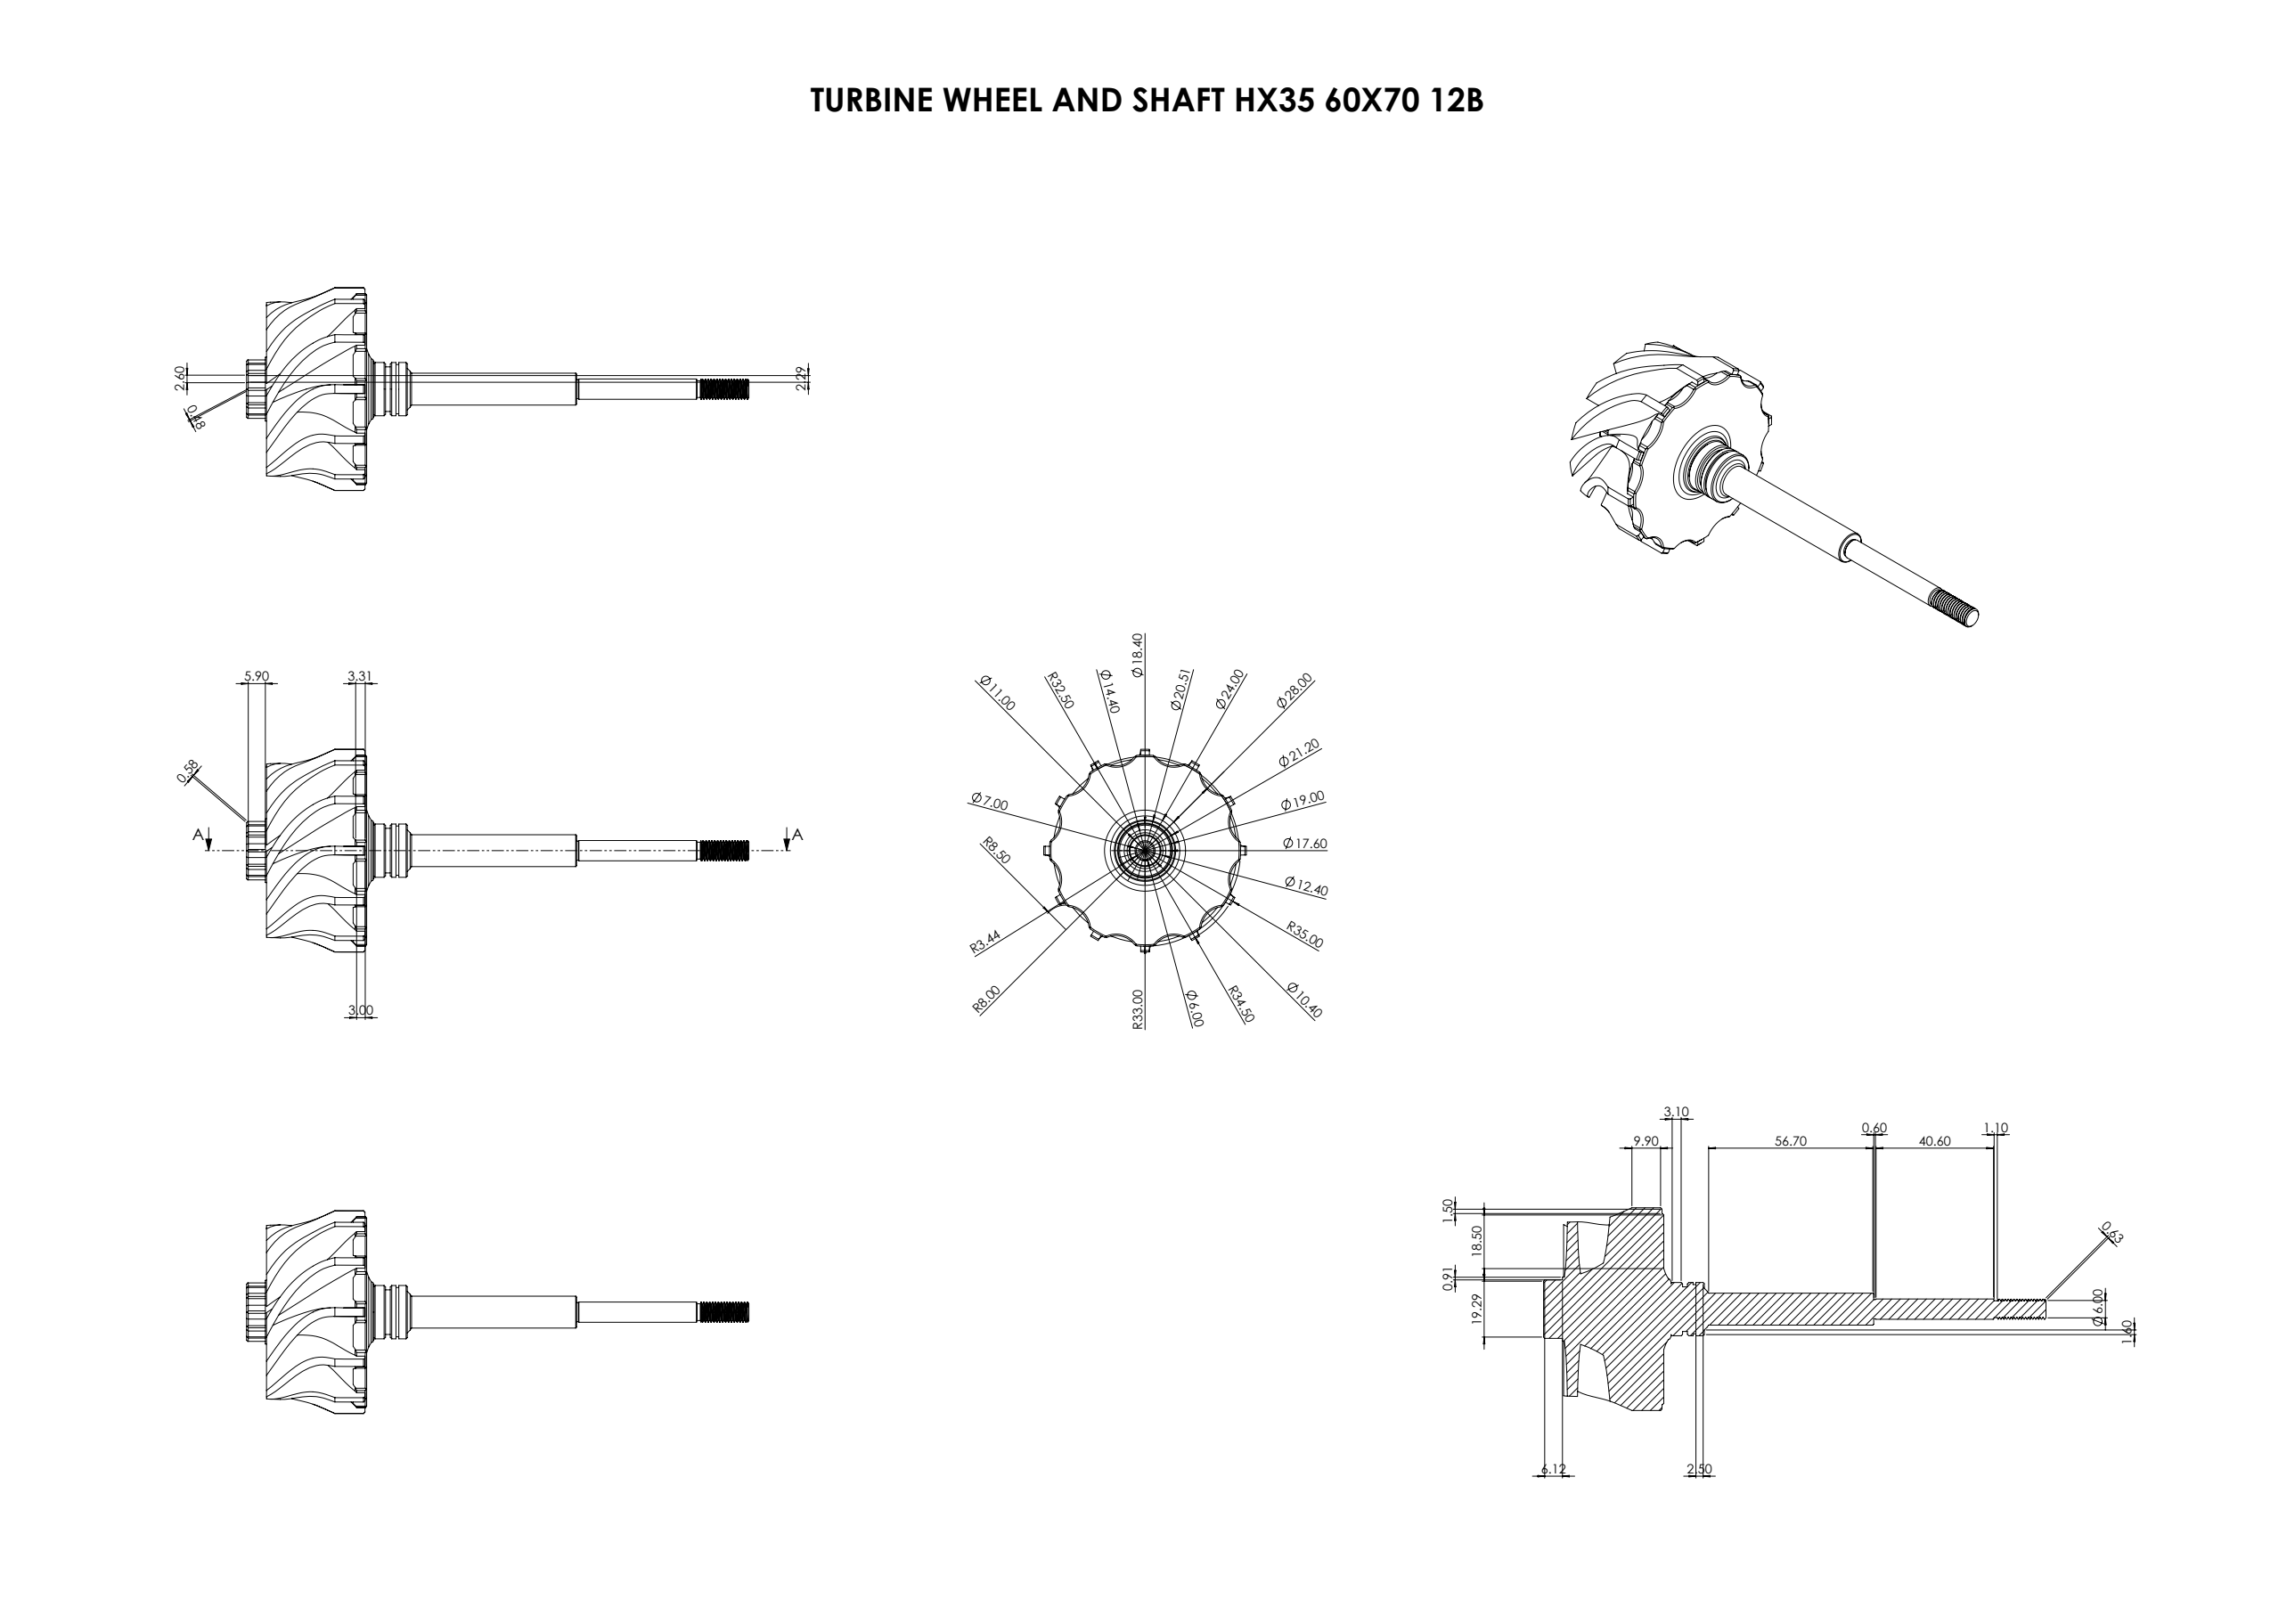
ISO-10303-21;
HEADER;
/* Generated by software containing ST-Developer
 * from STEP Tools, Inc. (www.steptools.com) 
 */

FILE_DESCRIPTION(
/* description */ (''),
/* implementation_level */ '2;1');

FILE_NAME(
/* name */ '01_Turbine_Wheel_and_Shaft_HX35_60x70_12B.step',
/* time_stamp */ '2026-10-25T01:10:36-07:00',
/* author */ (''),
/* organization */ (''),
/* preprocessor_version */ 'ST-DEVELOPER v20.2',
/* originating_system */ 'Autodesk Translation Framework v15.15.0.0',
/* authorisation */ '');

FILE_SCHEMA (('AUTOMOTIVE_DESIGN { 1 0 10303 214 3 1 1 }'));
ENDSEC;

DATA;
#10=MECHANICAL_DESIGN_GEOMETRIC_PRESENTATION_REPRESENTATION('',(#1098,#1099,#1100,#1101,#1102,#1103,#1104,#1105,#1106,#1107,#1108,#1109,#1110,#1111,#1112,#1113,#1114,#1115,#1116,#1117,#1118,#1119,#1120,#1121,#1122,#1123,#1124,#1125,#1126,#1127,#1128,#1129,#1130,#1131,#1132,#1133,#1134,#1135,#1136,#1137,#1138,#1139,#1140,#1141,#1142,#1143,#1144,#1145,#1146,#1147,#1148,#1149,#1150,#1151,#1152,#1153,#1154,#1155,#1156,#1157,#1158,#1159,#1160,#1161,#1162,#1163,#1164,#1165,#1166,#1167,#1168,#1169,#1170,#1171,#1172,#1173,#1174,#1175,#1176,#1177,#1178,#1179,#1180,#1181,#1182,#1183,#1184,#1185,#1186,#1187,#1188,#1189,#1190,#1191,#1192,#1193,#1194,#1195,#1196,#1197,#1198,#1199,#1200,#1201,#1202,#1203,#1204,#1205,#1206,#1207,#1208,#1209,#1210,#1211,#1212,#1213,#1214,#1215,#1216,#1217,#1218,#1219,#1220,#1221,#1222,#1223,#1224,#1225,#1226,#1227,#1228,#1229,#1230,#1231,#1232,#1233,#1234,#1235,#1236,#1237,#1238,#1239,#1240,#1241,#1242,#1243,#1244,#1245,#1246,#1247,#1248,#1249,#1250,#1251,#1252,#1253,#1254,#1255,#1256,#1257,#1258,#1259,#1260,#1261,#1262,#1263,#1264,#1265,#1266,#1267,#1268,#1269,#1270,#1271,#1272,#1273,#1274,#1275,#1276,#1277,#1278,#1279,#1280,#1281,#1282,#1283,#1284,#1285,#1286,#1287,#1288,#1289,#1290,#1291,#1292,#1293,#1294,#1295),#60365);
#67=SHAPE_REPRESENTATION_RELATIONSHIP('SRR','None',#60407,#77);
#77=ADVANCED_BREP_SHAPE_REPRESENTATION('',(#87),#60355);
#87=MANIFOLD_SOLID_BREP('Body1',#18297);
#97=B_SPLINE_SURFACE_WITH_KNOTS('',3,3,((#27482,#27483,#27484,#27485,#27486,
#27487,#27488,#27489,#27490,#27491,#27492,#27493,#27494,#27495,#27496,#27497,
#27498,#27499,#27500,#27501,#27502,#27503,#27504,#27505,#27506,#27507,#27508,
#27509,#27510,#27511,#27512,#27513,#27514,#27515,#27516,#27517,#27518,#27519,
#27520,#27521,#27522,#27523),(#27524,#27525,#27526,#27527,#27528,#27529,
#27530,#27531,#27532,#27533,#27534,#27535,#27536,#27537,#27538,#27539,#27540,
#27541,#27542,#27543,#27544,#27545,#27546,#27547,#27548,#27549,#27550,#27551,
#27552,#27553,#27554,#27555,#27556,#27557,#27558,#27559,#27560,#27561,#27562,
#27563,#27564,#27565),(#27566,#27567,#27568,#27569,#27570,#27571,#27572,
#27573,#27574,#27575,#27576,#27577,#27578,#27579,#27580,#27581,#27582,#27583,
#27584,#27585,#27586,#27587,#27588,#27589,#27590,#27591,#27592,#27593,#27594,
#27595,#27596,#27597,#27598,#27599,#27600,#27601,#27602,#27603,#27604,#27605,
#27606,#27607),(#27608,#27609,#27610,#27611,#27612,#27613,#27614,#27615,
#27616,#27617,#27618,#27619,#27620,#27621,#27622,#27623,#27624,#27625,#27626,
#27627,#27628,#27629,#27630,#27631,#27632,#27633,#27634,#27635,#27636,#27637,
#27638,#27639,#27640,#27641,#27642,#27643,#27644,#27645,#27646,#27647,#27648,
#27649),(#27650,#27651,#27652,#27653,#27654,#27655,#27656,#27657,#27658,
#27659,#27660,#27661,#27662,#27663,#27664,#27665,#27666,#27667,#27668,#27669,
#27670,#27671,#27672,#27673,#27674,#27675,#27676,#27677,#27678,#27679,#27680,
#27681,#27682,#27683,#27684,#27685,#27686,#27687,#27688,#27689,#27690,#27691)),
 .UNSPECIFIED.,.F.,.F.,.F.,(4,1,4),(4,2,2,2,2,2,1,1,2,1,1,1,1,1,1,2,1,2,
1,1,1,1,2,1,1,1,1,1,1,1,4),(0.10381731230502,0.585202227283102,0.946240913516665),
(0.0903575719412648,0.100793262783688,0.212043315812054,0.313257792411489,
0.405143101782566,0.488664067632647,0.50778607271066,0.526908077788674,
0.565152087944702,0.574062129417373,0.582972170890044,0.600792253835385,
0.618612336780727,0.627522378253398,0.631977398989734,0.636432419726069,
0.66210667165326,0.704897091531912,0.716247203396069,0.727597315260226,
0.736109899158344,0.750297538988541,0.79569798644517,0.806906221911025,
0.815312398510416,0.81811445737688,0.840530928308591,0.851739163774446,
0.874155634706157,0.885363870172012,0.975029753898854),.UNSPECIFIED.);
#98=B_SPLINE_SURFACE_WITH_KNOTS('',3,3,((#27985,#27986,#27987,#27988,#27989,
#27990,#27991,#27992,#27993,#27994,#27995,#27996,#27997,#27998,#27999,#28000,
#28001,#28002,#28003,#28004,#28005,#28006,#28007,#28008,#28009,#28010,#28011,
#28012,#28013,#28014,#28015,#28016,#28017,#28018,#28019,#28020,#28021,#28022),
(#28023,#28024,#28025,#28026,#28027,#28028,#28029,#28030,#28031,#28032,
#28033,#28034,#28035,#28036,#28037,#28038,#28039,#28040,#28041,#28042,#28043,
#28044,#28045,#28046,#28047,#28048,#28049,#28050,#28051,#28052,#28053,#28054,
#28055,#28056,#28057,#28058,#28059,#28060),(#28061,#28062,#28063,#28064,
#28065,#28066,#28067,#28068,#28069,#28070,#28071,#28072,#28073,#28074,#28075,
#28076,#28077,#28078,#28079,#28080,#28081,#28082,#28083,#28084,#28085,#28086,
#28087,#28088,#28089,#28090,#28091,#28092,#28093,#28094,#28095,#28096,#28097,
#28098),(#28099,#28100,#28101,#28102,#28103,#28104,#28105,#28106,#28107,
#28108,#28109,#28110,#28111,#28112,#28113,#28114,#28115,#28116,#28117,#28118,
#28119,#28120,#28121,#28122,#28123,#28124,#28125,#28126,#28127,#28128,#28129,
#28130,#28131,#28132,#28133,#28134,#28135,#28136),(#28137,#28138,#28139,
#28140,#28141,#28142,#28143,#28144,#28145,#28146,#28147,#28148,#28149,#28150,
#28151,#28152,#28153,#28154,#28155,#28156,#28157,#28158,#28159,#28160,#28161,
#28162,#28163,#28164,#28165,#28166,#28167,#28168,#28169,#28170,#28171,#28172,
#28173,#28174)),.UNSPECIFIED.,.F.,.F.,.F.,(4,1,4),(4,2,2,2,2,2,1,1,2,1,
1,1,1,1,2,1,2,1,1,1,2,1,1,1,1,1,4),(0.10381731230502,0.464855998538582,
0.946240913516665),(0.0903575719412648,0.100793262783688,0.212043315812054,
0.313257792411489,0.405143101782566,0.488664067632647,0.50778607271066,
0.526908077788674,0.565152087944702,0.574062129417373,0.582972170890044,
0.600792253835385,0.609702295308056,0.618612336780727,0.636432419726069,
0.65354858767753,0.704897091531912,0.716247203396069,0.727597315260226,
0.750297538988541,0.79569798644517,0.806906221911025,0.81811445737688,0.840530928308591,
0.862947399240301,0.885363870172012,0.975029753898854),.UNSPECIFIED.);
#99=B_SPLINE_SURFACE_WITH_KNOTS('',3,3,((#28427,#28428,#28429,#28430,#28431,
#28432,#28433,#28434,#28435,#28436,#28437,#28438,#28439,#28440,#28441,#28442,
#28443,#28444,#28445,#28446,#28447,#28448,#28449,#28450,#28451,#28452,#28453,
#28454,#28455,#28456,#28457,#28458,#28459,#28460,#28461,#28462,#28463,#28464,
#28465,#28466,#28467,#28468,#28469,#28470),(#28471,#28472,#28473,#28474,
#28475,#28476,#28477,#28478,#28479,#28480,#28481,#28482,#28483,#28484,#28485,
#28486,#28487,#28488,#28489,#28490,#28491,#28492,#28493,#28494,#28495,#28496,
#28497,#28498,#28499,#28500,#28501,#28502,#28503,#28504,#28505,#28506,#28507,
#28508,#28509,#28510,#28511,#28512,#28513,#28514),(#28515,#28516,#28517,
#28518,#28519,#28520,#28521,#28522,#28523,#28524,#28525,#28526,#28527,#28528,
#28529,#28530,#28531,#28532,#28533,#28534,#28535,#28536,#28537,#28538,#28539,
#28540,#28541,#28542,#28543,#28544,#28545,#28546,#28547,#28548,#28549,#28550,
#28551,#28552,#28553,#28554,#28555,#28556,#28557,#28558),(#28559,#28560,
#28561,#28562,#28563,#28564,#28565,#28566,#28567,#28568,#28569,#28570,#28571,
#28572,#28573,#28574,#28575,#28576,#28577,#28578,#28579,#28580,#28581,#28582,
#28583,#28584,#28585,#28586,#28587,#28588,#28589,#28590,#28591,#28592,#28593,
#28594,#28595,#28596,#28597,#28598,#28599,#28600,#28601,#28602),(#28603,
#28604,#28605,#28606,#28607,#28608,#28609,#28610,#28611,#28612,#28613,#28614,
#28615,#28616,#28617,#28618,#28619,#28620,#28621,#28622,#28623,#28624,#28625,
#28626,#28627,#28628,#28629,#28630,#28631,#28632,#28633,#28634,#28635,#28636,
#28637,#28638,#28639,#28640,#28641,#28642,#28643,#28644,#28645,#28646)),
 .UNSPECIFIED.,.F.,.F.,.F.,(4,1,4),(4,2,2,2,2,2,1,1,1,2,1,1,1,1,1,1,1,2,
1,2,1,1,1,1,1,2,1,1,1,1,1,1,4),(0.10381731230502,0.464855998538582,0.946240913516665),
(0.0903575719412648,0.100793262783688,0.212043315812054,0.313257792411489,
0.405143101782566,0.488664067632647,0.50778607271066,0.526908077788674,
0.546030082866688,0.565152087944702,0.574062129417373,0.582972170890044,
0.600792253835385,0.609702295308056,0.618612336780727,0.627522378253398,
0.631977398989734,0.636432419726069,0.670664755628991,0.704897091531912,
0.71057214746399,0.716247203396069,0.727597315260226,0.738947427124383,
0.750297538988541,0.79569798644517,0.806906221911025,0.81811445737688,0.829322692842735,
0.840530928308591,0.862947399240301,0.885363870172012,0.975029753898854),
 .UNSPECIFIED.);
#100=B_SPLINE_SURFACE_WITH_KNOTS('',3,3,((#28899,#28900,#28901,#28902,#28903,
#28904,#28905,#28906,#28907,#28908,#28909,#28910,#28911,#28912,#28913,#28914,
#28915,#28916,#28917,#28918,#28919,#28920,#28921,#28922,#28923,#28924,#28925,
#28926,#28927,#28928,#28929,#28930,#28931,#28932,#28933,#28934,#28935,#28936,
#28937,#28938,#28939,#28940),(#28941,#28942,#28943,#28944,#28945,#28946,
#28947,#28948,#28949,#28950,#28951,#28952,#28953,#28954,#28955,#28956,#28957,
#28958,#28959,#28960,#28961,#28962,#28963,#28964,#28965,#28966,#28967,#28968,
#28969,#28970,#28971,#28972,#28973,#28974,#28975,#28976,#28977,#28978,#28979,
#28980,#28981,#28982),(#28983,#28984,#28985,#28986,#28987,#28988,#28989,
#28990,#28991,#28992,#28993,#28994,#28995,#28996,#28997,#28998,#28999,#29000,
#29001,#29002,#29003,#29004,#29005,#29006,#29007,#29008,#29009,#29010,#29011,
#29012,#29013,#29014,#29015,#29016,#29017,#29018,#29019,#29020,#29021,#29022,
#29023,#29024),(#29025,#29026,#29027,#29028,#29029,#29030,#29031,#29032,
#29033,#29034,#29035,#29036,#29037,#29038,#29039,#29040,#29041,#29042,#29043,
#29044,#29045,#29046,#29047,#29048,#29049,#29050,#29051,#29052,#29053,#29054,
#29055,#29056,#29057,#29058,#29059,#29060,#29061,#29062,#29063,#29064,#29065,
#29066),(#29067,#29068,#29069,#29070,#29071,#29072,#29073,#29074,#29075,
#29076,#29077,#29078,#29079,#29080,#29081,#29082,#29083,#29084,#29085,#29086,
#29087,#29088,#29089,#29090,#29091,#29092,#29093,#29094,#29095,#29096,#29097,
#29098,#29099,#29100,#29101,#29102,#29103,#29104,#29105,#29106,#29107,#29108)),
 .UNSPECIFIED.,.F.,.F.,.F.,(4,1,4),(4,2,2,2,2,2,1,1,2,1,1,1,1,1,1,2,1,2,
1,1,1,1,2,1,1,1,1,1,1,1,4),(0.10381731230502,0.585202227283103,0.946240913516665),
(0.0903575719412648,0.100793262783688,0.212043315812054,0.313257792411489,
0.405143101782566,0.488664067632647,0.50778607271066,0.526908077788674,
0.565152087944702,0.574062129417373,0.582972170890044,0.600792253835385,
0.618612336780727,0.627522378253398,0.631977398989734,0.636432419726069,
0.66210667165326,0.704897091531912,0.716247203396069,0.727597315260226,
0.736109899158344,0.750297538988541,0.79569798644517,0.806906221911025,
0.815312398510416,0.81811445737688,0.840530928308591,0.851739163774446,
0.874155634706157,0.885363870172012,0.975029753898854),.UNSPECIFIED.);
#101=B_SPLINE_SURFACE_WITH_KNOTS('',3,3,((#29355,#29356,#29357,#29358,#29359,
#29360,#29361,#29362,#29363,#29364,#29365,#29366,#29367,#29368,#29369,#29370,
#29371,#29372,#29373,#29374,#29375,#29376,#29377,#29378,#29379,#29380,#29381,
#29382,#29383,#29384,#29385,#29386,#29387,#29388,#29389,#29390,#29391,#29392),
(#29393,#29394,#29395,#29396,#29397,#29398,#29399,#29400,#29401,#29402,
#29403,#29404,#29405,#29406,#29407,#29408,#29409,#29410,#29411,#29412,#29413,
#29414,#29415,#29416,#29417,#29418,#29419,#29420,#29421,#29422,#29423,#29424,
#29425,#29426,#29427,#29428,#29429,#29430),(#29431,#29432,#29433,#29434,
#29435,#29436,#29437,#29438,#29439,#29440,#29441,#29442,#29443,#29444,#29445,
#29446,#29447,#29448,#29449,#29450,#29451,#29452,#29453,#29454,#29455,#29456,
#29457,#29458,#29459,#29460,#29461,#29462,#29463,#29464,#29465,#29466,#29467,
#29468),(#29469,#29470,#29471,#29472,#29473,#29474,#29475,#29476,#29477,
#29478,#29479,#29480,#29481,#29482,#29483,#29484,#29485,#29486,#29487,#29488,
#29489,#29490,#29491,#29492,#29493,#29494,#29495,#29496,#29497,#29498,#29499,
#29500,#29501,#29502,#29503,#29504,#29505,#29506),(#29507,#29508,#29509,
#29510,#29511,#29512,#29513,#29514,#29515,#29516,#29517,#29518,#29519,#29520,
#29521,#29522,#29523,#29524,#29525,#29526,#29527,#29528,#29529,#29530,#29531,
#29532,#29533,#29534,#29535,#29536,#29537,#29538,#29539,#29540,#29541,#29542,
#29543,#29544)),.UNSPECIFIED.,.F.,.F.,.F.,(4,1,4),(4,2,2,2,2,2,1,1,2,1,
1,1,1,1,2,1,2,1,1,1,2,1,1,1,1,1,4),(0.10381731230502,0.464855998538582,
0.946240913516665),(0.0903575719412648,0.100793262783688,0.212043315812054,
0.313257792411489,0.405143101782566,0.488664067632647,0.50778607271066,
0.526908077788674,0.565152087944702,0.574062129417373,0.582972170890044,
0.600792253835385,0.609702295308056,0.618612336780727,0.636432419726069,
0.65354858767753,0.704897091531912,0.716247203396069,0.727597315260226,
0.750297538988541,0.79569798644517,0.806906221911025,0.81811445737688,0.840530928308591,
0.862947399240301,0.885363870172012,0.975029753898854),.UNSPECIFIED.);
#102=B_SPLINE_SURFACE_WITH_KNOTS('',3,3,((#29797,#29798,#29799,#29800,#29801,
#29802,#29803,#29804,#29805,#29806,#29807,#29808,#29809,#29810,#29811,#29812,
#29813,#29814,#29815,#29816,#29817,#29818,#29819,#29820,#29821,#29822,#29823,
#29824,#29825,#29826,#29827,#29828,#29829,#29830,#29831,#29832,#29833,#29834,
#29835,#29836,#29837,#29838,#29839,#29840),(#29841,#29842,#29843,#29844,
#29845,#29846,#29847,#29848,#29849,#29850,#29851,#29852,#29853,#29854,#29855,
#29856,#29857,#29858,#29859,#29860,#29861,#29862,#29863,#29864,#29865,#29866,
#29867,#29868,#29869,#29870,#29871,#29872,#29873,#29874,#29875,#29876,#29877,
#29878,#29879,#29880,#29881,#29882,#29883,#29884),(#29885,#29886,#29887,
#29888,#29889,#29890,#29891,#29892,#29893,#29894,#29895,#29896,#29897,#29898,
#29899,#29900,#29901,#29902,#29903,#29904,#29905,#29906,#29907,#29908,#29909,
#29910,#29911,#29912,#29913,#29914,#29915,#29916,#29917,#29918,#29919,#29920,
#29921,#29922,#29923,#29924,#29925,#29926,#29927,#29928),(#29929,#29930,
#29931,#29932,#29933,#29934,#29935,#29936,#29937,#29938,#29939,#29940,#29941,
#29942,#29943,#29944,#29945,#29946,#29947,#29948,#29949,#29950,#29951,#29952,
#29953,#29954,#29955,#29956,#29957,#29958,#29959,#29960,#29961,#29962,#29963,
#29964,#29965,#29966,#29967,#29968,#29969,#29970,#29971,#29972),(#29973,
#29974,#29975,#29976,#29977,#29978,#29979,#29980,#29981,#29982,#29983,#29984,
#29985,#29986,#29987,#29988,#29989,#29990,#29991,#29992,#29993,#29994,#29995,
#29996,#29997,#29998,#29999,#30000,#30001,#30002,#30003,#30004,#30005,#30006,
#30007,#30008,#30009,#30010,#30011,#30012,#30013,#30014,#30015,#30016)),
 .UNSPECIFIED.,.F.,.F.,.F.,(4,1,4),(4,2,2,2,2,2,1,1,1,2,1,1,1,1,1,1,1,2,
1,2,1,1,1,1,1,2,1,1,1,1,1,1,4),(0.10381731230502,0.585202227283102,0.946240913516665),
(0.0903575719412648,0.100793262783688,0.212043315812054,0.313257792411489,
0.405143101782566,0.488664067632647,0.50778607271066,0.526908077788674,
0.546030082866688,0.565152087944702,0.574062129417373,0.582972170890044,
0.600792253835385,0.609702295308056,0.618612336780727,0.627522378253398,
0.631977398989734,0.636432419726069,0.670664755628991,0.704897091531912,
0.71057214746399,0.716247203396069,0.727597315260226,0.738947427124383,
0.750297538988541,0.79569798644517,0.806906221911025,0.81811445737688,0.829322692842735,
0.840530928308591,0.862947399240301,0.885363870172012,0.975029753898854),
 .UNSPECIFIED.);
#103=B_SPLINE_SURFACE_WITH_KNOTS('',3,3,((#30269,#30270,#30271,#30272,#30273,
#30274,#30275,#30276,#30277,#30278,#30279,#30280,#30281,#30282,#30283,#30284,
#30285,#30286,#30287,#30288,#30289,#30290,#30291,#30292,#30293,#30294,#30295,
#30296,#30297,#30298,#30299,#30300,#30301,#30302,#30303,#30304,#30305,#30306,
#30307,#30308,#30309,#30310),(#30311,#30312,#30313,#30314,#30315,#30316,
#30317,#30318,#30319,#30320,#30321,#30322,#30323,#30324,#30325,#30326,#30327,
#30328,#30329,#30330,#30331,#30332,#30333,#30334,#30335,#30336,#30337,#30338,
#30339,#30340,#30341,#30342,#30343,#30344,#30345,#30346,#30347,#30348,#30349,
#30350,#30351,#30352),(#30353,#30354,#30355,#30356,#30357,#30358,#30359,
#30360,#30361,#30362,#30363,#30364,#30365,#30366,#30367,#30368,#30369,#30370,
#30371,#30372,#30373,#30374,#30375,#30376,#30377,#30378,#30379,#30380,#30381,
#30382,#30383,#30384,#30385,#30386,#30387,#30388,#30389,#30390,#30391,#30392,
#30393,#30394),(#30395,#30396,#30397,#30398,#30399,#30400,#30401,#30402,
#30403,#30404,#30405,#30406,#30407,#30408,#30409,#30410,#30411,#30412,#30413,
#30414,#30415,#30416,#30417,#30418,#30419,#30420,#30421,#30422,#30423,#30424,
#30425,#30426,#30427,#30428,#30429,#30430,#30431,#30432,#30433,#30434,#30435,
#30436),(#30437,#30438,#30439,#30440,#30441,#30442,#30443,#30444,#30445,
#30446,#30447,#30448,#30449,#30450,#30451,#30452,#30453,#30454,#30455,#30456,
#30457,#30458,#30459,#30460,#30461,#30462,#30463,#30464,#30465,#30466,#30467,
#30468,#30469,#30470,#30471,#30472,#30473,#30474,#30475,#30476,#30477,#30478)),
 .UNSPECIFIED.,.F.,.F.,.F.,(4,1,4),(4,2,2,2,2,2,1,1,2,1,1,1,1,1,1,2,1,2,
1,1,1,1,2,1,1,1,1,1,1,1,4),(0.10381731230502,0.585202227283102,0.946240913516665),
(0.0903575719412648,0.100793262783688,0.212043315812054,0.313257792411489,
0.405143101782566,0.488664067632647,0.50778607271066,0.526908077788674,
0.565152087944702,0.574062129417373,0.582972170890044,0.600792253835385,
0.618612336780727,0.627522378253398,0.631977398989734,0.636432419726069,
0.66210667165326,0.704897091531912,0.716247203396069,0.727597315260226,
0.736109899158344,0.750297538988541,0.79569798644517,0.806906221911025,
0.815312398510416,0.81811445737688,0.840530928308591,0.851739163774446,
0.874155634706157,0.885363870172012,0.975029753898854),.UNSPECIFIED.);
#104=B_SPLINE_SURFACE_WITH_KNOTS('',3,3,((#30725,#30726,#30727,#30728,#30729,
#30730,#30731,#30732,#30733,#30734,#30735,#30736,#30737,#30738,#30739,#30740,
#30741,#30742,#30743,#30744,#30745,#30746,#30747,#30748,#30749,#30750,#30751,
#30752,#30753,#30754,#30755,#30756,#30757,#30758,#30759,#30760,#30761,#30762),
(#30763,#30764,#30765,#30766,#30767,#30768,#30769,#30770,#30771,#30772,
#30773,#30774,#30775,#30776,#30777,#30778,#30779,#30780,#30781,#30782,#30783,
#30784,#30785,#30786,#30787,#30788,#30789,#30790,#30791,#30792,#30793,#30794,
#30795,#30796,#30797,#30798,#30799,#30800),(#30801,#30802,#30803,#30804,
#30805,#30806,#30807,#30808,#30809,#30810,#30811,#30812,#30813,#30814,#30815,
#30816,#30817,#30818,#30819,#30820,#30821,#30822,#30823,#30824,#30825,#30826,
#30827,#30828,#30829,#30830,#30831,#30832,#30833,#30834,#30835,#30836,#30837,
#30838),(#30839,#30840,#30841,#30842,#30843,#30844,#30845,#30846,#30847,
#30848,#30849,#30850,#30851,#30852,#30853,#30854,#30855,#30856,#30857,#30858,
#30859,#30860,#30861,#30862,#30863,#30864,#30865,#30866,#30867,#30868,#30869,
#30870,#30871,#30872,#30873,#30874,#30875,#30876),(#30877,#30878,#30879,
#30880,#30881,#30882,#30883,#30884,#30885,#30886,#30887,#30888,#30889,#30890,
#30891,#30892,#30893,#30894,#30895,#30896,#30897,#30898,#30899,#30900,#30901,
#30902,#30903,#30904,#30905,#30906,#30907,#30908,#30909,#30910,#30911,#30912,
#30913,#30914)),.UNSPECIFIED.,.F.,.F.,.F.,(4,1,4),(4,2,2,2,2,2,1,1,2,1,
1,1,1,1,2,1,2,1,1,1,2,1,1,1,1,1,4),(0.10381731230502,0.464855998538582,
0.946240913516665),(0.0903575719412648,0.100793262783688,0.212043315812054,
0.313257792411489,0.405143101782566,0.488664067632647,0.50778607271066,
0.526908077788674,0.565152087944702,0.574062129417373,0.582972170890044,
0.600792253835385,0.609702295308056,0.618612336780727,0.636432419726069,
0.65354858767753,0.704897091531912,0.716247203396069,0.727597315260226,
0.750297538988541,0.79569798644517,0.806906221911025,0.81811445737688,0.840530928308591,
0.862947399240301,0.885363870172012,0.975029753898854),.UNSPECIFIED.);
#105=B_SPLINE_SURFACE_WITH_KNOTS('',3,3,((#31167,#31168,#31169,#31170,#31171,
#31172,#31173,#31174,#31175,#31176,#31177,#31178,#31179,#31180,#31181,#31182,
#31183,#31184,#31185,#31186,#31187,#31188,#31189,#31190,#31191,#31192,#31193,
#31194,#31195,#31196,#31197,#31198,#31199,#31200,#31201,#31202,#31203,#31204,
#31205,#31206,#31207,#31208,#31209,#31210),(#31211,#31212,#31213,#31214,
#31215,#31216,#31217,#31218,#31219,#31220,#31221,#31222,#31223,#31224,#31225,
#31226,#31227,#31228,#31229,#31230,#31231,#31232,#31233,#31234,#31235,#31236,
#31237,#31238,#31239,#31240,#31241,#31242,#31243,#31244,#31245,#31246,#31247,
#31248,#31249,#31250,#31251,#31252,#31253,#31254),(#31255,#31256,#31257,
#31258,#31259,#31260,#31261,#31262,#31263,#31264,#31265,#31266,#31267,#31268,
#31269,#31270,#31271,#31272,#31273,#31274,#31275,#31276,#31277,#31278,#31279,
#31280,#31281,#31282,#31283,#31284,#31285,#31286,#31287,#31288,#31289,#31290,
#31291,#31292,#31293,#31294,#31295,#31296,#31297,#31298),(#31299,#31300,
#31301,#31302,#31303,#31304,#31305,#31306,#31307,#31308,#31309,#31310,#31311,
#31312,#31313,#31314,#31315,#31316,#31317,#31318,#31319,#31320,#31321,#31322,
#31323,#31324,#31325,#31326,#31327,#31328,#31329,#31330,#31331,#31332,#31333,
#31334,#31335,#31336,#31337,#31338,#31339,#31340,#31341,#31342),(#31343,
#31344,#31345,#31346,#31347,#31348,#31349,#31350,#31351,#31352,#31353,#31354,
#31355,#31356,#31357,#31358,#31359,#31360,#31361,#31362,#31363,#31364,#31365,
#31366,#31367,#31368,#31369,#31370,#31371,#31372,#31373,#31374,#31375,#31376,
#31377,#31378,#31379,#31380,#31381,#31382,#31383,#31384,#31385,#31386)),
 .UNSPECIFIED.,.F.,.F.,.F.,(4,1,4),(4,2,2,2,2,2,1,1,1,2,1,1,1,1,1,1,1,2,
1,2,1,1,1,1,1,2,1,1,1,1,1,1,4),(0.10381731230502,0.464855998538582,0.946240913516665),
(0.0903575719412648,0.100793262783688,0.212043315812054,0.313257792411489,
0.405143101782566,0.488664067632647,0.50778607271066,0.526908077788674,
0.546030082866688,0.565152087944702,0.574062129417373,0.582972170890044,
0.600792253835385,0.609702295308056,0.618612336780727,0.627522378253398,
0.631977398989734,0.636432419726069,0.670664755628991,0.704897091531912,
0.71057214746399,0.716247203396069,0.727597315260226,0.738947427124383,
0.750297538988541,0.79569798644517,0.806906221911025,0.81811445737688,0.829322692842735,
0.840530928308591,0.862947399240301,0.885363870172012,0.975029753898854),
 .UNSPECIFIED.);
#106=B_SPLINE_SURFACE_WITH_KNOTS('',3,3,((#31639,#31640,#31641,#31642,#31643,
#31644,#31645,#31646,#31647,#31648,#31649,#31650,#31651,#31652,#31653,#31654,
#31655,#31656,#31657,#31658,#31659,#31660,#31661,#31662,#31663,#31664,#31665,
#31666,#31667,#31668,#31669,#31670,#31671,#31672,#31673,#31674,#31675,#31676,
#31677,#31678,#31679,#31680),(#31681,#31682,#31683,#31684,#31685,#31686,
#31687,#31688,#31689,#31690,#31691,#31692,#31693,#31694,#31695,#31696,#31697,
#31698,#31699,#31700,#31701,#31702,#31703,#31704,#31705,#31706,#31707,#31708,
#31709,#31710,#31711,#31712,#31713,#31714,#31715,#31716,#31717,#31718,#31719,
#31720,#31721,#31722),(#31723,#31724,#31725,#31726,#31727,#31728,#31729,
#31730,#31731,#31732,#31733,#31734,#31735,#31736,#31737,#31738,#31739,#31740,
#31741,#31742,#31743,#31744,#31745,#31746,#31747,#31748,#31749,#31750,#31751,
#31752,#31753,#31754,#31755,#31756,#31757,#31758,#31759,#31760,#31761,#31762,
#31763,#31764),(#31765,#31766,#31767,#31768,#31769,#31770,#31771,#31772,
#31773,#31774,#31775,#31776,#31777,#31778,#31779,#31780,#31781,#31782,#31783,
#31784,#31785,#31786,#31787,#31788,#31789,#31790,#31791,#31792,#31793,#31794,
#31795,#31796,#31797,#31798,#31799,#31800,#31801,#31802,#31803,#31804,#31805,
#31806),(#31807,#31808,#31809,#31810,#31811,#31812,#31813,#31814,#31815,
#31816,#31817,#31818,#31819,#31820,#31821,#31822,#31823,#31824,#31825,#31826,
#31827,#31828,#31829,#31830,#31831,#31832,#31833,#31834,#31835,#31836,#31837,
#31838,#31839,#31840,#31841,#31842,#31843,#31844,#31845,#31846,#31847,#31848)),
 .UNSPECIFIED.,.F.,.F.,.F.,(4,1,4),(4,2,2,2,2,2,1,1,2,1,1,1,1,1,1,2,1,2,
1,1,1,1,2,1,1,1,1,1,1,1,4),(0.10381731230502,0.464855998538582,0.946240913516665),
(0.0903575719412648,0.100793262783688,0.212043315812054,0.313257792411489,
0.405143101782566,0.488664067632647,0.50778607271066,0.526908077788674,
0.565152087944702,0.574062129417373,0.582972170890044,0.600792253835385,
0.618612336780727,0.627522378253398,0.631977398989734,0.636432419726069,
0.66210667165326,0.704897091531912,0.716247203396069,0.727597315260226,
0.736109899158344,0.750297538988541,0.79569798644517,0.806906221911025,
0.815312398510416,0.81811445737688,0.840530928308591,0.851739163774446,
0.874155634706157,0.885363870172012,0.975029753898854),.UNSPECIFIED.);
#107=B_SPLINE_SURFACE_WITH_KNOTS('',3,3,((#32095,#32096,#32097,#32098,#32099,
#32100,#32101,#32102,#32103,#32104,#32105,#32106,#32107,#32108,#32109,#32110,
#32111,#32112,#32113,#32114,#32115,#32116,#32117,#32118,#32119,#32120,#32121,
#32122,#32123,#32124,#32125,#32126,#32127,#32128,#32129,#32130,#32131,#32132),
(#32133,#32134,#32135,#32136,#32137,#32138,#32139,#32140,#32141,#32142,
#32143,#32144,#32145,#32146,#32147,#32148,#32149,#32150,#32151,#32152,#32153,
#32154,#32155,#32156,#32157,#32158,#32159,#32160,#32161,#32162,#32163,#32164,
#32165,#32166,#32167,#32168,#32169,#32170),(#32171,#32172,#32173,#32174,
#32175,#32176,#32177,#32178,#32179,#32180,#32181,#32182,#32183,#32184,#32185,
#32186,#32187,#32188,#32189,#32190,#32191,#32192,#32193,#32194,#32195,#32196,
#32197,#32198,#32199,#32200,#32201,#32202,#32203,#32204,#32205,#32206,#32207,
#32208),(#32209,#32210,#32211,#32212,#32213,#32214,#32215,#32216,#32217,
#32218,#32219,#32220,#32221,#32222,#32223,#32224,#32225,#32226,#32227,#32228,
#32229,#32230,#32231,#32232,#32233,#32234,#32235,#32236,#32237,#32238,#32239,
#32240,#32241,#32242,#32243,#32244,#32245,#32246),(#32247,#32248,#32249,
#32250,#32251,#32252,#32253,#32254,#32255,#32256,#32257,#32258,#32259,#32260,
#32261,#32262,#32263,#32264,#32265,#32266,#32267,#32268,#32269,#32270,#32271,
#32272,#32273,#32274,#32275,#32276,#32277,#32278,#32279,#32280,#32281,#32282,
#32283,#32284)),.UNSPECIFIED.,.F.,.F.,.F.,(4,1,4),(4,2,2,2,2,2,1,1,2,1,
1,1,1,1,2,1,2,1,1,1,2,1,1,1,1,1,4),(0.10381731230502,0.464855998538582,
0.946240913516665),(0.0903575719412648,0.100793262783688,0.212043315812054,
0.313257792411489,0.405143101782566,0.488664067632647,0.50778607271066,
0.526908077788674,0.565152087944702,0.574062129417373,0.582972170890044,
0.600792253835385,0.609702295308056,0.618612336780727,0.636432419726069,
0.65354858767753,0.704897091531912,0.716247203396069,0.727597315260226,
0.750297538988541,0.79569798644517,0.806906221911025,0.81811445737688,0.840530928308591,
0.862947399240301,0.885363870172012,0.975029753898854),.UNSPECIFIED.);
#108=B_SPLINE_SURFACE_WITH_KNOTS('',3,3,((#32537,#32538,#32539,#32540,#32541,
#32542,#32543,#32544,#32545,#32546,#32547,#32548,#32549,#32550,#32551,#32552,
#32553,#32554,#32555,#32556,#32557,#32558,#32559,#32560,#32561,#32562,#32563,
#32564,#32565,#32566,#32567,#32568,#32569,#32570,#32571,#32572,#32573,#32574,
#32575,#32576,#32577,#32578,#32579,#32580),(#32581,#32582,#32583,#32584,
#32585,#32586,#32587,#32588,#32589,#32590,#32591,#32592,#32593,#32594,#32595,
#32596,#32597,#32598,#32599,#32600,#32601,#32602,#32603,#32604,#32605,#32606,
#32607,#32608,#32609,#32610,#32611,#32612,#32613,#32614,#32615,#32616,#32617,
#32618,#32619,#32620,#32621,#32622,#32623,#32624),(#32625,#32626,#32627,
#32628,#32629,#32630,#32631,#32632,#32633,#32634,#32635,#32636,#32637,#32638,
#32639,#32640,#32641,#32642,#32643,#32644,#32645,#32646,#32647,#32648,#32649,
#32650,#32651,#32652,#32653,#32654,#32655,#32656,#32657,#32658,#32659,#32660,
#32661,#32662,#32663,#32664,#32665,#32666,#32667,#32668),(#32669,#32670,
#32671,#32672,#32673,#32674,#32675,#32676,#32677,#32678,#32679,#32680,#32681,
#32682,#32683,#32684,#32685,#32686,#32687,#32688,#32689,#32690,#32691,#32692,
#32693,#32694,#32695,#32696,#32697,#32698,#32699,#32700,#32701,#32702,#32703,
#32704,#32705,#32706,#32707,#32708,#32709,#32710,#32711,#32712),(#32713,
#32714,#32715,#32716,#32717,#32718,#32719,#32720,#32721,#32722,#32723,#32724,
#32725,#32726,#32727,#32728,#32729,#32730,#32731,#32732,#32733,#32734,#32735,
#32736,#32737,#32738,#32739,#32740,#32741,#32742,#32743,#32744,#32745,#32746,
#32747,#32748,#32749,#32750,#32751,#32752,#32753,#32754,#32755,#32756)),
 .UNSPECIFIED.,.F.,.F.,.F.,(4,1,4),(4,2,2,2,2,2,1,1,1,2,1,1,1,1,1,1,1,2,
1,2,1,1,1,1,1,2,1,1,1,1,1,1,4),(0.10381731230502,0.585202227283103,0.946240913516665),
(0.0903575719412648,0.100793262783688,0.212043315812054,0.313257792411489,
0.405143101782566,0.488664067632647,0.50778607271066,0.526908077788674,
0.546030082866688,0.565152087944702,0.574062129417373,0.582972170890044,
0.600792253835385,0.609702295308056,0.618612336780727,0.627522378253398,
0.631977398989734,0.636432419726069,0.670664755628991,0.704897091531912,
0.71057214746399,0.716247203396069,0.727597315260226,0.738947427124383,
0.750297538988541,0.79569798644517,0.806906221911025,0.81811445737688,0.829322692842735,
0.840530928308591,0.862947399240301,0.885363870172012,0.975029753898854),
 .UNSPECIFIED.);
#109=B_SPLINE_SURFACE_WITH_KNOTS('',3,3,((#33831,#33832,#33833,#33834,#33835,
#33836,#33837,#33838,#33839,#33840,#33841,#33842,#33843,#33844,#33845,#33846,
#33847,#33848,#33849,#33850,#33851,#33852,#33853,#33854,#33855,#33856,#33857,
#33858,#33859,#33860,#33861,#33862,#33863,#33864,#33865,#33866,#33867,#33868,
#33869,#33870,#33871,#33872,#33873,#33874,#33875,#33876,#33877,#33878,#33879,
#33880,#33881,#33882,#33883,#33884,#33885,#33886,#33887,#33888,#33889,#33890,
#33891,#33892,#33893,#33894,#33895,#33896,#33897,#33898,#33899,#33900,#33901,
#33902,#33903,#33904,#33905,#33906,#33907,#33908,#33909,#33910,#33911,#33912,
#33913,#33914,#33915,#33916,#33917,#33918,#33919,#33920,#33921,#33922,#33923,
#33924,#33925,#33926,#33927,#33928,#33929,#33930,#33931,#33932,#33933,#33934,
#33935,#33936,#33937),(#33938,#33939,#33940,#33941,#33942,#33943,#33944,
#33945,#33946,#33947,#33948,#33949,#33950,#33951,#33952,#33953,#33954,#33955,
#33956,#33957,#33958,#33959,#33960,#33961,#33962,#33963,#33964,#33965,#33966,
#33967,#33968,#33969,#33970,#33971,#33972,#33973,#33974,#33975,#33976,#33977,
#33978,#33979,#33980,#33981,#33982,#33983,#33984,#33985,#33986,#33987,#33988,
#33989,#33990,#33991,#33992,#33993,#33994,#33995,#33996,#33997,#33998,#33999,
#34000,#34001,#34002,#34003,#34004,#34005,#34006,#34007,#34008,#34009,#34010,
#34011,#34012,#34013,#34014,#34015,#34016,#34017,#34018,#34019,#34020,#34021,
#34022,#34023,#34024,#34025,#34026,#34027,#34028,#34029,#34030,#34031,#34032,
#34033,#34034,#34035,#34036,#34037,#34038,#34039,#34040,#34041,#34042,#34043,
#34044),(#34045,#34046,#34047,#34048,#34049,#34050,#34051,#34052,#34053,
#34054,#34055,#34056,#34057,#34058,#34059,#34060,#34061,#34062,#34063,#34064,
#34065,#34066,#34067,#34068,#34069,#34070,#34071,#34072,#34073,#34074,#34075,
#34076,#34077,#34078,#34079,#34080,#34081,#34082,#34083,#34084,#34085,#34086,
#34087,#34088,#34089,#34090,#34091,#34092,#34093,#34094,#34095,#34096,#34097,
#34098,#34099,#34100,#34101,#34102,#34103,#34104,#34105,#34106,#34107,#34108,
#34109,#34110,#34111,#34112,#34113,#34114,#34115,#34116,#34117,#34118,#34119,
#34120,#34121,#34122,#34123,#34124,#34125,#34126,#34127,#34128,#34129,#34130,
#34131,#34132,#34133,#34134,#34135,#34136,#34137,#34138,#34139,#34140,#34141,
#34142,#34143,#34144,#34145,#34146,#34147,#34148,#34149,#34150,#34151),
(#34152,#34153,#34154,#34155,#34156,#34157,#34158,#34159,#34160,#34161,
#34162,#34163,#34164,#34165,#34166,#34167,#34168,#34169,#34170,#34171,#34172,
#34173,#34174,#34175,#34176,#34177,#34178,#34179,#34180,#34181,#34182,#34183,
#34184,#34185,#34186,#34187,#34188,#34189,#34190,#34191,#34192,#34193,#34194,
#34195,#34196,#34197,#34198,#34199,#34200,#34201,#34202,#34203,#34204,#34205,
#34206,#34207,#34208,#34209,#34210,#34211,#34212,#34213,#34214,#34215,#34216,
#34217,#34218,#34219,#34220,#34221,#34222,#34223,#34224,#34225,#34226,#34227,
#34228,#34229,#34230,#34231,#34232,#34233,#34234,#34235,#34236,#34237,#34238,
#34239,#34240,#34241,#34242,#34243,#34244,#34245,#34246,#34247,#34248,#34249,
#34250,#34251,#34252,#34253,#34254,#34255,#34256,#34257,#34258)),
 .UNSPECIFIED.,.F.,.F.,.F.,(4,4),(4,1,1,1,1,1,1,1,1,1,1,1,1,1,1,1,1,1,1,
1,1,1,1,1,1,1,1,1,1,1,1,1,1,1,1,1,1,1,1,1,1,1,1,1,1,1,1,1,1,1,1,1,1,1,1,
1,1,1,1,1,1,1,1,1,1,1,1,1,1,1,1,1,1,1,1,1,1,1,1,1,1,1,1,1,1,1,1,1,1,1,1,
1,1,1,1,1,1,1,1,1,1,1,1,1,4),(0.,0.0658179306876168),(8.30838445208336,
9.3001665031586,10.2919485542338,11.2837306053091,12.2755126563843,13.2672947074596,
14.2590767585348,15.25085880961,16.2426408606853,17.2344229117605,18.2262049628358,
19.217987013911,20.2097690649862,21.2015511160615,22.1933331671367,23.185115218212,
24.1768972692872,25.1686793203624,26.1604613714377,27.1522434225129,28.1440254735882,
29.1358075246634,30.1275895757386,31.1193716268139,32.1111536778891,33.1029357289644,
34.0947177800396,35.0864998311148,36.0782818821901,37.0700639332653,38.0618459843406,
39.0536280354158,40.0454100864911,41.0371921375663,42.0289741886415,43.0207562397168,
44.012538290792,45.0043203418673,45.9961023929425,46.9878844440177,47.979666495093,
48.9714485461682,49.9632305972435,50.9550126483187,51.9467946993939,52.9385767504692,
53.9303588015444,54.9221408526197,55.9139229036949,56.9057049547701,57.8974870058454,
58.8892690569206,59.8810511079959,60.8728331590711,61.8646152101463,62.8563972612216,
63.8481793122968,64.8399613633721,65.8317434144473,66.8235254655226,67.8153075165978,
68.807089567673,69.7988716187483,70.7906536698235,71.7824357208987,72.774217771974,
73.7659998230492,74.7577818741245,75.7495639251997,76.741345976275,77.7331280273502,
78.7249100784254,79.7166921295007,80.7084741805759,81.7002562316512,82.6920382827264,
83.6838203338016,84.6756023848769,85.6673844359521,86.6591664870274,87.6509485381026,
88.6427305891778,89.6345126402531,90.6262946913283,91.6180767424036,92.6098587934788,
93.601640844554,94.5934228956293,95.5852049467045,96.5769869977798,97.568769048855,
98.5605510999303,99.5523331510055,100.544115202081,101.535897253156,102.527679304231,
103.519461355306,104.511243406382,105.503025457457,106.494807508532,107.486589559607,
108.478371610683,109.470153661758,110.461935712833,111.453717763908),
 .UNSPECIFIED.);
#110=B_SPLINE_SURFACE_WITH_KNOTS('',3,3,((#34494,#34495,#34496,#34497,#34498,
#34499,#34500,#34501,#34502,#34503,#34504,#34505,#34506,#34507,#34508,#34509,
#34510,#34511,#34512,#34513,#34514,#34515,#34516,#34517,#34518,#34519,#34520,
#34521,#34522,#34523,#34524,#34525,#34526,#34527,#34528,#34529,#34530,#34531,
#34532,#34533,#34534,#34535,#34536,#34537,#34538,#34539,#34540,#34541,#34542,
#34543,#34544,#34545,#34546,#34547,#34548,#34549,#34550,#34551,#34552,#34553,
#34554,#34555,#34556,#34557,#34558,#34559,#34560,#34561,#34562,#34563,#34564,
#34565,#34566,#34567,#34568,#34569,#34570,#34571,#34572,#34573,#34574,#34575,
#34576,#34577,#34578,#34579,#34580,#34581,#34582,#34583,#34584,#34585,#34586,
#34587,#34588,#34589,#34590,#34591,#34592,#34593,#34594,#34595,#34596,#34597,
#34598,#34599,#34600),(#34601,#34602,#34603,#34604,#34605,#34606,#34607,
#34608,#34609,#34610,#34611,#34612,#34613,#34614,#34615,#34616,#34617,#34618,
#34619,#34620,#34621,#34622,#34623,#34624,#34625,#34626,#34627,#34628,#34629,
#34630,#34631,#34632,#34633,#34634,#34635,#34636,#34637,#34638,#34639,#34640,
#34641,#34642,#34643,#34644,#34645,#34646,#34647,#34648,#34649,#34650,#34651,
#34652,#34653,#34654,#34655,#34656,#34657,#34658,#34659,#34660,#34661,#34662,
#34663,#34664,#34665,#34666,#34667,#34668,#34669,#34670,#34671,#34672,#34673,
#34674,#34675,#34676,#34677,#34678,#34679,#34680,#34681,#34682,#34683,#34684,
#34685,#34686,#34687,#34688,#34689,#34690,#34691,#34692,#34693,#34694,#34695,
#34696,#34697,#34698,#34699,#34700,#34701,#34702,#34703,#34704,#34705,#34706,
#34707),(#34708,#34709,#34710,#34711,#34712,#34713,#34714,#34715,#34716,
#34717,#34718,#34719,#34720,#34721,#34722,#34723,#34724,#34725,#34726,#34727,
#34728,#34729,#34730,#34731,#34732,#34733,#34734,#34735,#34736,#34737,#34738,
#34739,#34740,#34741,#34742,#34743,#34744,#34745,#34746,#34747,#34748,#34749,
#34750,#34751,#34752,#34753,#34754,#34755,#34756,#34757,#34758,#34759,#34760,
#34761,#34762,#34763,#34764,#34765,#34766,#34767,#34768,#34769,#34770,#34771,
#34772,#34773,#34774,#34775,#34776,#34777,#34778,#34779,#34780,#34781,#34782,
#34783,#34784,#34785,#34786,#34787,#34788,#34789,#34790,#34791,#34792,#34793,
#34794,#34795,#34796,#34797,#34798,#34799,#34800,#34801,#34802,#34803,#34804,
#34805,#34806,#34807,#34808,#34809,#34810,#34811,#34812,#34813,#34814),
(#34815,#34816,#34817,#34818,#34819,#34820,#34821,#34822,#34823,#34824,
#34825,#34826,#34827,#34828,#34829,#34830,#34831,#34832,#34833,#34834,#34835,
#34836,#34837,#34838,#34839,#34840,#34841,#34842,#34843,#34844,#34845,#34846,
#34847,#34848,#34849,#34850,#34851,#34852,#34853,#34854,#34855,#34856,#34857,
#34858,#34859,#34860,#34861,#34862,#34863,#34864,#34865,#34866,#34867,#34868,
#34869,#34870,#34871,#34872,#34873,#34874,#34875,#34876,#34877,#34878,#34879,
#34880,#34881,#34882,#34883,#34884,#34885,#34886,#34887,#34888,#34889,#34890,
#34891,#34892,#34893,#34894,#34895,#34896,#34897,#34898,#34899,#34900,#34901,
#34902,#34903,#34904,#34905,#34906,#34907,#34908,#34909,#34910,#34911,#34912,
#34913,#34914,#34915,#34916,#34917,#34918,#34919,#34920,#34921)),
 .UNSPECIFIED.,.F.,.F.,.F.,(4,4),(4,1,1,1,1,1,1,1,1,1,1,1,1,1,1,1,1,1,1,
1,1,1,1,1,1,1,1,1,1,1,1,1,1,1,1,1,1,1,1,1,1,1,1,1,1,1,1,1,1,1,1,1,1,1,1,
1,1,1,1,1,1,1,1,1,1,1,1,1,1,1,1,1,1,1,1,1,1,1,1,1,1,1,1,1,1,1,1,1,1,1,1,
1,1,1,1,1,1,1,1,1,1,1,1,1,4),(0.,0.0658179306876168),(11.6150328478185,
12.6068148988938,13.598596949969,14.5903790010443,15.5821610521195,16.5739431031947,
17.56572515427,18.5575072053452,19.5492892564205,20.5410713074957,21.5328533585709,
22.5246354096462,23.5164174607214,24.5081995117967,25.4999815628719,26.4917636139471,
27.4835456650224,28.4753277160976,29.4671097671729,30.4588918182481,31.4506738693233,
32.4424559203986,33.4342379714738,34.4260200225491,35.4178020736243,36.4095841246995,
37.4013661757748,38.39314822685,39.3849302779253,40.3767123290005,41.3684943800758,
42.360276431151,43.3520584822262,44.3438405333015,45.3356225843767,46.327404635452,
47.3191866865272,48.3109687376024,49.3027507886777,50.2945328397529,51.2863148908282,
52.2780969419034,53.2698789929786,54.2616610440539,55.2534430951291,56.2452251462044,
57.2370071972796,58.2287892483548,59.2205712994301,60.2123533505053,61.2041354015806,
62.1959174526558,63.187699503731,64.1794815548063,65.1712636058815,66.1630456569568,
67.154827708032,68.1466097591072,69.1383918101825,70.1301738612577,71.121955912333,
72.1137379634082,73.1055200144834,74.0973020655587,75.0890841166339,76.0808661677092,
77.0726482187844,78.0644302698597,79.0562123209349,80.0479943720101,81.0397764230854,
82.0315584741606,83.0233405252359,84.0151225763111,85.0069046273863,85.9986866784616,
86.9904687295368,87.9822507806121,88.9740328316873,89.9658148827625,90.9575969338378,
91.949378984913,92.9411610359883,93.9329430870635,94.9247251381387,95.916507189214,
96.9082892402892,97.9000712913645,98.8918533424397,99.883635393515,100.87541744459,
101.867199495665,102.858981546741,103.850763597816,104.842545648891,105.834327699966,
106.826109751042,107.817891802117,108.809673853192,109.801455904267,110.793237955343,
111.785020006418,112.776802057493,113.768584108568,114.760366159644),
 .UNSPECIFIED.);
#111=B_SPLINE_SURFACE_WITH_KNOTS('',3,3,((#35814,#35815,#35816,#35817,#35818,
#35819,#35820,#35821,#35822,#35823,#35824,#35825,#35826,#35827,#35828,#35829,
#35830,#35831,#35832,#35833,#35834,#35835,#35836,#35837,#35838,#35839,#35840,
#35841,#35842,#35843,#35844,#35845,#35846,#35847,#35848,#35849,#35850,#35851,
#35852,#35853),(#35854,#35855,#35856,#35857,#35858,#35859,#35860,#35861,
#35862,#35863,#35864,#35865,#35866,#35867,#35868,#35869,#35870,#35871,#35872,
#35873,#35874,#35875,#35876,#35877,#35878,#35879,#35880,#35881,#35882,#35883,
#35884,#35885,#35886,#35887,#35888,#35889,#35890,#35891,#35892,#35893),
(#35894,#35895,#35896,#35897,#35898,#35899,#35900,#35901,#35902,#35903,
#35904,#35905,#35906,#35907,#35908,#35909,#35910,#35911,#35912,#35913,#35914,
#35915,#35916,#35917,#35918,#35919,#35920,#35921,#35922,#35923,#35924,#35925,
#35926,#35927,#35928,#35929,#35930,#35931,#35932,#35933),(#35934,#35935,
#35936,#35937,#35938,#35939,#35940,#35941,#35942,#35943,#35944,#35945,#35946,
#35947,#35948,#35949,#35950,#35951,#35952,#35953,#35954,#35955,#35956,#35957,
#35958,#35959,#35960,#35961,#35962,#35963,#35964,#35965,#35966,#35967,#35968,
#35969,#35970,#35971,#35972,#35973),(#35974,#35975,#35976,#35977,#35978,
#35979,#35980,#35981,#35982,#35983,#35984,#35985,#35986,#35987,#35988,#35989,
#35990,#35991,#35992,#35993,#35994,#35995,#35996,#35997,#35998,#35999,#36000,
#36001,#36002,#36003,#36004,#36005,#36006,#36007,#36008,#36009,#36010,#36011,
#36012,#36013)),.UNSPECIFIED.,.F.,.F.,.F.,(4,1,4),(4,2,2,2,2,2,1,1,2,1,
1,1,1,1,1,2,1,2,1,1,1,1,2,1,1,1,1,1,4),(0.104020343629189,0.464972094135687,
0.946241094811018),(0.00211325483337195,0.100793262783688,0.212043315812054,
0.313257792411489,0.405143101782566,0.488664067632647,0.50778607271066,
0.526908077788674,0.565152087944702,0.569607108681037,0.574062129417373,
0.582972170890044,0.600792253835385,0.618612336780727,0.627522378253398,
0.636432419726069,0.670664755628991,0.704897091531912,0.71057214746399,
0.716247203396069,0.727597315260226,0.750297538988541,0.79569798644517,
0.806906221911025,0.81811445737688,0.840530928308591,0.862947399240301,
0.885363870172012,0.975029753898854),.UNSPECIFIED.);
#112=B_SPLINE_SURFACE_WITH_KNOTS('',3,3,((#36323,#36324,#36325,#36326,#36327,
#36328,#36329,#36330,#36331,#36332,#36333,#36334,#36335,#36336,#36337,#36338,
#36339,#36340,#36341,#36342,#36343,#36344,#36345,#36346,#36347,#36348,#36349,
#36350,#36351,#36352,#36353,#36354,#36355,#36356,#36357,#36358,#36359,#36360,
#36361,#36362,#36363,#36364),(#36365,#36366,#36367,#36368,#36369,#36370,
#36371,#36372,#36373,#36374,#36375,#36376,#36377,#36378,#36379,#36380,#36381,
#36382,#36383,#36384,#36385,#36386,#36387,#36388,#36389,#36390,#36391,#36392,
#36393,#36394,#36395,#36396,#36397,#36398,#36399,#36400,#36401,#36402,#36403,
#36404,#36405,#36406),(#36407,#36408,#36409,#36410,#36411,#36412,#36413,
#36414,#36415,#36416,#36417,#36418,#36419,#36420,#36421,#36422,#36423,#36424,
#36425,#36426,#36427,#36428,#36429,#36430,#36431,#36432,#36433,#36434,#36435,
#36436,#36437,#36438,#36439,#36440,#36441,#36442,#36443,#36444,#36445,#36446,
#36447,#36448),(#36449,#36450,#36451,#36452,#36453,#36454,#36455,#36456,
#36457,#36458,#36459,#36460,#36461,#36462,#36463,#36464,#36465,#36466,#36467,
#36468,#36469,#36470,#36471,#36472,#36473,#36474,#36475,#36476,#36477,#36478,
#36479,#36480,#36481,#36482,#36483,#36484,#36485,#36486,#36487,#36488,#36489,
#36490),(#36491,#36492,#36493,#36494,#36495,#36496,#36497,#36498,#36499,
#36500,#36501,#36502,#36503,#36504,#36505,#36506,#36507,#36508,#36509,#36510,
#36511,#36512,#36513,#36514,#36515,#36516,#36517,#36518,#36519,#36520,#36521,
#36522,#36523,#36524,#36525,#36526,#36527,#36528,#36529,#36530,#36531,#36532)),
 .UNSPECIFIED.,.F.,.F.,.F.,(4,1,4),(4,2,2,2,1,2,2,1,1,2,1,1,1,1,1,1,1,2,
1,2,1,1,1,1,2,1,1,1,1,1,4),(0.104020343629189,0.464972094135687,0.946241094811018),
(0.00211325483337195,0.100793262783688,0.212043315812054,0.313257792411489,
0.336229119754259,0.405143101782566,0.488664067632647,0.50778607271066,
0.526908077788674,0.565152087944702,0.582972170890044,0.600792253835385,
0.609702295308056,0.618612336780727,0.627522378253398,0.631977398989734,
0.634204909357901,0.636432419726069,0.670664755628991,0.704897091531912,
0.71057214746399,0.716247203396069,0.727597315260226,0.750297538988541,
0.79569798644517,0.806906221911025,0.81811445737688,0.840530928308591,0.862947399240301,
0.885363870172012,0.975029753898854),.UNSPECIFIED.);
#113=B_SPLINE_SURFACE_WITH_KNOTS('',3,3,((#36842,#36843,#36844,#36845,#36846,
#36847,#36848,#36849,#36850,#36851,#36852,#36853,#36854,#36855,#36856,#36857,
#36858,#36859,#36860,#36861,#36862,#36863,#36864,#36865,#36866,#36867,#36868,
#36869,#36870,#36871,#36872,#36873,#36874,#36875,#36876,#36877,#36878,#36879),
(#36880,#36881,#36882,#36883,#36884,#36885,#36886,#36887,#36888,#36889,
#36890,#36891,#36892,#36893,#36894,#36895,#36896,#36897,#36898,#36899,#36900,
#36901,#36902,#36903,#36904,#36905,#36906,#36907,#36908,#36909,#36910,#36911,
#36912,#36913,#36914,#36915,#36916,#36917),(#36918,#36919,#36920,#36921,
#36922,#36923,#36924,#36925,#36926,#36927,#36928,#36929,#36930,#36931,#36932,
#36933,#36934,#36935,#36936,#36937,#36938,#36939,#36940,#36941,#36942,#36943,
#36944,#36945,#36946,#36947,#36948,#36949,#36950,#36951,#36952,#36953,#36954,
#36955),(#36956,#36957,#36958,#36959,#36960,#36961,#36962,#36963,#36964,
#36965,#36966,#36967,#36968,#36969,#36970,#36971,#36972,#36973,#36974,#36975,
#36976,#36977,#36978,#36979,#36980,#36981,#36982,#36983,#36984,#36985,#36986,
#36987,#36988,#36989,#36990,#36991,#36992,#36993),(#36994,#36995,#36996,
#36997,#36998,#36999,#37000,#37001,#37002,#37003,#37004,#37005,#37006,#37007,
#37008,#37009,#37010,#37011,#37012,#37013,#37014,#37015,#37016,#37017,#37018,
#37019,#37020,#37021,#37022,#37023,#37024,#37025,#37026,#37027,#37028,#37029,
#37030,#37031)),.UNSPECIFIED.,.F.,.F.,.F.,(4,1,4),(4,2,2,2,1,2,2,1,2,1,
1,1,1,1,2,1,2,1,1,1,2,1,1,1,1,1,4),(0.104020343629189,0.464972094135687,
0.946241094811018),(0.00211325483337195,0.100793262783688,0.212043315812054,
0.313257792411489,0.336229119754259,0.405143101782566,0.488664067632647,
0.526908077788674,0.565152087944702,0.569607108681037,0.574062129417373,
0.582972170890044,0.600792253835385,0.618612336780727,0.636432419726069,
0.65354858767753,0.704897091531912,0.716247203396069,0.727597315260226,
0.750297538988541,0.79569798644517,0.806906221911025,0.81811445737688,0.840530928308591,
0.851739163774446,0.885363870172012,0.975029753898854),.UNSPECIFIED.);
#114=B_SPLINE_SURFACE_WITH_KNOTS('',3,3,((#37341,#37342,#37343,#37344,#37345,
#37346,#37347,#37348,#37349,#37350,#37351,#37352,#37353,#37354,#37355,#37356,
#37357,#37358,#37359,#37360,#37361,#37362,#37363,#37364,#37365,#37366,#37367,
#37368,#37369,#37370,#37371,#37372,#37373,#37374,#37375,#37376,#37377,#37378,
#37379,#37380),(#37381,#37382,#37383,#37384,#37385,#37386,#37387,#37388,
#37389,#37390,#37391,#37392,#37393,#37394,#37395,#37396,#37397,#37398,#37399,
#37400,#37401,#37402,#37403,#37404,#37405,#37406,#37407,#37408,#37409,#37410,
#37411,#37412,#37413,#37414,#37415,#37416,#37417,#37418,#37419,#37420),
(#37421,#37422,#37423,#37424,#37425,#37426,#37427,#37428,#37429,#37430,
#37431,#37432,#37433,#37434,#37435,#37436,#37437,#37438,#37439,#37440,#37441,
#37442,#37443,#37444,#37445,#37446,#37447,#37448,#37449,#37450,#37451,#37452,
#37453,#37454,#37455,#37456,#37457,#37458,#37459,#37460),(#37461,#37462,
#37463,#37464,#37465,#37466,#37467,#37468,#37469,#37470,#37471,#37472,#37473,
#37474,#37475,#37476,#37477,#37478,#37479,#37480,#37481,#37482,#37483,#37484,
#37485,#37486,#37487,#37488,#37489,#37490,#37491,#37492,#37493,#37494,#37495,
#37496,#37497,#37498,#37499,#37500),(#37501,#37502,#37503,#37504,#37505,
#37506,#37507,#37508,#37509,#37510,#37511,#37512,#37513,#37514,#37515,#37516,
#37517,#37518,#37519,#37520,#37521,#37522,#37523,#37524,#37525,#37526,#37527,
#37528,#37529,#37530,#37531,#37532,#37533,#37534,#37535,#37536,#37537,#37538,
#37539,#37540)),.UNSPECIFIED.,.F.,.F.,.F.,(4,1,4),(4,2,2,2,2,2,1,1,2,1,
1,1,1,1,1,2,1,2,1,1,1,1,2,1,1,1,1,1,4),(0.104020343629189,0.464972094135687,
0.946241094811018),(0.00211325483337195,0.100793262783688,0.212043315812054,
0.313257792411489,0.405143101782566,0.488664067632647,0.50778607271066,
0.526908077788674,0.565152087944702,0.569607108681037,0.574062129417373,
0.582972170890044,0.600792253835385,0.618612336780727,0.627522378253398,
0.636432419726069,0.670664755628991,0.704897091531912,0.71057214746399,
0.716247203396069,0.727597315260226,0.750297538988541,0.79569798644517,
0.806906221911025,0.81811445737688,0.840530928308591,0.862947399240301,
0.885363870172012,0.975029753898854),.UNSPECIFIED.);
#115=B_SPLINE_SURFACE_WITH_KNOTS('',3,3,((#37850,#37851,#37852,#37853,#37854,
#37855,#37856,#37857,#37858,#37859,#37860,#37861,#37862,#37863,#37864,#37865,
#37866,#37867,#37868,#37869,#37870,#37871,#37872,#37873,#37874,#37875,#37876,
#37877,#37878,#37879,#37880,#37881,#37882,#37883,#37884,#37885,#37886,#37887,
#37888,#37889,#37890,#37891),(#37892,#37893,#37894,#37895,#37896,#37897,
#37898,#37899,#37900,#37901,#37902,#37903,#37904,#37905,#37906,#37907,#37908,
#37909,#37910,#37911,#37912,#37913,#37914,#37915,#37916,#37917,#37918,#37919,
#37920,#37921,#37922,#37923,#37924,#37925,#37926,#37927,#37928,#37929,#37930,
#37931,#37932,#37933),(#37934,#37935,#37936,#37937,#37938,#37939,#37940,
#37941,#37942,#37943,#37944,#37945,#37946,#37947,#37948,#37949,#37950,#37951,
#37952,#37953,#37954,#37955,#37956,#37957,#37958,#37959,#37960,#37961,#37962,
#37963,#37964,#37965,#37966,#37967,#37968,#37969,#37970,#37971,#37972,#37973,
#37974,#37975),(#37976,#37977,#37978,#37979,#37980,#37981,#37982,#37983,
#37984,#37985,#37986,#37987,#37988,#37989,#37990,#37991,#37992,#37993,#37994,
#37995,#37996,#37997,#37998,#37999,#38000,#38001,#38002,#38003,#38004,#38005,
#38006,#38007,#38008,#38009,#38010,#38011,#38012,#38013,#38014,#38015,#38016,
#38017),(#38018,#38019,#38020,#38021,#38022,#38023,#38024,#38025,#38026,
#38027,#38028,#38029,#38030,#38031,#38032,#38033,#38034,#38035,#38036,#38037,
#38038,#38039,#38040,#38041,#38042,#38043,#38044,#38045,#38046,#38047,#38048,
#38049,#38050,#38051,#38052,#38053,#38054,#38055,#38056,#38057,#38058,#38059)),
 .UNSPECIFIED.,.F.,.F.,.F.,(4,1,4),(4,2,2,2,1,2,2,1,1,2,1,1,1,1,1,1,1,2,
1,2,1,1,1,1,2,1,1,1,1,1,4),(0.104020343629189,0.464972094135687,0.946241094811018),
(0.00211325483337195,0.100793262783688,0.212043315812054,0.313257792411489,
0.336229119754259,0.405143101782566,0.488664067632647,0.50778607271066,
0.526908077788674,0.565152087944702,0.582972170890044,0.600792253835385,
0.609702295308056,0.618612336780727,0.627522378253398,0.631977398989734,
0.634204909357901,0.636432419726069,0.670664755628991,0.704897091531912,
0.71057214746399,0.716247203396069,0.727597315260226,0.750297538988541,
0.79569798644517,0.806906221911025,0.81811445737688,0.840530928308591,0.862947399240301,
0.885363870172012,0.975029753898854),.UNSPECIFIED.);
#116=B_SPLINE_SURFACE_WITH_KNOTS('',3,3,((#38369,#38370,#38371,#38372,#38373,
#38374,#38375,#38376,#38377,#38378,#38379,#38380,#38381,#38382,#38383,#38384,
#38385,#38386,#38387,#38388,#38389,#38390,#38391,#38392,#38393,#38394,#38395,
#38396,#38397,#38398,#38399,#38400,#38401,#38402,#38403,#38404,#38405,#38406),
(#38407,#38408,#38409,#38410,#38411,#38412,#38413,#38414,#38415,#38416,
#38417,#38418,#38419,#38420,#38421,#38422,#38423,#38424,#38425,#38426,#38427,
#38428,#38429,#38430,#38431,#38432,#38433,#38434,#38435,#38436,#38437,#38438,
#38439,#38440,#38441,#38442,#38443,#38444),(#38445,#38446,#38447,#38448,
#38449,#38450,#38451,#38452,#38453,#38454,#38455,#38456,#38457,#38458,#38459,
#38460,#38461,#38462,#38463,#38464,#38465,#38466,#38467,#38468,#38469,#38470,
#38471,#38472,#38473,#38474,#38475,#38476,#38477,#38478,#38479,#38480,#38481,
#38482),(#38483,#38484,#38485,#38486,#38487,#38488,#38489,#38490,#38491,
#38492,#38493,#38494,#38495,#38496,#38497,#38498,#38499,#38500,#38501,#38502,
#38503,#38504,#38505,#38506,#38507,#38508,#38509,#38510,#38511,#38512,#38513,
#38514,#38515,#38516,#38517,#38518,#38519,#38520),(#38521,#38522,#38523,
#38524,#38525,#38526,#38527,#38528,#38529,#38530,#38531,#38532,#38533,#38534,
#38535,#38536,#38537,#38538,#38539,#38540,#38541,#38542,#38543,#38544,#38545,
#38546,#38547,#38548,#38549,#38550,#38551,#38552,#38553,#38554,#38555,#38556,
#38557,#38558)),.UNSPECIFIED.,.F.,.F.,.F.,(4,1,4),(4,2,2,2,1,2,2,1,2,1,
1,1,1,1,2,1,2,1,1,1,2,1,1,1,1,1,4),(0.104020343629189,0.464972094135687,
0.946241094811018),(0.00211325483337195,0.100793262783688,0.212043315812054,
0.313257792411489,0.336229119754259,0.405143101782566,0.488664067632647,
0.526908077788674,0.565152087944702,0.569607108681037,0.574062129417373,
0.582972170890044,0.600792253835385,0.618612336780727,0.636432419726069,
0.65354858767753,0.704897091531912,0.716247203396069,0.727597315260226,
0.750297538988541,0.79569798644517,0.806906221911025,0.81811445737688,0.840530928308591,
0.851739163774446,0.885363870172012,0.975029753898854),.UNSPECIFIED.);
#117=B_SPLINE_SURFACE_WITH_KNOTS('',3,3,((#38868,#38869,#38870,#38871,#38872,
#38873,#38874,#38875,#38876,#38877,#38878,#38879,#38880,#38881,#38882,#38883,
#38884,#38885,#38886,#38887,#38888,#38889,#38890,#38891,#38892,#38893,#38894,
#38895,#38896,#38897,#38898,#38899,#38900,#38901,#38902,#38903,#38904,#38905,
#38906,#38907),(#38908,#38909,#38910,#38911,#38912,#38913,#38914,#38915,
#38916,#38917,#38918,#38919,#38920,#38921,#38922,#38923,#38924,#38925,#38926,
#38927,#38928,#38929,#38930,#38931,#38932,#38933,#38934,#38935,#38936,#38937,
#38938,#38939,#38940,#38941,#38942,#38943,#38944,#38945,#38946,#38947),
(#38948,#38949,#38950,#38951,#38952,#38953,#38954,#38955,#38956,#38957,
#38958,#38959,#38960,#38961,#38962,#38963,#38964,#38965,#38966,#38967,#38968,
#38969,#38970,#38971,#38972,#38973,#38974,#38975,#38976,#38977,#38978,#38979,
#38980,#38981,#38982,#38983,#38984,#38985,#38986,#38987),(#38988,#38989,
#38990,#38991,#38992,#38993,#38994,#38995,#38996,#38997,#38998,#38999,#39000,
#39001,#39002,#39003,#39004,#39005,#39006,#39007,#39008,#39009,#39010,#39011,
#39012,#39013,#39014,#39015,#39016,#39017,#39018,#39019,#39020,#39021,#39022,
#39023,#39024,#39025,#39026,#39027),(#39028,#39029,#39030,#39031,#39032,
#39033,#39034,#39035,#39036,#39037,#39038,#39039,#39040,#39041,#39042,#39043,
#39044,#39045,#39046,#39047,#39048,#39049,#39050,#39051,#39052,#39053,#39054,
#39055,#39056,#39057,#39058,#39059,#39060,#39061,#39062,#39063,#39064,#39065,
#39066,#39067)),.UNSPECIFIED.,.F.,.F.,.F.,(4,1,4),(4,2,2,2,2,2,1,1,2,1,
1,1,1,1,1,2,1,2,1,1,1,1,2,1,1,1,1,1,4),(0.104020343629189,0.464972094135687,
0.946241094811018),(0.00211325483337195,0.100793262783688,0.212043315812054,
0.313257792411489,0.405143101782566,0.488664067632647,0.50778607271066,
0.526908077788674,0.565152087944702,0.569607108681037,0.574062129417373,
0.582972170890044,0.600792253835385,0.618612336780727,0.627522378253398,
0.636432419726069,0.670664755628991,0.704897091531912,0.71057214746399,
0.716247203396069,0.727597315260226,0.750297538988541,0.79569798644517,
0.806906221911025,0.81811445737688,0.840530928308591,0.862947399240301,
0.885363870172012,0.975029753898854),.UNSPECIFIED.);
#118=B_SPLINE_SURFACE_WITH_KNOTS('',3,3,((#39377,#39378,#39379,#39380,#39381,
#39382,#39383,#39384,#39385,#39386,#39387,#39388,#39389,#39390,#39391,#39392,
#39393,#39394,#39395,#39396,#39397,#39398,#39399,#39400,#39401,#39402,#39403,
#39404,#39405,#39406,#39407,#39408,#39409,#39410,#39411,#39412,#39413,#39414,
#39415,#39416,#39417,#39418),(#39419,#39420,#39421,#39422,#39423,#39424,
#39425,#39426,#39427,#39428,#39429,#39430,#39431,#39432,#39433,#39434,#39435,
#39436,#39437,#39438,#39439,#39440,#39441,#39442,#39443,#39444,#39445,#39446,
#39447,#39448,#39449,#39450,#39451,#39452,#39453,#39454,#39455,#39456,#39457,
#39458,#39459,#39460),(#39461,#39462,#39463,#39464,#39465,#39466,#39467,
#39468,#39469,#39470,#39471,#39472,#39473,#39474,#39475,#39476,#39477,#39478,
#39479,#39480,#39481,#39482,#39483,#39484,#39485,#39486,#39487,#39488,#39489,
#39490,#39491,#39492,#39493,#39494,#39495,#39496,#39497,#39498,#39499,#39500,
#39501,#39502),(#39503,#39504,#39505,#39506,#39507,#39508,#39509,#39510,
#39511,#39512,#39513,#39514,#39515,#39516,#39517,#39518,#39519,#39520,#39521,
#39522,#39523,#39524,#39525,#39526,#39527,#39528,#39529,#39530,#39531,#39532,
#39533,#39534,#39535,#39536,#39537,#39538,#39539,#39540,#39541,#39542,#39543,
#39544),(#39545,#39546,#39547,#39548,#39549,#39550,#39551,#39552,#39553,
#39554,#39555,#39556,#39557,#39558,#39559,#39560,#39561,#39562,#39563,#39564,
#39565,#39566,#39567,#39568,#39569,#39570,#39571,#39572,#39573,#39574,#39575,
#39576,#39577,#39578,#39579,#39580,#39581,#39582,#39583,#39584,#39585,#39586)),
 .UNSPECIFIED.,.F.,.F.,.F.,(4,1,4),(4,2,2,2,1,2,2,1,1,2,1,1,1,1,1,1,1,2,
1,2,1,1,1,1,2,1,1,1,1,1,4),(0.104020343629189,0.464972094135687,0.946241094811018),
(0.00211325483337195,0.100793262783688,0.212043315812054,0.313257792411489,
0.336229119754259,0.405143101782566,0.488664067632647,0.50778607271066,
0.526908077788674,0.565152087944702,0.582972170890044,0.600792253835385,
0.609702295308056,0.618612336780727,0.627522378253398,0.631977398989734,
0.634204909357901,0.636432419726069,0.670664755628991,0.704897091531912,
0.71057214746399,0.716247203396069,0.727597315260226,0.750297538988541,
0.79569798644517,0.806906221911025,0.81811445737688,0.840530928308591,0.862947399240301,
0.885363870172012,0.975029753898854),.UNSPECIFIED.);
#119=B_SPLINE_SURFACE_WITH_KNOTS('',3,3,((#39896,#39897,#39898,#39899,#39900,
#39901,#39902,#39903,#39904,#39905,#39906,#39907,#39908,#39909,#39910,#39911,
#39912,#39913,#39914,#39915,#39916,#39917,#39918,#39919,#39920,#39921,#39922,
#39923,#39924,#39925,#39926,#39927,#39928,#39929,#39930,#39931,#39932,#39933,
#39934,#39935),(#39936,#39937,#39938,#39939,#39940,#39941,#39942,#39943,
#39944,#39945,#39946,#39947,#39948,#39949,#39950,#39951,#39952,#39953,#39954,
#39955,#39956,#39957,#39958,#39959,#39960,#39961,#39962,#39963,#39964,#39965,
#39966,#39967,#39968,#39969,#39970,#39971,#39972,#39973,#39974,#39975),
(#39976,#39977,#39978,#39979,#39980,#39981,#39982,#39983,#39984,#39985,
#39986,#39987,#39988,#39989,#39990,#39991,#39992,#39993,#39994,#39995,#39996,
#39997,#39998,#39999,#40000,#40001,#40002,#40003,#40004,#40005,#40006,#40007,
#40008,#40009,#40010,#40011,#40012,#40013,#40014,#40015),(#40016,#40017,
#40018,#40019,#40020,#40021,#40022,#40023,#40024,#40025,#40026,#40027,#40028,
#40029,#40030,#40031,#40032,#40033,#40034,#40035,#40036,#40037,#40038,#40039,
#40040,#40041,#40042,#40043,#40044,#40045,#40046,#40047,#40048,#40049,#40050,
#40051,#40052,#40053,#40054,#40055),(#40056,#40057,#40058,#40059,#40060,
#40061,#40062,#40063,#40064,#40065,#40066,#40067,#40068,#40069,#40070,#40071,
#40072,#40073,#40074,#40075,#40076,#40077,#40078,#40079,#40080,#40081,#40082,
#40083,#40084,#40085,#40086,#40087,#40088,#40089,#40090,#40091,#40092,#40093,
#40094,#40095)),.UNSPECIFIED.,.F.,.F.,.F.,(4,1,4),(4,2,1,2,1,2,2,2,1,2,
1,1,1,1,1,1,2,1,2,1,1,1,2,1,1,1,1,1,4),(0.104020343629189,0.58528934430452,
0.946241094811018),(0.00211325483337195,0.100793262783688,0.184230802554962,
0.212043315812054,0.287954173261631,0.313257792411489,0.405143101782566,
0.488664067632647,0.526908077788674,0.565152087944702,0.569607108681037,
0.574062129417373,0.582972170890044,0.600792253835385,0.618612336780727,
0.627522378253398,0.636432419726069,0.65354858767753,0.704897091531912,
0.716247203396069,0.727597315260226,0.750297538988541,0.79569798644517,
0.806906221911025,0.81811445737688,0.840530928308591,0.851739163774446,
0.885363870172012,0.975029753898854),.UNSPECIFIED.);
#120=B_SPLINE_SURFACE_WITH_KNOTS('',3,3,((#40405,#40406,#40407,#40408,#40409,
#40410,#40411,#40412,#40413,#40414,#40415,#40416,#40417,#40418,#40419,#40420,
#40421,#40422,#40423,#40424,#40425,#40426,#40427,#40428,#40429,#40430,#40431,
#40432,#40433,#40434,#40435,#40436,#40437,#40438,#40439,#40440,#40441,#40442,
#40443,#40444),(#40445,#40446,#40447,#40448,#40449,#40450,#40451,#40452,
#40453,#40454,#40455,#40456,#40457,#40458,#40459,#40460,#40461,#40462,#40463,
#40464,#40465,#40466,#40467,#40468,#40469,#40470,#40471,#40472,#40473,#40474,
#40475,#40476,#40477,#40478,#40479,#40480,#40481,#40482,#40483,#40484),
(#40485,#40486,#40487,#40488,#40489,#40490,#40491,#40492,#40493,#40494,
#40495,#40496,#40497,#40498,#40499,#40500,#40501,#40502,#40503,#40504,#40505,
#40506,#40507,#40508,#40509,#40510,#40511,#40512,#40513,#40514,#40515,#40516,
#40517,#40518,#40519,#40520,#40521,#40522,#40523,#40524),(#40525,#40526,
#40527,#40528,#40529,#40530,#40531,#40532,#40533,#40534,#40535,#40536,#40537,
#40538,#40539,#40540,#40541,#40542,#40543,#40544,#40545,#40546,#40547,#40548,
#40549,#40550,#40551,#40552,#40553,#40554,#40555,#40556,#40557,#40558,#40559,
#40560,#40561,#40562,#40563,#40564),(#40565,#40566,#40567,#40568,#40569,
#40570,#40571,#40572,#40573,#40574,#40575,#40576,#40577,#40578,#40579,#40580,
#40581,#40582,#40583,#40584,#40585,#40586,#40587,#40588,#40589,#40590,#40591,
#40592,#40593,#40594,#40595,#40596,#40597,#40598,#40599,#40600,#40601,#40602,
#40603,#40604)),.UNSPECIFIED.,.F.,.F.,.F.,(4,1,4),(4,2,2,2,2,2,1,1,2,1,
1,1,1,1,1,2,1,2,1,1,1,1,2,1,1,1,1,1,4),(0.104020343629189,0.464972094135687,
0.946241094811018),(0.00211325483337195,0.100793262783688,0.212043315812054,
0.313257792411489,0.405143101782566,0.488664067632647,0.50778607271066,
0.526908077788674,0.565152087944702,0.569607108681037,0.574062129417373,
0.582972170890044,0.600792253835385,0.618612336780727,0.627522378253398,
0.636432419726069,0.670664755628991,0.704897091531912,0.71057214746399,
0.716247203396069,0.727597315260226,0.750297538988541,0.79569798644517,
0.806906221911025,0.81811445737688,0.840530928308591,0.862947399240301,
0.885363870172012,0.975029753898854),.UNSPECIFIED.);
#121=B_SPLINE_SURFACE_WITH_KNOTS('',3,3,((#40914,#40915,#40916,#40917,#40918,
#40919,#40920,#40921,#40922,#40923,#40924,#40925,#40926,#40927,#40928,#40929,
#40930,#40931,#40932,#40933,#40934,#40935,#40936,#40937,#40938,#40939,#40940,
#40941,#40942,#40943,#40944,#40945,#40946,#40947,#40948,#40949,#40950,#40951,
#40952,#40953,#40954,#40955),(#40956,#40957,#40958,#40959,#40960,#40961,
#40962,#40963,#40964,#40965,#40966,#40967,#40968,#40969,#40970,#40971,#40972,
#40973,#40974,#40975,#40976,#40977,#40978,#40979,#40980,#40981,#40982,#40983,
#40984,#40985,#40986,#40987,#40988,#40989,#40990,#40991,#40992,#40993,#40994,
#40995,#40996,#40997),(#40998,#40999,#41000,#41001,#41002,#41003,#41004,
#41005,#41006,#41007,#41008,#41009,#41010,#41011,#41012,#41013,#41014,#41015,
#41016,#41017,#41018,#41019,#41020,#41021,#41022,#41023,#41024,#41025,#41026,
#41027,#41028,#41029,#41030,#41031,#41032,#41033,#41034,#41035,#41036,#41037,
#41038,#41039),(#41040,#41041,#41042,#41043,#41044,#41045,#41046,#41047,
#41048,#41049,#41050,#41051,#41052,#41053,#41054,#41055,#41056,#41057,#41058,
#41059,#41060,#41061,#41062,#41063,#41064,#41065,#41066,#41067,#41068,#41069,
#41070,#41071,#41072,#41073,#41074,#41075,#41076,#41077,#41078,#41079,#41080,
#41081),(#41082,#41083,#41084,#41085,#41086,#41087,#41088,#41089,#41090,
#41091,#41092,#41093,#41094,#41095,#41096,#41097,#41098,#41099,#41100,#41101,
#41102,#41103,#41104,#41105,#41106,#41107,#41108,#41109,#41110,#41111,#41112,
#41113,#41114,#41115,#41116,#41117,#41118,#41119,#41120,#41121,#41122,#41123)),
 .UNSPECIFIED.,.F.,.F.,.F.,(4,1,4),(4,2,2,2,1,2,2,1,1,2,1,1,1,1,1,1,1,2,
1,2,1,1,1,1,2,1,1,1,1,1,4),(0.104020343629189,0.464972094135687,0.946241094811018),
(0.00211325483337195,0.100793262783688,0.212043315812054,0.313257792411489,
0.336229119754259,0.405143101782566,0.488664067632647,0.50778607271066,
0.526908077788674,0.565152087944702,0.582972170890044,0.600792253835385,
0.609702295308056,0.618612336780727,0.627522378253398,0.631977398989734,
0.634204909357901,0.636432419726069,0.670664755628991,0.704897091531912,
0.71057214746399,0.716247203396069,0.727597315260226,0.750297538988541,
0.79569798644517,0.806906221911025,0.81811445737688,0.840530928308591,0.862947399240301,
0.885363870172012,0.975029753898854),.UNSPECIFIED.);
#122=B_SPLINE_SURFACE_WITH_KNOTS('',3,3,((#41433,#41434,#41435,#41436,#41437,
#41438,#41439,#41440,#41441,#41442,#41443,#41444,#41445,#41446,#41447,#41448,
#41449,#41450,#41451,#41452,#41453,#41454,#41455,#41456,#41457,#41458,#41459,
#41460,#41461,#41462,#41463,#41464,#41465,#41466,#41467,#41468,#41469,#41470),
(#41471,#41472,#41473,#41474,#41475,#41476,#41477,#41478,#41479,#41480,
#41481,#41482,#41483,#41484,#41485,#41486,#41487,#41488,#41489,#41490,#41491,
#41492,#41493,#41494,#41495,#41496,#41497,#41498,#41499,#41500,#41501,#41502,
#41503,#41504,#41505,#41506,#41507,#41508),(#41509,#41510,#41511,#41512,
#41513,#41514,#41515,#41516,#41517,#41518,#41519,#41520,#41521,#41522,#41523,
#41524,#41525,#41526,#41527,#41528,#41529,#41530,#41531,#41532,#41533,#41534,
#41535,#41536,#41537,#41538,#41539,#41540,#41541,#41542,#41543,#41544,#41545,
#41546),(#41547,#41548,#41549,#41550,#41551,#41552,#41553,#41554,#41555,
#41556,#41557,#41558,#41559,#41560,#41561,#41562,#41563,#41564,#41565,#41566,
#41567,#41568,#41569,#41570,#41571,#41572,#41573,#41574,#41575,#41576,#41577,
#41578,#41579,#41580,#41581,#41582,#41583,#41584),(#41585,#41586,#41587,
#41588,#41589,#41590,#41591,#41592,#41593,#41594,#41595,#41596,#41597,#41598,
#41599,#41600,#41601,#41602,#41603,#41604,#41605,#41606,#41607,#41608,#41609,
#41610,#41611,#41612,#41613,#41614,#41615,#41616,#41617,#41618,#41619,#41620,
#41621,#41622)),.UNSPECIFIED.,.F.,.F.,.F.,(4,1,4),(4,2,2,2,1,2,2,1,2,1,
1,1,1,1,2,1,2,1,1,1,2,1,1,1,1,1,4),(0.104020343629189,0.464972094135687,
0.946241094811018),(0.00211325483337195,0.100793262783688,0.212043315812054,
0.313257792411489,0.336229119754259,0.405143101782566,0.488664067632647,
0.526908077788674,0.565152087944702,0.569607108681037,0.574062129417373,
0.582972170890044,0.600792253835385,0.618612336780727,0.636432419726069,
0.65354858767753,0.704897091531912,0.716247203396069,0.727597315260226,
0.750297538988541,0.79569798644517,0.806906221911025,0.81811445737688,0.840530928308591,
0.851739163774446,0.885363870172012,0.975029753898854),.UNSPECIFIED.);
#197=FACE_BOUND('',#2305,.T.);
#198=FACE_BOUND('',#2391,.T.);
#199=FACE_BOUND('',#2395,.T.);
#200=FACE_BOUND('',#2424,.T.);
#201=FACE_BOUND('',#2515,.T.);
#202=FACE_BOUND('',#2517,.T.);
#203=FACE_BOUND('',#2583,.T.);
#204=FACE_BOUND('',#2589,.T.);
#205=FACE_BOUND('',#2595,.T.);
#264=PLANE('',#18483);
#265=PLANE('',#18485);
#266=PLANE('',#18486);
#267=PLANE('',#18487);
#268=PLANE('',#18488);
#269=PLANE('',#18489);
#270=PLANE('',#18490);
#271=PLANE('',#18491);
#272=PLANE('',#18492);
#273=PLANE('',#18493);
#274=PLANE('',#18494);
#275=PLANE('',#18495);
#276=PLANE('',#18496);
#277=PLANE('',#18497);
#278=PLANE('',#18498);
#279=PLANE('',#18499);
#280=PLANE('',#18500);
#281=PLANE('',#18501);
#282=PLANE('',#18502);
#283=PLANE('',#18503);
#284=PLANE('',#18504);
#285=PLANE('',#18505);
#286=PLANE('',#18506);
#287=PLANE('',#18507);
#288=PLANE('',#18508);
#289=PLANE('',#18509);
#290=PLANE('',#18510);
#291=PLANE('',#18511);
#292=PLANE('',#18512);
#293=PLANE('',#18513);
#294=PLANE('',#18514);
#295=PLANE('',#18515);
#296=PLANE('',#18516);
#297=PLANE('',#18517);
#298=PLANE('',#18518);
#299=PLANE('',#18519);
#300=PLANE('',#18520);
#301=PLANE('',#18521);
#302=PLANE('',#18522);
#303=PLANE('',#18523);
#304=PLANE('',#18524);
#305=PLANE('',#18525);
#306=PLANE('',#18526);
#307=PLANE('',#18527);
#308=PLANE('',#18528);
#309=PLANE('',#18529);
#310=PLANE('',#18530);
#311=PLANE('',#18531);
#312=PLANE('',#18595);
#313=PLANE('',#18602);
#314=PLANE('',#18606);
#315=PLANE('',#18617);
#316=PLANE('',#18621);
#317=PLANE('',#18629);
#318=PLANE('',#18633);
#319=PLANE('',#18641);
#320=PLANE('',#18645);
#321=PLANE('',#18653);
#322=PLANE('',#18657);
#323=PLANE('',#18665);
#324=PLANE('',#18669);
#325=PLANE('',#18686);
#326=PLANE('',#18691);
#327=PLANE('',#18696);
#328=PLANE('',#18701);
#329=PLANE('',#18706);
#330=PLANE('',#18711);
#331=PLANE('',#18716);
#332=PLANE('',#18721);
#333=PLANE('',#18726);
#334=PLANE('',#18731);
#335=PLANE('',#18736);
#336=PLANE('',#18741);
#337=PLANE('',#18752);
#338=PLANE('',#18755);
#339=PLANE('',#18760);
#340=PLANE('',#18763);
#341=PLANE('',#18768);
#342=PLANE('',#18771);
#343=PLANE('',#18776);
#344=PLANE('',#18781);
#345=PLANE('',#18786);
#346=PLANE('',#18791);
#347=PLANE('',#18796);
#348=PLANE('',#18801);
#349=PLANE('',#18806);
#350=PLANE('',#18811);
#351=PLANE('',#18816);
#352=PLANE('',#18819);
#353=PLANE('',#18825);
#354=PLANE('',#18826);
#355=PLANE('',#18831);
#356=PLANE('',#18833);
#357=PLANE('',#18834);
#358=PLANE('',#18836);
#359=PLANE('',#18837);
#360=PLANE('',#18839);
#361=PLANE('',#18840);
#362=PLANE('',#18842);
#363=PLANE('',#18843);
#364=PLANE('',#18845);
#365=PLANE('',#18846);
#366=PLANE('',#18848);
#367=PLANE('',#18849);
#368=PLANE('',#18851);
#369=PLANE('',#18852);
#370=PLANE('',#18854);
#371=PLANE('',#18855);
#372=PLANE('',#18857);
#373=PLANE('',#18858);
#374=PLANE('',#18860);
#375=PLANE('',#18861);
#376=PLANE('',#18863);
#377=PLANE('',#18864);
#378=PLANE('',#18866);
#379=PLANE('',#18867);
#380=PLANE('',#18868);
#381=PLANE('',#18869);
#382=PLANE('',#18870);
#383=PLANE('',#18871);
#384=PLANE('',#18872);
#385=PLANE('',#18873);
#386=PLANE('',#18874);
#387=PLANE('',#18875);
#388=PLANE('',#18876);
#389=PLANE('',#18877);
#390=PLANE('',#18878);
#391=PLANE('',#18879);
#392=PLANE('',#18880);
#393=PLANE('',#18881);
#394=PLANE('',#18888);
#395=PLANE('',#18898);
#396=PLANE('',#18915);
#827=CONICAL_SURFACE('',#18477,9.87862393885688,1.05560791353274);
#828=CONICAL_SURFACE('',#18481,10.3,0.540419500270582);
#829=CONICAL_SURFACE('',#18532,34.75,0.785398163397448);
#830=CONICAL_SURFACE('',#18537,34.75,0.785398163397448);
#831=CONICAL_SURFACE('',#18542,34.75,0.785398163397453);
#832=CONICAL_SURFACE('',#18547,34.75,0.785398163397448);
#833=CONICAL_SURFACE('',#18552,34.75,0.785398163397453);
#834=CONICAL_SURFACE('',#18557,34.75,0.785398163397443);
#835=CONICAL_SURFACE('',#18562,34.75,0.785398163397448);
#836=CONICAL_SURFACE('',#18567,34.75,0.785398163397456);
#837=CONICAL_SURFACE('',#18572,34.75,0.785398163397453);
#838=CONICAL_SURFACE('',#18577,34.75,0.785398163397448);
#839=CONICAL_SURFACE('',#18582,34.75,0.785398163397448);
#840=CONICAL_SURFACE('',#18587,34.75,0.785398163397453);
#841=CONICAL_SURFACE('',#18592,8.95,0.785398163397451);
#842=CONICAL_SURFACE('',#18599,8.95,0.785398163397451);
#843=CONICAL_SURFACE('',#18607,8.25,0.785398163397452);
#844=CONICAL_SURFACE('',#18610,32.75,0.785398163397439);
#845=CONICAL_SURFACE('',#18618,8.25,0.785398163397449);
#846=CONICAL_SURFACE('',#18622,32.75,0.785398163397439);
#847=CONICAL_SURFACE('',#18630,8.25,0.785398163397451);
#848=CONICAL_SURFACE('',#18634,32.75,0.785398163397439);
#849=CONICAL_SURFACE('',#18642,8.25,0.785398163397452);
#850=CONICAL_SURFACE('',#18646,32.75,0.785398163397439);
#851=CONICAL_SURFACE('',#18654,8.25,0.785398163397449);
#852=CONICAL_SURFACE('',#18658,32.75,0.785398163397439);
#853=CONICAL_SURFACE('',#18666,8.25,0.785398163397451);
#854=CONICAL_SURFACE('',#18684,32.75,0.785398163397439);
#855=CONICAL_SURFACE('',#18697,8.25,0.785398163397452);
#856=CONICAL_SURFACE('',#18699,32.75,0.785398163397439);
#857=CONICAL_SURFACE('',#18707,8.25,0.785398163397454);
#858=CONICAL_SURFACE('',#18709,32.75,0.785398163397439);
#859=CONICAL_SURFACE('',#18717,8.25,0.785398163397451);
#860=CONICAL_SURFACE('',#18719,32.75,0.785398163397439);
#861=CONICAL_SURFACE('',#18727,8.25,0.785398163397452);
#862=CONICAL_SURFACE('',#18729,32.75,0.785398163397439);
#863=CONICAL_SURFACE('',#18737,8.25,0.78539816339745);
#864=CONICAL_SURFACE('',#18739,32.75,0.785398163397439);
#865=CONICAL_SURFACE('',#18747,32.75,0.785398163397439);
#866=CONICAL_SURFACE('',#18753,8.25,0.785398163397451);
#867=CONICAL_SURFACE('',#18756,32.7,0.876058050598196);
#868=CONICAL_SURFACE('',#18770,32.7,0.876058050598196);
#869=CONICAL_SURFACE('',#18774,32.7,0.876058050598196);
#870=CONICAL_SURFACE('',#18775,32.7,0.876058050598196);
#871=CONICAL_SURFACE('',#18779,32.7,0.876058050598196);
#872=CONICAL_SURFACE('',#18780,32.7,0.876058050598196);
#873=CONICAL_SURFACE('',#18784,32.7,0.876058050598196);
#874=CONICAL_SURFACE('',#18785,32.7,0.876058050598196);
#875=CONICAL_SURFACE('',#18789,32.7,0.876058050598196);
#876=CONICAL_SURFACE('',#18790,32.7,0.876058050598196);
#877=CONICAL_SURFACE('',#18794,32.7,0.876058050598196);
#878=CONICAL_SURFACE('',#18795,32.7,0.876058050598196);
#879=CONICAL_SURFACE('',#18799,32.7,0.876058050598196);
#880=CONICAL_SURFACE('',#18800,32.7,0.876058050598196);
#881=CONICAL_SURFACE('',#18804,32.7,0.876058050598196);
#882=CONICAL_SURFACE('',#18805,32.7,0.876058050598196);
#883=CONICAL_SURFACE('',#18809,32.7,0.876058050598196);
#884=CONICAL_SURFACE('',#18810,32.7,0.876058050598196);
#885=CONICAL_SURFACE('',#18814,32.7,0.876058050598196);
#886=CONICAL_SURFACE('',#18815,32.7,0.876058050598196);
#887=CONICAL_SURFACE('',#18817,32.7,0.876058050598196);
#888=CONICAL_SURFACE('',#18818,32.7,0.876058050598196);
#889=CONICAL_SURFACE('',#18820,32.7,0.876058050598196);
#890=CONICAL_SURFACE('',#18821,32.7,0.876058050598196);
#891=CONICAL_SURFACE('',#18882,13.,1.23412150740817);
#892=CONICAL_SURFACE('',#18884,11.3,1.05165021254838);
#893=CONICAL_SURFACE('',#18885,9.,0.785398163397459);
#894=CONICAL_SURFACE('',#18886,9.,0.785398163397448);
#895=CONICAL_SURFACE('',#18890,6.7,0.785398163397446);
#896=CONICAL_SURFACE('',#18892,5.85,0.950546840812077);
#897=CONICAL_SURFACE('',#18896,5.35,0.785398163397459);
#898=CONICAL_SURFACE('',#18902,3.4,0.785398163397415);
#899=CONICAL_SURFACE('',#18906,3.2,1.24904577239829);
#900=CONICAL_SURFACE('',#18910,3.2,1.10714871779408);
#901=CONICAL_SURFACE('',#18913,3.25,0.785398163397441);
#976=(
BOUNDED_CURVE()
B_SPLINE_CURVE(5,(#24658,#24659,#24660,#24661,#24662,#24663,#24664,#24665,
#24666,#24667,#24668),.UNSPECIFIED.,.F.,.F.)
B_SPLINE_CURVE_WITH_KNOTS((6,1,1,1,1,1,6),(0.167063732147151,0.2,0.24,0.28,
0.32,0.36,0.378267291341468),.UNSPECIFIED.)
CURVE()
GEOMETRIC_REPRESENTATION_ITEM()
RATIONAL_B_SPLINE_CURVE((1.,1.,1.,1.,1.,1.,1.,1.,1.,1.,1.))
REPRESENTATION_ITEM('')
);
#977=(
BOUNDED_CURVE()
B_SPLINE_CURVE(5,(#24696,#24697,#24698,#24699,#24700,#24701),
 .UNSPECIFIED.,.F.,.F.)
B_SPLINE_CURVE_WITH_KNOTS((6,6),(0.,0.0177013282315284),.UNSPECIFIED.)
CURVE()
GEOMETRIC_REPRESENTATION_ITEM()
RATIONAL_B_SPLINE_CURVE((1.,1.,1.,1.,1.,1.))
REPRESENTATION_ITEM('')
);
#978=(
BOUNDED_CURVE()
B_SPLINE_CURVE(2,(#32858,#32859,#32860),.UNSPECIFIED.,.F.,.F.)
B_SPLINE_CURVE_WITH_KNOTS((3,3),(0.0642390630877484,0.159883011113203),
 .UNSPECIFIED.)
CURVE()
GEOMETRIC_REPRESENTATION_ITEM()
RATIONAL_B_SPLINE_CURVE((1.00013237845317,1.00016634217764,1.00000799154408))
REPRESENTATION_ITEM('')
);
#979=(
BOUNDED_CURVE()
B_SPLINE_CURVE(2,(#32864,#32865,#32866),.UNSPECIFIED.,.F.,.F.)
B_SPLINE_CURVE_WITH_KNOTS((3,3),(0.000526061815849738,0.0490373321941988),
 .UNSPECIFIED.)
CURVE()
GEOMETRIC_REPRESENTATION_ITEM()
RATIONAL_B_SPLINE_CURVE((1.00000140604824,1.00006598064969,1.00008344962655))
REPRESENTATION_ITEM('')
);
#980=(
BOUNDED_CURVE()
B_SPLINE_CURVE(2,(#32868,#32869,#32870),.UNSPECIFIED.,.F.,.F.)
B_SPLINE_CURVE_WITH_KNOTS((3,3),(0.0729556909351875,0.123986559684229),
 .UNSPECIFIED.)
CURVE()
GEOMETRIC_REPRESENTATION_ITEM()
RATIONAL_B_SPLINE_CURVE((1.00116052526037,1.0009929348209,1.00002308400869))
REPRESENTATION_ITEM('')
);
#981=(
BOUNDED_CURVE()
B_SPLINE_CURVE(2,(#32886,#32887,#32888),.UNSPECIFIED.,.F.,.F.)
B_SPLINE_CURVE_WITH_KNOTS((3,3),(0.0378274750358814,0.0817111642791895),
 .UNSPECIFIED.)
CURVE()
GEOMETRIC_REPRESENTATION_ITEM()
RATIONAL_B_SPLINE_CURVE((1.01190199115935,1.01846995640957,1.02425882037767))
REPRESENTATION_ITEM('')
);
#982=(
BOUNDED_CURVE()
B_SPLINE_CURVE(2,(#32894,#32895,#32896),.UNSPECIFIED.,.F.,.F.)
B_SPLINE_CURVE_WITH_KNOTS((3,3),(0.0850178447349258,0.133529115174433),
 .UNSPECIFIED.)
CURVE()
GEOMETRIC_REPRESENTATION_ITEM()
RATIONAL_B_SPLINE_CURVE((1.00008344962585,1.00006598064918,1.00000140604823))
REPRESENTATION_ITEM('')
);
#983=(
BOUNDED_CURVE()
B_SPLINE_CURVE(2,(#32917,#32918,#32919),.UNSPECIFIED.,.F.,.F.)
B_SPLINE_CURVE_WITH_KNOTS((3,3),(0.00295018481962982,0.0985937601702449),
 .UNSPECIFIED.)
CURVE()
GEOMETRIC_REPRESENTATION_ITEM()
RATIONAL_B_SPLINE_CURVE((1.00000995626948,1.00016837897441,1.00013448693778))
REPRESENTATION_ITEM('')
);
#984=(
BOUNDED_CURVE()
B_SPLINE_CURVE(2,(#32922,#32923,#32924),.UNSPECIFIED.,.F.,.F.)
B_SPLINE_CURVE_WITH_KNOTS((3,3),(0.000473184985766772,0.0515065306432952),
 .UNSPECIFIED.)
CURVE()
GEOMETRIC_REPRESENTATION_ITEM()
RATIONAL_B_SPLINE_CURVE((1.00001807280714,1.00098893623079,1.00115754364118))
REPRESENTATION_ITEM('')
);
#985=(
BOUNDED_CURVE()
B_SPLINE_CURVE(2,(#32929,#32930,#32931),.UNSPECIFIED.,.F.,.F.)
B_SPLINE_CURVE_WITH_KNOTS((3,3),(0.072955690935184,0.123986559684228),
 .UNSPECIFIED.)
CURVE()
GEOMETRIC_REPRESENTATION_ITEM()
RATIONAL_B_SPLINE_CURVE((1.00116052526042,1.00099293482093,1.00002308400869))
REPRESENTATION_ITEM('')
);
#986=(
BOUNDED_CURVE()
B_SPLINE_CURVE(2,(#32941,#32942,#32943),.UNSPECIFIED.,.F.,.F.)
B_SPLINE_CURVE_WITH_KNOTS((3,3),(0.0642390630877414,0.159883011113205),
 .UNSPECIFIED.)
CURVE()
GEOMETRIC_REPRESENTATION_ITEM()
RATIONAL_B_SPLINE_CURVE((1.00013237845415,1.00016634217886,1.00000799154414))
REPRESENTATION_ITEM('')
);
#987=(
BOUNDED_CURVE()
B_SPLINE_CURVE(2,(#32946,#32947,#32948),.UNSPECIFIED.,.F.,.F.)
B_SPLINE_CURVE_WITH_KNOTS((3,3),(0.000526061815844321,0.0490373321941647),
 .UNSPECIFIED.)
CURVE()
GEOMETRIC_REPRESENTATION_ITEM()
RATIONAL_B_SPLINE_CURVE((1.00000140604826,1.00006598065031,1.00008344962734))
REPRESENTATION_ITEM('')
);
#988=(
BOUNDED_CURVE()
B_SPLINE_CURVE(2,(#32954,#32955,#32956),.UNSPECIFIED.,.F.,.F.)
B_SPLINE_CURVE_WITH_KNOTS((3,3),(0.0850178447349365,0.133529115174432),
 .UNSPECIFIED.)
CURVE()
GEOMETRIC_REPRESENTATION_ITEM()
RATIONAL_B_SPLINE_CURVE((1.00008344962713,1.0000659806502,1.00000140604825))
REPRESENTATION_ITEM('')
);
#989=(
BOUNDED_CURVE()
B_SPLINE_CURVE(2,(#32977,#32978,#32979),.UNSPECIFIED.,.F.,.F.)
B_SPLINE_CURVE_WITH_KNOTS((3,3),(0.0029501848132628,0.0985937601638959),
 .UNSPECIFIED.)
CURVE()
GEOMETRIC_REPRESENTATION_ITEM()
RATIONAL_B_SPLINE_CURVE((1.00000995626947,1.00016837897463,1.00013448693795))
REPRESENTATION_ITEM('')
);
#990=(
BOUNDED_CURVE()
B_SPLINE_CURVE(2,(#32982,#32983,#32984),.UNSPECIFIED.,.F.,.F.)
B_SPLINE_CURVE_WITH_KNOTS((3,3),(0.000473184985766719,0.0515065306433004),
 .UNSPECIFIED.)
CURVE()
GEOMETRIC_REPRESENTATION_ITEM()
RATIONAL_B_SPLINE_CURVE((1.00001807280713,1.00098893623043,1.00115754364076))
REPRESENTATION_ITEM('')
);
#991=(
BOUNDED_CURVE()
B_SPLINE_CURVE(2,(#32989,#32990,#32991),.UNSPECIFIED.,.F.,.F.)
B_SPLINE_CURVE_WITH_KNOTS((3,3),(0.0729556909351876,0.123986559684229),
 .UNSPECIFIED.)
CURVE()
GEOMETRIC_REPRESENTATION_ITEM()
RATIONAL_B_SPLINE_CURVE((1.00116052526059,1.00099293482108,1.0000230840087))
REPRESENTATION_ITEM('')
);
#992=(
BOUNDED_CURVE()
B_SPLINE_CURVE(2,(#33001,#33002,#33003),.UNSPECIFIED.,.F.,.F.)
B_SPLINE_CURVE_WITH_KNOTS((3,3),(0.0642390630877381,0.159883011113203),
 .UNSPECIFIED.)
CURVE()
GEOMETRIC_REPRESENTATION_ITEM()
RATIONAL_B_SPLINE_CURVE((1.00013237845351,1.00016634217805,1.0000079915441))
REPRESENTATION_ITEM('')
);
#993=(
BOUNDED_CURVE()
B_SPLINE_CURVE(2,(#33006,#33007,#33008),.UNSPECIFIED.,.F.,.F.)
B_SPLINE_CURVE_WITH_KNOTS((3,3),(0.000526061815846924,0.0490373321942014),
 .UNSPECIFIED.)
CURVE()
GEOMETRIC_REPRESENTATION_ITEM()
RATIONAL_B_SPLINE_CURVE((1.00000140604824,1.00006598064965,1.0000834496265))
REPRESENTATION_ITEM('')
);
#994=(
BOUNDED_CURVE()
B_SPLINE_CURVE(2,(#33014,#33015,#33016),.UNSPECIFIED.,.F.,.F.)
B_SPLINE_CURVE_WITH_KNOTS((3,3),(0.0850178447349793,0.133529115174434),
 .UNSPECIFIED.)
CURVE()
GEOMETRIC_REPRESENTATION_ITEM()
RATIONAL_B_SPLINE_CURVE((1.00008344962783,1.00006598065075,1.00000140604826))
REPRESENTATION_ITEM('')
);
#995=(
BOUNDED_CURVE()
B_SPLINE_CURVE(2,(#33037,#33038,#33039),.UNSPECIFIED.,.F.,.F.)
B_SPLINE_CURVE_WITH_KNOTS((3,3),(0.00295018481782719,0.0985937601684328),
 .UNSPECIFIED.)
CURVE()
GEOMETRIC_REPRESENTATION_ITEM()
RATIONAL_B_SPLINE_CURVE((1.00000995626944,1.00016837897378,1.00013448693728))
REPRESENTATION_ITEM('')
);
#996=(
BOUNDED_CURVE()
B_SPLINE_CURVE(2,(#33042,#33043,#33044),.UNSPECIFIED.,.F.,.F.)
B_SPLINE_CURVE_WITH_KNOTS((3,3),(0.00047318498576828,0.0515065306432978),
 .UNSPECIFIED.)
CURVE()
GEOMETRIC_REPRESENTATION_ITEM()
RATIONAL_B_SPLINE_CURVE((1.00001807280714,1.00098893623049,1.00115754364084))
REPRESENTATION_ITEM('')
);
#997=(
BOUNDED_CURVE()
B_SPLINE_CURVE(2,(#33049,#33050,#33051),.UNSPECIFIED.,.F.,.F.)
B_SPLINE_CURVE_WITH_KNOTS((3,3),(0.0729556909351862,0.123986559684229),
 .UNSPECIFIED.)
CURVE()
GEOMETRIC_REPRESENTATION_ITEM()
RATIONAL_B_SPLINE_CURVE((1.00116052526039,1.00099293482091,1.00002308400869))
REPRESENTATION_ITEM('')
);
#998=(
BOUNDED_CURVE()
B_SPLINE_CURVE(2,(#33061,#33062,#33063),.UNSPECIFIED.,.F.,.F.)
B_SPLINE_CURVE_WITH_KNOTS((3,3),(0.0642390630877591,0.159883011113204),
 .UNSPECIFIED.)
CURVE()
GEOMETRIC_REPRESENTATION_ITEM()
RATIONAL_B_SPLINE_CURVE((1.00013237845324,1.00016634217771,1.00000799154408))
REPRESENTATION_ITEM('')
);
#999=(
BOUNDED_CURVE()
B_SPLINE_CURVE(2,(#33066,#33067,#33068),.UNSPECIFIED.,.F.,.F.)
B_SPLINE_CURVE_WITH_KNOTS((3,3),(0.000526061815843999,0.0490373321941597),
 .UNSPECIFIED.)
CURVE()
GEOMETRIC_REPRESENTATION_ITEM()
RATIONAL_B_SPLINE_CURVE((1.00000140604825,1.00006598065026,1.00008344962727))
REPRESENTATION_ITEM('')
);
#1000=(
BOUNDED_CURVE()
B_SPLINE_CURVE(2,(#33074,#33075,#33076),.UNSPECIFIED.,.F.,.F.)
B_SPLINE_CURVE_WITH_KNOTS((3,3),(0.085017844734947,0.133529115174433),
 .UNSPECIFIED.)
CURVE()
GEOMETRIC_REPRESENTATION_ITEM()
RATIONAL_B_SPLINE_CURVE((1.00008344962705,1.00006598065013,1.00000140604825))
REPRESENTATION_ITEM('')
);
#1001=(
BOUNDED_CURVE()
B_SPLINE_CURVE(2,(#33097,#33098,#33099),.UNSPECIFIED.,.F.,.F.)
B_SPLINE_CURVE_WITH_KNOTS((3,3),(0.00295018481896423,0.0985937601695785),
 .UNSPECIFIED.)
CURVE()
GEOMETRIC_REPRESENTATION_ITEM()
RATIONAL_B_SPLINE_CURVE((1.00000995626949,1.00016837897465,1.00013448693797))
REPRESENTATION_ITEM('')
);
#1002=(
BOUNDED_CURVE()
B_SPLINE_CURVE(2,(#33102,#33103,#33104),.UNSPECIFIED.,.F.,.F.)
B_SPLINE_CURVE_WITH_KNOTS((3,3),(0.000473184985764736,0.0515065306432933),
 .UNSPECIFIED.)
CURVE()
GEOMETRIC_REPRESENTATION_ITEM()
RATIONAL_B_SPLINE_CURVE((1.00001807280714,1.00098893623083,1.00115754364123))
REPRESENTATION_ITEM('')
);
#1003=(
BOUNDED_CURVE()
B_SPLINE_CURVE(2,(#33109,#33110,#33111),.UNSPECIFIED.,.F.,.F.)
B_SPLINE_CURVE_WITH_KNOTS((3,3),(0.0729556909351823,0.123986559684223),
 .UNSPECIFIED.)
CURVE()
GEOMETRIC_REPRESENTATION_ITEM()
RATIONAL_B_SPLINE_CURVE((1.0011605252602,1.00099293482075,1.00002308400869))
REPRESENTATION_ITEM('')
);
#1004=(
BOUNDED_CURVE()
B_SPLINE_CURVE(2,(#33121,#33122,#33123),.UNSPECIFIED.,.F.,.F.)
B_SPLINE_CURVE_WITH_KNOTS((3,3),(0.0642390630877405,0.159883011113205),
 .UNSPECIFIED.)
CURVE()
GEOMETRIC_REPRESENTATION_ITEM()
RATIONAL_B_SPLINE_CURVE((1.0001323784534,1.00016634217792,1.00000799154409))
REPRESENTATION_ITEM('')
);
#1005=(
BOUNDED_CURVE()
B_SPLINE_CURVE(2,(#33126,#33127,#33128),.UNSPECIFIED.,.F.,.F.)
B_SPLINE_CURVE_WITH_KNOTS((3,3),(0.000526061815841318,0.0490373321941963),
 .UNSPECIFIED.)
CURVE()
GEOMETRIC_REPRESENTATION_ITEM()
RATIONAL_B_SPLINE_CURVE((1.00000140604824,1.00006598064947,1.00008344962627))
REPRESENTATION_ITEM('')
);
#1006=(
BOUNDED_CURVE()
B_SPLINE_CURVE(2,(#33134,#33135,#33136),.UNSPECIFIED.,.F.,.F.)
B_SPLINE_CURVE_WITH_KNOTS((3,3),(0.0850178447349235,0.133529115174428),
 .UNSPECIFIED.)
CURVE()
GEOMETRIC_REPRESENTATION_ITEM()
RATIONAL_B_SPLINE_CURVE((1.00008344962713,1.0000659806502,1.00000140604825))
REPRESENTATION_ITEM('')
);
#1007=(
BOUNDED_CURVE()
B_SPLINE_CURVE(2,(#33157,#33158,#33159),.UNSPECIFIED.,.F.,.F.)
B_SPLINE_CURVE_WITH_KNOTS((3,3),(0.00295018482096791,0.0985937601715863),
 .UNSPECIFIED.)
CURVE()
GEOMETRIC_REPRESENTATION_ITEM()
RATIONAL_B_SPLINE_CURVE((1.00000995626946,1.00016837897397,1.00013448693743))
REPRESENTATION_ITEM('')
);
#1008=(
BOUNDED_CURVE()
B_SPLINE_CURVE(2,(#33162,#33163,#33164),.UNSPECIFIED.,.F.,.F.)
B_SPLINE_CURVE_WITH_KNOTS((3,3),(0.000474651750499241,0.0515079945407172),
 .UNSPECIFIED.)
CURVE()
GEOMETRIC_REPRESENTATION_ITEM()
RATIONAL_B_SPLINE_CURVE((1.0000181290019,1.00098899015283,1.00115759524465))
REPRESENTATION_ITEM('')
);
#1009=(
BOUNDED_CURVE()
B_SPLINE_CURVE(2,(#33169,#33170,#33171),.UNSPECIFIED.,.F.,.F.)
B_SPLINE_CURVE_WITH_KNOTS((3,3),(0.73383872017312,0.777722409416427),
 .UNSPECIFIED.)
CURVE()
GEOMETRIC_REPRESENTATION_ITEM()
RATIONAL_B_SPLINE_CURVE((1.02425882037767,1.01846995640957,1.01190199115935))
REPRESENTATION_ITEM('')
);
#1010=(
BOUNDED_CURVE()
B_SPLINE_CURVE(2,(#33208,#33209,#33210),.UNSPECIFIED.,.F.,.F.)
B_SPLINE_CURVE_WITH_KNOTS((3,3),(0.000478034212987197,0.0489893198676105),
 .UNSPECIFIED.)
CURVE()
GEOMETRIC_REPRESENTATION_ITEM()
RATIONAL_B_SPLINE_CURVE((1.00000127717582,1.00006584948475,1.00008331617371))
REPRESENTATION_ITEM('')
);
#1011=(
BOUNDED_CURVE()
B_SPLINE_CURVE(2,(#33214,#33215,#33216),.UNSPECIFIED.,.F.,.F.)
B_SPLINE_CURVE_WITH_KNOTS((3,3),(0.0849651357209515,0.133476420621903),
 .UNSPECIFIED.)
CURVE()
GEOMETRIC_REPRESENTATION_ITEM()
RATIONAL_B_SPLINE_CURVE((1.00008331617332,1.00006584948388,1.00000127717582))
REPRESENTATION_ITEM('')
);
#1012=(
BOUNDED_CURVE()
B_SPLINE_CURVE(2,(#33225,#33226,#33227),.UNSPECIFIED.,.F.,.F.)
B_SPLINE_CURVE_WITH_KNOTS((3,3),(0.0642390630877396,0.159883011113208),
 .UNSPECIFIED.)
CURVE()
GEOMETRIC_REPRESENTATION_ITEM()
RATIONAL_B_SPLINE_CURVE((1.00013237845388,1.00016634217853,1.00000799154412))
REPRESENTATION_ITEM('')
);
#1013=(
BOUNDED_CURVE()
B_SPLINE_CURVE(2,(#33261,#33262,#33263),.UNSPECIFIED.,.F.,.F.)
B_SPLINE_CURVE_WITH_KNOTS((3,3),(0.0850174365043124,0.13352847207702),
 .UNSPECIFIED.)
CURVE()
GEOMETRIC_REPRESENTATION_ITEM()
RATIONAL_B_SPLINE_CURVE((1.00008336789045,1.00006587559557,1.00000127768044))
REPRESENTATION_ITEM('')
);
#1014=(
BOUNDED_CURVE()
B_SPLINE_CURVE(2,(#33266,#33267,#33268),.UNSPECIFIED.,.F.,.F.)
B_SPLINE_CURVE_WITH_KNOTS((3,3),(0.0029501848107848,0.0985937601613831),
 .UNSPECIFIED.)
CURVE()
GEOMETRIC_REPRESENTATION_ITEM()
RATIONAL_B_SPLINE_CURVE((1.00000995626935,1.00016837897274,1.00013448693644))
REPRESENTATION_ITEM('')
);
#1015=(
BOUNDED_CURVE()
B_SPLINE_CURVE(2,(#33283,#33284,#33285),.UNSPECIFIED.,.F.,.F.)
B_SPLINE_CURVE_WITH_KNOTS((3,3),(0.00295018481829096,0.0985937601689052),
 .UNSPECIFIED.)
CURVE()
GEOMETRIC_REPRESENTATION_ITEM()
RATIONAL_B_SPLINE_CURVE((1.00000995626949,1.00016837897471,1.00013448693802))
REPRESENTATION_ITEM('')
);
#1016=(
BOUNDED_CURVE()
B_SPLINE_CURVE(2,(#33288,#33289,#33290),.UNSPECIFIED.,.F.,.F.)
B_SPLINE_CURVE_WITH_KNOTS((3,3),(0.000474646853444211,0.0515079897376496),
 .UNSPECIFIED.)
CURVE()
GEOMETRIC_REPRESENTATION_ITEM()
RATIONAL_B_SPLINE_CURVE((1.00001812881482,1.00098899000409,1.00115759513441))
REPRESENTATION_ITEM('')
);
#1017=(
BOUNDED_CURVE()
B_SPLINE_CURVE(2,(#33295,#33296,#33297),.UNSPECIFIED.,.F.,.F.)
B_SPLINE_CURVE_WITH_KNOTS((3,3),(0.733838720173112,0.777722409416418),
 .UNSPECIFIED.)
CURVE()
GEOMETRIC_REPRESENTATION_ITEM()
RATIONAL_B_SPLINE_CURVE((1.02425882037767,1.01846995640957,1.01190199115935))
REPRESENTATION_ITEM('')
);
#1018=(
BOUNDED_CURVE()
B_SPLINE_CURVE(2,(#33304,#33305,#33306),.UNSPECIFIED.,.F.,.F.)
B_SPLINE_CURVE_WITH_KNOTS((3,3),(0.000478034212982558,0.0489893198675958),
 .UNSPECIFIED.)
CURVE()
GEOMETRIC_REPRESENTATION_ITEM()
RATIONAL_B_SPLINE_CURVE((1.00000127717582,1.00006584948482,1.0000833161738))
REPRESENTATION_ITEM('')
);
#1019=(
BOUNDED_CURVE()
B_SPLINE_CURVE(2,(#33310,#33311,#33312),.UNSPECIFIED.,.F.,.F.)
B_SPLINE_CURVE_WITH_KNOTS((3,3),(0.084965135720964,0.133476420621902),
 .UNSPECIFIED.)
CURVE()
GEOMETRIC_REPRESENTATION_ITEM()
RATIONAL_B_SPLINE_CURVE((1.00008331617392,1.00006584948435,1.00000127717583))
REPRESENTATION_ITEM('')
);
#1020=(
BOUNDED_CURVE()
B_SPLINE_CURVE(2,(#33321,#33322,#33323),.UNSPECIFIED.,.F.,.F.)
B_SPLINE_CURVE_WITH_KNOTS((3,3),(0.0642390630877467,0.159883011113209),
 .UNSPECIFIED.)
CURVE()
GEOMETRIC_REPRESENTATION_ITEM()
RATIONAL_B_SPLINE_CURVE((1.00013237845391,1.00016634217857,1.00000799154412))
REPRESENTATION_ITEM('')
);
#1021=(
BOUNDED_CURVE()
B_SPLINE_CURVE(2,(#33339,#33340,#33341),.UNSPECIFIED.,.F.,.F.)
B_SPLINE_CURVE_WITH_KNOTS((3,3),(0.00295018480947799,0.0985937601601038),
 .UNSPECIFIED.)
CURVE()
GEOMETRIC_REPRESENTATION_ITEM()
RATIONAL_B_SPLINE_CURVE((1.00000995626944,1.00016837897428,1.00013448693767))
REPRESENTATION_ITEM('')
);
#1022=(
BOUNDED_CURVE()
B_SPLINE_CURVE(2,(#33344,#33345,#33346),.UNSPECIFIED.,.F.,.F.)
B_SPLINE_CURVE_WITH_KNOTS((3,3),(0.000474646853447348,0.0515079897376581),
 .UNSPECIFIED.)
CURVE()
GEOMETRIC_REPRESENTATION_ITEM()
RATIONAL_B_SPLINE_CURVE((1.00001812881482,1.00098899000384,1.00115759513413))
REPRESENTATION_ITEM('')
);
#1023=(
BOUNDED_CURVE()
B_SPLINE_CURVE(2,(#33351,#33352,#33353),.UNSPECIFIED.,.F.,.F.)
B_SPLINE_CURVE_WITH_KNOTS((3,3),(0.733838720173119,0.777722409416428),
 .UNSPECIFIED.)
CURVE()
GEOMETRIC_REPRESENTATION_ITEM()
RATIONAL_B_SPLINE_CURVE((1.02425882037767,1.01846995640957,1.01190199115935))
REPRESENTATION_ITEM('')
);
#1024=(
BOUNDED_CURVE()
B_SPLINE_CURVE(2,(#33360,#33361,#33362),.UNSPECIFIED.,.F.,.F.)
B_SPLINE_CURVE_WITH_KNOTS((3,3),(0.00047803421298473,0.0489893198675923),
 .UNSPECIFIED.)
CURVE()
GEOMETRIC_REPRESENTATION_ITEM()
RATIONAL_B_SPLINE_CURVE((1.00000127717583,1.00006584948522,1.00008331617429))
REPRESENTATION_ITEM('')
);
#1025=(
BOUNDED_CURVE()
B_SPLINE_CURVE(2,(#33366,#33367,#33368),.UNSPECIFIED.,.F.,.F.)
B_SPLINE_CURVE_WITH_KNOTS((3,3),(0.0849651357209518,0.133476420621905),
 .UNSPECIFIED.)
CURVE()
GEOMETRIC_REPRESENTATION_ITEM()
RATIONAL_B_SPLINE_CURVE((1.00008331617313,1.00006584948373,1.00000127717582))
REPRESENTATION_ITEM('')
);
#1026=(
BOUNDED_CURVE()
B_SPLINE_CURVE(2,(#33377,#33378,#33379),.UNSPECIFIED.,.F.,.F.)
B_SPLINE_CURVE_WITH_KNOTS((3,3),(0.0642390630877352,0.15988301111321),
 .UNSPECIFIED.)
CURVE()
GEOMETRIC_REPRESENTATION_ITEM()
RATIONAL_B_SPLINE_CURVE((1.00013237845418,1.0001663421789,1.00000799154414))
REPRESENTATION_ITEM('')
);
#1027=(
BOUNDED_CURVE()
B_SPLINE_CURVE(2,(#33395,#33396,#33397),.UNSPECIFIED.,.F.,.F.)
B_SPLINE_CURVE_WITH_KNOTS((3,3),(0.00295018481006126,0.0985937601607044),
 .UNSPECIFIED.)
CURVE()
GEOMETRIC_REPRESENTATION_ITEM()
RATIONAL_B_SPLINE_CURVE((1.00000995626951,1.00016837897535,1.00013448693852))
REPRESENTATION_ITEM('')
);
#1028=(
BOUNDED_CURVE()
B_SPLINE_CURVE(2,(#33400,#33401,#33402),.UNSPECIFIED.,.F.,.F.)
B_SPLINE_CURVE_WITH_KNOTS((3,3),(0.000474646853442338,0.0515079897376532),
 .UNSPECIFIED.)
CURVE()
GEOMETRIC_REPRESENTATION_ITEM()
RATIONAL_B_SPLINE_CURVE((1.00001812881482,1.00098899000395,1.00115759513426))
REPRESENTATION_ITEM('')
);
#1029=(
BOUNDED_CURVE()
B_SPLINE_CURVE(2,(#33407,#33408,#33409),.UNSPECIFIED.,.F.,.F.)
B_SPLINE_CURVE_WITH_KNOTS((3,3),(0.733838720173123,0.777722409416431),
 .UNSPECIFIED.)
CURVE()
GEOMETRIC_REPRESENTATION_ITEM()
RATIONAL_B_SPLINE_CURVE((1.02425882037767,1.01846995640957,1.01190199115935))
REPRESENTATION_ITEM('')
);
#1030=(
BOUNDED_CURVE()
B_SPLINE_CURVE(2,(#33416,#33417,#33418),.UNSPECIFIED.,.F.,.F.)
B_SPLINE_CURVE_WITH_KNOTS((3,3),(0.000478034212989242,0.0489893198676443),
 .UNSPECIFIED.)
CURVE()
GEOMETRIC_REPRESENTATION_ITEM()
RATIONAL_B_SPLINE_CURVE((1.0000012771758,1.00006584948372,1.0000833161724))
REPRESENTATION_ITEM('')
);
#1031=(
BOUNDED_CURVE()
B_SPLINE_CURVE(2,(#33422,#33423,#33424),.UNSPECIFIED.,.F.,.F.)
B_SPLINE_CURVE_WITH_KNOTS((3,3),(0.0849651357209273,0.133476420621905),
 .UNSPECIFIED.)
CURVE()
GEOMETRIC_REPRESENTATION_ITEM()
RATIONAL_B_SPLINE_CURVE((1.00008331617315,1.00006584948374,1.00000127717582))
REPRESENTATION_ITEM('')
);
#1032=(
BOUNDED_CURVE()
B_SPLINE_CURVE(2,(#33433,#33434,#33435),.UNSPECIFIED.,.F.,.F.)
B_SPLINE_CURVE_WITH_KNOTS((3,3),(0.0642390630877532,0.159883011113204),
 .UNSPECIFIED.)
CURVE()
GEOMETRIC_REPRESENTATION_ITEM()
RATIONAL_B_SPLINE_CURVE((1.00013237845329,1.00016634217778,1.00000799154408))
REPRESENTATION_ITEM('')
);
#1033=(
BOUNDED_CURVE()
B_SPLINE_CURVE(2,(#33451,#33452,#33453),.UNSPECIFIED.,.F.,.F.)
B_SPLINE_CURVE_WITH_KNOTS((3,3),(0.00295018481501485,0.0985937601656302),
 .UNSPECIFIED.)
CURVE()
GEOMETRIC_REPRESENTATION_ITEM()
RATIONAL_B_SPLINE_CURVE((1.00000995626945,1.0001683789741,1.00013448693753))
REPRESENTATION_ITEM('')
);
#1034=(
BOUNDED_CURVE()
B_SPLINE_CURVE(2,(#33456,#33457,#33458),.UNSPECIFIED.,.F.,.F.)
B_SPLINE_CURVE_WITH_KNOTS((3,3),(0.000474646853444173,0.0515079897376518),
 .UNSPECIFIED.)
CURVE()
GEOMETRIC_REPRESENTATION_ITEM()
RATIONAL_B_SPLINE_CURVE((1.00001812881482,1.00098899000411,1.00115759513444))
REPRESENTATION_ITEM('')
);
#1035=(
BOUNDED_CURVE()
B_SPLINE_CURVE(2,(#33463,#33464,#33465),.UNSPECIFIED.,.F.,.F.)
B_SPLINE_CURVE_WITH_KNOTS((3,3),(0.733838720173153,0.777722409416459),
 .UNSPECIFIED.)
CURVE()
GEOMETRIC_REPRESENTATION_ITEM()
RATIONAL_B_SPLINE_CURVE((1.02425882037767,1.01846995640957,1.01190199115935))
REPRESENTATION_ITEM('')
);
#1036=(
BOUNDED_CURVE()
B_SPLINE_CURVE(2,(#33472,#33473,#33474),.UNSPECIFIED.,.F.,.F.)
B_SPLINE_CURVE_WITH_KNOTS((3,3),(0.000478034212985405,0.0489893198675976),
 .UNSPECIFIED.)
CURVE()
GEOMETRIC_REPRESENTATION_ITEM()
RATIONAL_B_SPLINE_CURVE((1.00000127717583,1.00006584948535,1.00008331617446))
REPRESENTATION_ITEM('')
);
#1037=(
BOUNDED_CURVE()
B_SPLINE_CURVE(2,(#33478,#33479,#33480),.UNSPECIFIED.,.F.,.F.)
B_SPLINE_CURVE_WITH_KNOTS((3,3),(0.0849651357209773,0.133476420621906),
 .UNSPECIFIED.)
CURVE()
GEOMETRIC_REPRESENTATION_ITEM()
RATIONAL_B_SPLINE_CURVE((1.00008331617476,1.00006584948501,1.00000127717584))
REPRESENTATION_ITEM('')
);
#1038=(
BOUNDED_CURVE()
B_SPLINE_CURVE(2,(#33489,#33490,#33491),.UNSPECIFIED.,.F.,.F.)
B_SPLINE_CURVE_WITH_KNOTS((3,3),(0.0642390630877643,0.159883011113209),
 .UNSPECIFIED.)
CURVE()
GEOMETRIC_REPRESENTATION_ITEM()
RATIONAL_B_SPLINE_CURVE((1.00013237845267,1.000166342177,1.00000799154405))
REPRESENTATION_ITEM('')
);
#1039=(
BOUNDED_CURVE()
B_SPLINE_CURVE(2,(#33507,#33508,#33509),.UNSPECIFIED.,.F.,.F.)
B_SPLINE_CURVE_WITH_KNOTS((3,3),(0.00295018481095983,0.0985937601615901),
 .UNSPECIFIED.)
CURVE()
GEOMETRIC_REPRESENTATION_ITEM()
RATIONAL_B_SPLINE_CURVE((1.00000995626948,1.00016837897492,1.00013448693818))
REPRESENTATION_ITEM('')
);
#1040=(
BOUNDED_CURVE()
B_SPLINE_CURVE(2,(#33512,#33513,#33514),.UNSPECIFIED.,.F.,.F.)
B_SPLINE_CURVE_WITH_KNOTS((3,3),(0.000474646853443493,0.0515079897376577),
 .UNSPECIFIED.)
CURVE()
GEOMETRIC_REPRESENTATION_ITEM()
RATIONAL_B_SPLINE_CURVE((1.00001812881482,1.00098899000373,1.00115759513399))
REPRESENTATION_ITEM('')
);
#1041=(
BOUNDED_CURVE()
B_SPLINE_CURVE(2,(#33519,#33520,#33521),.UNSPECIFIED.,.F.,.F.)
B_SPLINE_CURVE_WITH_KNOTS((3,3),(0.733838720173112,0.77772240941642),
 .UNSPECIFIED.)
CURVE()
GEOMETRIC_REPRESENTATION_ITEM()
RATIONAL_B_SPLINE_CURVE((1.02425882037767,1.01846995640957,1.01190199115935))
REPRESENTATION_ITEM('')
);
#1042=(
BOUNDED_CURVE()
B_SPLINE_CURVE(2,(#33528,#33529,#33530),.UNSPECIFIED.,.F.,.F.)
B_SPLINE_CURVE_WITH_KNOTS((3,3),(0.000478034212986085,0.0489893198676214),
 .UNSPECIFIED.)
CURVE()
GEOMETRIC_REPRESENTATION_ITEM()
RATIONAL_B_SPLINE_CURVE((1.00000127717582,1.00006584948496,1.00008331617397))
REPRESENTATION_ITEM('')
);
#1043=(
BOUNDED_CURVE()
B_SPLINE_CURVE(2,(#33534,#33535,#33536),.UNSPECIFIED.,.F.,.F.)
B_SPLINE_CURVE_WITH_KNOTS((3,3),(0.0849651357209684,0.133476420621907),
 .UNSPECIFIED.)
CURVE()
GEOMETRIC_REPRESENTATION_ITEM()
RATIONAL_B_SPLINE_CURVE((1.00008331617452,1.00006584948482,1.00000127717584))
REPRESENTATION_ITEM('')
);
#1044=(
BOUNDED_CURVE()
B_SPLINE_CURVE(2,(#33545,#33546,#33547),.UNSPECIFIED.,.F.,.F.)
B_SPLINE_CURVE_WITH_KNOTS((3,3),(0.0642390630877575,0.159883011113204),
 .UNSPECIFIED.)
CURVE()
GEOMETRIC_REPRESENTATION_ITEM()
RATIONAL_B_SPLINE_CURVE((1.00013237845349,1.00016634217804,1.0000079915441))
REPRESENTATION_ITEM('')
);
#1045=(
BOUNDED_CURVE()
B_SPLINE_CURVE(2,(#33569,#33570,#33571),.UNSPECIFIED.,.F.,.F.)
B_SPLINE_CURVE_WITH_KNOTS((3,3),(0.000478034212987892,0.0489893198676202),
 .UNSPECIFIED.)
CURVE()
GEOMETRIC_REPRESENTATION_ITEM()
RATIONAL_B_SPLINE_CURVE((1.00000127717582,1.00006584948477,1.00008331617373))
REPRESENTATION_ITEM('')
);
#1046=(
BOUNDED_CURVE()
B_SPLINE_CURVE(2,(#33586,#33587,#33588),.UNSPECIFIED.,.F.,.F.)
B_SPLINE_CURVE_WITH_KNOTS((3,3),(0.002950184815266,0.0985937601658534),
 .UNSPECIFIED.)
CURVE()
GEOMETRIC_REPRESENTATION_ITEM()
RATIONAL_B_SPLINE_CURVE((1.00000995626939,1.00016837897316,1.00013448693678))
REPRESENTATION_ITEM('')
);
#1047=(
BOUNDED_CURVE()
B_SPLINE_CURVE(2,(#33591,#33592,#33593),.UNSPECIFIED.,.F.,.F.)
B_SPLINE_CURVE_WITH_KNOTS((3,3),(0.000474646853442315,0.051507989737653),
 .UNSPECIFIED.)
CURVE()
GEOMETRIC_REPRESENTATION_ITEM()
RATIONAL_B_SPLINE_CURVE((1.00001812881482,1.00098899000397,1.00115759513428))
REPRESENTATION_ITEM('')
);
#1048=(
BOUNDED_CURVE()
B_SPLINE_CURVE(2,(#33597,#33598,#33599),.UNSPECIFIED.,.F.,.F.)
B_SPLINE_CURVE_WITH_KNOTS((3,3),(0.733838720173123,0.777722409416431),
 .UNSPECIFIED.)
CURVE()
GEOMETRIC_REPRESENTATION_ITEM()
RATIONAL_B_SPLINE_CURVE((1.02425882037767,1.01846995640957,1.01190199115935))
REPRESENTATION_ITEM('')
);
#1049=(
BOUNDED_CURVE()
B_SPLINE_CURVE(2,(#33603,#33604,#33605),.UNSPECIFIED.,.F.,.F.)
B_SPLINE_CURVE_WITH_KNOTS((3,3),(0.0642390630877507,0.159883011113205),
 .UNSPECIFIED.)
CURVE()
GEOMETRIC_REPRESENTATION_ITEM()
RATIONAL_B_SPLINE_CURVE((1.00013237845344,1.00016634217798,1.00000799154409))
REPRESENTATION_ITEM('')
);
#1064=(
BOUNDED_SURFACE()
B_SPLINE_SURFACE(5,2,((#24386,#24387,#24388,#24389,#24390,#24391,#24392,
#24393,#24394),(#24395,#24396,#24397,#24398,#24399,#24400,#24401,#24402,
#24403),(#24404,#24405,#24406,#24407,#24408,#24409,#24410,#24411,#24412),
(#24413,#24414,#24415,#24416,#24417,#24418,#24419,#24420,#24421),(#24422,
#24423,#24424,#24425,#24426,#24427,#24428,#24429,#24430),(#24431,#24432,
#24433,#24434,#24435,#24436,#24437,#24438,#24439),(#24440,#24441,#24442,
#24443,#24444,#24445,#24446,#24447,#24448),(#24449,#24450,#24451,#24452,
#24453,#24454,#24455,#24456,#24457),(#24458,#24459,#24460,#24461,#24462,
#24463,#24464,#24465,#24466),(#24467,#24468,#24469,#24470,#24471,#24472,
#24473,#24474,#24475),(#24476,#24477,#24478,#24479,#24480,#24481,#24482,
#24483,#24484),(#24485,#24486,#24487,#24488,#24489,#24490,#24491,#24492,
#24493),(#24494,#24495,#24496,#24497,#24498,#24499,#24500,#24501,#24502),
(#24503,#24504,#24505,#24506,#24507,#24508,#24509,#24510,#24511),(#24512,
#24513,#24514,#24515,#24516,#24517,#24518,#24519,#24520),(#24521,#24522,
#24523,#24524,#24525,#24526,#24527,#24528,#24529),(#24530,#24531,#24532,
#24533,#24534,#24535,#24536,#24537,#24538),(#24539,#24540,#24541,#24542,
#24543,#24544,#24545,#24546,#24547),(#24548,#24549,#24550,#24551,#24552,
#24553,#24554,#24555,#24556),(#24557,#24558,#24559,#24560,#24561,#24562,
#24563,#24564,#24565),(#24566,#24567,#24568,#24569,#24570,#24571,#24572,
#24573,#24574),(#24575,#24576,#24577,#24578,#24579,#24580,#24581,#24582,
#24583),(#24584,#24585,#24586,#24587,#24588,#24589,#24590,#24591,#24592),
(#24593,#24594,#24595,#24596,#24597,#24598,#24599,#24600,#24601),(#24602,
#24603,#24604,#24605,#24606,#24607,#24608,#24609,#24610),(#24611,#24612,
#24613,#24614,#24615,#24616,#24617,#24618,#24619),(#24620,#24621,#24622,
#24623,#24624,#24625,#24626,#24627,#24628),(#24629,#24630,#24631,#24632,
#24633,#24634,#24635,#24636,#24637),(#24638,#24639,#24640,#24641,#24642,
#24643,#24644,#24645,#24646),(#24647,#24648,#24649,#24650,#24651,#24652,
#24653,#24654,#24655)),.UNSPECIFIED.,.F.,.T.,.F.)
B_SPLINE_SURFACE_WITH_KNOTS((6,1,1,1,1,1,1,1,1,1,1,1,1,1,1,1,1,1,1,1,1,
1,1,1,1,6),(3,2,2,2,3),(-1.,-0.96,-0.92,-0.88,-0.84,-0.8,-0.76,-0.72,-0.68,
-0.64,-0.6,-0.56,-0.52,-0.48,-0.44,-0.4,-0.36,-0.32,-0.28,-0.24,-0.2,-0.16,
-0.12,-0.08,-0.04,0.),(0.,1.5707963267949,3.14159265358979,4.71238898038469,
6.28318530717959),.UNSPECIFIED.)
GEOMETRIC_REPRESENTATION_ITEM()
RATIONAL_B_SPLINE_SURFACE(((1.,0.707106781186548,1.,0.707106781186548,1.,
0.707106781186548,1.,0.707106781186548,1.),(1.,0.707106781186548,1.,0.707106781186548,
1.,0.707106781186548,1.,0.707106781186548,1.),(1.,0.707106781186548,1.,
0.707106781186548,1.,0.707106781186548,1.,0.707106781186548,1.),(1.,0.707106781186548,
1.,0.707106781186548,1.,0.707106781186548,1.,0.707106781186548,1.),(1.,
0.707106781186548,1.,0.707106781186548,1.,0.707106781186548,1.,0.707106781186548,
1.),(1.,0.707106781186548,1.,0.707106781186548,1.,0.707106781186548,1.,
0.707106781186548,1.),(1.,0.707106781186548,1.,0.707106781186548,1.,0.707106781186548,
1.,0.707106781186548,1.),(1.,0.707106781186548,1.,0.707106781186548,1.,
0.707106781186548,1.,0.707106781186548,1.),(1.,0.707106781186548,1.,0.707106781186548,
1.,0.707106781186548,1.,0.707106781186548,1.),(1.,0.707106781186548,1.,
0.707106781186548,1.,0.707106781186548,1.,0.707106781186548,1.),(1.,0.707106781186548,
1.,0.707106781186548,1.,0.707106781186548,1.,0.707106781186548,1.),(1.,
0.707106781186548,1.,0.707106781186548,1.,0.707106781186548,1.,0.707106781186548,
1.),(1.,0.707106781186548,1.,0.707106781186548,1.,0.707106781186548,1.,
0.707106781186548,1.),(1.,0.707106781186548,1.,0.707106781186548,1.,0.707106781186548,
1.,0.707106781186548,1.),(1.,0.707106781186548,1.,0.707106781186548,1.,
0.707106781186548,1.,0.707106781186548,1.),(1.,0.707106781186548,1.,0.707106781186548,
1.,0.707106781186548,1.,0.707106781186548,1.),(1.,0.707106781186548,1.,
0.707106781186548,1.,0.707106781186548,1.,0.707106781186548,1.),(1.,0.707106781186548,
1.,0.707106781186548,1.,0.707106781186548,1.,0.707106781186548,1.),(1.,
0.707106781186548,1.,0.707106781186548,1.,0.707106781186548,1.,0.707106781186548,
1.),(1.,0.707106781186548,1.,0.707106781186548,1.,0.707106781186548,1.,
0.707106781186548,1.),(1.,0.707106781186548,1.,0.707106781186548,1.,0.707106781186548,
1.,0.707106781186548,1.),(1.,0.707106781186548,1.,0.707106781186548,1.,
0.707106781186548,1.,0.707106781186548,1.),(1.,0.707106781186548,1.,0.707106781186548,
1.,0.707106781186548,1.,0.707106781186548,1.),(1.,0.707106781186548,1.,
0.707106781186548,1.,0.707106781186548,1.,0.707106781186548,1.),(1.,0.707106781186548,
1.,0.707106781186548,1.,0.707106781186548,1.,0.707106781186548,1.),(1.,
0.707106781186548,1.,0.707106781186548,1.,0.707106781186548,1.,0.707106781186548,
1.),(1.,0.707106781186548,1.,0.707106781186548,1.,0.707106781186548,1.,
0.707106781186548,1.),(1.,0.707106781186548,1.,0.707106781186548,1.,0.707106781186548,
1.,0.707106781186548,1.),(1.,0.707106781186548,1.,0.707106781186548,1.,
0.707106781186548,1.,0.707106781186548,1.),(1.,0.707106781186548,1.,0.707106781186548,
1.,0.707106781186548,1.,0.707106781186548,1.)))
REPRESENTATION_ITEM('')
SURFACE()
);
#1065=(
BOUNDED_SURFACE()
B_SPLINE_SURFACE(5,2,((#34945,#34946,#34947,#34948,#34949,#34950,#34951,
#34952,#34953),(#34954,#34955,#34956,#34957,#34958,#34959,#34960,#34961,
#34962),(#34963,#34964,#34965,#34966,#34967,#34968,#34969,#34970,#34971),
(#34972,#34973,#34974,#34975,#34976,#34977,#34978,#34979,#34980),(#34981,
#34982,#34983,#34984,#34985,#34986,#34987,#34988,#34989),(#34990,#34991,
#34992,#34993,#34994,#34995,#34996,#34997,#34998),(#34999,#35000,#35001,
#35002,#35003,#35004,#35005,#35006,#35007),(#35008,#35009,#35010,#35011,
#35012,#35013,#35014,#35015,#35016),(#35017,#35018,#35019,#35020,#35021,
#35022,#35023,#35024,#35025),(#35026,#35027,#35028,#35029,#35030,#35031,
#35032,#35033,#35034),(#35035,#35036,#35037,#35038,#35039,#35040,#35041,
#35042,#35043),(#35044,#35045,#35046,#35047,#35048,#35049,#35050,#35051,
#35052),(#35053,#35054,#35055,#35056,#35057,#35058,#35059,#35060,#35061),
(#35062,#35063,#35064,#35065,#35066,#35067,#35068,#35069,#35070),(#35071,
#35072,#35073,#35074,#35075,#35076,#35077,#35078,#35079),(#35080,#35081,
#35082,#35083,#35084,#35085,#35086,#35087,#35088),(#35089,#35090,#35091,
#35092,#35093,#35094,#35095,#35096,#35097),(#35098,#35099,#35100,#35101,
#35102,#35103,#35104,#35105,#35106),(#35107,#35108,#35109,#35110,#35111,
#35112,#35113,#35114,#35115),(#35116,#35117,#35118,#35119,#35120,#35121,
#35122,#35123,#35124),(#35125,#35126,#35127,#35128,#35129,#35130,#35131,
#35132,#35133),(#35134,#35135,#35136,#35137,#35138,#35139,#35140,#35141,
#35142),(#35143,#35144,#35145,#35146,#35147,#35148,#35149,#35150,#35151),
(#35152,#35153,#35154,#35155,#35156,#35157,#35158,#35159,#35160),(#35161,
#35162,#35163,#35164,#35165,#35166,#35167,#35168,#35169),(#35170,#35171,
#35172,#35173,#35174,#35175,#35176,#35177,#35178),(#35179,#35180,#35181,
#35182,#35183,#35184,#35185,#35186,#35187),(#35188,#35189,#35190,#35191,
#35192,#35193,#35194,#35195,#35196),(#35197,#35198,#35199,#35200,#35201,
#35202,#35203,#35204,#35205),(#35206,#35207,#35208,#35209,#35210,#35211,
#35212,#35213,#35214)),.UNSPECIFIED.,.F.,.T.,.F.)
B_SPLINE_SURFACE_WITH_KNOTS((6,1,1,1,1,1,1,1,1,1,1,1,1,1,1,1,1,1,1,1,1,
1,1,1,1,6),(3,2,2,2,3),(-1.,-0.96,-0.92,-0.88,-0.84,-0.8,-0.76,-0.72,-0.68,
-0.64,-0.6,-0.56,-0.52,-0.48,-0.44,-0.4,-0.36,-0.32,-0.28,-0.24,-0.2,-0.16,
-0.12,-0.08,-0.04,0.),(0.,1.5707963267949,3.14159265358979,4.71238898038469,
6.28318530717959),.UNSPECIFIED.)
GEOMETRIC_REPRESENTATION_ITEM()
RATIONAL_B_SPLINE_SURFACE(((1.,0.707106781186548,1.,0.707106781186548,1.,
0.707106781186548,1.,0.707106781186548,1.),(1.,0.707106781186548,1.,0.707106781186548,
1.,0.707106781186548,1.,0.707106781186548,1.),(1.,0.707106781186548,1.,
0.707106781186548,1.,0.707106781186548,1.,0.707106781186548,1.),(1.,0.707106781186548,
1.,0.707106781186548,1.,0.707106781186548,1.,0.707106781186548,1.),(1.,
0.707106781186548,1.,0.707106781186548,1.,0.707106781186548,1.,0.707106781186548,
1.),(1.,0.707106781186548,1.,0.707106781186548,1.,0.707106781186548,1.,
0.707106781186548,1.),(1.,0.707106781186548,1.,0.707106781186548,1.,0.707106781186548,
1.,0.707106781186548,1.),(1.,0.707106781186548,1.,0.707106781186548,1.,
0.707106781186548,1.,0.707106781186548,1.),(1.,0.707106781186548,1.,0.707106781186548,
1.,0.707106781186548,1.,0.707106781186548,1.),(1.,0.707106781186548,1.,
0.707106781186548,1.,0.707106781186548,1.,0.707106781186548,1.),(1.,0.707106781186548,
1.,0.707106781186548,1.,0.707106781186548,1.,0.707106781186548,1.),(1.,
0.707106781186548,1.,0.707106781186548,1.,0.707106781186548,1.,0.707106781186548,
1.),(1.,0.707106781186548,1.,0.707106781186548,1.,0.707106781186548,1.,
0.707106781186548,1.),(1.,0.707106781186548,1.,0.707106781186548,1.,0.707106781186548,
1.,0.707106781186548,1.),(1.,0.707106781186548,1.,0.707106781186548,1.,
0.707106781186548,1.,0.707106781186548,1.),(1.,0.707106781186548,1.,0.707106781186548,
1.,0.707106781186548,1.,0.707106781186548,1.),(1.,0.707106781186548,1.,
0.707106781186548,1.,0.707106781186548,1.,0.707106781186548,1.),(1.,0.707106781186548,
1.,0.707106781186548,1.,0.707106781186548,1.,0.707106781186548,1.),(1.,
0.707106781186548,1.,0.707106781186548,1.,0.707106781186548,1.,0.707106781186548,
1.),(1.,0.707106781186548,1.,0.707106781186548,1.,0.707106781186548,1.,
0.707106781186548,1.),(1.,0.707106781186548,1.,0.707106781186548,1.,0.707106781186548,
1.,0.707106781186548,1.),(1.,0.707106781186548,1.,0.707106781186548,1.,
0.707106781186548,1.,0.707106781186548,1.),(1.,0.707106781186548,1.,0.707106781186548,
1.,0.707106781186548,1.,0.707106781186548,1.),(1.,0.707106781186548,1.,
0.707106781186548,1.,0.707106781186548,1.,0.707106781186548,1.),(1.,0.707106781186548,
1.,0.707106781186548,1.,0.707106781186548,1.,0.707106781186548,1.),(1.,
0.707106781186548,1.,0.707106781186548,1.,0.707106781186548,1.,0.707106781186548,
1.),(1.,0.707106781186548,1.,0.707106781186548,1.,0.707106781186548,1.,
0.707106781186548,1.),(1.,0.707106781186548,1.,0.707106781186548,1.,0.707106781186548,
1.,0.707106781186548,1.),(1.,0.707106781186548,1.,0.707106781186548,1.,
0.707106781186548,1.,0.707106781186548,1.),(1.,0.707106781186548,1.,0.707106781186548,
1.,0.707106781186548,1.,0.707106781186548,1.)))
REPRESENTATION_ITEM('')
SURFACE()
);
#1066=(
BOUNDED_SURFACE()
B_SPLINE_SURFACE(5,2,((#35519,#35520,#35521,#35522,#35523,#35524,#35525,
#35526,#35527,#35528,#35529),(#35530,#35531,#35532,#35533,#35534,#35535,
#35536,#35537,#35538,#35539,#35540),(#35541,#35542,#35543,#35544,#35545,
#35546,#35547,#35548,#35549,#35550,#35551),(#35552,#35553,#35554,#35555,
#35556,#35557,#35558,#35559,#35560,#35561,#35562),(#35563,#35564,#35565,
#35566,#35567,#35568,#35569,#35570,#35571,#35572,#35573),(#35574,#35575,
#35576,#35577,#35578,#35579,#35580,#35581,#35582,#35583,#35584),(#35585,
#35586,#35587,#35588,#35589,#35590,#35591,#35592,#35593,#35594,#35595),
(#35596,#35597,#35598,#35599,#35600,#35601,#35602,#35603,#35604,#35605,
#35606),(#35607,#35608,#35609,#35610,#35611,#35612,#35613,#35614,#35615,
#35616,#35617),(#35618,#35619,#35620,#35621,#35622,#35623,#35624,#35625,
#35626,#35627,#35628),(#35629,#35630,#35631,#35632,#35633,#35634,#35635,
#35636,#35637,#35638,#35639),(#35640,#35641,#35642,#35643,#35644,#35645,
#35646,#35647,#35648,#35649,#35650),(#35651,#35652,#35653,#35654,#35655,
#35656,#35657,#35658,#35659,#35660,#35661),(#35662,#35663,#35664,#35665,
#35666,#35667,#35668,#35669,#35670,#35671,#35672),(#35673,#35674,#35675,
#35676,#35677,#35678,#35679,#35680,#35681,#35682,#35683),(#35684,#35685,
#35686,#35687,#35688,#35689,#35690,#35691,#35692,#35693,#35694),(#35695,
#35696,#35697,#35698,#35699,#35700,#35701,#35702,#35703,#35704,#35705),
(#35706,#35707,#35708,#35709,#35710,#35711,#35712,#35713,#35714,#35715,
#35716),(#35717,#35718,#35719,#35720,#35721,#35722,#35723,#35724,#35725,
#35726,#35727),(#35728,#35729,#35730,#35731,#35732,#35733,#35734,#35735,
#35736,#35737,#35738),(#35739,#35740,#35741,#35742,#35743,#35744,#35745,
#35746,#35747,#35748,#35749),(#35750,#35751,#35752,#35753,#35754,#35755,
#35756,#35757,#35758,#35759,#35760),(#35761,#35762,#35763,#35764,#35765,
#35766,#35767,#35768,#35769,#35770,#35771),(#35772,#35773,#35774,#35775,
#35776,#35777,#35778,#35779,#35780,#35781,#35782),(#35783,#35784,#35785,
#35786,#35787,#35788,#35789,#35790,#35791,#35792,#35793)),.UNSPECIFIED.,
 .F.,.T.,.F.)
B_SPLINE_SURFACE_WITH_KNOTS((6,1,1,1,1,1,1,1,1,1,1,1,1,1,1,1,1,1,1,1,6),
(3,2,2,2,2,3),(-1.,-0.95,-0.9,-0.85,-0.8,-0.75,-0.7,-0.65,-0.6,-0.55,-0.5,
-0.45,-0.4,-0.35,-0.3,-0.25,-0.2,-0.15,-0.1,-0.05,0.),(-0.0491117278067552,
0.,1.5707963267949,3.14159265358979,4.71238898038469,6.23407357937283),
 .UNSPECIFIED.)
GEOMETRIC_REPRESENTATION_ITEM()
RATIONAL_B_SPLINE_SURFACE(((0.982257720483865,0.990842547952629,1.,0.707106781186548,
1.,0.707106781186548,1.,0.707106781186548,1.,0.716264233233919,0.982257720483865),
(0.982257720483865,0.990842547952629,1.,0.707106781186548,1.,0.707106781186548,
1.,0.707106781186548,1.,0.716264233233919,0.982257720483865),(0.982257720483865,
0.990842547952629,1.,0.707106781186548,1.,0.707106781186548,1.,0.707106781186548,
1.,0.716264233233919,0.982257720483865),(0.982257720483865,0.990842547952629,
1.,0.707106781186548,1.,0.707106781186548,1.,0.707106781186548,1.,0.716264233233919,
0.982257720483865),(0.982257720483865,0.990842547952629,1.,0.707106781186548,
1.,0.707106781186548,1.,0.707106781186548,1.,0.716264233233919,0.982257720483865),
(0.982257720483865,0.990842547952629,1.,0.707106781186548,1.,0.707106781186548,
1.,0.707106781186548,1.,0.716264233233919,0.982257720483865),(0.982257720483865,
0.990842547952629,1.,0.707106781186548,1.,0.707106781186548,1.,0.707106781186548,
1.,0.716264233233919,0.982257720483865),(0.982257720483865,0.990842547952629,
1.,0.707106781186548,1.,0.707106781186548,1.,0.707106781186548,1.,0.716264233233919,
0.982257720483865),(0.982257720483865,0.990842547952629,1.,0.707106781186548,
1.,0.707106781186548,1.,0.707106781186548,1.,0.716264233233919,0.982257720483865),
(0.982257720483865,0.990842547952629,1.,0.707106781186548,1.,0.707106781186548,
1.,0.707106781186548,1.,0.716264233233919,0.982257720483865),(0.982257720483865,
0.990842547952629,1.,0.707106781186548,1.,0.707106781186548,1.,0.707106781186548,
1.,0.716264233233919,0.982257720483865),(0.982257720483865,0.990842547952629,
1.,0.707106781186548,1.,0.707106781186548,1.,0.707106781186548,1.,0.716264233233919,
0.982257720483865),(0.982257720483865,0.990842547952629,1.,0.707106781186548,
1.,0.707106781186548,1.,0.707106781186548,1.,0.716264233233919,0.982257720483865),
(0.982257720483865,0.990842547952629,1.,0.707106781186548,1.,0.707106781186548,
1.,0.707106781186548,1.,0.716264233233919,0.982257720483865),(0.982257720483865,
0.990842547952629,1.,0.707106781186548,1.,0.707106781186548,1.,0.707106781186548,
1.,0.716264233233919,0.982257720483865),(0.982257720483865,0.990842547952629,
1.,0.707106781186548,1.,0.707106781186548,1.,0.707106781186548,1.,0.716264233233919,
0.982257720483865),(0.982257720483865,0.990842547952629,1.,0.707106781186548,
1.,0.707106781186548,1.,0.707106781186548,1.,0.716264233233919,0.982257720483865),
(0.982257720483865,0.990842547952629,1.,0.707106781186548,1.,0.707106781186548,
1.,0.707106781186548,1.,0.716264233233919,0.982257720483865),(0.982257720483865,
0.990842547952629,1.,0.707106781186548,1.,0.707106781186548,1.,0.707106781186548,
1.,0.716264233233919,0.982257720483865),(0.982257720483865,0.990842547952629,
1.,0.707106781186548,1.,0.707106781186548,1.,0.707106781186548,1.,0.716264233233919,
0.982257720483865),(0.982257720483865,0.990842547952629,1.,0.707106781186548,
1.,0.707106781186548,1.,0.707106781186548,1.,0.716264233233919,0.982257720483865),
(0.982257720483865,0.990842547952629,1.,0.707106781186548,1.,0.707106781186548,
1.,0.707106781186548,1.,0.716264233233919,0.982257720483865),(0.982257720483865,
0.990842547952629,1.,0.707106781186548,1.,0.707106781186548,1.,0.707106781186548,
1.,0.716264233233919,0.982257720483865),(0.982257720483865,0.990842547952629,
1.,0.707106781186548,1.,0.707106781186548,1.,0.707106781186548,1.,0.716264233233919,
0.982257720483865),(0.982257720483865,0.990842547952629,1.,0.707106781186548,
1.,0.707106781186548,1.,0.707106781186548,1.,0.716264233233919,0.982257720483865)))
REPRESENTATION_ITEM('')
SURFACE()
);
#1067=(
BOUNDED_SURFACE()
B_SPLINE_SURFACE(5,2,((#36028,#36029,#36030,#36031,#36032,#36033,#36034,
#36035,#36036,#36037,#36038),(#36039,#36040,#36041,#36042,#36043,#36044,
#36045,#36046,#36047,#36048,#36049),(#36050,#36051,#36052,#36053,#36054,
#36055,#36056,#36057,#36058,#36059,#36060),(#36061,#36062,#36063,#36064,
#36065,#36066,#36067,#36068,#36069,#36070,#36071),(#36072,#36073,#36074,
#36075,#36076,#36077,#36078,#36079,#36080,#36081,#36082),(#36083,#36084,
#36085,#36086,#36087,#36088,#36089,#36090,#36091,#36092,#36093),(#36094,
#36095,#36096,#36097,#36098,#36099,#36100,#36101,#36102,#36103,#36104),
(#36105,#36106,#36107,#36108,#36109,#36110,#36111,#36112,#36113,#36114,
#36115),(#36116,#36117,#36118,#36119,#36120,#36121,#36122,#36123,#36124,
#36125,#36126),(#36127,#36128,#36129,#36130,#36131,#36132,#36133,#36134,
#36135,#36136,#36137),(#36138,#36139,#36140,#36141,#36142,#36143,#36144,
#36145,#36146,#36147,#36148),(#36149,#36150,#36151,#36152,#36153,#36154,
#36155,#36156,#36157,#36158,#36159),(#36160,#36161,#36162,#36163,#36164,
#36165,#36166,#36167,#36168,#36169,#36170),(#36171,#36172,#36173,#36174,
#36175,#36176,#36177,#36178,#36179,#36180,#36181),(#36182,#36183,#36184,
#36185,#36186,#36187,#36188,#36189,#36190,#36191,#36192),(#36193,#36194,
#36195,#36196,#36197,#36198,#36199,#36200,#36201,#36202,#36203),(#36204,
#36205,#36206,#36207,#36208,#36209,#36210,#36211,#36212,#36213,#36214),
(#36215,#36216,#36217,#36218,#36219,#36220,#36221,#36222,#36223,#36224,
#36225),(#36226,#36227,#36228,#36229,#36230,#36231,#36232,#36233,#36234,
#36235,#36236),(#36237,#36238,#36239,#36240,#36241,#36242,#36243,#36244,
#36245,#36246,#36247),(#36248,#36249,#36250,#36251,#36252,#36253,#36254,
#36255,#36256,#36257,#36258),(#36259,#36260,#36261,#36262,#36263,#36264,
#36265,#36266,#36267,#36268,#36269),(#36270,#36271,#36272,#36273,#36274,
#36275,#36276,#36277,#36278,#36279,#36280),(#36281,#36282,#36283,#36284,
#36285,#36286,#36287,#36288,#36289,#36290,#36291),(#36292,#36293,#36294,
#36295,#36296,#36297,#36298,#36299,#36300,#36301,#36302)),.UNSPECIFIED.,
 .F.,.T.,.F.)
B_SPLINE_SURFACE_WITH_KNOTS((6,1,1,1,1,1,1,1,1,1,1,1,1,1,1,1,1,1,1,1,6),
(3,2,2,2,2,3),(-1.,-0.95,-0.9,-0.85,-0.8,-0.75,-0.7,-0.65,-0.6,-0.55,-0.5,
-0.45,-0.4,-0.35,-0.3,-0.25,-0.2,-0.15,-0.1,-0.05,0.),(-0.0491117278067552,
0.,1.5707963267949,3.14159265358979,4.71238898038469,6.23407357937283),
 .UNSPECIFIED.)
GEOMETRIC_REPRESENTATION_ITEM()
RATIONAL_B_SPLINE_SURFACE(((0.982257720483865,0.990842547952629,1.,0.707106781186548,
1.,0.707106781186548,1.,0.707106781186548,1.,0.716264233233919,0.982257720483865),
(0.982257720483865,0.990842547952629,1.,0.707106781186548,1.,0.707106781186548,
1.,0.707106781186548,1.,0.716264233233919,0.982257720483865),(0.982257720483865,
0.990842547952629,1.,0.707106781186548,1.,0.707106781186548,1.,0.707106781186548,
1.,0.716264233233919,0.982257720483865),(0.982257720483865,0.990842547952629,
1.,0.707106781186548,1.,0.707106781186548,1.,0.707106781186548,1.,0.716264233233919,
0.982257720483865),(0.982257720483865,0.990842547952629,1.,0.707106781186548,
1.,0.707106781186548,1.,0.707106781186548,1.,0.716264233233919,0.982257720483865),
(0.982257720483865,0.990842547952629,1.,0.707106781186548,1.,0.707106781186548,
1.,0.707106781186548,1.,0.716264233233919,0.982257720483865),(0.982257720483865,
0.990842547952629,1.,0.707106781186548,1.,0.707106781186548,1.,0.707106781186548,
1.,0.716264233233919,0.982257720483865),(0.982257720483865,0.990842547952629,
1.,0.707106781186548,1.,0.707106781186548,1.,0.707106781186548,1.,0.716264233233919,
0.982257720483865),(0.982257720483865,0.990842547952629,1.,0.707106781186548,
1.,0.707106781186548,1.,0.707106781186548,1.,0.716264233233919,0.982257720483865),
(0.982257720483865,0.990842547952629,1.,0.707106781186548,1.,0.707106781186548,
1.,0.707106781186548,1.,0.716264233233919,0.982257720483865),(0.982257720483865,
0.990842547952629,1.,0.707106781186548,1.,0.707106781186548,1.,0.707106781186548,
1.,0.716264233233919,0.982257720483865),(0.982257720483865,0.990842547952629,
1.,0.707106781186548,1.,0.707106781186548,1.,0.707106781186548,1.,0.716264233233919,
0.982257720483865),(0.982257720483865,0.990842547952629,1.,0.707106781186548,
1.,0.707106781186548,1.,0.707106781186548,1.,0.716264233233919,0.982257720483865),
(0.982257720483865,0.990842547952629,1.,0.707106781186548,1.,0.707106781186548,
1.,0.707106781186548,1.,0.716264233233919,0.982257720483865),(0.982257720483865,
0.990842547952629,1.,0.707106781186548,1.,0.707106781186548,1.,0.707106781186548,
1.,0.716264233233919,0.982257720483865),(0.982257720483865,0.990842547952629,
1.,0.707106781186548,1.,0.707106781186548,1.,0.707106781186548,1.,0.716264233233919,
0.982257720483865),(0.982257720483865,0.990842547952629,1.,0.707106781186548,
1.,0.707106781186548,1.,0.707106781186548,1.,0.716264233233919,0.982257720483865),
(0.982257720483865,0.990842547952629,1.,0.707106781186548,1.,0.707106781186548,
1.,0.707106781186548,1.,0.716264233233919,0.982257720483865),(0.982257720483865,
0.990842547952629,1.,0.707106781186548,1.,0.707106781186548,1.,0.707106781186548,
1.,0.716264233233919,0.982257720483865),(0.982257720483865,0.990842547952629,
1.,0.707106781186548,1.,0.707106781186548,1.,0.707106781186548,1.,0.716264233233919,
0.982257720483865),(0.982257720483865,0.990842547952629,1.,0.707106781186548,
1.,0.707106781186548,1.,0.707106781186548,1.,0.716264233233919,0.982257720483865),
(0.982257720483865,0.990842547952629,1.,0.707106781186548,1.,0.707106781186548,
1.,0.707106781186548,1.,0.716264233233919,0.982257720483865),(0.982257720483865,
0.990842547952629,1.,0.707106781186548,1.,0.707106781186548,1.,0.707106781186548,
1.,0.716264233233919,0.982257720483865),(0.982257720483865,0.990842547952629,
1.,0.707106781186548,1.,0.707106781186548,1.,0.707106781186548,1.,0.716264233233919,
0.982257720483865),(0.982257720483865,0.990842547952629,1.,0.707106781186548,
1.,0.707106781186548,1.,0.707106781186548,1.,0.716264233233919,0.982257720483865)))
REPRESENTATION_ITEM('')
SURFACE()
);
#1068=(
BOUNDED_SURFACE()
B_SPLINE_SURFACE(5,2,((#36547,#36548,#36549,#36550,#36551,#36552,#36553,
#36554,#36555,#36556,#36557),(#36558,#36559,#36560,#36561,#36562,#36563,
#36564,#36565,#36566,#36567,#36568),(#36569,#36570,#36571,#36572,#36573,
#36574,#36575,#36576,#36577,#36578,#36579),(#36580,#36581,#36582,#36583,
#36584,#36585,#36586,#36587,#36588,#36589,#36590),(#36591,#36592,#36593,
#36594,#36595,#36596,#36597,#36598,#36599,#36600,#36601),(#36602,#36603,
#36604,#36605,#36606,#36607,#36608,#36609,#36610,#36611,#36612),(#36613,
#36614,#36615,#36616,#36617,#36618,#36619,#36620,#36621,#36622,#36623),
(#36624,#36625,#36626,#36627,#36628,#36629,#36630,#36631,#36632,#36633,
#36634),(#36635,#36636,#36637,#36638,#36639,#36640,#36641,#36642,#36643,
#36644,#36645),(#36646,#36647,#36648,#36649,#36650,#36651,#36652,#36653,
#36654,#36655,#36656),(#36657,#36658,#36659,#36660,#36661,#36662,#36663,
#36664,#36665,#36666,#36667),(#36668,#36669,#36670,#36671,#36672,#36673,
#36674,#36675,#36676,#36677,#36678),(#36679,#36680,#36681,#36682,#36683,
#36684,#36685,#36686,#36687,#36688,#36689),(#36690,#36691,#36692,#36693,
#36694,#36695,#36696,#36697,#36698,#36699,#36700),(#36701,#36702,#36703,
#36704,#36705,#36706,#36707,#36708,#36709,#36710,#36711),(#36712,#36713,
#36714,#36715,#36716,#36717,#36718,#36719,#36720,#36721,#36722),(#36723,
#36724,#36725,#36726,#36727,#36728,#36729,#36730,#36731,#36732,#36733),
(#36734,#36735,#36736,#36737,#36738,#36739,#36740,#36741,#36742,#36743,
#36744),(#36745,#36746,#36747,#36748,#36749,#36750,#36751,#36752,#36753,
#36754,#36755),(#36756,#36757,#36758,#36759,#36760,#36761,#36762,#36763,
#36764,#36765,#36766),(#36767,#36768,#36769,#36770,#36771,#36772,#36773,
#36774,#36775,#36776,#36777),(#36778,#36779,#36780,#36781,#36782,#36783,
#36784,#36785,#36786,#36787,#36788),(#36789,#36790,#36791,#36792,#36793,
#36794,#36795,#36796,#36797,#36798,#36799),(#36800,#36801,#36802,#36803,
#36804,#36805,#36806,#36807,#36808,#36809,#36810),(#36811,#36812,#36813,
#36814,#36815,#36816,#36817,#36818,#36819,#36820,#36821)),.UNSPECIFIED.,
 .F.,.T.,.F.)
B_SPLINE_SURFACE_WITH_KNOTS((6,1,1,1,1,1,1,1,1,1,1,1,1,1,1,1,1,1,1,1,6),
(3,2,2,2,2,3),(-1.,-0.95,-0.9,-0.85,-0.8,-0.75,-0.7,-0.65,-0.6,-0.55,-0.5,
-0.45,-0.4,-0.35,-0.3,-0.25,-0.2,-0.15,-0.1,-0.05,0.),(-0.0491117278067552,
0.,1.5707963267949,3.14159265358979,4.71238898038469,6.23407357937283),
 .UNSPECIFIED.)
GEOMETRIC_REPRESENTATION_ITEM()
RATIONAL_B_SPLINE_SURFACE(((0.982257720483865,0.990842547952629,1.,0.707106781186548,
1.,0.707106781186548,1.,0.707106781186548,1.,0.716264233233919,0.982257720483865),
(0.982257720483865,0.990842547952629,1.,0.707106781186548,1.,0.707106781186548,
1.,0.707106781186548,1.,0.716264233233919,0.982257720483865),(0.982257720483865,
0.990842547952629,1.,0.707106781186548,1.,0.707106781186548,1.,0.707106781186548,
1.,0.716264233233919,0.982257720483865),(0.982257720483865,0.990842547952629,
1.,0.707106781186548,1.,0.707106781186548,1.,0.707106781186548,1.,0.716264233233919,
0.982257720483865),(0.982257720483865,0.990842547952629,1.,0.707106781186548,
1.,0.707106781186548,1.,0.707106781186548,1.,0.716264233233919,0.982257720483865),
(0.982257720483865,0.990842547952629,1.,0.707106781186548,1.,0.707106781186548,
1.,0.707106781186548,1.,0.716264233233919,0.982257720483865),(0.982257720483865,
0.990842547952629,1.,0.707106781186548,1.,0.707106781186548,1.,0.707106781186548,
1.,0.716264233233919,0.982257720483865),(0.982257720483865,0.990842547952629,
1.,0.707106781186548,1.,0.707106781186548,1.,0.707106781186548,1.,0.716264233233919,
0.982257720483865),(0.982257720483865,0.990842547952629,1.,0.707106781186548,
1.,0.707106781186548,1.,0.707106781186548,1.,0.716264233233919,0.982257720483865),
(0.982257720483865,0.990842547952629,1.,0.707106781186548,1.,0.707106781186548,
1.,0.707106781186548,1.,0.716264233233919,0.982257720483865),(0.982257720483865,
0.990842547952629,1.,0.707106781186548,1.,0.707106781186548,1.,0.707106781186548,
1.,0.716264233233919,0.982257720483865),(0.982257720483865,0.990842547952629,
1.,0.707106781186548,1.,0.707106781186548,1.,0.707106781186548,1.,0.716264233233919,
0.982257720483865),(0.982257720483865,0.990842547952629,1.,0.707106781186548,
1.,0.707106781186548,1.,0.707106781186548,1.,0.716264233233919,0.982257720483865),
(0.982257720483865,0.990842547952629,1.,0.707106781186548,1.,0.707106781186548,
1.,0.707106781186548,1.,0.716264233233919,0.982257720483865),(0.982257720483865,
0.990842547952629,1.,0.707106781186548,1.,0.707106781186548,1.,0.707106781186548,
1.,0.716264233233919,0.982257720483865),(0.982257720483865,0.990842547952629,
1.,0.707106781186548,1.,0.707106781186548,1.,0.707106781186548,1.,0.716264233233919,
0.982257720483865),(0.982257720483865,0.990842547952629,1.,0.707106781186548,
1.,0.707106781186548,1.,0.707106781186548,1.,0.716264233233919,0.982257720483865),
(0.982257720483865,0.990842547952629,1.,0.707106781186548,1.,0.707106781186548,
1.,0.707106781186548,1.,0.716264233233919,0.982257720483865),(0.982257720483865,
0.990842547952629,1.,0.707106781186548,1.,0.707106781186548,1.,0.707106781186548,
1.,0.716264233233919,0.982257720483865),(0.982257720483865,0.990842547952629,
1.,0.707106781186548,1.,0.707106781186548,1.,0.707106781186548,1.,0.716264233233919,
0.982257720483865),(0.982257720483865,0.990842547952629,1.,0.707106781186548,
1.,0.707106781186548,1.,0.707106781186548,1.,0.716264233233919,0.982257720483865),
(0.982257720483865,0.990842547952629,1.,0.707106781186548,1.,0.707106781186548,
1.,0.707106781186548,1.,0.716264233233919,0.982257720483865),(0.982257720483865,
0.990842547952629,1.,0.707106781186548,1.,0.707106781186548,1.,0.707106781186548,
1.,0.716264233233919,0.982257720483865),(0.982257720483865,0.990842547952629,
1.,0.707106781186548,1.,0.707106781186548,1.,0.707106781186548,1.,0.716264233233919,
0.982257720483865),(0.982257720483865,0.990842547952629,1.,0.707106781186548,
1.,0.707106781186548,1.,0.707106781186548,1.,0.716264233233919,0.982257720483865)))
REPRESENTATION_ITEM('')
SURFACE()
);
#1069=(
BOUNDED_SURFACE()
B_SPLINE_SURFACE(5,2,((#37046,#37047,#37048,#37049,#37050,#37051,#37052,
#37053,#37054,#37055,#37056),(#37057,#37058,#37059,#37060,#37061,#37062,
#37063,#37064,#37065,#37066,#37067),(#37068,#37069,#37070,#37071,#37072,
#37073,#37074,#37075,#37076,#37077,#37078),(#37079,#37080,#37081,#37082,
#37083,#37084,#37085,#37086,#37087,#37088,#37089),(#37090,#37091,#37092,
#37093,#37094,#37095,#37096,#37097,#37098,#37099,#37100),(#37101,#37102,
#37103,#37104,#37105,#37106,#37107,#37108,#37109,#37110,#37111),(#37112,
#37113,#37114,#37115,#37116,#37117,#37118,#37119,#37120,#37121,#37122),
(#37123,#37124,#37125,#37126,#37127,#37128,#37129,#37130,#37131,#37132,
#37133),(#37134,#37135,#37136,#37137,#37138,#37139,#37140,#37141,#37142,
#37143,#37144),(#37145,#37146,#37147,#37148,#37149,#37150,#37151,#37152,
#37153,#37154,#37155),(#37156,#37157,#37158,#37159,#37160,#37161,#37162,
#37163,#37164,#37165,#37166),(#37167,#37168,#37169,#37170,#37171,#37172,
#37173,#37174,#37175,#37176,#37177),(#37178,#37179,#37180,#37181,#37182,
#37183,#37184,#37185,#37186,#37187,#37188),(#37189,#37190,#37191,#37192,
#37193,#37194,#37195,#37196,#37197,#37198,#37199),(#37200,#37201,#37202,
#37203,#37204,#37205,#37206,#37207,#37208,#37209,#37210),(#37211,#37212,
#37213,#37214,#37215,#37216,#37217,#37218,#37219,#37220,#37221),(#37222,
#37223,#37224,#37225,#37226,#37227,#37228,#37229,#37230,#37231,#37232),
(#37233,#37234,#37235,#37236,#37237,#37238,#37239,#37240,#37241,#37242,
#37243),(#37244,#37245,#37246,#37247,#37248,#37249,#37250,#37251,#37252,
#37253,#37254),(#37255,#37256,#37257,#37258,#37259,#37260,#37261,#37262,
#37263,#37264,#37265),(#37266,#37267,#37268,#37269,#37270,#37271,#37272,
#37273,#37274,#37275,#37276),(#37277,#37278,#37279,#37280,#37281,#37282,
#37283,#37284,#37285,#37286,#37287),(#37288,#37289,#37290,#37291,#37292,
#37293,#37294,#37295,#37296,#37297,#37298),(#37299,#37300,#37301,#37302,
#37303,#37304,#37305,#37306,#37307,#37308,#37309),(#37310,#37311,#37312,
#37313,#37314,#37315,#37316,#37317,#37318,#37319,#37320)),.UNSPECIFIED.,
 .F.,.T.,.F.)
B_SPLINE_SURFACE_WITH_KNOTS((6,1,1,1,1,1,1,1,1,1,1,1,1,1,1,1,1,1,1,1,6),
(3,2,2,2,2,3),(-1.,-0.95,-0.9,-0.85,-0.8,-0.75,-0.7,-0.65,-0.6,-0.55,-0.5,
-0.45,-0.4,-0.35,-0.3,-0.25,-0.2,-0.15,-0.1,-0.05,0.),(-0.0491117278067552,
0.,1.5707963267949,3.14159265358979,4.71238898038469,6.23407357937283),
 .UNSPECIFIED.)
GEOMETRIC_REPRESENTATION_ITEM()
RATIONAL_B_SPLINE_SURFACE(((0.982257720483865,0.990842547952629,1.,0.707106781186548,
1.,0.707106781186548,1.,0.707106781186548,1.,0.716264233233919,0.982257720483865),
(0.982257720483865,0.990842547952629,1.,0.707106781186548,1.,0.707106781186548,
1.,0.707106781186548,1.,0.716264233233919,0.982257720483865),(0.982257720483865,
0.990842547952629,1.,0.707106781186548,1.,0.707106781186548,1.,0.707106781186548,
1.,0.716264233233919,0.982257720483865),(0.982257720483865,0.990842547952629,
1.,0.707106781186548,1.,0.707106781186548,1.,0.707106781186548,1.,0.716264233233919,
0.982257720483865),(0.982257720483865,0.990842547952629,1.,0.707106781186548,
1.,0.707106781186548,1.,0.707106781186548,1.,0.716264233233919,0.982257720483865),
(0.982257720483865,0.990842547952629,1.,0.707106781186548,1.,0.707106781186548,
1.,0.707106781186548,1.,0.716264233233919,0.982257720483865),(0.982257720483865,
0.990842547952629,1.,0.707106781186548,1.,0.707106781186548,1.,0.707106781186548,
1.,0.716264233233919,0.982257720483865),(0.982257720483865,0.990842547952629,
1.,0.707106781186548,1.,0.707106781186548,1.,0.707106781186548,1.,0.716264233233919,
0.982257720483865),(0.982257720483865,0.990842547952629,1.,0.707106781186548,
1.,0.707106781186548,1.,0.707106781186548,1.,0.716264233233919,0.982257720483865),
(0.982257720483865,0.990842547952629,1.,0.707106781186548,1.,0.707106781186548,
1.,0.707106781186548,1.,0.716264233233919,0.982257720483865),(0.982257720483865,
0.990842547952629,1.,0.707106781186548,1.,0.707106781186548,1.,0.707106781186548,
1.,0.716264233233919,0.982257720483865),(0.982257720483865,0.990842547952629,
1.,0.707106781186548,1.,0.707106781186548,1.,0.707106781186548,1.,0.716264233233919,
0.982257720483865),(0.982257720483865,0.990842547952629,1.,0.707106781186548,
1.,0.707106781186548,1.,0.707106781186548,1.,0.716264233233919,0.982257720483865),
(0.982257720483865,0.990842547952629,1.,0.707106781186548,1.,0.707106781186548,
1.,0.707106781186548,1.,0.716264233233919,0.982257720483865),(0.982257720483865,
0.990842547952629,1.,0.707106781186548,1.,0.707106781186548,1.,0.707106781186548,
1.,0.716264233233919,0.982257720483865),(0.982257720483865,0.990842547952629,
1.,0.707106781186548,1.,0.707106781186548,1.,0.707106781186548,1.,0.716264233233919,
0.982257720483865),(0.982257720483865,0.990842547952629,1.,0.707106781186548,
1.,0.707106781186548,1.,0.707106781186548,1.,0.716264233233919,0.982257720483865),
(0.982257720483865,0.990842547952629,1.,0.707106781186548,1.,0.707106781186548,
1.,0.707106781186548,1.,0.716264233233919,0.982257720483865),(0.982257720483865,
0.990842547952629,1.,0.707106781186548,1.,0.707106781186548,1.,0.707106781186548,
1.,0.716264233233919,0.982257720483865),(0.982257720483865,0.990842547952629,
1.,0.707106781186548,1.,0.707106781186548,1.,0.707106781186548,1.,0.716264233233919,
0.982257720483865),(0.982257720483865,0.990842547952629,1.,0.707106781186548,
1.,0.707106781186548,1.,0.707106781186548,1.,0.716264233233919,0.982257720483865),
(0.982257720483865,0.990842547952629,1.,0.707106781186548,1.,0.707106781186548,
1.,0.707106781186548,1.,0.716264233233919,0.982257720483865),(0.982257720483865,
0.990842547952629,1.,0.707106781186548,1.,0.707106781186548,1.,0.707106781186548,
1.,0.716264233233919,0.982257720483865),(0.982257720483865,0.990842547952629,
1.,0.707106781186548,1.,0.707106781186548,1.,0.707106781186548,1.,0.716264233233919,
0.982257720483865),(0.982257720483865,0.990842547952629,1.,0.707106781186548,
1.,0.707106781186548,1.,0.707106781186548,1.,0.716264233233919,0.982257720483865)))
REPRESENTATION_ITEM('')
SURFACE()
);
#1070=(
BOUNDED_SURFACE()
B_SPLINE_SURFACE(5,2,((#37555,#37556,#37557,#37558,#37559,#37560,#37561,
#37562,#37563,#37564,#37565),(#37566,#37567,#37568,#37569,#37570,#37571,
#37572,#37573,#37574,#37575,#37576),(#37577,#37578,#37579,#37580,#37581,
#37582,#37583,#37584,#37585,#37586,#37587),(#37588,#37589,#37590,#37591,
#37592,#37593,#37594,#37595,#37596,#37597,#37598),(#37599,#37600,#37601,
#37602,#37603,#37604,#37605,#37606,#37607,#37608,#37609),(#37610,#37611,
#37612,#37613,#37614,#37615,#37616,#37617,#37618,#37619,#37620),(#37621,
#37622,#37623,#37624,#37625,#37626,#37627,#37628,#37629,#37630,#37631),
(#37632,#37633,#37634,#37635,#37636,#37637,#37638,#37639,#37640,#37641,
#37642),(#37643,#37644,#37645,#37646,#37647,#37648,#37649,#37650,#37651,
#37652,#37653),(#37654,#37655,#37656,#37657,#37658,#37659,#37660,#37661,
#37662,#37663,#37664),(#37665,#37666,#37667,#37668,#37669,#37670,#37671,
#37672,#37673,#37674,#37675),(#37676,#37677,#37678,#37679,#37680,#37681,
#37682,#37683,#37684,#37685,#37686),(#37687,#37688,#37689,#37690,#37691,
#37692,#37693,#37694,#37695,#37696,#37697),(#37698,#37699,#37700,#37701,
#37702,#37703,#37704,#37705,#37706,#37707,#37708),(#37709,#37710,#37711,
#37712,#37713,#37714,#37715,#37716,#37717,#37718,#37719),(#37720,#37721,
#37722,#37723,#37724,#37725,#37726,#37727,#37728,#37729,#37730),(#37731,
#37732,#37733,#37734,#37735,#37736,#37737,#37738,#37739,#37740,#37741),
(#37742,#37743,#37744,#37745,#37746,#37747,#37748,#37749,#37750,#37751,
#37752),(#37753,#37754,#37755,#37756,#37757,#37758,#37759,#37760,#37761,
#37762,#37763),(#37764,#37765,#37766,#37767,#37768,#37769,#37770,#37771,
#37772,#37773,#37774),(#37775,#37776,#37777,#37778,#37779,#37780,#37781,
#37782,#37783,#37784,#37785),(#37786,#37787,#37788,#37789,#37790,#37791,
#37792,#37793,#37794,#37795,#37796),(#37797,#37798,#37799,#37800,#37801,
#37802,#37803,#37804,#37805,#37806,#37807),(#37808,#37809,#37810,#37811,
#37812,#37813,#37814,#37815,#37816,#37817,#37818),(#37819,#37820,#37821,
#37822,#37823,#37824,#37825,#37826,#37827,#37828,#37829)),.UNSPECIFIED.,
 .F.,.T.,.F.)
B_SPLINE_SURFACE_WITH_KNOTS((6,1,1,1,1,1,1,1,1,1,1,1,1,1,1,1,1,1,1,1,6),
(3,2,2,2,2,3),(-1.,-0.95,-0.9,-0.85,-0.8,-0.75,-0.7,-0.65,-0.6,-0.55,-0.5,
-0.45,-0.4,-0.35,-0.3,-0.25,-0.2,-0.15,-0.1,-0.05,0.),(-0.0491117278067552,
0.,1.5707963267949,3.14159265358979,4.71238898038469,6.23407357937283),
 .UNSPECIFIED.)
GEOMETRIC_REPRESENTATION_ITEM()
RATIONAL_B_SPLINE_SURFACE(((0.982257720483865,0.990842547952629,1.,0.707106781186548,
1.,0.707106781186548,1.,0.707106781186548,1.,0.716264233233919,0.982257720483865),
(0.982257720483865,0.990842547952629,1.,0.707106781186548,1.,0.707106781186548,
1.,0.707106781186548,1.,0.716264233233919,0.982257720483865),(0.982257720483865,
0.990842547952629,1.,0.707106781186548,1.,0.707106781186548,1.,0.707106781186548,
1.,0.716264233233919,0.982257720483865),(0.982257720483865,0.990842547952629,
1.,0.707106781186548,1.,0.707106781186548,1.,0.707106781186548,1.,0.716264233233919,
0.982257720483865),(0.982257720483865,0.990842547952629,1.,0.707106781186548,
1.,0.707106781186548,1.,0.707106781186548,1.,0.716264233233919,0.982257720483865),
(0.982257720483865,0.990842547952629,1.,0.707106781186548,1.,0.707106781186548,
1.,0.707106781186548,1.,0.716264233233919,0.982257720483865),(0.982257720483865,
0.990842547952629,1.,0.707106781186548,1.,0.707106781186548,1.,0.707106781186548,
1.,0.716264233233919,0.982257720483865),(0.982257720483865,0.990842547952629,
1.,0.707106781186548,1.,0.707106781186548,1.,0.707106781186548,1.,0.716264233233919,
0.982257720483865),(0.982257720483865,0.990842547952629,1.,0.707106781186548,
1.,0.707106781186548,1.,0.707106781186548,1.,0.716264233233919,0.982257720483865),
(0.982257720483865,0.990842547952629,1.,0.707106781186548,1.,0.707106781186548,
1.,0.707106781186548,1.,0.716264233233919,0.982257720483865),(0.982257720483865,
0.990842547952629,1.,0.707106781186548,1.,0.707106781186548,1.,0.707106781186548,
1.,0.716264233233919,0.982257720483865),(0.982257720483865,0.990842547952629,
1.,0.707106781186548,1.,0.707106781186548,1.,0.707106781186548,1.,0.716264233233919,
0.982257720483865),(0.982257720483865,0.990842547952629,1.,0.707106781186548,
1.,0.707106781186548,1.,0.707106781186548,1.,0.716264233233919,0.982257720483865),
(0.982257720483865,0.990842547952629,1.,0.707106781186548,1.,0.707106781186548,
1.,0.707106781186548,1.,0.716264233233919,0.982257720483865),(0.982257720483865,
0.990842547952629,1.,0.707106781186548,1.,0.707106781186548,1.,0.707106781186548,
1.,0.716264233233919,0.982257720483865),(0.982257720483865,0.990842547952629,
1.,0.707106781186548,1.,0.707106781186548,1.,0.707106781186548,1.,0.716264233233919,
0.982257720483865),(0.982257720483865,0.990842547952629,1.,0.707106781186548,
1.,0.707106781186548,1.,0.707106781186548,1.,0.716264233233919,0.982257720483865),
(0.982257720483865,0.990842547952629,1.,0.707106781186548,1.,0.707106781186548,
1.,0.707106781186548,1.,0.716264233233919,0.982257720483865),(0.982257720483865,
0.990842547952629,1.,0.707106781186548,1.,0.707106781186548,1.,0.707106781186548,
1.,0.716264233233919,0.982257720483865),(0.982257720483865,0.990842547952629,
1.,0.707106781186548,1.,0.707106781186548,1.,0.707106781186548,1.,0.716264233233919,
0.982257720483865),(0.982257720483865,0.990842547952629,1.,0.707106781186548,
1.,0.707106781186548,1.,0.707106781186548,1.,0.716264233233919,0.982257720483865),
(0.982257720483865,0.990842547952629,1.,0.707106781186548,1.,0.707106781186548,
1.,0.707106781186548,1.,0.716264233233919,0.982257720483865),(0.982257720483865,
0.990842547952629,1.,0.707106781186548,1.,0.707106781186548,1.,0.707106781186548,
1.,0.716264233233919,0.982257720483865),(0.982257720483865,0.990842547952629,
1.,0.707106781186548,1.,0.707106781186548,1.,0.707106781186548,1.,0.716264233233919,
0.982257720483865),(0.982257720483865,0.990842547952629,1.,0.707106781186548,
1.,0.707106781186548,1.,0.707106781186548,1.,0.716264233233919,0.982257720483865)))
REPRESENTATION_ITEM('')
SURFACE()
);
#1071=(
BOUNDED_SURFACE()
B_SPLINE_SURFACE(5,2,((#38074,#38075,#38076,#38077,#38078,#38079,#38080,
#38081,#38082,#38083,#38084),(#38085,#38086,#38087,#38088,#38089,#38090,
#38091,#38092,#38093,#38094,#38095),(#38096,#38097,#38098,#38099,#38100,
#38101,#38102,#38103,#38104,#38105,#38106),(#38107,#38108,#38109,#38110,
#38111,#38112,#38113,#38114,#38115,#38116,#38117),(#38118,#38119,#38120,
#38121,#38122,#38123,#38124,#38125,#38126,#38127,#38128),(#38129,#38130,
#38131,#38132,#38133,#38134,#38135,#38136,#38137,#38138,#38139),(#38140,
#38141,#38142,#38143,#38144,#38145,#38146,#38147,#38148,#38149,#38150),
(#38151,#38152,#38153,#38154,#38155,#38156,#38157,#38158,#38159,#38160,
#38161),(#38162,#38163,#38164,#38165,#38166,#38167,#38168,#38169,#38170,
#38171,#38172),(#38173,#38174,#38175,#38176,#38177,#38178,#38179,#38180,
#38181,#38182,#38183),(#38184,#38185,#38186,#38187,#38188,#38189,#38190,
#38191,#38192,#38193,#38194),(#38195,#38196,#38197,#38198,#38199,#38200,
#38201,#38202,#38203,#38204,#38205),(#38206,#38207,#38208,#38209,#38210,
#38211,#38212,#38213,#38214,#38215,#38216),(#38217,#38218,#38219,#38220,
#38221,#38222,#38223,#38224,#38225,#38226,#38227),(#38228,#38229,#38230,
#38231,#38232,#38233,#38234,#38235,#38236,#38237,#38238),(#38239,#38240,
#38241,#38242,#38243,#38244,#38245,#38246,#38247,#38248,#38249),(#38250,
#38251,#38252,#38253,#38254,#38255,#38256,#38257,#38258,#38259,#38260),
(#38261,#38262,#38263,#38264,#38265,#38266,#38267,#38268,#38269,#38270,
#38271),(#38272,#38273,#38274,#38275,#38276,#38277,#38278,#38279,#38280,
#38281,#38282),(#38283,#38284,#38285,#38286,#38287,#38288,#38289,#38290,
#38291,#38292,#38293),(#38294,#38295,#38296,#38297,#38298,#38299,#38300,
#38301,#38302,#38303,#38304),(#38305,#38306,#38307,#38308,#38309,#38310,
#38311,#38312,#38313,#38314,#38315),(#38316,#38317,#38318,#38319,#38320,
#38321,#38322,#38323,#38324,#38325,#38326),(#38327,#38328,#38329,#38330,
#38331,#38332,#38333,#38334,#38335,#38336,#38337),(#38338,#38339,#38340,
#38341,#38342,#38343,#38344,#38345,#38346,#38347,#38348)),.UNSPECIFIED.,
 .F.,.T.,.F.)
B_SPLINE_SURFACE_WITH_KNOTS((6,1,1,1,1,1,1,1,1,1,1,1,1,1,1,1,1,1,1,1,6),
(3,2,2,2,2,3),(-1.,-0.95,-0.9,-0.85,-0.8,-0.75,-0.7,-0.65,-0.6,-0.55,-0.5,
-0.45,-0.4,-0.35,-0.3,-0.25,-0.2,-0.15,-0.1,-0.05,0.),(-0.0491117278067552,
0.,1.5707963267949,3.14159265358979,4.71238898038469,6.23407357937283),
 .UNSPECIFIED.)
GEOMETRIC_REPRESENTATION_ITEM()
RATIONAL_B_SPLINE_SURFACE(((0.982257720483865,0.990842547952629,1.,0.707106781186548,
1.,0.707106781186548,1.,0.707106781186548,1.,0.716264233233919,0.982257720483865),
(0.982257720483865,0.990842547952629,1.,0.707106781186548,1.,0.707106781186548,
1.,0.707106781186548,1.,0.716264233233919,0.982257720483865),(0.982257720483865,
0.990842547952629,1.,0.707106781186548,1.,0.707106781186548,1.,0.707106781186548,
1.,0.716264233233919,0.982257720483865),(0.982257720483865,0.990842547952629,
1.,0.707106781186548,1.,0.707106781186548,1.,0.707106781186548,1.,0.716264233233919,
0.982257720483865),(0.982257720483865,0.990842547952629,1.,0.707106781186548,
1.,0.707106781186548,1.,0.707106781186548,1.,0.716264233233919,0.982257720483865),
(0.982257720483865,0.990842547952629,1.,0.707106781186548,1.,0.707106781186548,
1.,0.707106781186548,1.,0.716264233233919,0.982257720483865),(0.982257720483865,
0.990842547952629,1.,0.707106781186548,1.,0.707106781186548,1.,0.707106781186548,
1.,0.716264233233919,0.982257720483865),(0.982257720483865,0.990842547952629,
1.,0.707106781186548,1.,0.707106781186548,1.,0.707106781186548,1.,0.716264233233919,
0.982257720483865),(0.982257720483865,0.990842547952629,1.,0.707106781186548,
1.,0.707106781186548,1.,0.707106781186548,1.,0.716264233233919,0.982257720483865),
(0.982257720483865,0.990842547952629,1.,0.707106781186548,1.,0.707106781186548,
1.,0.707106781186548,1.,0.716264233233919,0.982257720483865),(0.982257720483865,
0.990842547952629,1.,0.707106781186548,1.,0.707106781186548,1.,0.707106781186548,
1.,0.716264233233919,0.982257720483865),(0.982257720483865,0.990842547952629,
1.,0.707106781186548,1.,0.707106781186548,1.,0.707106781186548,1.,0.716264233233919,
0.982257720483865),(0.982257720483865,0.990842547952629,1.,0.707106781186548,
1.,0.707106781186548,1.,0.707106781186548,1.,0.716264233233919,0.982257720483865),
(0.982257720483865,0.990842547952629,1.,0.707106781186548,1.,0.707106781186548,
1.,0.707106781186548,1.,0.716264233233919,0.982257720483865),(0.982257720483865,
0.990842547952629,1.,0.707106781186548,1.,0.707106781186548,1.,0.707106781186548,
1.,0.716264233233919,0.982257720483865),(0.982257720483865,0.990842547952629,
1.,0.707106781186548,1.,0.707106781186548,1.,0.707106781186548,1.,0.716264233233919,
0.982257720483865),(0.982257720483865,0.990842547952629,1.,0.707106781186548,
1.,0.707106781186548,1.,0.707106781186548,1.,0.716264233233919,0.982257720483865),
(0.982257720483865,0.990842547952629,1.,0.707106781186548,1.,0.707106781186548,
1.,0.707106781186548,1.,0.716264233233919,0.982257720483865),(0.982257720483865,
0.990842547952629,1.,0.707106781186548,1.,0.707106781186548,1.,0.707106781186548,
1.,0.716264233233919,0.982257720483865),(0.982257720483865,0.990842547952629,
1.,0.707106781186548,1.,0.707106781186548,1.,0.707106781186548,1.,0.716264233233919,
0.982257720483865),(0.982257720483865,0.990842547952629,1.,0.707106781186548,
1.,0.707106781186548,1.,0.707106781186548,1.,0.716264233233919,0.982257720483865),
(0.982257720483865,0.990842547952629,1.,0.707106781186548,1.,0.707106781186548,
1.,0.707106781186548,1.,0.716264233233919,0.982257720483865),(0.982257720483865,
0.990842547952629,1.,0.707106781186548,1.,0.707106781186548,1.,0.707106781186548,
1.,0.716264233233919,0.982257720483865),(0.982257720483865,0.990842547952629,
1.,0.707106781186548,1.,0.707106781186548,1.,0.707106781186548,1.,0.716264233233919,
0.982257720483865),(0.982257720483865,0.990842547952629,1.,0.707106781186548,
1.,0.707106781186548,1.,0.707106781186548,1.,0.716264233233919,0.982257720483865)))
REPRESENTATION_ITEM('')
SURFACE()
);
#1072=(
BOUNDED_SURFACE()
B_SPLINE_SURFACE(5,2,((#38573,#38574,#38575,#38576,#38577,#38578,#38579,
#38580,#38581,#38582,#38583),(#38584,#38585,#38586,#38587,#38588,#38589,
#38590,#38591,#38592,#38593,#38594),(#38595,#38596,#38597,#38598,#38599,
#38600,#38601,#38602,#38603,#38604,#38605),(#38606,#38607,#38608,#38609,
#38610,#38611,#38612,#38613,#38614,#38615,#38616),(#38617,#38618,#38619,
#38620,#38621,#38622,#38623,#38624,#38625,#38626,#38627),(#38628,#38629,
#38630,#38631,#38632,#38633,#38634,#38635,#38636,#38637,#38638),(#38639,
#38640,#38641,#38642,#38643,#38644,#38645,#38646,#38647,#38648,#38649),
(#38650,#38651,#38652,#38653,#38654,#38655,#38656,#38657,#38658,#38659,
#38660),(#38661,#38662,#38663,#38664,#38665,#38666,#38667,#38668,#38669,
#38670,#38671),(#38672,#38673,#38674,#38675,#38676,#38677,#38678,#38679,
#38680,#38681,#38682),(#38683,#38684,#38685,#38686,#38687,#38688,#38689,
#38690,#38691,#38692,#38693),(#38694,#38695,#38696,#38697,#38698,#38699,
#38700,#38701,#38702,#38703,#38704),(#38705,#38706,#38707,#38708,#38709,
#38710,#38711,#38712,#38713,#38714,#38715),(#38716,#38717,#38718,#38719,
#38720,#38721,#38722,#38723,#38724,#38725,#38726),(#38727,#38728,#38729,
#38730,#38731,#38732,#38733,#38734,#38735,#38736,#38737),(#38738,#38739,
#38740,#38741,#38742,#38743,#38744,#38745,#38746,#38747,#38748),(#38749,
#38750,#38751,#38752,#38753,#38754,#38755,#38756,#38757,#38758,#38759),
(#38760,#38761,#38762,#38763,#38764,#38765,#38766,#38767,#38768,#38769,
#38770),(#38771,#38772,#38773,#38774,#38775,#38776,#38777,#38778,#38779,
#38780,#38781),(#38782,#38783,#38784,#38785,#38786,#38787,#38788,#38789,
#38790,#38791,#38792),(#38793,#38794,#38795,#38796,#38797,#38798,#38799,
#38800,#38801,#38802,#38803),(#38804,#38805,#38806,#38807,#38808,#38809,
#38810,#38811,#38812,#38813,#38814),(#38815,#38816,#38817,#38818,#38819,
#38820,#38821,#38822,#38823,#38824,#38825),(#38826,#38827,#38828,#38829,
#38830,#38831,#38832,#38833,#38834,#38835,#38836),(#38837,#38838,#38839,
#38840,#38841,#38842,#38843,#38844,#38845,#38846,#38847)),.UNSPECIFIED.,
 .F.,.T.,.F.)
B_SPLINE_SURFACE_WITH_KNOTS((6,1,1,1,1,1,1,1,1,1,1,1,1,1,1,1,1,1,1,1,6),
(3,2,2,2,2,3),(-1.,-0.95,-0.9,-0.85,-0.8,-0.75,-0.7,-0.65,-0.6,-0.55,-0.5,
-0.45,-0.4,-0.35,-0.3,-0.25,-0.2,-0.15,-0.1,-0.05,0.),(-0.0491117278067552,
0.,1.5707963267949,3.14159265358979,4.71238898038469,6.23407357937283),
 .UNSPECIFIED.)
GEOMETRIC_REPRESENTATION_ITEM()
RATIONAL_B_SPLINE_SURFACE(((0.982257720483865,0.990842547952629,1.,0.707106781186548,
1.,0.707106781186548,1.,0.707106781186548,1.,0.716264233233919,0.982257720483865),
(0.982257720483865,0.990842547952629,1.,0.707106781186548,1.,0.707106781186548,
1.,0.707106781186548,1.,0.716264233233919,0.982257720483865),(0.982257720483865,
0.990842547952629,1.,0.707106781186548,1.,0.707106781186548,1.,0.707106781186548,
1.,0.716264233233919,0.982257720483865),(0.982257720483865,0.990842547952629,
1.,0.707106781186548,1.,0.707106781186548,1.,0.707106781186548,1.,0.716264233233919,
0.982257720483865),(0.982257720483865,0.990842547952629,1.,0.707106781186548,
1.,0.707106781186548,1.,0.707106781186548,1.,0.716264233233919,0.982257720483865),
(0.982257720483865,0.990842547952629,1.,0.707106781186548,1.,0.707106781186548,
1.,0.707106781186548,1.,0.716264233233919,0.982257720483865),(0.982257720483865,
0.990842547952629,1.,0.707106781186548,1.,0.707106781186548,1.,0.707106781186548,
1.,0.716264233233919,0.982257720483865),(0.982257720483865,0.990842547952629,
1.,0.707106781186548,1.,0.707106781186548,1.,0.707106781186548,1.,0.716264233233919,
0.982257720483865),(0.982257720483865,0.990842547952629,1.,0.707106781186548,
1.,0.707106781186548,1.,0.707106781186548,1.,0.716264233233919,0.982257720483865),
(0.982257720483865,0.990842547952629,1.,0.707106781186548,1.,0.707106781186548,
1.,0.707106781186548,1.,0.716264233233919,0.982257720483865),(0.982257720483865,
0.990842547952629,1.,0.707106781186548,1.,0.707106781186548,1.,0.707106781186548,
1.,0.716264233233919,0.982257720483865),(0.982257720483865,0.990842547952629,
1.,0.707106781186548,1.,0.707106781186548,1.,0.707106781186548,1.,0.716264233233919,
0.982257720483865),(0.982257720483865,0.990842547952629,1.,0.707106781186548,
1.,0.707106781186548,1.,0.707106781186548,1.,0.716264233233919,0.982257720483865),
(0.982257720483865,0.990842547952629,1.,0.707106781186548,1.,0.707106781186548,
1.,0.707106781186548,1.,0.716264233233919,0.982257720483865),(0.982257720483865,
0.990842547952629,1.,0.707106781186548,1.,0.707106781186548,1.,0.707106781186548,
1.,0.716264233233919,0.982257720483865),(0.982257720483865,0.990842547952629,
1.,0.707106781186548,1.,0.707106781186548,1.,0.707106781186548,1.,0.716264233233919,
0.982257720483865),(0.982257720483865,0.990842547952629,1.,0.707106781186548,
1.,0.707106781186548,1.,0.707106781186548,1.,0.716264233233919,0.982257720483865),
(0.982257720483865,0.990842547952629,1.,0.707106781186548,1.,0.707106781186548,
1.,0.707106781186548,1.,0.716264233233919,0.982257720483865),(0.982257720483865,
0.990842547952629,1.,0.707106781186548,1.,0.707106781186548,1.,0.707106781186548,
1.,0.716264233233919,0.982257720483865),(0.982257720483865,0.990842547952629,
1.,0.707106781186548,1.,0.707106781186548,1.,0.707106781186548,1.,0.716264233233919,
0.982257720483865),(0.982257720483865,0.990842547952629,1.,0.707106781186548,
1.,0.707106781186548,1.,0.707106781186548,1.,0.716264233233919,0.982257720483865),
(0.982257720483865,0.990842547952629,1.,0.707106781186548,1.,0.707106781186548,
1.,0.707106781186548,1.,0.716264233233919,0.982257720483865),(0.982257720483865,
0.990842547952629,1.,0.707106781186548,1.,0.707106781186548,1.,0.707106781186548,
1.,0.716264233233919,0.982257720483865),(0.982257720483865,0.990842547952629,
1.,0.707106781186548,1.,0.707106781186548,1.,0.707106781186548,1.,0.716264233233919,
0.982257720483865),(0.982257720483865,0.990842547952629,1.,0.707106781186548,
1.,0.707106781186548,1.,0.707106781186548,1.,0.716264233233919,0.982257720483865)))
REPRESENTATION_ITEM('')
SURFACE()
);
#1073=(
BOUNDED_SURFACE()
B_SPLINE_SURFACE(5,2,((#39082,#39083,#39084,#39085,#39086,#39087,#39088,
#39089,#39090,#39091,#39092),(#39093,#39094,#39095,#39096,#39097,#39098,
#39099,#39100,#39101,#39102,#39103),(#39104,#39105,#39106,#39107,#39108,
#39109,#39110,#39111,#39112,#39113,#39114),(#39115,#39116,#39117,#39118,
#39119,#39120,#39121,#39122,#39123,#39124,#39125),(#39126,#39127,#39128,
#39129,#39130,#39131,#39132,#39133,#39134,#39135,#39136),(#39137,#39138,
#39139,#39140,#39141,#39142,#39143,#39144,#39145,#39146,#39147),(#39148,
#39149,#39150,#39151,#39152,#39153,#39154,#39155,#39156,#39157,#39158),
(#39159,#39160,#39161,#39162,#39163,#39164,#39165,#39166,#39167,#39168,
#39169),(#39170,#39171,#39172,#39173,#39174,#39175,#39176,#39177,#39178,
#39179,#39180),(#39181,#39182,#39183,#39184,#39185,#39186,#39187,#39188,
#39189,#39190,#39191),(#39192,#39193,#39194,#39195,#39196,#39197,#39198,
#39199,#39200,#39201,#39202),(#39203,#39204,#39205,#39206,#39207,#39208,
#39209,#39210,#39211,#39212,#39213),(#39214,#39215,#39216,#39217,#39218,
#39219,#39220,#39221,#39222,#39223,#39224),(#39225,#39226,#39227,#39228,
#39229,#39230,#39231,#39232,#39233,#39234,#39235),(#39236,#39237,#39238,
#39239,#39240,#39241,#39242,#39243,#39244,#39245,#39246),(#39247,#39248,
#39249,#39250,#39251,#39252,#39253,#39254,#39255,#39256,#39257),(#39258,
#39259,#39260,#39261,#39262,#39263,#39264,#39265,#39266,#39267,#39268),
(#39269,#39270,#39271,#39272,#39273,#39274,#39275,#39276,#39277,#39278,
#39279),(#39280,#39281,#39282,#39283,#39284,#39285,#39286,#39287,#39288,
#39289,#39290),(#39291,#39292,#39293,#39294,#39295,#39296,#39297,#39298,
#39299,#39300,#39301),(#39302,#39303,#39304,#39305,#39306,#39307,#39308,
#39309,#39310,#39311,#39312),(#39313,#39314,#39315,#39316,#39317,#39318,
#39319,#39320,#39321,#39322,#39323),(#39324,#39325,#39326,#39327,#39328,
#39329,#39330,#39331,#39332,#39333,#39334),(#39335,#39336,#39337,#39338,
#39339,#39340,#39341,#39342,#39343,#39344,#39345),(#39346,#39347,#39348,
#39349,#39350,#39351,#39352,#39353,#39354,#39355,#39356)),.UNSPECIFIED.,
 .F.,.T.,.F.)
B_SPLINE_SURFACE_WITH_KNOTS((6,1,1,1,1,1,1,1,1,1,1,1,1,1,1,1,1,1,1,1,6),
(3,2,2,2,2,3),(-1.,-0.95,-0.9,-0.85,-0.8,-0.75,-0.7,-0.65,-0.6,-0.55,-0.5,
-0.45,-0.4,-0.35,-0.3,-0.25,-0.2,-0.15,-0.1,-0.05,0.),(-0.0491117278067552,
0.,1.5707963267949,3.14159265358979,4.71238898038469,6.23407357937283),
 .UNSPECIFIED.)
GEOMETRIC_REPRESENTATION_ITEM()
RATIONAL_B_SPLINE_SURFACE(((0.982257720483865,0.990842547952629,1.,0.707106781186548,
1.,0.707106781186548,1.,0.707106781186548,1.,0.716264233233919,0.982257720483865),
(0.982257720483865,0.990842547952629,1.,0.707106781186548,1.,0.707106781186548,
1.,0.707106781186548,1.,0.716264233233919,0.982257720483865),(0.982257720483865,
0.990842547952629,1.,0.707106781186548,1.,0.707106781186548,1.,0.707106781186548,
1.,0.716264233233919,0.982257720483865),(0.982257720483865,0.990842547952629,
1.,0.707106781186548,1.,0.707106781186548,1.,0.707106781186548,1.,0.716264233233919,
0.982257720483865),(0.982257720483865,0.990842547952629,1.,0.707106781186548,
1.,0.707106781186548,1.,0.707106781186548,1.,0.716264233233919,0.982257720483865),
(0.982257720483865,0.990842547952629,1.,0.707106781186548,1.,0.707106781186548,
1.,0.707106781186548,1.,0.716264233233919,0.982257720483865),(0.982257720483865,
0.990842547952629,1.,0.707106781186548,1.,0.707106781186548,1.,0.707106781186548,
1.,0.716264233233919,0.982257720483865),(0.982257720483865,0.990842547952629,
1.,0.707106781186548,1.,0.707106781186548,1.,0.707106781186548,1.,0.716264233233919,
0.982257720483865),(0.982257720483865,0.990842547952629,1.,0.707106781186548,
1.,0.707106781186548,1.,0.707106781186548,1.,0.716264233233919,0.982257720483865),
(0.982257720483865,0.990842547952629,1.,0.707106781186548,1.,0.707106781186548,
1.,0.707106781186548,1.,0.716264233233919,0.982257720483865),(0.982257720483865,
0.990842547952629,1.,0.707106781186548,1.,0.707106781186548,1.,0.707106781186548,
1.,0.716264233233919,0.982257720483865),(0.982257720483865,0.990842547952629,
1.,0.707106781186548,1.,0.707106781186548,1.,0.707106781186548,1.,0.716264233233919,
0.982257720483865),(0.982257720483865,0.990842547952629,1.,0.707106781186548,
1.,0.707106781186548,1.,0.707106781186548,1.,0.716264233233919,0.982257720483865),
(0.982257720483865,0.990842547952629,1.,0.707106781186548,1.,0.707106781186548,
1.,0.707106781186548,1.,0.716264233233919,0.982257720483865),(0.982257720483865,
0.990842547952629,1.,0.707106781186548,1.,0.707106781186548,1.,0.707106781186548,
1.,0.716264233233919,0.982257720483865),(0.982257720483865,0.990842547952629,
1.,0.707106781186548,1.,0.707106781186548,1.,0.707106781186548,1.,0.716264233233919,
0.982257720483865),(0.982257720483865,0.990842547952629,1.,0.707106781186548,
1.,0.707106781186548,1.,0.707106781186548,1.,0.716264233233919,0.982257720483865),
(0.982257720483865,0.990842547952629,1.,0.707106781186548,1.,0.707106781186548,
1.,0.707106781186548,1.,0.716264233233919,0.982257720483865),(0.982257720483865,
0.990842547952629,1.,0.707106781186548,1.,0.707106781186548,1.,0.707106781186548,
1.,0.716264233233919,0.982257720483865),(0.982257720483865,0.990842547952629,
1.,0.707106781186548,1.,0.707106781186548,1.,0.707106781186548,1.,0.716264233233919,
0.982257720483865),(0.982257720483865,0.990842547952629,1.,0.707106781186548,
1.,0.707106781186548,1.,0.707106781186548,1.,0.716264233233919,0.982257720483865),
(0.982257720483865,0.990842547952629,1.,0.707106781186548,1.,0.707106781186548,
1.,0.707106781186548,1.,0.716264233233919,0.982257720483865),(0.982257720483865,
0.990842547952629,1.,0.707106781186548,1.,0.707106781186548,1.,0.707106781186548,
1.,0.716264233233919,0.982257720483865),(0.982257720483865,0.990842547952629,
1.,0.707106781186548,1.,0.707106781186548,1.,0.707106781186548,1.,0.716264233233919,
0.982257720483865),(0.982257720483865,0.990842547952629,1.,0.707106781186548,
1.,0.707106781186548,1.,0.707106781186548,1.,0.716264233233919,0.982257720483865)))
REPRESENTATION_ITEM('')
SURFACE()
);
#1074=(
BOUNDED_SURFACE()
B_SPLINE_SURFACE(5,2,((#39601,#39602,#39603,#39604,#39605,#39606,#39607,
#39608,#39609,#39610,#39611),(#39612,#39613,#39614,#39615,#39616,#39617,
#39618,#39619,#39620,#39621,#39622),(#39623,#39624,#39625,#39626,#39627,
#39628,#39629,#39630,#39631,#39632,#39633),(#39634,#39635,#39636,#39637,
#39638,#39639,#39640,#39641,#39642,#39643,#39644),(#39645,#39646,#39647,
#39648,#39649,#39650,#39651,#39652,#39653,#39654,#39655),(#39656,#39657,
#39658,#39659,#39660,#39661,#39662,#39663,#39664,#39665,#39666),(#39667,
#39668,#39669,#39670,#39671,#39672,#39673,#39674,#39675,#39676,#39677),
(#39678,#39679,#39680,#39681,#39682,#39683,#39684,#39685,#39686,#39687,
#39688),(#39689,#39690,#39691,#39692,#39693,#39694,#39695,#39696,#39697,
#39698,#39699),(#39700,#39701,#39702,#39703,#39704,#39705,#39706,#39707,
#39708,#39709,#39710),(#39711,#39712,#39713,#39714,#39715,#39716,#39717,
#39718,#39719,#39720,#39721),(#39722,#39723,#39724,#39725,#39726,#39727,
#39728,#39729,#39730,#39731,#39732),(#39733,#39734,#39735,#39736,#39737,
#39738,#39739,#39740,#39741,#39742,#39743),(#39744,#39745,#39746,#39747,
#39748,#39749,#39750,#39751,#39752,#39753,#39754),(#39755,#39756,#39757,
#39758,#39759,#39760,#39761,#39762,#39763,#39764,#39765),(#39766,#39767,
#39768,#39769,#39770,#39771,#39772,#39773,#39774,#39775,#39776),(#39777,
#39778,#39779,#39780,#39781,#39782,#39783,#39784,#39785,#39786,#39787),
(#39788,#39789,#39790,#39791,#39792,#39793,#39794,#39795,#39796,#39797,
#39798),(#39799,#39800,#39801,#39802,#39803,#39804,#39805,#39806,#39807,
#39808,#39809),(#39810,#39811,#39812,#39813,#39814,#39815,#39816,#39817,
#39818,#39819,#39820),(#39821,#39822,#39823,#39824,#39825,#39826,#39827,
#39828,#39829,#39830,#39831),(#39832,#39833,#39834,#39835,#39836,#39837,
#39838,#39839,#39840,#39841,#39842),(#39843,#39844,#39845,#39846,#39847,
#39848,#39849,#39850,#39851,#39852,#39853),(#39854,#39855,#39856,#39857,
#39858,#39859,#39860,#39861,#39862,#39863,#39864),(#39865,#39866,#39867,
#39868,#39869,#39870,#39871,#39872,#39873,#39874,#39875)),.UNSPECIFIED.,
 .F.,.T.,.F.)
B_SPLINE_SURFACE_WITH_KNOTS((6,1,1,1,1,1,1,1,1,1,1,1,1,1,1,1,1,1,1,1,6),
(3,2,2,2,2,3),(-1.,-0.95,-0.9,-0.85,-0.8,-0.75,-0.7,-0.65,-0.6,-0.55,-0.5,
-0.45,-0.4,-0.35,-0.3,-0.25,-0.2,-0.15,-0.1,-0.05,0.),(-0.0491117278067552,
0.,1.5707963267949,3.14159265358979,4.71238898038469,6.23407357937283),
 .UNSPECIFIED.)
GEOMETRIC_REPRESENTATION_ITEM()
RATIONAL_B_SPLINE_SURFACE(((0.982257720483865,0.990842547952629,1.,0.707106781186548,
1.,0.707106781186548,1.,0.707106781186548,1.,0.716264233233919,0.982257720483865),
(0.982257720483865,0.990842547952629,1.,0.707106781186548,1.,0.707106781186548,
1.,0.707106781186548,1.,0.716264233233919,0.982257720483865),(0.982257720483865,
0.990842547952629,1.,0.707106781186548,1.,0.707106781186548,1.,0.707106781186548,
1.,0.716264233233919,0.982257720483865),(0.982257720483865,0.990842547952629,
1.,0.707106781186548,1.,0.707106781186548,1.,0.707106781186548,1.,0.716264233233919,
0.982257720483865),(0.982257720483865,0.990842547952629,1.,0.707106781186548,
1.,0.707106781186548,1.,0.707106781186548,1.,0.716264233233919,0.982257720483865),
(0.982257720483865,0.990842547952629,1.,0.707106781186548,1.,0.707106781186548,
1.,0.707106781186548,1.,0.716264233233919,0.982257720483865),(0.982257720483865,
0.990842547952629,1.,0.707106781186548,1.,0.707106781186548,1.,0.707106781186548,
1.,0.716264233233919,0.982257720483865),(0.982257720483865,0.990842547952629,
1.,0.707106781186548,1.,0.707106781186548,1.,0.707106781186548,1.,0.716264233233919,
0.982257720483865),(0.982257720483865,0.990842547952629,1.,0.707106781186548,
1.,0.707106781186548,1.,0.707106781186548,1.,0.716264233233919,0.982257720483865),
(0.982257720483865,0.990842547952629,1.,0.707106781186548,1.,0.707106781186548,
1.,0.707106781186548,1.,0.716264233233919,0.982257720483865),(0.982257720483865,
0.990842547952629,1.,0.707106781186548,1.,0.707106781186548,1.,0.707106781186548,
1.,0.716264233233919,0.982257720483865),(0.982257720483865,0.990842547952629,
1.,0.707106781186548,1.,0.707106781186548,1.,0.707106781186548,1.,0.716264233233919,
0.982257720483865),(0.982257720483865,0.990842547952629,1.,0.707106781186548,
1.,0.707106781186548,1.,0.707106781186548,1.,0.716264233233919,0.982257720483865),
(0.982257720483865,0.990842547952629,1.,0.707106781186548,1.,0.707106781186548,
1.,0.707106781186548,1.,0.716264233233919,0.982257720483865),(0.982257720483865,
0.990842547952629,1.,0.707106781186548,1.,0.707106781186548,1.,0.707106781186548,
1.,0.716264233233919,0.982257720483865),(0.982257720483865,0.990842547952629,
1.,0.707106781186548,1.,0.707106781186548,1.,0.707106781186548,1.,0.716264233233919,
0.982257720483865),(0.982257720483865,0.990842547952629,1.,0.707106781186548,
1.,0.707106781186548,1.,0.707106781186548,1.,0.716264233233919,0.982257720483865),
(0.982257720483865,0.990842547952629,1.,0.707106781186548,1.,0.707106781186548,
1.,0.707106781186548,1.,0.716264233233919,0.982257720483865),(0.982257720483865,
0.990842547952629,1.,0.707106781186548,1.,0.707106781186548,1.,0.707106781186548,
1.,0.716264233233919,0.982257720483865),(0.982257720483865,0.990842547952629,
1.,0.707106781186548,1.,0.707106781186548,1.,0.707106781186548,1.,0.716264233233919,
0.982257720483865),(0.982257720483865,0.990842547952629,1.,0.707106781186548,
1.,0.707106781186548,1.,0.707106781186548,1.,0.716264233233919,0.982257720483865),
(0.982257720483865,0.990842547952629,1.,0.707106781186548,1.,0.707106781186548,
1.,0.707106781186548,1.,0.716264233233919,0.982257720483865),(0.982257720483865,
0.990842547952629,1.,0.707106781186548,1.,0.707106781186548,1.,0.707106781186548,
1.,0.716264233233919,0.982257720483865),(0.982257720483865,0.990842547952629,
1.,0.707106781186548,1.,0.707106781186548,1.,0.707106781186548,1.,0.716264233233919,
0.982257720483865),(0.982257720483865,0.990842547952629,1.,0.707106781186548,
1.,0.707106781186548,1.,0.707106781186548,1.,0.716264233233919,0.982257720483865)))
REPRESENTATION_ITEM('')
SURFACE()
);
#1075=(
BOUNDED_SURFACE()
B_SPLINE_SURFACE(5,2,((#40110,#40111,#40112,#40113,#40114,#40115,#40116,
#40117,#40118,#40119,#40120),(#40121,#40122,#40123,#40124,#40125,#40126,
#40127,#40128,#40129,#40130,#40131),(#40132,#40133,#40134,#40135,#40136,
#40137,#40138,#40139,#40140,#40141,#40142),(#40143,#40144,#40145,#40146,
#40147,#40148,#40149,#40150,#40151,#40152,#40153),(#40154,#40155,#40156,
#40157,#40158,#40159,#40160,#40161,#40162,#40163,#40164),(#40165,#40166,
#40167,#40168,#40169,#40170,#40171,#40172,#40173,#40174,#40175),(#40176,
#40177,#40178,#40179,#40180,#40181,#40182,#40183,#40184,#40185,#40186),
(#40187,#40188,#40189,#40190,#40191,#40192,#40193,#40194,#40195,#40196,
#40197),(#40198,#40199,#40200,#40201,#40202,#40203,#40204,#40205,#40206,
#40207,#40208),(#40209,#40210,#40211,#40212,#40213,#40214,#40215,#40216,
#40217,#40218,#40219),(#40220,#40221,#40222,#40223,#40224,#40225,#40226,
#40227,#40228,#40229,#40230),(#40231,#40232,#40233,#40234,#40235,#40236,
#40237,#40238,#40239,#40240,#40241),(#40242,#40243,#40244,#40245,#40246,
#40247,#40248,#40249,#40250,#40251,#40252),(#40253,#40254,#40255,#40256,
#40257,#40258,#40259,#40260,#40261,#40262,#40263),(#40264,#40265,#40266,
#40267,#40268,#40269,#40270,#40271,#40272,#40273,#40274),(#40275,#40276,
#40277,#40278,#40279,#40280,#40281,#40282,#40283,#40284,#40285),(#40286,
#40287,#40288,#40289,#40290,#40291,#40292,#40293,#40294,#40295,#40296),
(#40297,#40298,#40299,#40300,#40301,#40302,#40303,#40304,#40305,#40306,
#40307),(#40308,#40309,#40310,#40311,#40312,#40313,#40314,#40315,#40316,
#40317,#40318),(#40319,#40320,#40321,#40322,#40323,#40324,#40325,#40326,
#40327,#40328,#40329),(#40330,#40331,#40332,#40333,#40334,#40335,#40336,
#40337,#40338,#40339,#40340),(#40341,#40342,#40343,#40344,#40345,#40346,
#40347,#40348,#40349,#40350,#40351),(#40352,#40353,#40354,#40355,#40356,
#40357,#40358,#40359,#40360,#40361,#40362),(#40363,#40364,#40365,#40366,
#40367,#40368,#40369,#40370,#40371,#40372,#40373),(#40374,#40375,#40376,
#40377,#40378,#40379,#40380,#40381,#40382,#40383,#40384)),.UNSPECIFIED.,
 .F.,.T.,.F.)
B_SPLINE_SURFACE_WITH_KNOTS((6,1,1,1,1,1,1,1,1,1,1,1,1,1,1,1,1,1,1,1,6),
(3,2,2,2,2,3),(-1.,-0.95,-0.9,-0.85,-0.8,-0.75,-0.7,-0.65,-0.6,-0.55,-0.5,
-0.45,-0.4,-0.35,-0.3,-0.25,-0.2,-0.15,-0.1,-0.05,0.),(-0.0491117278067552,
0.,1.5707963267949,3.14159265358979,4.71238898038469,6.23407357937283),
 .UNSPECIFIED.)
GEOMETRIC_REPRESENTATION_ITEM()
RATIONAL_B_SPLINE_SURFACE(((0.982257720483865,0.990842547952629,1.,0.707106781186548,
1.,0.707106781186548,1.,0.707106781186548,1.,0.716264233233919,0.982257720483865),
(0.982257720483865,0.990842547952629,1.,0.707106781186548,1.,0.707106781186548,
1.,0.707106781186548,1.,0.716264233233919,0.982257720483865),(0.982257720483865,
0.990842547952629,1.,0.707106781186548,1.,0.707106781186548,1.,0.707106781186548,
1.,0.716264233233919,0.982257720483865),(0.982257720483865,0.990842547952629,
1.,0.707106781186548,1.,0.707106781186548,1.,0.707106781186548,1.,0.716264233233919,
0.982257720483865),(0.982257720483865,0.990842547952629,1.,0.707106781186548,
1.,0.707106781186548,1.,0.707106781186548,1.,0.716264233233919,0.982257720483865),
(0.982257720483865,0.990842547952629,1.,0.707106781186548,1.,0.707106781186548,
1.,0.707106781186548,1.,0.716264233233919,0.982257720483865),(0.982257720483865,
0.990842547952629,1.,0.707106781186548,1.,0.707106781186548,1.,0.707106781186548,
1.,0.716264233233919,0.982257720483865),(0.982257720483865,0.990842547952629,
1.,0.707106781186548,1.,0.707106781186548,1.,0.707106781186548,1.,0.716264233233919,
0.982257720483865),(0.982257720483865,0.990842547952629,1.,0.707106781186548,
1.,0.707106781186548,1.,0.707106781186548,1.,0.716264233233919,0.982257720483865),
(0.982257720483865,0.990842547952629,1.,0.707106781186548,1.,0.707106781186548,
1.,0.707106781186548,1.,0.716264233233919,0.982257720483865),(0.982257720483865,
0.990842547952629,1.,0.707106781186548,1.,0.707106781186548,1.,0.707106781186548,
1.,0.716264233233919,0.982257720483865),(0.982257720483865,0.990842547952629,
1.,0.707106781186548,1.,0.707106781186548,1.,0.707106781186548,1.,0.716264233233919,
0.982257720483865),(0.982257720483865,0.990842547952629,1.,0.707106781186548,
1.,0.707106781186548,1.,0.707106781186548,1.,0.716264233233919,0.982257720483865),
(0.982257720483865,0.990842547952629,1.,0.707106781186548,1.,0.707106781186548,
1.,0.707106781186548,1.,0.716264233233919,0.982257720483865),(0.982257720483865,
0.990842547952629,1.,0.707106781186548,1.,0.707106781186548,1.,0.707106781186548,
1.,0.716264233233919,0.982257720483865),(0.982257720483865,0.990842547952629,
1.,0.707106781186548,1.,0.707106781186548,1.,0.707106781186548,1.,0.716264233233919,
0.982257720483865),(0.982257720483865,0.990842547952629,1.,0.707106781186548,
1.,0.707106781186548,1.,0.707106781186548,1.,0.716264233233919,0.982257720483865),
(0.982257720483865,0.990842547952629,1.,0.707106781186548,1.,0.707106781186548,
1.,0.707106781186548,1.,0.716264233233919,0.982257720483865),(0.982257720483865,
0.990842547952629,1.,0.707106781186548,1.,0.707106781186548,1.,0.707106781186548,
1.,0.716264233233919,0.982257720483865),(0.982257720483865,0.990842547952629,
1.,0.707106781186548,1.,0.707106781186548,1.,0.707106781186548,1.,0.716264233233919,
0.982257720483865),(0.982257720483865,0.990842547952629,1.,0.707106781186548,
1.,0.707106781186548,1.,0.707106781186548,1.,0.716264233233919,0.982257720483865),
(0.982257720483865,0.990842547952629,1.,0.707106781186548,1.,0.707106781186548,
1.,0.707106781186548,1.,0.716264233233919,0.982257720483865),(0.982257720483865,
0.990842547952629,1.,0.707106781186548,1.,0.707106781186548,1.,0.707106781186548,
1.,0.716264233233919,0.982257720483865),(0.982257720483865,0.990842547952629,
1.,0.707106781186548,1.,0.707106781186548,1.,0.707106781186548,1.,0.716264233233919,
0.982257720483865),(0.982257720483865,0.990842547952629,1.,0.707106781186548,
1.,0.707106781186548,1.,0.707106781186548,1.,0.716264233233919,0.982257720483865)))
REPRESENTATION_ITEM('')
SURFACE()
);
#1076=(
BOUNDED_SURFACE()
B_SPLINE_SURFACE(5,2,((#40619,#40620,#40621,#40622,#40623,#40624,#40625,
#40626,#40627,#40628,#40629),(#40630,#40631,#40632,#40633,#40634,#40635,
#40636,#40637,#40638,#40639,#40640),(#40641,#40642,#40643,#40644,#40645,
#40646,#40647,#40648,#40649,#40650,#40651),(#40652,#40653,#40654,#40655,
#40656,#40657,#40658,#40659,#40660,#40661,#40662),(#40663,#40664,#40665,
#40666,#40667,#40668,#40669,#40670,#40671,#40672,#40673),(#40674,#40675,
#40676,#40677,#40678,#40679,#40680,#40681,#40682,#40683,#40684),(#40685,
#40686,#40687,#40688,#40689,#40690,#40691,#40692,#40693,#40694,#40695),
(#40696,#40697,#40698,#40699,#40700,#40701,#40702,#40703,#40704,#40705,
#40706),(#40707,#40708,#40709,#40710,#40711,#40712,#40713,#40714,#40715,
#40716,#40717),(#40718,#40719,#40720,#40721,#40722,#40723,#40724,#40725,
#40726,#40727,#40728),(#40729,#40730,#40731,#40732,#40733,#40734,#40735,
#40736,#40737,#40738,#40739),(#40740,#40741,#40742,#40743,#40744,#40745,
#40746,#40747,#40748,#40749,#40750),(#40751,#40752,#40753,#40754,#40755,
#40756,#40757,#40758,#40759,#40760,#40761),(#40762,#40763,#40764,#40765,
#40766,#40767,#40768,#40769,#40770,#40771,#40772),(#40773,#40774,#40775,
#40776,#40777,#40778,#40779,#40780,#40781,#40782,#40783),(#40784,#40785,
#40786,#40787,#40788,#40789,#40790,#40791,#40792,#40793,#40794),(#40795,
#40796,#40797,#40798,#40799,#40800,#40801,#40802,#40803,#40804,#40805),
(#40806,#40807,#40808,#40809,#40810,#40811,#40812,#40813,#40814,#40815,
#40816),(#40817,#40818,#40819,#40820,#40821,#40822,#40823,#40824,#40825,
#40826,#40827),(#40828,#40829,#40830,#40831,#40832,#40833,#40834,#40835,
#40836,#40837,#40838),(#40839,#40840,#40841,#40842,#40843,#40844,#40845,
#40846,#40847,#40848,#40849),(#40850,#40851,#40852,#40853,#40854,#40855,
#40856,#40857,#40858,#40859,#40860),(#40861,#40862,#40863,#40864,#40865,
#40866,#40867,#40868,#40869,#40870,#40871),(#40872,#40873,#40874,#40875,
#40876,#40877,#40878,#40879,#40880,#40881,#40882),(#40883,#40884,#40885,
#40886,#40887,#40888,#40889,#40890,#40891,#40892,#40893)),.UNSPECIFIED.,
 .F.,.T.,.F.)
B_SPLINE_SURFACE_WITH_KNOTS((6,1,1,1,1,1,1,1,1,1,1,1,1,1,1,1,1,1,1,1,6),
(3,2,2,2,2,3),(-1.,-0.95,-0.9,-0.85,-0.8,-0.75,-0.7,-0.65,-0.6,-0.55,-0.5,
-0.45,-0.4,-0.35,-0.3,-0.25,-0.2,-0.15,-0.1,-0.05,0.),(-0.0491117278067552,
0.,1.5707963267949,3.14159265358979,4.71238898038469,6.23407357937283),
 .UNSPECIFIED.)
GEOMETRIC_REPRESENTATION_ITEM()
RATIONAL_B_SPLINE_SURFACE(((0.982257720483865,0.990842547952629,1.,0.707106781186548,
1.,0.707106781186548,1.,0.707106781186548,1.,0.716264233233919,0.982257720483865),
(0.982257720483865,0.990842547952629,1.,0.707106781186548,1.,0.707106781186548,
1.,0.707106781186548,1.,0.716264233233919,0.982257720483865),(0.982257720483865,
0.990842547952629,1.,0.707106781186548,1.,0.707106781186548,1.,0.707106781186548,
1.,0.716264233233919,0.982257720483865),(0.982257720483865,0.990842547952629,
1.,0.707106781186548,1.,0.707106781186548,1.,0.707106781186548,1.,0.716264233233919,
0.982257720483865),(0.982257720483865,0.990842547952629,1.,0.707106781186548,
1.,0.707106781186548,1.,0.707106781186548,1.,0.716264233233919,0.982257720483865),
(0.982257720483865,0.990842547952629,1.,0.707106781186548,1.,0.707106781186548,
1.,0.707106781186548,1.,0.716264233233919,0.982257720483865),(0.982257720483865,
0.990842547952629,1.,0.707106781186548,1.,0.707106781186548,1.,0.707106781186548,
1.,0.716264233233919,0.982257720483865),(0.982257720483865,0.990842547952629,
1.,0.707106781186548,1.,0.707106781186548,1.,0.707106781186548,1.,0.716264233233919,
0.982257720483865),(0.982257720483865,0.990842547952629,1.,0.707106781186548,
1.,0.707106781186548,1.,0.707106781186548,1.,0.716264233233919,0.982257720483865),
(0.982257720483865,0.990842547952629,1.,0.707106781186548,1.,0.707106781186548,
1.,0.707106781186548,1.,0.716264233233919,0.982257720483865),(0.982257720483865,
0.990842547952629,1.,0.707106781186548,1.,0.707106781186548,1.,0.707106781186548,
1.,0.716264233233919,0.982257720483865),(0.982257720483865,0.990842547952629,
1.,0.707106781186548,1.,0.707106781186548,1.,0.707106781186548,1.,0.716264233233919,
0.982257720483865),(0.982257720483865,0.990842547952629,1.,0.707106781186548,
1.,0.707106781186548,1.,0.707106781186548,1.,0.716264233233919,0.982257720483865),
(0.982257720483865,0.990842547952629,1.,0.707106781186548,1.,0.707106781186548,
1.,0.707106781186548,1.,0.716264233233919,0.982257720483865),(0.982257720483865,
0.990842547952629,1.,0.707106781186548,1.,0.707106781186548,1.,0.707106781186548,
1.,0.716264233233919,0.982257720483865),(0.982257720483865,0.990842547952629,
1.,0.707106781186548,1.,0.707106781186548,1.,0.707106781186548,1.,0.716264233233919,
0.982257720483865),(0.982257720483865,0.990842547952629,1.,0.707106781186548,
1.,0.707106781186548,1.,0.707106781186548,1.,0.716264233233919,0.982257720483865),
(0.982257720483865,0.990842547952629,1.,0.707106781186548,1.,0.707106781186548,
1.,0.707106781186548,1.,0.716264233233919,0.982257720483865),(0.982257720483865,
0.990842547952629,1.,0.707106781186548,1.,0.707106781186548,1.,0.707106781186548,
1.,0.716264233233919,0.982257720483865),(0.982257720483865,0.990842547952629,
1.,0.707106781186548,1.,0.707106781186548,1.,0.707106781186548,1.,0.716264233233919,
0.982257720483865),(0.982257720483865,0.990842547952629,1.,0.707106781186548,
1.,0.707106781186548,1.,0.707106781186548,1.,0.716264233233919,0.982257720483865),
(0.982257720483865,0.990842547952629,1.,0.707106781186548,1.,0.707106781186548,
1.,0.707106781186548,1.,0.716264233233919,0.982257720483865),(0.982257720483865,
0.990842547952629,1.,0.707106781186548,1.,0.707106781186548,1.,0.707106781186548,
1.,0.716264233233919,0.982257720483865),(0.982257720483865,0.990842547952629,
1.,0.707106781186548,1.,0.707106781186548,1.,0.707106781186548,1.,0.716264233233919,
0.982257720483865),(0.982257720483865,0.990842547952629,1.,0.707106781186548,
1.,0.707106781186548,1.,0.707106781186548,1.,0.716264233233919,0.982257720483865)))
REPRESENTATION_ITEM('')
SURFACE()
);
#1077=(
BOUNDED_SURFACE()
B_SPLINE_SURFACE(5,2,((#41138,#41139,#41140,#41141,#41142,#41143,#41144,
#41145,#41146,#41147,#41148),(#41149,#41150,#41151,#41152,#41153,#41154,
#41155,#41156,#41157,#41158,#41159),(#41160,#41161,#41162,#41163,#41164,
#41165,#41166,#41167,#41168,#41169,#41170),(#41171,#41172,#41173,#41174,
#41175,#41176,#41177,#41178,#41179,#41180,#41181),(#41182,#41183,#41184,
#41185,#41186,#41187,#41188,#41189,#41190,#41191,#41192),(#41193,#41194,
#41195,#41196,#41197,#41198,#41199,#41200,#41201,#41202,#41203),(#41204,
#41205,#41206,#41207,#41208,#41209,#41210,#41211,#41212,#41213,#41214),
(#41215,#41216,#41217,#41218,#41219,#41220,#41221,#41222,#41223,#41224,
#41225),(#41226,#41227,#41228,#41229,#41230,#41231,#41232,#41233,#41234,
#41235,#41236),(#41237,#41238,#41239,#41240,#41241,#41242,#41243,#41244,
#41245,#41246,#41247),(#41248,#41249,#41250,#41251,#41252,#41253,#41254,
#41255,#41256,#41257,#41258),(#41259,#41260,#41261,#41262,#41263,#41264,
#41265,#41266,#41267,#41268,#41269),(#41270,#41271,#41272,#41273,#41274,
#41275,#41276,#41277,#41278,#41279,#41280),(#41281,#41282,#41283,#41284,
#41285,#41286,#41287,#41288,#41289,#41290,#41291),(#41292,#41293,#41294,
#41295,#41296,#41297,#41298,#41299,#41300,#41301,#41302),(#41303,#41304,
#41305,#41306,#41307,#41308,#41309,#41310,#41311,#41312,#41313),(#41314,
#41315,#41316,#41317,#41318,#41319,#41320,#41321,#41322,#41323,#41324),
(#41325,#41326,#41327,#41328,#41329,#41330,#41331,#41332,#41333,#41334,
#41335),(#41336,#41337,#41338,#41339,#41340,#41341,#41342,#41343,#41344,
#41345,#41346),(#41347,#41348,#41349,#41350,#41351,#41352,#41353,#41354,
#41355,#41356,#41357),(#41358,#41359,#41360,#41361,#41362,#41363,#41364,
#41365,#41366,#41367,#41368),(#41369,#41370,#41371,#41372,#41373,#41374,
#41375,#41376,#41377,#41378,#41379),(#41380,#41381,#41382,#41383,#41384,
#41385,#41386,#41387,#41388,#41389,#41390),(#41391,#41392,#41393,#41394,
#41395,#41396,#41397,#41398,#41399,#41400,#41401),(#41402,#41403,#41404,
#41405,#41406,#41407,#41408,#41409,#41410,#41411,#41412)),.UNSPECIFIED.,
 .F.,.T.,.F.)
B_SPLINE_SURFACE_WITH_KNOTS((6,1,1,1,1,1,1,1,1,1,1,1,1,1,1,1,1,1,1,1,6),
(3,2,2,2,2,3),(-1.,-0.95,-0.9,-0.85,-0.8,-0.75,-0.7,-0.65,-0.6,-0.55,-0.5,
-0.45,-0.4,-0.35,-0.3,-0.25,-0.2,-0.15,-0.1,-0.05,0.),(-0.0491117278067552,
0.,1.5707963267949,3.14159265358979,4.71238898038469,6.23407357937283),
 .UNSPECIFIED.)
GEOMETRIC_REPRESENTATION_ITEM()
RATIONAL_B_SPLINE_SURFACE(((0.982257720483865,0.990842547952629,1.,0.707106781186548,
1.,0.707106781186548,1.,0.707106781186548,1.,0.716264233233919,0.982257720483865),
(0.982257720483865,0.990842547952629,1.,0.707106781186548,1.,0.707106781186548,
1.,0.707106781186548,1.,0.716264233233919,0.982257720483865),(0.982257720483865,
0.990842547952629,1.,0.707106781186548,1.,0.707106781186548,1.,0.707106781186548,
1.,0.716264233233919,0.982257720483865),(0.982257720483865,0.990842547952629,
1.,0.707106781186548,1.,0.707106781186548,1.,0.707106781186548,1.,0.716264233233919,
0.982257720483865),(0.982257720483865,0.990842547952629,1.,0.707106781186548,
1.,0.707106781186548,1.,0.707106781186548,1.,0.716264233233919,0.982257720483865),
(0.982257720483865,0.990842547952629,1.,0.707106781186548,1.,0.707106781186548,
1.,0.707106781186548,1.,0.716264233233919,0.982257720483865),(0.982257720483865,
0.990842547952629,1.,0.707106781186548,1.,0.707106781186548,1.,0.707106781186548,
1.,0.716264233233919,0.982257720483865),(0.982257720483865,0.990842547952629,
1.,0.707106781186548,1.,0.707106781186548,1.,0.707106781186548,1.,0.716264233233919,
0.982257720483865),(0.982257720483865,0.990842547952629,1.,0.707106781186548,
1.,0.707106781186548,1.,0.707106781186548,1.,0.716264233233919,0.982257720483865),
(0.982257720483865,0.990842547952629,1.,0.707106781186548,1.,0.707106781186548,
1.,0.707106781186548,1.,0.716264233233919,0.982257720483865),(0.982257720483865,
0.990842547952629,1.,0.707106781186548,1.,0.707106781186548,1.,0.707106781186548,
1.,0.716264233233919,0.982257720483865),(0.982257720483865,0.990842547952629,
1.,0.707106781186548,1.,0.707106781186548,1.,0.707106781186548,1.,0.716264233233919,
0.982257720483865),(0.982257720483865,0.990842547952629,1.,0.707106781186548,
1.,0.707106781186548,1.,0.707106781186548,1.,0.716264233233919,0.982257720483865),
(0.982257720483865,0.990842547952629,1.,0.707106781186548,1.,0.707106781186548,
1.,0.707106781186548,1.,0.716264233233919,0.982257720483865),(0.982257720483865,
0.990842547952629,1.,0.707106781186548,1.,0.707106781186548,1.,0.707106781186548,
1.,0.716264233233919,0.982257720483865),(0.982257720483865,0.990842547952629,
1.,0.707106781186548,1.,0.707106781186548,1.,0.707106781186548,1.,0.716264233233919,
0.982257720483865),(0.982257720483865,0.990842547952629,1.,0.707106781186548,
1.,0.707106781186548,1.,0.707106781186548,1.,0.716264233233919,0.982257720483865),
(0.982257720483865,0.990842547952629,1.,0.707106781186548,1.,0.707106781186548,
1.,0.707106781186548,1.,0.716264233233919,0.982257720483865),(0.982257720483865,
0.990842547952629,1.,0.707106781186548,1.,0.707106781186548,1.,0.707106781186548,
1.,0.716264233233919,0.982257720483865),(0.982257720483865,0.990842547952629,
1.,0.707106781186548,1.,0.707106781186548,1.,0.707106781186548,1.,0.716264233233919,
0.982257720483865),(0.982257720483865,0.990842547952629,1.,0.707106781186548,
1.,0.707106781186548,1.,0.707106781186548,1.,0.716264233233919,0.982257720483865),
(0.982257720483865,0.990842547952629,1.,0.707106781186548,1.,0.707106781186548,
1.,0.707106781186548,1.,0.716264233233919,0.982257720483865),(0.982257720483865,
0.990842547952629,1.,0.707106781186548,1.,0.707106781186548,1.,0.707106781186548,
1.,0.716264233233919,0.982257720483865),(0.982257720483865,0.990842547952629,
1.,0.707106781186548,1.,0.707106781186548,1.,0.707106781186548,1.,0.716264233233919,
0.982257720483865),(0.982257720483865,0.990842547952629,1.,0.707106781186548,
1.,0.707106781186548,1.,0.707106781186548,1.,0.716264233233919,0.982257720483865)))
REPRESENTATION_ITEM('')
SURFACE()
);
#1098=STYLED_ITEM('',(#60527),#17349);
#1099=STYLED_ITEM('',(#60527),#17370);
#1100=STYLED_ITEM('',(#60527),#17371);
#1101=STYLED_ITEM('',(#60527),#17372);
#1102=STYLED_ITEM('',(#60527),#17374);
#1103=STYLED_ITEM('',(#60527),#17375);
#1104=STYLED_ITEM('',(#60527),#17376);
#1105=STYLED_ITEM('',(#60527),#17378);
#1106=STYLED_ITEM('',(#60527),#17379);
#1107=STYLED_ITEM('',(#60527),#17380);
#1108=STYLED_ITEM('',(#60527),#17382);
#1109=STYLED_ITEM('',(#60527),#17383);
#1110=STYLED_ITEM('',(#60527),#17384);
#1111=STYLED_ITEM('',(#60527),#17386);
#1112=STYLED_ITEM('',(#60527),#17387);
#1113=STYLED_ITEM('',(#60527),#17388);
#1114=STYLED_ITEM('',(#60527),#17390);
#1115=STYLED_ITEM('',(#60527),#17391);
#1116=STYLED_ITEM('',(#60527),#17392);
#1117=STYLED_ITEM('',(#60527),#17394);
#1118=STYLED_ITEM('',(#60527),#17395);
#1119=STYLED_ITEM('',(#60527),#17397);
#1120=STYLED_ITEM('',(#60527),#17398);
#1121=STYLED_ITEM('',(#60527),#17399);
#1122=STYLED_ITEM('',(#60527),#17401);
#1123=STYLED_ITEM('',(#60527),#17402);
#1124=STYLED_ITEM('',(#60527),#17403);
#1125=STYLED_ITEM('',(#60527),#17405);
#1126=STYLED_ITEM('',(#60527),#17406);
#1127=STYLED_ITEM('',(#60527),#17407);
#1128=STYLED_ITEM('',(#60527),#17409);
#1129=STYLED_ITEM('',(#60527),#17410);
#1130=STYLED_ITEM('',(#60527),#17411);
#1131=STYLED_ITEM('',(#60527),#17413);
#1132=STYLED_ITEM('',(#60527),#17414);
#1133=STYLED_ITEM('',(#60527),#17415);
#1134=STYLED_ITEM('',(#60527),#17417);
#1135=STYLED_ITEM('',(#60527),#17418);
#1136=STYLED_ITEM('',(#60527),#17420);
#1137=STYLED_ITEM('',(#60527),#17421);
#1138=STYLED_ITEM('',(#60527),#17423);
#1139=STYLED_ITEM('',(#60527),#17424);
#1140=STYLED_ITEM('',(#60527),#17426);
#1141=STYLED_ITEM('',(#60527),#17427);
#1142=STYLED_ITEM('',(#60527),#17429);
#1143=STYLED_ITEM('',(#60527),#17430);
#1144=STYLED_ITEM('',(#60527),#17432);
#1145=STYLED_ITEM('',(#60527),#17433);
#1146=STYLED_ITEM('',(#60527),#17435);
#1147=STYLED_ITEM('',(#60527),#17436);
#1148=STYLED_ITEM('',(#60527),#17438);
#1149=STYLED_ITEM('',(#60527),#17439);
#1150=STYLED_ITEM('',(#60527),#17441);
#1151=STYLED_ITEM('',(#60527),#17442);
#1152=STYLED_ITEM('',(#60527),#17444);
#1153=STYLED_ITEM('',(#60527),#17445);
#1154=STYLED_ITEM('',(#60527),#17447);
#1155=STYLED_ITEM('',(#60527),#17448);
#1156=STYLED_ITEM('',(#60527),#17450);
#1157=STYLED_ITEM('',(#60527),#17451);
#1158=STYLED_ITEM('',(#60527),#17460);
#1159=STYLED_ITEM('',(#60527),#17461);
#1160=STYLED_ITEM('',(#60527),#17465);
#1161=STYLED_ITEM('',(#60527),#17466);
#1162=STYLED_ITEM('',(#60527),#17470);
#1163=STYLED_ITEM('',(#60527),#17471);
#1164=STYLED_ITEM('',(#60527),#17475);
#1165=STYLED_ITEM('',(#60527),#17476);
#1166=STYLED_ITEM('',(#60527),#17480);
#1167=STYLED_ITEM('',(#60527),#17481);
#1168=STYLED_ITEM('',(#60527),#17484);
#1169=STYLED_ITEM('',(#60527),#17485);
#1170=STYLED_ITEM('',(#60527),#17487);
#1171=STYLED_ITEM('',(#60527),#17488);
#1172=STYLED_ITEM('',(#60527),#17490);
#1173=STYLED_ITEM('',(#60527),#17493);
#1174=STYLED_ITEM('',(#60527),#17495);
#1175=STYLED_ITEM('',(#60527),#17498);
#1176=STYLED_ITEM('',(#60527),#17500);
#1177=STYLED_ITEM('',(#60527),#17503);
#1178=STYLED_ITEM('',(#60527),#17505);
#1179=STYLED_ITEM('',(#60527),#17508);
#1180=STYLED_ITEM('',(#60527),#17510);
#1181=STYLED_ITEM('',(#60527),#17513);
#1182=STYLED_ITEM('',(#60527),#17515);
#1183=STYLED_ITEM('',(#60527),#17516);
#1184=STYLED_ITEM('',(#60527),#17517);
#1185=STYLED_ITEM('',(#60527),#17521);
#1186=STYLED_ITEM('',(#60527),#17522);
#1187=STYLED_ITEM('',(#60527),#17528);
#1188=STYLED_ITEM('',(#60527),#17529);
#1189=STYLED_ITEM('',(#60527),#17530);
#1190=STYLED_ITEM('',(#60527),#17531);
#1191=STYLED_ITEM('',(#60527),#17532);
#1192=STYLED_ITEM('',(#60527),#17533);
#1193=STYLED_ITEM('',(#60527),#17534);
#1194=STYLED_ITEM('',(#60527),#17535);
#1195=STYLED_ITEM('',(#60527),#17536);
#1196=STYLED_ITEM('',(#60527),#17537);
#1197=STYLED_ITEM('',(#60527),#17538);
#1198=STYLED_ITEM('',(#60527),#17539);
#1199=STYLED_ITEM('',(#60527),#17540);
#1200=STYLED_ITEM('',(#60527),#17541);
#1201=STYLED_ITEM('',(#60527),#17542);
#1202=STYLED_ITEM('',(#60527),#17543);
#1203=STYLED_ITEM('',(#60527),#17544);
#1204=STYLED_ITEM('',(#60527),#17545);
#1205=STYLED_ITEM('',(#60527),#17546);
#1206=STYLED_ITEM('',(#60527),#17547);
#1207=STYLED_ITEM('',(#60527),#17548);
#1208=STYLED_ITEM('',(#60527),#17549);
#1209=STYLED_ITEM('',(#60527),#17550);
#1210=STYLED_ITEM('',(#60527),#17551);
#1211=STYLED_ITEM('',(#60527),#17552);
#1212=STYLED_ITEM('',(#60527),#17553);
#1213=STYLED_ITEM('',(#60527),#17554);
#1214=STYLED_ITEM('',(#60527),#17555);
#1215=STYLED_ITEM('',(#60527),#17556);
#1216=STYLED_ITEM('',(#60527),#17557);
#1217=STYLED_ITEM('',(#60527),#17558);
#1218=STYLED_ITEM('',(#60527),#17559);
#1219=STYLED_ITEM('',(#60527),#17560);
#1220=STYLED_ITEM('',(#60527),#17561);
#1221=STYLED_ITEM('',(#60527),#17562);
#1222=STYLED_ITEM('',(#60527),#17563);
#1223=STYLED_ITEM('',(#60527),#17564);
#1224=STYLED_ITEM('',(#60527),#17565);
#1225=STYLED_ITEM('',(#60527),#17566);
#1226=STYLED_ITEM('',(#60527),#17567);
#1227=STYLED_ITEM('',(#60527),#17568);
#1228=STYLED_ITEM('',(#60527),#17569);
#1229=STYLED_ITEM('',(#60527),#17570);
#1230=STYLED_ITEM('',(#60527),#17571);
#1231=STYLED_ITEM('',(#60527),#17572);
#1232=STYLED_ITEM('',(#60527),#17578);
#1233=STYLED_ITEM('',(#60527),#17579);
#1234=STYLED_ITEM('',(#60527),#17580);
#1235=STYLED_ITEM('',(#60527),#17581);
#1236=STYLED_ITEM('',(#60527),#17582);
#1237=STYLED_ITEM('',(#60527),#17583);
#1238=STYLED_ITEM('',(#60527),#17584);
#1239=STYLED_ITEM('',(#60527),#17585);
#1240=STYLED_ITEM('',(#60527),#17586);
#1241=STYLED_ITEM('',(#60527),#17587);
#1242=STYLED_ITEM('',(#60527),#17588);
#1243=STYLED_ITEM('',(#60527),#17589);
#1244=STYLED_ITEM('',(#60527),#17590);
#1245=STYLED_ITEM('',(#60527),#17591);
#1246=STYLED_ITEM('',(#60527),#17592);
#1247=STYLED_ITEM('',(#60527),#17593);
#1248=STYLED_ITEM('',(#60527),#17594);
#1249=STYLED_ITEM('',(#60527),#17595);
#1250=STYLED_ITEM('',(#60527),#17596);
#1251=STYLED_ITEM('',(#60527),#17597);
#1252=STYLED_ITEM('',(#60527),#17598);
#1253=STYLED_ITEM('',(#60527),#17599);
#1254=STYLED_ITEM('',(#60527),#17600);
#1255=STYLED_ITEM('',(#60527),#17601);
#1256=STYLED_ITEM('',(#60527),#17602);
#1257=STYLED_ITEM('',(#60527),#17603);
#1258=STYLED_ITEM('',(#60527),#17604);
#1259=STYLED_ITEM('',(#60527),#17605);
#1260=STYLED_ITEM('',(#60527),#17606);
#1261=STYLED_ITEM('',(#60527),#17607);
#1262=STYLED_ITEM('',(#60527),#17608);
#1263=STYLED_ITEM('',(#60527),#17609);
#1264=STYLED_ITEM('',(#60527),#17610);
#1265=STYLED_ITEM('',(#60527),#17611);
#1266=STYLED_ITEM('',(#60527),#17612);
#1267=STYLED_ITEM('',(#60527),#17613);
#1268=STYLED_ITEM('',(#60527),#17614);
#1269=STYLED_ITEM('',(#60527),#17615);
#1270=STYLED_ITEM('',(#60527),#17616);
#1271=STYLED_ITEM('',(#60527),#17617);
#1272=STYLED_ITEM('',(#60527),#17618);
#1273=STYLED_ITEM('',(#60527),#17619);
#1274=STYLED_ITEM('',(#60527),#17620);
#1275=STYLED_ITEM('',(#60527),#17621);
#1276=STYLED_ITEM('',(#60527),#17622);
#1277=STYLED_ITEM('',(#60527),#17623);
#1278=STYLED_ITEM('',(#60527),#17624);
#1279=STYLED_ITEM('',(#60527),#17625);
#1280=STYLED_ITEM('',(#60527),#17626);
#1281=STYLED_ITEM('',(#60527),#17627);
#1282=STYLED_ITEM('',(#60527),#17628);
#1283=STYLED_ITEM('',(#60527),#17629);
#1284=STYLED_ITEM('',(#60527),#17630);
#1285=STYLED_ITEM('',(#60527),#17631);
#1286=STYLED_ITEM('',(#60527),#17632);
#1287=STYLED_ITEM('',(#60527),#17633);
#1288=STYLED_ITEM('',(#60527),#17634);
#1289=STYLED_ITEM('',(#60527),#17635);
#1290=STYLED_ITEM('',(#60527),#17636);
#1291=STYLED_ITEM('',(#60527),#17637);
#1292=STYLED_ITEM('',(#60527),#17638);
#1293=STYLED_ITEM('',(#60527),#17639);
#1294=STYLED_ITEM('',(#60527),#17640);
#1295=STYLED_ITEM('',(#60527),#87);
#1305=FACE_OUTER_BOUND('',#2269,.T.);
#1306=FACE_OUTER_BOUND('',#2270,.T.);
#1307=FACE_OUTER_BOUND('',#2271,.T.);
#1308=FACE_OUTER_BOUND('',#2272,.T.);
#1309=FACE_OUTER_BOUND('',#2273,.T.);
#1310=FACE_OUTER_BOUND('',#2274,.T.);
#1311=FACE_OUTER_BOUND('',#2275,.T.);
#1312=FACE_OUTER_BOUND('',#2276,.T.);
#1313=FACE_OUTER_BOUND('',#2277,.T.);
#1314=FACE_OUTER_BOUND('',#2278,.T.);
#1315=FACE_OUTER_BOUND('',#2279,.T.);
#1316=FACE_OUTER_BOUND('',#2280,.T.);
#1317=FACE_OUTER_BOUND('',#2281,.T.);
#1318=FACE_OUTER_BOUND('',#2282,.T.);
#1319=FACE_OUTER_BOUND('',#2283,.T.);
#1320=FACE_OUTER_BOUND('',#2284,.T.);
#1321=FACE_OUTER_BOUND('',#2285,.T.);
#1322=FACE_OUTER_BOUND('',#2286,.T.);
#1323=FACE_OUTER_BOUND('',#2287,.T.);
#1324=FACE_OUTER_BOUND('',#2288,.T.);
#1325=FACE_OUTER_BOUND('',#2289,.T.);
#1326=FACE_OUTER_BOUND('',#2290,.T.);
#1327=FACE_OUTER_BOUND('',#2291,.T.);
#1328=FACE_OUTER_BOUND('',#2292,.T.);
#1329=FACE_OUTER_BOUND('',#2293,.T.);
#1330=FACE_OUTER_BOUND('',#2294,.T.);
#1331=FACE_OUTER_BOUND('',#2295,.T.);
#1332=FACE_OUTER_BOUND('',#2296,.T.);
#1333=FACE_OUTER_BOUND('',#2297,.T.);
#1334=FACE_OUTER_BOUND('',#2298,.T.);
#1335=FACE_OUTER_BOUND('',#2299,.T.);
#1336=FACE_OUTER_BOUND('',#2300,.T.);
#1337=FACE_OUTER_BOUND('',#2301,.T.);
#1338=FACE_OUTER_BOUND('',#2302,.T.);
#1339=FACE_OUTER_BOUND('',#2303,.T.);
#1340=FACE_OUTER_BOUND('',#2304,.T.);
#1341=FACE_OUTER_BOUND('',#2306,.T.);
#1342=FACE_OUTER_BOUND('',#2307,.T.);
#1343=FACE_OUTER_BOUND('',#2308,.T.);
#1344=FACE_OUTER_BOUND('',#2309,.T.);
#1345=FACE_OUTER_BOUND('',#2310,.T.);
#1346=FACE_OUTER_BOUND('',#2311,.T.);
#1347=FACE_OUTER_BOUND('',#2312,.T.);
#1348=FACE_OUTER_BOUND('',#2313,.T.);
#1349=FACE_OUTER_BOUND('',#2314,.T.);
#1350=FACE_OUTER_BOUND('',#2315,.T.);
#1351=FACE_OUTER_BOUND('',#2316,.T.);
#1352=FACE_OUTER_BOUND('',#2317,.T.);
#1353=FACE_OUTER_BOUND('',#2318,.T.);
#1354=FACE_OUTER_BOUND('',#2319,.T.);
#1355=FACE_OUTER_BOUND('',#2320,.T.);
#1356=FACE_OUTER_BOUND('',#2321,.T.);
#1357=FACE_OUTER_BOUND('',#2322,.T.);
#1358=FACE_OUTER_BOUND('',#2323,.T.);
#1359=FACE_OUTER_BOUND('',#2324,.T.);
#1360=FACE_OUTER_BOUND('',#2325,.T.);
#1361=FACE_OUTER_BOUND('',#2326,.T.);
#1362=FACE_OUTER_BOUND('',#2327,.T.);
#1363=FACE_OUTER_BOUND('',#2328,.T.);
#1364=FACE_OUTER_BOUND('',#2329,.T.);
#1365=FACE_OUTER_BOUND('',#2330,.T.);
#1366=FACE_OUTER_BOUND('',#2331,.T.);
#1367=FACE_OUTER_BOUND('',#2332,.T.);
#1368=FACE_OUTER_BOUND('',#2333,.T.);
#1369=FACE_OUTER_BOUND('',#2334,.T.);
#1370=FACE_OUTER_BOUND('',#2335,.T.);
#1371=FACE_OUTER_BOUND('',#2336,.T.);
#1372=FACE_OUTER_BOUND('',#2337,.T.);
#1373=FACE_OUTER_BOUND('',#2338,.T.);
#1374=FACE_OUTER_BOUND('',#2339,.T.);
#1375=FACE_OUTER_BOUND('',#2340,.T.);
#1376=FACE_OUTER_BOUND('',#2341,.T.);
#1377=FACE_OUTER_BOUND('',#2342,.T.);
#1378=FACE_OUTER_BOUND('',#2343,.T.);
#1379=FACE_OUTER_BOUND('',#2344,.T.);
#1380=FACE_OUTER_BOUND('',#2345,.T.);
#1381=FACE_OUTER_BOUND('',#2346,.T.);
#1382=FACE_OUTER_BOUND('',#2347,.T.);
#1383=FACE_OUTER_BOUND('',#2348,.T.);
#1384=FACE_OUTER_BOUND('',#2349,.T.);
#1385=FACE_OUTER_BOUND('',#2350,.T.);
#1386=FACE_OUTER_BOUND('',#2351,.T.);
#1387=FACE_OUTER_BOUND('',#2352,.T.);
#1388=FACE_OUTER_BOUND('',#2353,.T.);
#1389=FACE_OUTER_BOUND('',#2354,.T.);
#1390=FACE_OUTER_BOUND('',#2355,.T.);
#1391=FACE_OUTER_BOUND('',#2356,.T.);
#1392=FACE_OUTER_BOUND('',#2357,.T.);
#1393=FACE_OUTER_BOUND('',#2358,.T.);
#1394=FACE_OUTER_BOUND('',#2359,.T.);
#1395=FACE_OUTER_BOUND('',#2360,.T.);
#1396=FACE_OUTER_BOUND('',#2361,.T.);
#1397=FACE_OUTER_BOUND('',#2362,.T.);
#1398=FACE_OUTER_BOUND('',#2363,.T.);
#1399=FACE_OUTER_BOUND('',#2364,.T.);
#1400=FACE_OUTER_BOUND('',#2365,.T.);
#1401=FACE_OUTER_BOUND('',#2366,.T.);
#1402=FACE_OUTER_BOUND('',#2367,.T.);
#1403=FACE_OUTER_BOUND('',#2368,.T.);
#1404=FACE_OUTER_BOUND('',#2369,.T.);
#1405=FACE_OUTER_BOUND('',#2370,.T.);
#1406=FACE_OUTER_BOUND('',#2371,.T.);
#1407=FACE_OUTER_BOUND('',#2372,.T.);
#1408=FACE_OUTER_BOUND('',#2373,.T.);
#1409=FACE_OUTER_BOUND('',#2374,.T.);
#1410=FACE_OUTER_BOUND('',#2375,.T.);
#1411=FACE_OUTER_BOUND('',#2376,.T.);
#1412=FACE_OUTER_BOUND('',#2377,.T.);
#1413=FACE_OUTER_BOUND('',#2378,.T.);
#1414=FACE_OUTER_BOUND('',#2379,.T.);
#1415=FACE_OUTER_BOUND('',#2380,.T.);
#1416=FACE_OUTER_BOUND('',#2381,.T.);
#1417=FACE_OUTER_BOUND('',#2382,.T.);
#1418=FACE_OUTER_BOUND('',#2383,.T.);
#1419=FACE_OUTER_BOUND('',#2384,.T.);
#1420=FACE_OUTER_BOUND('',#2385,.T.);
#1421=FACE_OUTER_BOUND('',#2386,.T.);
#1422=FACE_OUTER_BOUND('',#2387,.T.);
#1423=FACE_OUTER_BOUND('',#2388,.T.);
#1424=FACE_OUTER_BOUND('',#2389,.T.);
#1425=FACE_OUTER_BOUND('',#2390,.T.);
#1426=FACE_OUTER_BOUND('',#2392,.T.);
#1427=FACE_OUTER_BOUND('',#2393,.T.);
#1428=FACE_OUTER_BOUND('',#2394,.T.);
#1429=FACE_OUTER_BOUND('',#2396,.T.);
#1430=FACE_OUTER_BOUND('',#2397,.T.);
#1431=FACE_OUTER_BOUND('',#2398,.T.);
#1432=FACE_OUTER_BOUND('',#2399,.T.);
#1433=FACE_OUTER_BOUND('',#2400,.T.);
#1434=FACE_OUTER_BOUND('',#2401,.T.);
#1435=FACE_OUTER_BOUND('',#2402,.T.);
#1436=FACE_OUTER_BOUND('',#2403,.T.);
#1437=FACE_OUTER_BOUND('',#2404,.T.);
#1438=FACE_OUTER_BOUND('',#2405,.T.);
#1439=FACE_OUTER_BOUND('',#2406,.T.);
#1440=FACE_OUTER_BOUND('',#2407,.T.);
#1441=FACE_OUTER_BOUND('',#2408,.T.);
#1442=FACE_OUTER_BOUND('',#2409,.T.);
#1443=FACE_OUTER_BOUND('',#2410,.T.);
#1444=FACE_OUTER_BOUND('',#2411,.T.);
#1445=FACE_OUTER_BOUND('',#2412,.T.);
#1446=FACE_OUTER_BOUND('',#2413,.T.);
#1447=FACE_OUTER_BOUND('',#2414,.T.);
#1448=FACE_OUTER_BOUND('',#2415,.T.);
#1449=FACE_OUTER_BOUND('',#2416,.T.);
#1450=FACE_OUTER_BOUND('',#2417,.T.);
#1451=FACE_OUTER_BOUND('',#2418,.T.);
#1452=FACE_OUTER_BOUND('',#2419,.T.);
#1453=FACE_OUTER_BOUND('',#2420,.T.);
#1454=FACE_OUTER_BOUND('',#2421,.T.);
#1455=FACE_OUTER_BOUND('',#2422,.T.);
#1456=FACE_OUTER_BOUND('',#2423,.T.);
#1457=FACE_OUTER_BOUND('',#2425,.T.);
#1458=FACE_OUTER_BOUND('',#2426,.T.);
#1459=FACE_OUTER_BOUND('',#2427,.T.);
#1460=FACE_OUTER_BOUND('',#2428,.T.);
#1461=FACE_OUTER_BOUND('',#2429,.T.);
#1462=FACE_OUTER_BOUND('',#2430,.T.);
#1463=FACE_OUTER_BOUND('',#2431,.T.);
#1464=FACE_OUTER_BOUND('',#2432,.T.);
#1465=FACE_OUTER_BOUND('',#2433,.T.);
#1466=FACE_OUTER_BOUND('',#2434,.T.);
#1467=FACE_OUTER_BOUND('',#2435,.T.);
#1468=FACE_OUTER_BOUND('',#2436,.T.);
#1469=FACE_OUTER_BOUND('',#2437,.T.);
#1470=FACE_OUTER_BOUND('',#2438,.T.);
#1471=FACE_OUTER_BOUND('',#2439,.T.);
#1472=FACE_OUTER_BOUND('',#2440,.T.);
#1473=FACE_OUTER_BOUND('',#2441,.T.);
#1474=FACE_OUTER_BOUND('',#2442,.T.);
#1475=FACE_OUTER_BOUND('',#2443,.T.);
#1476=FACE_OUTER_BOUND('',#2444,.T.);
#1477=FACE_OUTER_BOUND('',#2445,.T.);
#1478=FACE_OUTER_BOUND('',#2446,.T.);
#1479=FACE_OUTER_BOUND('',#2447,.T.);
#1480=FACE_OUTER_BOUND('',#2448,.T.);
#1481=FACE_OUTER_BOUND('',#2449,.T.);
#1482=FACE_OUTER_BOUND('',#2450,.T.);
#1483=FACE_OUTER_BOUND('',#2451,.T.);
#1484=FACE_OUTER_BOUND('',#2452,.T.);
#1485=FACE_OUTER_BOUND('',#2453,.T.);
#1486=FACE_OUTER_BOUND('',#2454,.T.);
#1487=FACE_OUTER_BOUND('',#2455,.T.);
#1488=FACE_OUTER_BOUND('',#2456,.T.);
#1489=FACE_OUTER_BOUND('',#2457,.T.);
#1490=FACE_OUTER_BOUND('',#2458,.T.);
#1491=FACE_OUTER_BOUND('',#2459,.T.);
#1492=FACE_OUTER_BOUND('',#2460,.T.);
#1493=FACE_OUTER_BOUND('',#2461,.T.);
#1494=FACE_OUTER_BOUND('',#2462,.T.);
#1495=FACE_OUTER_BOUND('',#2463,.T.);
#1496=FACE_OUTER_BOUND('',#2464,.T.);
#1497=FACE_OUTER_BOUND('',#2465,.T.);
#1498=FACE_OUTER_BOUND('',#2466,.T.);
#1499=FACE_OUTER_BOUND('',#2467,.T.);
#1500=FACE_OUTER_BOUND('',#2468,.T.);
#1501=FACE_OUTER_BOUND('',#2469,.T.);
#1502=FACE_OUTER_BOUND('',#2470,.T.);
#1503=FACE_OUTER_BOUND('',#2471,.T.);
#1504=FACE_OUTER_BOUND('',#2472,.T.);
#1505=FACE_OUTER_BOUND('',#2473,.T.);
#1506=FACE_OUTER_BOUND('',#2474,.T.);
#1507=FACE_OUTER_BOUND('',#2475,.T.);
#1508=FACE_OUTER_BOUND('',#2476,.T.);
#1509=FACE_OUTER_BOUND('',#2477,.T.);
#1510=FACE_OUTER_BOUND('',#2478,.T.);
#1511=FACE_OUTER_BOUND('',#2479,.T.);
#1512=FACE_OUTER_BOUND('',#2480,.T.);
#1513=FACE_OUTER_BOUND('',#2481,.T.);
#1514=FACE_OUTER_BOUND('',#2482,.T.);
#1515=FACE_OUTER_BOUND('',#2483,.T.);
#1516=FACE_OUTER_BOUND('',#2484,.T.);
#1517=FACE_OUTER_BOUND('',#2485,.T.);
#1518=FACE_OUTER_BOUND('',#2486,.T.);
#1519=FACE_OUTER_BOUND('',#2487,.T.);
#1520=FACE_OUTER_BOUND('',#2488,.T.);
#1521=FACE_OUTER_BOUND('',#2489,.T.);
#1522=FACE_OUTER_BOUND('',#2490,.T.);
#1523=FACE_OUTER_BOUND('',#2491,.T.);
#1524=FACE_OUTER_BOUND('',#2492,.T.);
#1525=FACE_OUTER_BOUND('',#2493,.T.);
#1526=FACE_OUTER_BOUND('',#2494,.T.);
#1527=FACE_OUTER_BOUND('',#2495,.T.);
#1528=FACE_OUTER_BOUND('',#2496,.T.);
#1529=FACE_OUTER_BOUND('',#2497,.T.);
#1530=FACE_OUTER_BOUND('',#2498,.T.);
#1531=FACE_OUTER_BOUND('',#2499,.T.);
#1532=FACE_OUTER_BOUND('',#2500,.T.);
#1533=FACE_OUTER_BOUND('',#2501,.T.);
#1534=FACE_OUTER_BOUND('',#2502,.T.);
#1535=FACE_OUTER_BOUND('',#2503,.T.);
#1536=FACE_OUTER_BOUND('',#2504,.T.);
#1537=FACE_OUTER_BOUND('',#2505,.T.);
#1538=FACE_OUTER_BOUND('',#2506,.T.);
#1539=FACE_OUTER_BOUND('',#2507,.T.);
#1540=FACE_OUTER_BOUND('',#2508,.T.);
#1541=FACE_OUTER_BOUND('',#2509,.T.);
#1542=FACE_OUTER_BOUND('',#2510,.T.);
#1543=FACE_OUTER_BOUND('',#2511,.T.);
#1544=FACE_OUTER_BOUND('',#2512,.T.);
#1545=FACE_OUTER_BOUND('',#2513,.T.);
#1546=FACE_OUTER_BOUND('',#2514,.T.);
#1547=FACE_OUTER_BOUND('',#2516,.T.);
#1548=FACE_OUTER_BOUND('',#2518,.T.);
#1549=FACE_OUTER_BOUND('',#2519,.T.);
#1550=FACE_OUTER_BOUND('',#2520,.T.);
#1551=FACE_OUTER_BOUND('',#2521,.T.);
#1552=FACE_OUTER_BOUND('',#2522,.T.);
#1553=FACE_OUTER_BOUND('',#2523,.T.);
#1554=FACE_OUTER_BOUND('',#2524,.T.);
#1555=FACE_OUTER_BOUND('',#2525,.T.);
#1556=FACE_OUTER_BOUND('',#2526,.T.);
#1557=FACE_OUTER_BOUND('',#2527,.T.);
#1558=FACE_OUTER_BOUND('',#2528,.T.);
#1559=FACE_OUTER_BOUND('',#2529,.T.);
#1560=FACE_OUTER_BOUND('',#2530,.T.);
#1561=FACE_OUTER_BOUND('',#2531,.T.);
#1562=FACE_OUTER_BOUND('',#2532,.T.);
#1563=FACE_OUTER_BOUND('',#2533,.T.);
#1564=FACE_OUTER_BOUND('',#2534,.T.);
#1565=FACE_OUTER_BOUND('',#2535,.T.);
#1566=FACE_OUTER_BOUND('',#2536,.T.);
#1567=FACE_OUTER_BOUND('',#2537,.T.);
#1568=FACE_OUTER_BOUND('',#2538,.T.);
#1569=FACE_OUTER_BOUND('',#2539,.T.);
#1570=FACE_OUTER_BOUND('',#2540,.T.);
#1571=FACE_OUTER_BOUND('',#2541,.T.);
#1572=FACE_OUTER_BOUND('',#2542,.T.);
#1573=FACE_OUTER_BOUND('',#2543,.T.);
#1574=FACE_OUTER_BOUND('',#2544,.T.);
#1575=FACE_OUTER_BOUND('',#2545,.T.);
#1576=FACE_OUTER_BOUND('',#2546,.T.);
#1577=FACE_OUTER_BOUND('',#2547,.T.);
#1578=FACE_OUTER_BOUND('',#2548,.T.);
#1579=FACE_OUTER_BOUND('',#2549,.T.);
#1580=FACE_OUTER_BOUND('',#2550,.T.);
#1581=FACE_OUTER_BOUND('',#2551,.T.);
#1582=FACE_OUTER_BOUND('',#2552,.T.);
#1583=FACE_OUTER_BOUND('',#2553,.T.);
#1584=FACE_OUTER_BOUND('',#2554,.T.);
#1585=FACE_OUTER_BOUND('',#2555,.T.);
#1586=FACE_OUTER_BOUND('',#2556,.T.);
#1587=FACE_OUTER_BOUND('',#2557,.T.);
#1588=FACE_OUTER_BOUND('',#2558,.T.);
#1589=FACE_OUTER_BOUND('',#2559,.T.);
#1590=FACE_OUTER_BOUND('',#2560,.T.);
#1591=FACE_OUTER_BOUND('',#2561,.T.);
#1592=FACE_OUTER_BOUND('',#2562,.T.);
#1593=FACE_OUTER_BOUND('',#2563,.T.);
#1594=FACE_OUTER_BOUND('',#2564,.T.);
#1595=FACE_OUTER_BOUND('',#2565,.T.);
#1596=FACE_OUTER_BOUND('',#2566,.T.);
#1597=FACE_OUTER_BOUND('',#2567,.T.);
#1598=FACE_OUTER_BOUND('',#2568,.T.);
#1599=FACE_OUTER_BOUND('',#2569,.T.);
#1600=FACE_OUTER_BOUND('',#2570,.T.);
#1601=FACE_OUTER_BOUND('',#2571,.T.);
#1602=FACE_OUTER_BOUND('',#2572,.T.);
#1603=FACE_OUTER_BOUND('',#2573,.T.);
#1604=FACE_OUTER_BOUND('',#2574,.T.);
#1605=FACE_OUTER_BOUND('',#2575,.T.);
#1606=FACE_OUTER_BOUND('',#2576,.T.);
#1607=FACE_OUTER_BOUND('',#2577,.T.);
#1608=FACE_OUTER_BOUND('',#2578,.T.);
#1609=FACE_OUTER_BOUND('',#2579,.T.);
#1610=FACE_OUTER_BOUND('',#2580,.T.);
#1611=FACE_OUTER_BOUND('',#2581,.T.);
#1612=FACE_OUTER_BOUND('',#2582,.T.);
#1613=FACE_OUTER_BOUND('',#2584,.T.);
#1614=FACE_OUTER_BOUND('',#2585,.T.);
#1615=FACE_OUTER_BOUND('',#2586,.T.);
#1616=FACE_OUTER_BOUND('',#2587,.T.);
#1617=FACE_OUTER_BOUND('',#2588,.T.);
#1618=FACE_OUTER_BOUND('',#2590,.T.);
#1619=FACE_OUTER_BOUND('',#2591,.T.);
#1620=FACE_OUTER_BOUND('',#2592,.T.);
#1621=FACE_OUTER_BOUND('',#2593,.T.);
#1622=FACE_OUTER_BOUND('',#2594,.T.);
#1623=FACE_OUTER_BOUND('',#2596,.T.);
#1624=FACE_OUTER_BOUND('',#2597,.T.);
#1625=FACE_OUTER_BOUND('',#2598,.T.);
#1626=FACE_OUTER_BOUND('',#2599,.T.);
#1627=FACE_OUTER_BOUND('',#2600,.T.);
#1628=FACE_OUTER_BOUND('',#2601,.T.);
#1629=FACE_OUTER_BOUND('',#2602,.T.);
#1630=FACE_OUTER_BOUND('',#2603,.T.);
#1631=FACE_OUTER_BOUND('',#2604,.T.);
#2269=EDGE_LOOP('',(#11815,#11816,#11817,#11818));
#2270=EDGE_LOOP('',(#11819,#11820,#11821,#11822));
#2271=EDGE_LOOP('',(#11823,#11824,#11825,#11826));
#2272=EDGE_LOOP('',(#11827,#11828,#11829,#11830));
#2273=EDGE_LOOP('',(#11831,#11832,#11833,#11834));
#2274=EDGE_LOOP('',(#11835,#11836,#11837,#11838));
#2275=EDGE_LOOP('',(#11839,#11840,#11841,#11842));
#2276=EDGE_LOOP('',(#11843,#11844,#11845,#11846));
#2277=EDGE_LOOP('',(#11847,#11848,#11849,#11850));
#2278=EDGE_LOOP('',(#11851,#11852,#11853,#11854));
#2279=EDGE_LOOP('',(#11855,#11856,#11857,#11858));
#2280=EDGE_LOOP('',(#11859,#11860,#11861,#11862));
#2281=EDGE_LOOP('',(#11863,#11864,#11865,#11866));
#2282=EDGE_LOOP('',(#11867,#11868,#11869,#11870));
#2283=EDGE_LOOP('',(#11871,#11872,#11873,#11874));
#2284=EDGE_LOOP('',(#11875,#11876,#11877,#11878));
#2285=EDGE_LOOP('',(#11879,#11880,#11881,#11882,#11883,#11884,#11885,#11886,
#11887,#11888,#11889,#11890,#11891,#11892,#11893,#11894,#11895,#11896,#11897,
#11898,#11899,#11900,#11901,#11902,#11903,#11904,#11905,#11906,#11907,#11908,
#11909,#11910,#11911,#11912,#11913,#11914,#11915,#11916,#11917,#11918,#11919,
#11920,#11921,#11922,#11923,#11924,#11925,#11926,#11927,#11928,#11929,#11930,
#11931,#11932,#11933,#11934,#11935,#11936,#11937,#11938,#11939,#11940,#11941,
#11942,#11943,#11944,#11945,#11946,#11947,#11948,#11949,#11950,#11951,#11952,
#11953,#11954,#11955,#11956,#11957,#11958,#11959,#11960,#11961,#11962,#11963,
#11964,#11965,#11966,#11967,#11968,#11969,#11970,#11971,#11972,#11973,#11974));
#2286=EDGE_LOOP('',(#11975,#11976,#11977,#11978));
#2287=EDGE_LOOP('',(#11979,#11980,#11981,#11982));
#2288=EDGE_LOOP('',(#11983,#11984,#11985,#11986));
#2289=EDGE_LOOP('',(#11987,#11988,#11989,#11990));
#2290=EDGE_LOOP('',(#11991,#11992,#11993,#11994));
#2291=EDGE_LOOP('',(#11995,#11996,#11997,#11998));
#2292=EDGE_LOOP('',(#11999,#12000,#12001,#12002));
#2293=EDGE_LOOP('',(#12003,#12004,#12005,#12006));
#2294=EDGE_LOOP('',(#12007,#12008,#12009,#12010));
#2295=EDGE_LOOP('',(#12011,#12012,#12013,#12014));
#2296=EDGE_LOOP('',(#12015,#12016,#12017,#12018));
#2297=EDGE_LOOP('',(#12019,#12020,#12021,#12022));
#2298=EDGE_LOOP('',(#12023,#12024,#12025,#12026));
#2299=EDGE_LOOP('',(#12027,#12028,#12029,#12030));
#2300=EDGE_LOOP('',(#12031,#12032,#12033,#12034));
#2301=EDGE_LOOP('',(#12035,#12036,#12037,#12038));
#2302=EDGE_LOOP('',(#12039,#12040,#12041,#12042,#12043));
#2303=EDGE_LOOP('',(#12044,#12045,#12046,#12047,#12048));
#2304=EDGE_LOOP('',(#12049));
#2305=EDGE_LOOP('',(#12050));
#2306=EDGE_LOOP('',(#12051,#12052,#12053,#12054,#12055));
#2307=EDGE_LOOP('',(#12056,#12057,#12058,#12059));
#2308=EDGE_LOOP('',(#12060,#12061,#12062,#12063,#12064));
#2309=EDGE_LOOP('',(#12065,#12066,#12067,#12068,#12069));
#2310=EDGE_LOOP('',(#12070,#12071,#12072,#12073,#12074));
#2311=EDGE_LOOP('',(#12075,#12076,#12077,#12078));
#2312=EDGE_LOOP('',(#12079,#12080,#12081,#12082,#12083));
#2313=EDGE_LOOP('',(#12084,#12085,#12086,#12087,#12088));
#2314=EDGE_LOOP('',(#12089,#12090,#12091,#12092,#12093));
#2315=EDGE_LOOP('',(#12094,#12095,#12096,#12097));
#2316=EDGE_LOOP('',(#12098,#12099,#12100,#12101,#12102));
#2317=EDGE_LOOP('',(#12103,#12104,#12105,#12106,#12107));
#2318=EDGE_LOOP('',(#12108,#12109,#12110,#12111,#12112));
#2319=EDGE_LOOP('',(#12113,#12114,#12115,#12116));
#2320=EDGE_LOOP('',(#12117,#12118,#12119,#12120,#12121));
#2321=EDGE_LOOP('',(#12122,#12123,#12124,#12125,#12126));
#2322=EDGE_LOOP('',(#12127,#12128,#12129,#12130,#12131));
#2323=EDGE_LOOP('',(#12132,#12133,#12134,#12135));
#2324=EDGE_LOOP('',(#12136,#12137,#12138,#12139,#12140));
#2325=EDGE_LOOP('',(#12141,#12142,#12143,#12144,#12145));
#2326=EDGE_LOOP('',(#12146,#12147,#12148,#12149,#12150));
#2327=EDGE_LOOP('',(#12151,#12152,#12153,#12154));
#2328=EDGE_LOOP('',(#12155,#12156,#12157,#12158,#12159));
#2329=EDGE_LOOP('',(#12160,#12161,#12162,#12163,#12164));
#2330=EDGE_LOOP('',(#12165,#12166,#12167,#12168,#12169));
#2331=EDGE_LOOP('',(#12170,#12171,#12172,#12173));
#2332=EDGE_LOOP('',(#12174,#12175,#12176,#12177,#12178));
#2333=EDGE_LOOP('',(#12179,#12180,#12181,#12182,#12183));
#2334=EDGE_LOOP('',(#12184,#12185,#12186,#12187));
#2335=EDGE_LOOP('',(#12188,#12189,#12190,#12191,#12192));
#2336=EDGE_LOOP('',(#12193,#12194,#12195,#12196,#12197));
#2337=EDGE_LOOP('',(#12198,#12199,#12200,#12201,#12202));
#2338=EDGE_LOOP('',(#12203,#12204,#12205,#12206));
#2339=EDGE_LOOP('',(#12207,#12208,#12209,#12210,#12211));
#2340=EDGE_LOOP('',(#12212,#12213,#12214,#12215,#12216));
#2341=EDGE_LOOP('',(#12217,#12218,#12219,#12220,#12221));
#2342=EDGE_LOOP('',(#12222,#12223,#12224,#12225));
#2343=EDGE_LOOP('',(#12226,#12227,#12228,#12229,#12230));
#2344=EDGE_LOOP('',(#12231,#12232,#12233,#12234,#12235));
#2345=EDGE_LOOP('',(#12236,#12237,#12238,#12239,#12240));
#2346=EDGE_LOOP('',(#12241,#12242,#12243,#12244));
#2347=EDGE_LOOP('',(#12245,#12246,#12247,#12248,#12249));
#2348=EDGE_LOOP('',(#12250,#12251,#12252,#12253,#12254));
#2349=EDGE_LOOP('',(#12255,#12256,#12257,#12258,#12259));
#2350=EDGE_LOOP('',(#12260,#12261,#12262,#12263));
#2351=EDGE_LOOP('',(#12264,#12265,#12266,#12267,#12268));
#2352=EDGE_LOOP('',(#12269,#12270,#12271,#12272,#12273));
#2353=EDGE_LOOP('',(#12274,#12275,#12276,#12277));
#2354=EDGE_LOOP('',(#12278,#12279,#12280,#12281));
#2355=EDGE_LOOP('',(#12282,#12283,#12284,#12285,#12286,#12287,#12288,#12289,
#12290,#12291));
#2356=EDGE_LOOP('',(#12292,#12293,#12294,#12295));
#2357=EDGE_LOOP('',(#12296,#12297,#12298,#12299));
#2358=EDGE_LOOP('',(#12300,#12301,#12302,#12303,#12304,#12305,#12306,#12307,
#12308));
#2359=EDGE_LOOP('',(#12309,#12310,#12311,#12312));
#2360=EDGE_LOOP('',(#12313,#12314,#12315,#12316));
#2361=EDGE_LOOP('',(#12317,#12318,#12319,#12320,#12321,#12322,#12323,#12324,
#12325));
#2362=EDGE_LOOP('',(#12326,#12327,#12328,#12329));
#2363=EDGE_LOOP('',(#12330,#12331,#12332,#12333));
#2364=EDGE_LOOP('',(#12334,#12335,#12336,#12337,#12338,#12339,#12340,#12341,
#12342));
#2365=EDGE_LOOP('',(#12343,#12344,#12345,#12346));
#2366=EDGE_LOOP('',(#12347,#12348,#12349,#12350));
#2367=EDGE_LOOP('',(#12351,#12352,#12353,#12354,#12355,#12356,#12357,#12358,
#12359));
#2368=EDGE_LOOP('',(#12360,#12361,#12362,#12363));
#2369=EDGE_LOOP('',(#12364,#12365,#12366,#12367));
#2370=EDGE_LOOP('',(#12368,#12369,#12370,#12371,#12372,#12373,#12374,#12375,
#12376));
#2371=EDGE_LOOP('',(#12377,#12378,#12379,#12380));
#2372=EDGE_LOOP('',(#12381,#12382,#12383,#12384));
#2373=EDGE_LOOP('',(#12385,#12386,#12387,#12388,#12389,#12390,#12391,#12392,
#12393));
#2374=EDGE_LOOP('',(#12394,#12395,#12396,#12397));
#2375=EDGE_LOOP('',(#12398,#12399,#12400,#12401));
#2376=EDGE_LOOP('',(#12402,#12403,#12404,#12405,#12406,#12407,#12408,#12409,
#12410));
#2377=EDGE_LOOP('',(#12411,#12412,#12413,#12414));
#2378=EDGE_LOOP('',(#12415,#12416,#12417,#12418));
#2379=EDGE_LOOP('',(#12419,#12420,#12421,#12422,#12423,#12424,#12425,#12426,
#12427));
#2380=EDGE_LOOP('',(#12428,#12429,#12430,#12431));
#2381=EDGE_LOOP('',(#12432,#12433,#12434,#12435));
#2382=EDGE_LOOP('',(#12436,#12437,#12438,#12439,#12440,#12441,#12442,#12443,
#12444));
#2383=EDGE_LOOP('',(#12445,#12446,#12447,#12448));
#2384=EDGE_LOOP('',(#12449,#12450,#12451,#12452));
#2385=EDGE_LOOP('',(#12453,#12454,#12455,#12456,#12457,#12458,#12459,#12460,
#12461));
#2386=EDGE_LOOP('',(#12462,#12463,#12464,#12465));
#2387=EDGE_LOOP('',(#12466,#12467,#12468,#12469));
#2388=EDGE_LOOP('',(#12470,#12471,#12472,#12473,#12474,#12475,#12476,#12477,
#12478,#12479));
#2389=EDGE_LOOP('',(#12480,#12481,#12482,#12483));
#2390=EDGE_LOOP('',(#12484));
#2391=EDGE_LOOP('',(#12485));
#2392=EDGE_LOOP('',(#12486,#12487,#12488,#12489));
#2393=EDGE_LOOP('',(#12490,#12491,#12492,#12493));
#2394=EDGE_LOOP('',(#12494));
#2395=EDGE_LOOP('',(#12495));
#2396=EDGE_LOOP('',(#12496,#12497,#12498,#12499));
#2397=EDGE_LOOP('',(#12500,#12501,#12502,#12503,#12504));
#2398=EDGE_LOOP('',(#12505,#12506,#12507,#12508,#12509,#12510));
#2399=EDGE_LOOP('',(#12511,#12512,#12513,#12514,#12515,#12516));
#2400=EDGE_LOOP('',(#12517,#12518,#12519,#12520,#12521,#12522,#12523,#12524));
#2401=EDGE_LOOP('',(#12525,#12526,#12527,#12528,#12529));
#2402=EDGE_LOOP('',(#12530,#12531,#12532,#12533,#12534,#12535));
#2403=EDGE_LOOP('',(#12536,#12537,#12538,#12539,#12540));
#2404=EDGE_LOOP('',(#12541,#12542,#12543,#12544,#12545,#12546));
#2405=EDGE_LOOP('',(#12547,#12548,#12549,#12550,#12551,#12552,#12553,#12554));
#2406=EDGE_LOOP('',(#12555,#12556,#12557,#12558,#12559));
#2407=EDGE_LOOP('',(#12560,#12561,#12562,#12563,#12564,#12565));
#2408=EDGE_LOOP('',(#12566,#12567,#12568,#12569,#12570));
#2409=EDGE_LOOP('',(#12571,#12572,#12573,#12574,#12575,#12576));
#2410=EDGE_LOOP('',(#12577,#12578,#12579,#12580,#12581,#12582,#12583,#12584));
#2411=EDGE_LOOP('',(#12585,#12586,#12587,#12588,#12589));
#2412=EDGE_LOOP('',(#12590,#12591,#12592,#12593,#12594,#12595));
#2413=EDGE_LOOP('',(#12596,#12597,#12598,#12599,#12600));
#2414=EDGE_LOOP('',(#12601,#12602,#12603,#12604,#12605,#12606));
#2415=EDGE_LOOP('',(#12607,#12608,#12609,#12610,#12611,#12612,#12613,#12614));
#2416=EDGE_LOOP('',(#12615,#12616,#12617,#12618,#12619));
#2417=EDGE_LOOP('',(#12620,#12621,#12622,#12623,#12624,#12625));
#2418=EDGE_LOOP('',(#12626,#12627,#12628,#12629,#12630));
#2419=EDGE_LOOP('',(#12631,#12632,#12633,#12634,#12635,#12636));
#2420=EDGE_LOOP('',(#12637,#12638,#12639,#12640,#12641,#12642,#12643,#12644));
#2421=EDGE_LOOP('',(#12645,#12646,#12647,#12648,#12649));
#2422=EDGE_LOOP('',(#12650,#12651,#12652,#12653,#12654,#12655));
#2423=EDGE_LOOP('',(#12656,#12657,#12658,#12659,#12660,#12661,#12662,#12663,
#12664,#12665,#12666,#12667,#12668,#12669,#12670,#12671,#12672,#12673,#12674,
#12675,#12676,#12677,#12678,#12679));
#2424=EDGE_LOOP('',(#12680));
#2425=EDGE_LOOP('',(#12681,#12682,#12683,#12684,#12685,#12686));
#2426=EDGE_LOOP('',(#12687,#12688,#12689,#12690,#12691));
#2427=EDGE_LOOP('',(#12692,#12693,#12694,#12695,#12696,#12697,#12698,#12699));
#2428=EDGE_LOOP('',(#12700,#12701,#12702,#12703,#12704,#12705,#12706,#12707));
#2429=EDGE_LOOP('',(#12708,#12709,#12710,#12711,#12712));
#2430=EDGE_LOOP('',(#12713,#12714,#12715,#12716,#12717,#12718,#12719,#12720));
#2431=EDGE_LOOP('',(#12721,#12722,#12723,#12724,#12725));
#2432=EDGE_LOOP('',(#12726,#12727,#12728,#12729,#12730,#12731));
#2433=EDGE_LOOP('',(#12732,#12733,#12734,#12735,#12736,#12737));
#2434=EDGE_LOOP('',(#12738,#12739,#12740,#12741,#12742));
#2435=EDGE_LOOP('',(#12743,#12744,#12745,#12746,#12747,#12748,#12749,#12750));
#2436=EDGE_LOOP('',(#12751,#12752,#12753,#12754,#12755));
#2437=EDGE_LOOP('',(#12756,#12757,#12758,#12759,#12760,#12761));
#2438=EDGE_LOOP('',(#12762,#12763,#12764,#12765,#12766,#12767));
#2439=EDGE_LOOP('',(#12768,#12769,#12770,#12771,#12772));
#2440=EDGE_LOOP('',(#12773,#12774,#12775,#12776,#12777,#12778,#12779,#12780));
#2441=EDGE_LOOP('',(#12781,#12782,#12783,#12784,#12785));
#2442=EDGE_LOOP('',(#12786,#12787,#12788,#12789,#12790,#12791));
#2443=EDGE_LOOP('',(#12792,#12793,#12794,#12795,#12796,#12797));
#2444=EDGE_LOOP('',(#12798,#12799,#12800,#12801,#12802));
#2445=EDGE_LOOP('',(#12803,#12804,#12805,#12806,#12807,#12808,#12809,#12810));
#2446=EDGE_LOOP('',(#12811,#12812,#12813,#12814,#12815));
#2447=EDGE_LOOP('',(#12816,#12817,#12818,#12819,#12820,#12821));
#2448=EDGE_LOOP('',(#12822,#12823,#12824,#12825,#12826,#12827));
#2449=EDGE_LOOP('',(#12828,#12829,#12830,#12831,#12832));
#2450=EDGE_LOOP('',(#12833,#12834,#12835,#12836,#12837,#12838,#12839,#12840));
#2451=EDGE_LOOP('',(#12841,#12842,#12843,#12844,#12845));
#2452=EDGE_LOOP('',(#12846,#12847,#12848,#12849,#12850,#12851));
#2453=EDGE_LOOP('',(#12852,#12853,#12854,#12855,#12856,#12857));
#2454=EDGE_LOOP('',(#12858,#12859,#12860,#12861,#12862));
#2455=EDGE_LOOP('',(#12863,#12864,#12865,#12866,#12867,#12868,#12869,#12870));
#2456=EDGE_LOOP('',(#12871,#12872,#12873,#12874,#12875,#12876));
#2457=EDGE_LOOP('',(#12877,#12878,#12879,#12880,#12881,#12882,#12883,#12884));
#2458=EDGE_LOOP('',(#12885,#12886,#12887,#12888,#12889));
#2459=EDGE_LOOP('',(#12890,#12891,#12892,#12893,#12894,#12895));
#2460=EDGE_LOOP('',(#12896,#12897,#12898,#12899,#12900));
#2461=EDGE_LOOP('',(#12901,#12902,#12903,#12904,#12905));
#2462=EDGE_LOOP('',(#12906,#12907,#12908,#12909,#12910,#12911,#12912,#12913));
#2463=EDGE_LOOP('',(#12914,#12915,#12916,#12917,#12918));
#2464=EDGE_LOOP('',(#12919,#12920,#12921,#12922,#12923,#12924,#12925,#12926,
#12927,#12928,#12929,#12930,#12931,#12932,#12933,#12934,#12935,#12936,#12937,
#12938,#12939,#12940,#12941,#12942,#12943,#12944,#12945,#12946,#12947,#12948,
#12949,#12950,#12951,#12952,#12953,#12954));
#2465=EDGE_LOOP('',(#12955,#12956,#12957,#12958,#12959));
#2466=EDGE_LOOP('',(#12960,#12961,#12962,#12963));
#2467=EDGE_LOOP('',(#12964,#12965,#12966,#12967,#12968,#12969,#12970,#12971,
#12972,#12973,#12974,#12975,#12976,#12977,#12978,#12979,#12980,#12981,#12982,
#12983,#12984,#12985,#12986,#12987,#12988,#12989,#12990,#12991,#12992,#12993,
#12994,#12995,#12996,#12997,#12998,#12999));
#2468=EDGE_LOOP('',(#13000,#13001));
#2469=EDGE_LOOP('',(#13002,#13003,#13004,#13005,#13006,#13007,#13008,#13009));
#2470=EDGE_LOOP('',(#13010,#13011,#13012,#13013,#13014));
#2471=EDGE_LOOP('',(#13015,#13016));
#2472=EDGE_LOOP('',(#13017,#13018,#13019,#13020,#13021,#13022,#13023,#13024));
#2473=EDGE_LOOP('',(#13025,#13026,#13027,#13028,#13029));
#2474=EDGE_LOOP('',(#13030,#13031,#13032,#13033,#13034));
#2475=EDGE_LOOP('',(#13035,#13036));
#2476=EDGE_LOOP('',(#13037,#13038,#13039,#13040,#13041,#13042,#13043,#13044));
#2477=EDGE_LOOP('',(#13045,#13046,#13047,#13048,#13049));
#2478=EDGE_LOOP('',(#13050,#13051,#13052,#13053,#13054));
#2479=EDGE_LOOP('',(#13055,#13056));
#2480=EDGE_LOOP('',(#13057,#13058,#13059,#13060,#13061,#13062,#13063,#13064));
#2481=EDGE_LOOP('',(#13065,#13066,#13067,#13068,#13069));
#2482=EDGE_LOOP('',(#13070,#13071,#13072,#13073,#13074));
#2483=EDGE_LOOP('',(#13075,#13076));
#2484=EDGE_LOOP('',(#13077,#13078,#13079,#13080,#13081,#13082,#13083,#13084));
#2485=EDGE_LOOP('',(#13085,#13086,#13087,#13088,#13089));
#2486=EDGE_LOOP('',(#13090,#13091,#13092,#13093,#13094));
#2487=EDGE_LOOP('',(#13095,#13096));
#2488=EDGE_LOOP('',(#13097,#13098,#13099,#13100,#13101,#13102,#13103,#13104));
#2489=EDGE_LOOP('',(#13105,#13106,#13107,#13108,#13109));
#2490=EDGE_LOOP('',(#13110,#13111,#13112,#13113,#13114));
#2491=EDGE_LOOP('',(#13115,#13116));
#2492=EDGE_LOOP('',(#13117,#13118,#13119,#13120,#13121,#13122,#13123,#13124));
#2493=EDGE_LOOP('',(#13125,#13126,#13127,#13128,#13129));
#2494=EDGE_LOOP('',(#13130,#13131,#13132,#13133,#13134));
#2495=EDGE_LOOP('',(#13135,#13136));
#2496=EDGE_LOOP('',(#13137,#13138,#13139,#13140,#13141,#13142,#13143,#13144));
#2497=EDGE_LOOP('',(#13145,#13146,#13147,#13148,#13149));
#2498=EDGE_LOOP('',(#13150,#13151,#13152,#13153,#13154));
#2499=EDGE_LOOP('',(#13155,#13156));
#2500=EDGE_LOOP('',(#13157,#13158,#13159,#13160,#13161,#13162,#13163,#13164));
#2501=EDGE_LOOP('',(#13165,#13166,#13167,#13168,#13169));
#2502=EDGE_LOOP('',(#13170,#13171,#13172,#13173,#13174));
#2503=EDGE_LOOP('',(#13175,#13176));
#2504=EDGE_LOOP('',(#13177,#13178,#13179,#13180,#13181,#13182,#13183,#13184));
#2505=EDGE_LOOP('',(#13185,#13186,#13187,#13188,#13189));
#2506=EDGE_LOOP('',(#13190,#13191,#13192,#13193,#13194));
#2507=EDGE_LOOP('',(#13195,#13196));
#2508=EDGE_LOOP('',(#13197,#13198,#13199,#13200,#13201));
#2509=EDGE_LOOP('',(#13202,#13203,#13204,#13205,#13206));
#2510=EDGE_LOOP('',(#13207,#13208));
#2511=EDGE_LOOP('',(#13209,#13210,#13211,#13212,#13213));
#2512=EDGE_LOOP('',(#13214,#13215,#13216,#13217,#13218));
#2513=EDGE_LOOP('',(#13219,#13220,#13221,#13222));
#2514=EDGE_LOOP('',(#13223));
#2515=EDGE_LOOP('',(#13224));
#2516=EDGE_LOOP('',(#13225));
#2517=EDGE_LOOP('',(#13226));
#2518=EDGE_LOOP('',(#13227,#13228,#13229,#13230));
#2519=EDGE_LOOP('',(#13231,#13232,#13233,#13234));
#2520=EDGE_LOOP('',(#13235,#13236,#13237,#13238));
#2521=EDGE_LOOP('',(#13239,#13240,#13241,#13242));
#2522=EDGE_LOOP('',(#13243,#13244,#13245,#13246,#13247));
#2523=EDGE_LOOP('',(#13248,#13249,#13250,#13251,#13252,#13253,#13254,#13255,
#13256));
#2524=EDGE_LOOP('',(#13257,#13258,#13259,#13260));
#2525=EDGE_LOOP('',(#13261,#13262,#13263,#13264));
#2526=EDGE_LOOP('',(#13265,#13266,#13267,#13268,#13269));
#2527=EDGE_LOOP('',(#13270,#13271,#13272,#13273,#13274,#13275,#13276,#13277));
#2528=EDGE_LOOP('',(#13278,#13279,#13280,#13281));
#2529=EDGE_LOOP('',(#13282,#13283,#13284,#13285));
#2530=EDGE_LOOP('',(#13286,#13287,#13288,#13289,#13290));
#2531=EDGE_LOOP('',(#13291,#13292,#13293,#13294,#13295,#13296,#13297,#13298));
#2532=EDGE_LOOP('',(#13299,#13300,#13301,#13302));
#2533=EDGE_LOOP('',(#13303,#13304,#13305,#13306));
#2534=EDGE_LOOP('',(#13307,#13308,#13309,#13310,#13311));
#2535=EDGE_LOOP('',(#13312,#13313,#13314,#13315,#13316,#13317,#13318,#13319));
#2536=EDGE_LOOP('',(#13320,#13321,#13322,#13323));
#2537=EDGE_LOOP('',(#13324,#13325,#13326,#13327));
#2538=EDGE_LOOP('',(#13328,#13329,#13330,#13331,#13332));
#2539=EDGE_LOOP('',(#13333,#13334,#13335,#13336,#13337,#13338,#13339,#13340));
#2540=EDGE_LOOP('',(#13341,#13342,#13343,#13344));
#2541=EDGE_LOOP('',(#13345,#13346,#13347,#13348));
#2542=EDGE_LOOP('',(#13349,#13350,#13351,#13352,#13353));
#2543=EDGE_LOOP('',(#13354,#13355,#13356,#13357,#13358,#13359,#13360,#13361));
#2544=EDGE_LOOP('',(#13362,#13363,#13364,#13365));
#2545=EDGE_LOOP('',(#13366,#13367,#13368,#13369));
#2546=EDGE_LOOP('',(#13370,#13371,#13372,#13373,#13374));
#2547=EDGE_LOOP('',(#13375,#13376,#13377,#13378,#13379,#13380,#13381,#13382));
#2548=EDGE_LOOP('',(#13383,#13384,#13385,#13386));
#2549=EDGE_LOOP('',(#13387,#13388,#13389,#13390));
#2550=EDGE_LOOP('',(#13391,#13392,#13393,#13394,#13395));
#2551=EDGE_LOOP('',(#13396,#13397,#13398,#13399,#13400,#13401,#13402,#13403));
#2552=EDGE_LOOP('',(#13404,#13405,#13406,#13407));
#2553=EDGE_LOOP('',(#13408,#13409,#13410,#13411));
#2554=EDGE_LOOP('',(#13412,#13413,#13414,#13415,#13416));
#2555=EDGE_LOOP('',(#13417,#13418,#13419,#13420,#13421,#13422,#13423,#13424));
#2556=EDGE_LOOP('',(#13425,#13426,#13427,#13428));
#2557=EDGE_LOOP('',(#13429,#13430,#13431,#13432));
#2558=EDGE_LOOP('',(#13433,#13434,#13435,#13436,#13437));
#2559=EDGE_LOOP('',(#13438,#13439,#13440,#13441,#13442,#13443,#13444,#13445));
#2560=EDGE_LOOP('',(#13446,#13447,#13448,#13449));
#2561=EDGE_LOOP('',(#13450,#13451,#13452,#13453));
#2562=EDGE_LOOP('',(#13454,#13455,#13456,#13457,#13458));
#2563=EDGE_LOOP('',(#13459,#13460,#13461,#13462,#13463,#13464,#13465,#13466));
#2564=EDGE_LOOP('',(#13467,#13468,#13469,#13470));
#2565=EDGE_LOOP('',(#13471,#13472,#13473,#13474));
#2566=EDGE_LOOP('',(#13475,#13476,#13477,#13478,#13479));
#2567=EDGE_LOOP('',(#13480,#13481,#13482,#13483,#13484,#13485,#13486,#13487));
#2568=EDGE_LOOP('',(#13488,#13489,#13490,#13491,#13492));
#2569=EDGE_LOOP('',(#13493,#13494,#13495,#13496));
#2570=EDGE_LOOP('',(#13497,#13498,#13499,#13500));
#2571=EDGE_LOOP('',(#13501,#13502,#13503,#13504));
#2572=EDGE_LOOP('',(#13505,#13506,#13507,#13508));
#2573=EDGE_LOOP('',(#13509,#13510,#13511,#13512));
#2574=EDGE_LOOP('',(#13513,#13514,#13515,#13516));
#2575=EDGE_LOOP('',(#13517,#13518,#13519,#13520,#13521,#13522,#13523,#13524,
#13525,#13526,#13527,#13528,#13529,#13530,#13531,#13532,#13533,#13534,#13535,
#13536,#13537,#13538,#13539,#13540));
#2576=EDGE_LOOP('',(#13541,#13542,#13543,#13544));
#2577=EDGE_LOOP('',(#13545,#13546,#13547,#13548));
#2578=EDGE_LOOP('',(#13549,#13550,#13551,#13552));
#2579=EDGE_LOOP('',(#13553,#13554,#13555,#13556));
#2580=EDGE_LOOP('',(#13557,#13558,#13559,#13560));
#2581=EDGE_LOOP('',(#13561,#13562,#13563,#13564));
#2582=EDGE_LOOP('',(#13565));
#2583=EDGE_LOOP('',(#13566,#13567,#13568,#13569,#13570,#13571,#13572,#13573,
#13574,#13575,#13576,#13577,#13578,#13579,#13580,#13581,#13582,#13583,#13584,
#13585,#13586,#13587,#13588,#13589,#13590,#13591,#13592,#13593,#13594,#13595,
#13596,#13597,#13598,#13599,#13600,#13601));
#2584=EDGE_LOOP('',(#13602,#13603,#13604,#13605));
#2585=EDGE_LOOP('',(#13606,#13607,#13608,#13609));
#2586=EDGE_LOOP('',(#13610,#13611,#13612,#13613));
#2587=EDGE_LOOP('',(#13614,#13615,#13616,#13617));
#2588=EDGE_LOOP('',(#13618));
#2589=EDGE_LOOP('',(#13619));
#2590=EDGE_LOOP('',(#13620,#13621,#13622,#13623));
#2591=EDGE_LOOP('',(#13624,#13625,#13626,#13627));
#2592=EDGE_LOOP('',(#13628,#13629,#13630,#13631));
#2593=EDGE_LOOP('',(#13632,#13633,#13634,#13635));
#2594=EDGE_LOOP('',(#13636));
#2595=EDGE_LOOP('',(#13637));
#2596=EDGE_LOOP('',(#13638,#13639,#13640,#13641));
#2597=EDGE_LOOP('',(#13642,#13643,#13644,#13645));
#2598=EDGE_LOOP('',(#13646,#13647,#13648,#13649));
#2599=EDGE_LOOP('',(#13650,#13651,#13652,#13653));
#2600=EDGE_LOOP('',(#13654,#13655,#13656,#13657));
#2601=EDGE_LOOP('',(#13658,#13659,#13660,#13661,#13662,#13663));
#2602=EDGE_LOOP('',(#13664,#13665,#13666,#13667));
#2603=EDGE_LOOP('',(#13668,#13669,#13670,#13671,#13672,#13673));
#2604=EDGE_LOOP('',(#13674));
#3300=CIRCLE('',#18421,3.442);
#3301=CIRCLE('',#18437,11.);
#3302=CIRCLE('',#18438,32.4);
#3303=CIRCLE('',#18439,32.4);
#3304=CIRCLE('',#18440,32.4);
#3305=CIRCLE('',#18441,32.4);
#3306=CIRCLE('',#18442,32.4);
#3307=CIRCLE('',#18443,32.4);
#3308=CIRCLE('',#18444,32.4);
#3309=CIRCLE('',#18445,32.4);
#3310=CIRCLE('',#18446,32.4);
#3311=CIRCLE('',#18447,32.4);
#3312=CIRCLE('',#18448,32.4);
#3313=CIRCLE('',#18449,32.4);
#3314=CIRCLE('',#18450,32.4);
#3315=CIRCLE('',#18451,32.4);
#3316=CIRCLE('',#18452,32.4);
#3317=CIRCLE('',#18453,32.4);
#3318=CIRCLE('',#18454,32.4);
#3319=CIRCLE('',#18455,32.4);
#3320=CIRCLE('',#18456,32.4);
#3321=CIRCLE('',#18457,32.4);
#3322=CIRCLE('',#18458,32.4);
#3323=CIRCLE('',#18459,32.4);
#3324=CIRCLE('',#18461,2.872);
#3325=CIRCLE('',#18478,9.5);
#3326=CIRCLE('',#18479,10.2572478777138);
#3327=CIRCLE('',#18480,10.2572478777138);
#3328=CIRCLE('',#18482,10.6);
#3329=CIRCLE('',#18484,8.8);
#3330=CIRCLE('',#18533,34.5);
#3331=CIRCLE('',#18534,35.);
#3332=CIRCLE('',#18536,35.);
#3333=CIRCLE('',#18538,34.5);
#3334=CIRCLE('',#18539,35.);
#3335=CIRCLE('',#18541,35.);
#3336=CIRCLE('',#18543,34.5);
#3337=CIRCLE('',#18544,35.);
#3338=CIRCLE('',#18546,35.);
#3339=CIRCLE('',#18548,34.5);
#3340=CIRCLE('',#18549,35.);
#3341=CIRCLE('',#18551,35.);
#3342=CIRCLE('',#18553,34.5);
#3343=CIRCLE('',#18554,35.);
#3344=CIRCLE('',#18556,35.);
#3345=CIRCLE('',#18558,34.5);
#3346=CIRCLE('',#18559,35.);
#3347=CIRCLE('',#18561,35.);
#3348=CIRCLE('',#18563,34.5);
#3349=CIRCLE('',#18564,35.);
#3350=CIRCLE('',#18566,35.);
#3351=CIRCLE('',#18568,34.5);
#3352=CIRCLE('',#18569,35.);
#3353=CIRCLE('',#18571,35.);
#3354=CIRCLE('',#18573,34.5);
#3355=CIRCLE('',#18574,35.);
#3356=CIRCLE('',#18576,35.);
#3357=CIRCLE('',#18578,34.5);
#3358=CIRCLE('',#18579,35.);
#3359=CIRCLE('',#18581,35.);
#3360=CIRCLE('',#18583,34.5);
#3361=CIRCLE('',#18584,35.);
#3362=CIRCLE('',#18586,35.);
#3363=CIRCLE('',#18588,34.5);
#3364=CIRCLE('',#18589,35.);
#3365=CIRCLE('',#18591,35.);
#3366=CIRCLE('',#18593,9.2);
#3367=CIRCLE('',#18594,8.7);
#3368=CIRCLE('',#18596,7.7);
#3369=CIRCLE('',#18598,9.2);
#3370=CIRCLE('',#18600,9.2);
#3371=CIRCLE('',#18601,8.7);
#3372=CIRCLE('',#18603,7.7);
#3373=CIRCLE('',#18605,9.2);
#3374=CIRCLE('',#18608,8.5);
#3375=CIRCLE('',#18609,8.);
#3376=CIRCLE('',#18611,33.);
#3377=CIRCLE('',#18612,32.5);
#3378=CIRCLE('',#18614,33.);
#3379=CIRCLE('',#18615,33.);
#3380=CIRCLE('',#18616,33.);
#3381=CIRCLE('',#18619,8.);
#3382=CIRCLE('',#18620,8.5);
#3383=CIRCLE('',#18623,33.);
#3384=CIRCLE('',#18624,32.5);
#3385=CIRCLE('',#18626,33.);
#3386=CIRCLE('',#18627,33.);
#3387=CIRCLE('',#18628,33.);
#3388=CIRCLE('',#18631,8.);
#3389=CIRCLE('',#18632,8.5);
#3390=CIRCLE('',#18635,33.);
#3391=CIRCLE('',#18636,32.5);
#3392=CIRCLE('',#18638,33.);
#3393=CIRCLE('',#18639,33.);
#3394=CIRCLE('',#18640,33.);
#3395=CIRCLE('',#18643,8.);
#3396=CIRCLE('',#18644,8.5);
#3397=CIRCLE('',#18647,33.);
#3398=CIRCLE('',#18648,32.5);
#3399=CIRCLE('',#18650,33.);
#3400=CIRCLE('',#18651,33.);
#3401=CIRCLE('',#18652,33.);
#3402=CIRCLE('',#18655,8.);
#3403=CIRCLE('',#18656,8.5);
#3404=CIRCLE('',#18659,33.);
#3405=CIRCLE('',#18660,32.5);
#3406=CIRCLE('',#18662,33.);
#3407=CIRCLE('',#18663,33.);
#3408=CIRCLE('',#18664,33.);
#3409=CIRCLE('',#18667,8.);
#3410=CIRCLE('',#18668,8.5);
#3411=CIRCLE('',#18670,32.5);
#3412=CIRCLE('',#18671,8.5);
#3413=CIRCLE('',#18672,32.5);
#3414=CIRCLE('',#18673,8.5);
#3415=CIRCLE('',#18674,32.5);
#3416=CIRCLE('',#18675,8.5);
#3417=CIRCLE('',#18676,32.5);
#3418=CIRCLE('',#18677,8.5);
#3419=CIRCLE('',#18678,32.5);
#3420=CIRCLE('',#18679,8.5);
#3421=CIRCLE('',#18680,32.5);
#3422=CIRCLE('',#18681,8.5);
#3423=CIRCLE('',#18682,32.5);
#3424=CIRCLE('',#18683,14.);
#3425=CIRCLE('',#18685,33.);
#3426=CIRCLE('',#18688,8.);
#3427=CIRCLE('',#18690,8.);
#3428=CIRCLE('',#18693,33.);
#3429=CIRCLE('',#18694,33.);
#3430=CIRCLE('',#18695,33.);
#3431=CIRCLE('',#18698,8.);
#3432=CIRCLE('',#18700,33.);
#3433=CIRCLE('',#18703,33.);
#3434=CIRCLE('',#18704,33.);
#3435=CIRCLE('',#18705,33.);
#3436=CIRCLE('',#18708,8.);
#3437=CIRCLE('',#18710,33.);
#3438=CIRCLE('',#18713,33.);
#3439=CIRCLE('',#18714,33.);
#3440=CIRCLE('',#18715,33.);
#3441=CIRCLE('',#18718,8.);
#3442=CIRCLE('',#18720,33.);
#3443=CIRCLE('',#18723,33.);
#3444=CIRCLE('',#18724,33.);
#3445=CIRCLE('',#18725,33.);
#3446=CIRCLE('',#18728,8.);
#3447=CIRCLE('',#18730,33.);
#3448=CIRCLE('',#18733,33.);
#3449=CIRCLE('',#18734,33.);
#3450=CIRCLE('',#18735,33.);
#3451=CIRCLE('',#18738,8.);
#3452=CIRCLE('',#18740,33.);
#3453=CIRCLE('',#18743,33.);
#3454=CIRCLE('',#18744,33.);
#3455=CIRCLE('',#18745,33.);
#3456=CIRCLE('',#18746,33.);
#3457=CIRCLE('',#18749,33.);
#3458=CIRCLE('',#18750,33.);
#3459=CIRCLE('',#18751,33.);
#3460=CIRCLE('',#18754,8.);
#3461=CIRCLE('',#18757,32.4);
#3462=CIRCLE('',#18759,8.);
#3463=CIRCLE('',#18761,3.442);
#3464=CIRCLE('',#18762,3.442);
#3465=CIRCLE('',#18764,3.442);
#3466=CIRCLE('',#18765,3.442);
#3467=CIRCLE('',#18766,2.872);
#3468=CIRCLE('',#18769,32.4);
#3469=CIRCLE('',#18772,8.);
#3470=CIRCLE('',#18777,8.);
#3471=CIRCLE('',#18782,8.);
#3472=CIRCLE('',#18787,8.);
#3473=CIRCLE('',#18792,8.);
#3474=CIRCLE('',#18797,8.);
#3475=CIRCLE('',#18802,8.);
#3476=CIRCLE('',#18807,8.);
#3477=CIRCLE('',#18812,8.);
#3478=CIRCLE('',#18823,8.5);
#3479=CIRCLE('',#18824,8.5);
#3480=CIRCLE('',#18827,9.2);
#3481=CIRCLE('',#18829,9.2);
#3482=CIRCLE('',#18832,30.);
#3483=CIRCLE('',#18835,30.);
#3484=CIRCLE('',#18838,30.);
#3485=CIRCLE('',#18841,30.);
#3486=CIRCLE('',#18844,30.);
#3487=CIRCLE('',#18847,30.);
#3488=CIRCLE('',#18850,30.);
#3489=CIRCLE('',#18853,30.);
#3490=CIRCLE('',#18856,30.);
#3491=CIRCLE('',#18859,30.);
#3492=CIRCLE('',#18862,30.);
#3493=CIRCLE('',#18865,30.);
#3494=CIRCLE('',#18883,12.);
#3495=CIRCLE('',#18887,8.8);
#3496=CIRCLE('',#18889,7.2);
#3497=CIRCLE('',#18891,6.2);
#3498=CIRCLE('',#18893,5.5);
#3499=CIRCLE('',#18895,5.5);
#3500=CIRCLE('',#18897,5.2);
#3501=CIRCLE('',#18899,3.3);
#3502=CIRCLE('',#18901,3.3);
#3503=CIRCLE('',#18903,3.5);
#3504=CIRCLE('',#18905,3.5);
#3505=CIRCLE('',#18907,2.9);
#3506=CIRCLE('',#18909,2.9);
#3507=CIRCLE('',#18912,3.442);
#3508=CIRCLE('',#18914,3.);
#3705=B_SPLINE_CURVE_WITH_KNOTS('',3,(#23617,#23618,#23619,#23620,#23621,
#23622,#23623,#23624,#23625,#23626),.UNSPECIFIED.,.F.,.F.,(4,3,3,4),(-4.0929304201303,
-3.96712820430096,-2.97534615322572,-2.06773127522693),.UNSPECIFIED.);
#3706=B_SPLINE_CURVE_WITH_KNOTS('',3,(#23629,#23630,#23631,#23632,#23633,
#23634,#23635),.UNSPECIFIED.,.F.,.F.,(4,3,4),(0.,0.991782051075235,1.1163935086858),
 .UNSPECIFIED.);
#3707=B_SPLINE_CURVE_WITH_KNOTS('',3,(#23640,#23641,#23642,#23643,#23644,
#23645,#23646,#23647,#23648,#23649,#23650,#23651,#23652,#23653,#23654,#23655,
#23656,#23657,#23658,#23659,#23660,#23661),.UNSPECIFIED.,.F.,.F.,(4,3,3,
3,3,3,3,4),(-10.37611572731,-9.9178205107524,-8.92603845967716,-7.93425640860193,
-6.94247435752668,-5.95069230645144,-4.9589102553762,-4.0929304201303),
 .UNSPECIFIED.);
#3708=B_SPLINE_CURVE_WITH_KNOTS('',3,(#23662,#23663,#23664,#23665,#23666,
#23667,#23668,#23669,#23670,#23671,#23672,#23673,#23674,#23675,#23676,#23677,
#23678,#23679,#23680,#23681,#23682,#23683),.UNSPECIFIED.,.F.,.F.,(4,3,3,
3,3,3,3,4),(1.1163935086858,1.98356410215048,2.97534615322572,3.96712820430096,
4.9589102553762,5.95069230645144,6.94247435752668,7.39957881586548),
 .UNSPECIFIED.);
#3709=B_SPLINE_CURVE_WITH_KNOTS('',3,(#23688,#23689,#23690,#23691,#23692,
#23693,#23694,#23695,#23696,#23697,#23698,#23699,#23700,#23701,#23702,#23703,
#23704,#23705,#23706,#23707,#23708,#23709),.UNSPECIFIED.,.F.,.F.,(4,3,3,
3,3,3,3,4),(-16.6593010344895,-15.8685128172038,-14.8767307661286,-13.8849487150534,
-12.8931666639781,-11.9013846129029,-10.9096025618276,-10.37611572731),
 .UNSPECIFIED.);
#3710=B_SPLINE_CURVE_WITH_KNOTS('',3,(#23710,#23711,#23712,#23713,#23714,
#23715,#23716,#23717,#23718,#23719,#23720,#23721,#23722,#23723,#23724,#23725,
#23726,#23727,#23728,#23729,#23730,#23731),.UNSPECIFIED.,.F.,.F.,(4,3,3,
3,3,3,3,4),(7.39957881586548,7.93425640860192,8.92603845967716,9.9178205107524,
10.9096025618276,11.9013846129029,12.8931666639781,13.682764123045),
 .UNSPECIFIED.);
#3711=B_SPLINE_CURVE_WITH_KNOTS('',3,(#23736,#23737,#23738,#23739,#23740,
#23741,#23742,#23743,#23744,#23745,#23746,#23747,#23748,#23749,#23750,#23751,
#23752,#23753,#23754,#23755,#23756,#23757,#23758,#23759,#23760),
 .UNSPECIFIED.,.F.,.F.,(4,3,3,3,3,3,3,3,4),(-22.9424863416691,-22.8109871747305,
-21.8192051236553,-20.8274230725801,-19.8356410215048,-18.8438589704296,
-17.8520769193543,-16.8602948682791,-16.6593010344895),.UNSPECIFIED.);
#3712=B_SPLINE_CURVE_WITH_KNOTS('',3,(#23761,#23762,#23763,#23764,#23765,
#23766,#23767,#23768,#23769,#23770,#23771,#23772,#23773,#23774,#23775,#23776,
#23777,#23778,#23779,#23780,#23781,#23782,#23783,#23784,#23785),
 .UNSPECIFIED.,.F.,.F.,(4,3,3,3,3,3,3,3,4),(13.682764123045,13.8849487150534,
14.8767307661286,15.8685128172039,16.8602948682791,17.8520769193543,18.8438589704296,
19.8356410215048,19.9659494302246),.UNSPECIFIED.);
#3713=B_SPLINE_CURVE_WITH_KNOTS('',3,(#23790,#23791,#23792,#23793,#23794,
#23795,#23796,#23797,#23798,#23799,#23800,#23801,#23802,#23803,#23804,#23805,
#23806,#23807,#23808,#23809,#23810,#23811),.UNSPECIFIED.,.F.,.F.,(4,3,3,
3,3,3,3,4),(-29.2256716488488,-28.761679481182,-27.7698974301067,-26.7781153790315,
-25.7863333279563,-24.794551276881,-23.8027692258058,-22.9424863416691),
 .UNSPECIFIED.);
#3714=B_SPLINE_CURVE_WITH_KNOTS('',3,(#23812,#23813,#23814,#23815,#23816,
#23817,#23818,#23819,#23820,#23821,#23822,#23823,#23824,#23825,#23826,#23827,
#23828,#23829,#23830,#23831,#23832,#23833),.UNSPECIFIED.,.F.,.F.,(4,3,3,
3,3,3,3,4),(19.9659494302246,20.8274230725801,21.8192051236553,22.8109871747305,
23.8027692258058,24.794551276881,25.7863333279562,26.2491347374043),
 .UNSPECIFIED.);
#3715=B_SPLINE_CURVE_WITH_KNOTS('',3,(#23838,#23839,#23840,#23841,#23842,
#23843,#23844,#23845,#23846,#23847,#23848,#23849,#23850,#23851,#23852,#23853,
#23854,#23855,#23856,#23857,#23858,#23859),.UNSPECIFIED.,.F.,.F.,(4,3,3,
3,3,3,3,4),(-35.5088569560282,-34.7123717876334,-33.7205897365582,-32.7288076854829,
-31.7370256344077,-30.7452435833325,-29.7534615322572,-29.2256716488488),
 .UNSPECIFIED.);
#3716=B_SPLINE_CURVE_WITH_KNOTS('',3,(#23860,#23861,#23862,#23863,#23864,
#23865,#23866,#23867,#23868,#23869,#23870,#23871,#23872,#23873,#23874,#23875,
#23876,#23877,#23878,#23879,#23880,#23881),.UNSPECIFIED.,.F.,.F.,(4,3,3,
3,3,3,3,4),(26.2491347374043,26.7781153790315,27.7698974301067,28.761679481182,
29.7534615322572,30.7452435833325,31.7370256344077,32.5323200445837),
 .UNSPECIFIED.);
#3717=B_SPLINE_CURVE_WITH_KNOTS('',3,(#23886,#23887,#23888,#23889,#23890,
#23891,#23892,#23893,#23894,#23895,#23896,#23897,#23898,#23899,#23900,#23901,
#23902,#23903,#23904,#23905,#23906,#23907,#23908,#23909,#23910),
 .UNSPECIFIED.,.F.,.F.,(4,3,3,3,3,3,3,3,4),(-41.7920422632079,-41.6548461451601,
-40.6630640940849,-39.6712820430096,-38.6794999919344,-37.6877179408591,
-36.6959358897839,-35.7041538387087,-35.5088569560282),.UNSPECIFIED.);
#3718=B_SPLINE_CURVE_WITH_KNOTS('',3,(#23911,#23912,#23913,#23914,#23915,
#23916,#23917,#23918,#23919,#23920,#23921,#23922,#23923,#23924,#23925,#23926,
#23927,#23928,#23929,#23930,#23931,#23932,#23933,#23934,#23935),
 .UNSPECIFIED.,.F.,.F.,(4,3,3,3,3,3,3,3,4),(32.5323200445837,32.7288076854829,
33.7205897365582,34.7123717876334,35.7041538387086,36.6959358897839,37.6877179408591,
38.6794999919344,38.8155053517634),.UNSPECIFIED.);
#3719=B_SPLINE_CURVE_WITH_KNOTS('',3,(#23940,#23941,#23942,#23943,#23944,
#23945,#23946,#23947,#23948,#23949,#23950,#23951,#23952,#23953,#23954,#23955,
#23956,#23957,#23958,#23959,#23960,#23961),.UNSPECIFIED.,.F.,.F.,(4,3,3,
3,3,3,3,4),(-48.0752275703874,-47.6055384516115,-46.6137564005363,-45.6219743494611,
-44.6301922983858,-43.6384102473106,-42.6466281962353,-41.7920422632079),
 .UNSPECIFIED.);
#3720=B_SPLINE_CURVE_WITH_KNOTS('',3,(#23962,#23963,#23964,#23965,#23966,
#23967,#23968,#23969,#23970,#23971,#23972,#23973,#23974,#23975,#23976,#23977,
#23978,#23979,#23980,#23981,#23982,#23983),.UNSPECIFIED.,.F.,.F.,(4,3,3,
3,3,3,3,4),(38.8155053517634,39.6712820430096,40.6630640940849,41.6548461451601,
42.6466281962353,43.6384102473106,44.6301922983858,45.0986906589429),
 .UNSPECIFIED.);
#3721=B_SPLINE_CURVE_WITH_KNOTS('',3,(#23988,#23989,#23990,#23991,#23992,
#23993,#23994,#23995,#23996,#23997,#23998,#23999,#24000,#24001,#24002,#24003,
#24004,#24005,#24006,#24007,#24008,#24009),.UNSPECIFIED.,.F.,.F.,(4,3,3,
3,3,3,3,4),(-54.358412877567,-53.556230758063,-52.5644487069877,-51.5726666559125,
-50.5808846048373,-49.589102553762,-48.5973205026868,-48.0752275703874),
 .UNSPECIFIED.);
#3722=B_SPLINE_CURVE_WITH_KNOTS('',3,(#24010,#24011,#24012,#24013,#24014,
#24015,#24016,#24017,#24018,#24019,#24020,#24021,#24022,#24023,#24024,#24025,
#24026,#24027,#24028,#24029,#24030,#24031),.UNSPECIFIED.,.F.,.F.,(4,3,3,
3,3,3,3,4),(45.0986906589429,45.6219743494611,46.6137564005363,47.6055384516115,
48.5973205026868,49.589102553762,50.5808846048373,51.3818759661225),
 .UNSPECIFIED.);
#3723=B_SPLINE_CURVE_WITH_KNOTS('',3,(#24036,#24037,#24038,#24039,#24040,
#24041,#24042,#24043,#24044,#24045,#24046,#24047,#24048,#24049,#24050,#24051,
#24052,#24053,#24054,#24055,#24056,#24057,#24058,#24059,#24060),
 .UNSPECIFIED.,.F.,.F.,(4,3,3,3,3,3,3,3,4),(-60.6415981847467,-60.4987051155897,
-59.5069230645144,-58.5151410134392,-57.5233589623639,-56.5315769112887,
-55.5397948602135,-54.5480128091382,-54.358412877567),.UNSPECIFIED.);
#3724=B_SPLINE_CURVE_WITH_KNOTS('',3,(#24061,#24062,#24063,#24064,#24065,
#24066,#24067,#24068,#24069,#24070,#24071,#24072,#24073,#24074,#24075,#24076,
#24077,#24078,#24079,#24080,#24081,#24082,#24083,#24084,#24085),
 .UNSPECIFIED.,.F.,.F.,(4,3,3,3,3,3,3,3,4),(51.3818759661225,51.5726666559125,
52.5644487069878,53.556230758063,54.5480128091382,55.5397948602135,56.5315769112887,
57.523358962364,57.6650612733022),.UNSPECIFIED.);
#3725=B_SPLINE_CURVE_WITH_KNOTS('',3,(#24090,#24091,#24092,#24093,#24094,
#24095,#24096,#24097,#24098,#24099,#24100,#24101,#24102,#24103,#24104,#24105,
#24106,#24107,#24108,#24109,#24110,#24111),.UNSPECIFIED.,.F.,.F.,(4,3,3,
3,3,3,3,4),(-66.9247834919262,-66.4493974220411,-65.4576153709659,-64.4658333198906,
-63.4740512688154,-62.4822692177402,-61.4904871666649,-60.6415981847467),
 .UNSPECIFIED.);
#3726=B_SPLINE_CURVE_WITH_KNOTS('',3,(#24112,#24113,#24114,#24115,#24116,
#24117,#24118,#24119,#24120,#24121,#24122,#24123,#24124,#24125,#24126,#24127,
#24128,#24129,#24130,#24131,#24132,#24133),.UNSPECIFIED.,.F.,.F.,(4,3,3,
3,3,3,3,4),(57.6650612733022,58.5151410134392,59.5069230645144,60.4987051155897,
61.4904871666649,62.4822692177402,63.4740512688154,63.9482465804817),
 .UNSPECIFIED.);
#3727=B_SPLINE_CURVE_WITH_KNOTS('',3,(#24138,#24139,#24140,#24141,#24142,
#24143,#24144,#24145,#24146,#24147,#24148,#24149,#24150,#24151,#24152,#24153,
#24154,#24155,#24156,#24157,#24158,#24159),.UNSPECIFIED.,.F.,.F.,(4,3,3,
3,3,3,3,4),(-73.2079687991058,-72.4000897284926,-71.4083076774173,-70.4165256263421,
-69.4247435752668,-68.4329615241916,-67.4411794731163,-66.9247834919262),
 .UNSPECIFIED.);
#3728=B_SPLINE_CURVE_WITH_KNOTS('',3,(#24160,#24161,#24162,#24163,#24164,
#24165,#24166,#24167,#24168,#24169,#24170,#24171,#24172,#24173,#24174,#24175,
#24176,#24177,#24178,#24179,#24180,#24181),.UNSPECIFIED.,.F.,.F.,(4,3,3,
3,3,3,3,4),(63.9482465804817,64.4658333198906,65.4576153709659,66.4493974220411,
67.4411794731163,68.4329615241916,69.4247435752668,70.2314318876613),
 .UNSPECIFIED.);
#3729=B_SPLINE_CURVE_WITH_KNOTS('',3,(#24186,#24187,#24188,#24189,#24190,
#24191,#24192,#24193,#24194,#24195,#24196,#24197,#24198,#24199,#24200,#24201,
#24202,#24203,#24204,#24205,#24206,#24207,#24208,#24209,#24210),
 .UNSPECIFIED.,.F.,.F.,(4,3,3,3,3,3,3,3,4),(-79.4911541062855,-79.3425640860193,
-78.350782034944,-77.3589999838688,-76.3672179327935,-75.3754358817183,
-74.383653830643,-73.3918717795678,-73.2079687991058),.UNSPECIFIED.);
#3730=B_SPLINE_CURVE_WITH_KNOTS('',3,(#24211,#24212,#24213,#24214,#24215,
#24216,#24217,#24218,#24219,#24220,#24221,#24222,#24223,#24224,#24225,#24226,
#24227,#24228,#24229,#24230,#24231,#24232,#24233,#24234,#24235),
 .UNSPECIFIED.,.F.,.F.,(4,3,3,3,3,3,3,3,4),(70.2314318876613,70.4165256263421,
71.4083076774173,72.4000897284925,73.3918717795678,74.383653830643,75.3754358817183,
76.3672179327935,76.514617194841),.UNSPECIFIED.);
#3731=B_SPLINE_CURVE_WITH_KNOTS('',3,(#24240,#24241,#24242,#24243,#24244,
#24245,#24246,#24247,#24248,#24249,#24250,#24251,#24252,#24253,#24254,#24255,
#24256,#24257,#24258,#24259,#24260,#24261),.UNSPECIFIED.,.F.,.F.,(4,3,3,
3,3,3,3,4),(-85.774339413465,-85.2932563924707,-84.3014743413955,-83.3096922903202,
-82.317910239245,-81.3261281881697,-80.3343461370945,-79.4911541062855),
 .UNSPECIFIED.);
#3732=B_SPLINE_CURVE_WITH_KNOTS('',3,(#24262,#24263,#24264,#24265,#24266,
#24267,#24268,#24269,#24270,#24271,#24272,#24273,#24274,#24275,#24276,#24277,
#24278,#24279,#24280,#24281,#24282,#24283),.UNSPECIFIED.,.F.,.F.,(4,3,3,
3,3,3,3,4),(76.514617194841,77.3589999838687,78.350782034944,79.3425640860192,
80.3343461370945,81.3261281881697,82.317910239245,82.7978025020205),
 .UNSPECIFIED.);
#3733=B_SPLINE_CURVE_WITH_KNOTS('',3,(#24288,#24289,#24290,#24291,#24292,
#24293,#24294,#24295,#24296,#24297,#24298,#24299,#24300,#24301,#24302,#24303,
#24304,#24305,#24306,#24307,#24308,#24309),.UNSPECIFIED.,.F.,.F.,(4,3,3,
3,3,3,3,4),(-92.0575247206446,-91.2439486989222,-90.2521666478469,-89.2603845967717,
-88.2686025456964,-87.2768204946212,-86.2850384435459,-85.774339413465),
 .UNSPECIFIED.);
#3734=B_SPLINE_CURVE_WITH_KNOTS('',3,(#24310,#24311,#24312,#24313,#24314,
#24315,#24316,#24317,#24318,#24319,#24320,#24321,#24322,#24323,#24324,#24325,
#24326,#24327,#24328,#24329,#24330,#24331),.UNSPECIFIED.,.F.,.F.,(4,3,3,
3,3,3,3,4),(82.7978025020205,83.3096922903202,84.3014743413955,85.2932563924707,
86.2850384435459,87.2768204946212,88.2686025456964,89.0809878092001),
 .UNSPECIFIED.);
#3735=B_SPLINE_CURVE_WITH_KNOTS('',3,(#24336,#24337,#24338,#24339,#24340,
#24341,#24342,#24343,#24344,#24345,#24346,#24347,#24348,#24349,#24350,#24351,
#24352,#24353,#24354,#24355,#24356,#24357,#24358,#24359,#24360),
 .UNSPECIFIED.,.F.,.F.,(4,3,3,3,3,3,3,3,4),(-98.3407100278241,-98.1864230564488,
-97.1946410053736,-96.2028589542983,-95.2110769032231,-94.2192948521479,
-93.2275128010726,-92.2357307499974,-92.0575247206446),.UNSPECIFIED.);
#3736=B_SPLINE_CURVE_WITH_KNOTS('',3,(#24361,#24362,#24363,#24364,#24365,
#24366,#24367,#24368,#24369,#24370,#24371,#24372,#24373,#24374,#24375,#24376,
#24377,#24378,#24379,#24380,#24381,#24382,#24383,#24384,#24385),
 .UNSPECIFIED.,.F.,.F.,(4,3,3,3,3,3,3,3,4),(89.0809878092001,89.2603845967717,
90.2521666478469,91.2439486989221,92.2357307499974,93.2275128010726,94.2192948521479,
95.2110769032231,95.3641731163798),.UNSPECIFIED.);
#3737=B_SPLINE_CURVE_WITH_KNOTS('',3,(#24670,#24671,#24672,#24673,#24674,
#24675,#24676,#24677,#24678,#24679,#24680,#24681,#24682),.UNSPECIFIED.,
 .F.,.F.,(4,3,3,3,4),(-0.621212683296683,-0.547442578207368,-0.286906424613279,
-0.13635260812343,-0.0501381164492948),.UNSPECIFIED.);
#3738=B_SPLINE_CURVE_WITH_KNOTS('',3,(#24684,#24685,#24686,#24687,#24688,
#24689),.UNSPECIFIED.,.F.,.F.,(4,2,4),(-0.59625459278609,-0.430840814871636,
-0.228304293786418),.UNSPECIFIED.);
#3739=B_SPLINE_CURVE_WITH_KNOTS('',3,(#24691,#24692,#24693,#24694),
 .UNSPECIFIED.,.F.,.F.,(4,4),(-7.28045043043161,-7.11297879609542),
 .UNSPECIFIED.);
#3740=B_SPLINE_CURVE_WITH_KNOTS('',3,(#24704,#24705,#24706,#24707,#24708,
#24709,#24710,#24711,#24712,#24713,#24714,#24715,#24716,#24717,#24718,#24719,
#24720,#24721,#24722,#24723,#24724,#24725,#24726,#24727,#24728,#24729,#24730,
#24731,#24732,#24733,#24734,#24735,#24736,#24737,#24738,#24739,#24740,#24741,
#24742,#24743,#24744,#24745,#24746,#24747,#24748,#24749,#24750,#24751,#24752,
#24753,#24754,#24755,#24756,#24757,#24758,#24759,#24760,#24761,#24762,#24763,
#24764,#24765,#24766,#24767,#24768,#24769,#24770),.UNSPECIFIED.,.F.,.F.,
(4,3,3,3,3,3,3,3,3,3,3,3,3,3,3,3,3,3,3,3,3,3,4),(-7.11297879609542,-7.10146924893286,
-5.58665127018164,-5.35053694579391,-5.18292437028481,-4.93518995665546,
-4.59847254575879,-4.20592684575953,-3.66025783498759,-3.16635853426091,
-2.76138423965328,-2.31987517722514,-2.01229466828823,-1.72292721736197,
-1.60295645902473,-1.18526991652666,-0.932600063372656,-0.806265136795657,
-0.720980394300845,-0.679930210218657,-0.615963294349632,-0.164312231354017,
0.),.UNSPECIFIED.);
#3741=B_SPLINE_CURVE_WITH_KNOTS('',3,(#24774,#24775,#24776,#24777),
 .UNSPECIFIED.,.F.,.F.,(4,4),(-0.123320533354435,0.),.UNSPECIFIED.);
#3742=B_SPLINE_CURVE_WITH_KNOTS('',3,(#24779,#24780,#24781,#24782,#24783,
#24784),.UNSPECIFIED.,.F.,.F.,(4,2,4),(-1.20932024771483,-0.985380063173393,
-0.454839283541959),.UNSPECIFIED.);
#3743=B_SPLINE_CURVE_WITH_KNOTS('',3,(#24786,#24787,#24788,#24789),
 .UNSPECIFIED.,.F.,.F.,(4,4),(-0.123345114071721,0.),.UNSPECIFIED.);
#3744=B_SPLINE_CURVE_WITH_KNOTS('',3,(#24793,#24794,#24795,#24796,#24797,
#24798,#24799,#24800,#24801,#24802,#24803,#24804,#24805,#24806,#24807,#24808,
#24809,#24810,#24811,#24812,#24813,#24814,#24815,#24816,#24817,#24818,#24819,
#24820,#24821,#24822,#24823,#24824,#24825,#24826,#24827,#24828,#24829,#24830,
#24831,#24832,#24833,#24834,#24835,#24836,#24837,#24838,#24839,#24840,#24841,
#24842,#24843,#24844,#24845,#24846,#24847,#24848,#24849,#24850,#24851,#24852,
#24853,#24854,#24855,#24856,#24857,#24858,#24859,#24860,#24861,#24862,#24863,
#24864,#24865),.UNSPECIFIED.,.F.,.F.,(4,3,3,3,3,3,3,3,3,3,3,3,3,3,3,3,3,
3,3,3,3,3,3,3,4),(-12.8459374903622,-11.4794095596864,-10.7961455943485,
-10.3238102702983,-10.1128816290106,-9.79002513500549,-7.17546445018599,
-5.86818410777624,-5.21454393657137,-4.88772385096893,-4.68535987608564,
-4.56090376536649,-4.42075803997013,-3.48474489263661,-2.76035534392185,
-2.17493233268881,-1.74712655326283,-1.70292711374468,-1.28137423833938,
-0.996111179634618,-0.765912925480064,-0.547442578207694,-0.286906424613352,
-0.136326843594367,-0.0501381164492894),.UNSPECIFIED.);
#3745=B_SPLINE_CURVE_WITH_KNOTS('',3,(#24867,#24868,#24869,#24870,#24871,
#24872),.UNSPECIFIED.,.F.,.F.,(4,2,4),(-0.993618385713602,-0.861681629743272,
-0.62552951637108),.UNSPECIFIED.);
#3746=B_SPLINE_CURVE_WITH_KNOTS('',3,(#24874,#24875,#24876,#24877,#24878,
#24879,#24880,#24881,#24882,#24883,#24884,#24885,#24886,#24887,#24888,#24889,
#24890,#24891,#24892,#24893,#24894,#24895,#24896,#24897,#24898,#24899,#24900,
#24901,#24902,#24903,#24904,#24905,#24906,#24907,#24908,#24909,#24910,#24911,
#24912,#24913,#24914,#24915,#24916,#24917,#24918,#24919,#24920,#24921,#24922,
#24923,#24924,#24925,#24926,#24927,#24928,#24929,#24930,#24931,#24932,#24933,
#24934,#24935,#24936,#24937,#24938,#24939,#24940),.UNSPECIFIED.,.F.,.F.,
(4,3,3,3,3,3,3,3,3,3,3,3,3,3,3,3,3,3,3,3,3,3,4),(-7.28045043097461,-7.10146924951175,
-5.58665127099474,-5.3505385242668,-5.18292571362766,-4.93518995738714,
-4.59847254647905,-4.20592684649596,-3.66025783571592,-3.16635853508255,
-2.76138424004969,-2.31987517755785,-2.01230406739047,-1.72292916443561,
-1.60295645915655,-1.18526991660116,-0.932600063410003,-0.806265136814425,
-0.720980394325866,-0.679930210218847,-0.615963294364446,-0.164312231361294,
0.),.UNSPECIFIED.);
#3747=B_SPLINE_CURVE_WITH_KNOTS('',3,(#24944,#24945,#24946,#24947),
 .UNSPECIFIED.,.F.,.F.,(4,4),(-0.123320533354439,0.),.UNSPECIFIED.);
#3748=B_SPLINE_CURVE_WITH_KNOTS('',3,(#24949,#24950,#24951,#24952),
 .UNSPECIFIED.,.F.,.F.,(4,4),(-1.0626156692464,-0.306410932880036),
 .UNSPECIFIED.);
#3749=B_SPLINE_CURVE_WITH_KNOTS('',3,(#24954,#24955,#24956,#24957),
 .UNSPECIFIED.,.F.,.F.,(4,4),(-0.12334511407167,0.),.UNSPECIFIED.);
#3750=B_SPLINE_CURVE_WITH_KNOTS('',3,(#24961,#24962,#24963,#24964,#24965,
#24966,#24967,#24968,#24969,#24970,#24971,#24972,#24973,#24974,#24975,#24976,
#24977,#24978,#24979,#24980,#24981,#24982,#24983,#24984,#24985,#24986,#24987,
#24988,#24989,#24990,#24991,#24992,#24993,#24994,#24995,#24996,#24997,#24998,
#24999,#25000,#25001,#25002,#25003,#25004,#25005,#25006,#25007,#25008,#25009,
#25010,#25011,#25012,#25013,#25014,#25015,#25016,#25017,#25018,#25019,#25020,
#25021,#25022,#25023,#25024,#25025,#25026,#25027,#25028,#25029,#25030,#25031,
#25032,#25033),.UNSPECIFIED.,.F.,.F.,(4,3,3,3,3,3,3,3,3,3,3,3,3,3,3,3,3,
3,3,3,3,3,3,3,4),(-12.8459374829188,-11.4794095553317,-10.7961455915381,
-10.3238102685133,-10.1128816277446,-9.79002513405492,-7.17546444972407,
-5.86818410755865,-5.21454393647594,-4.88772385093459,-4.68535987595121,
-4.56090376539323,-4.4207580397955,-3.48474489237297,-2.76035534392132,
-2.17493233268991,-1.74712655325337,-1.70292711374332,-1.28137423833823,
-0.996111179633743,-0.765912925479433,-0.547442578207301,-0.286906424613261,
-0.136326843593883,-0.0501381164492951),.UNSPECIFIED.);
#3751=B_SPLINE_CURVE_WITH_KNOTS('',3,(#25035,#25036,#25037,#25038,#25039,
#25040),.UNSPECIFIED.,.F.,.F.,(4,2,4),(-0.562962425256162,-0.401675631762058,
-0.194993927866297),.UNSPECIFIED.);
#3752=B_SPLINE_CURVE_WITH_KNOTS('',3,(#25042,#25043,#25044,#25045,#25046,
#25047,#25048,#25049,#25050,#25051,#25052,#25053,#25054,#25055,#25056,#25057,
#25058,#25059,#25060,#25061,#25062,#25063,#25064,#25065,#25066,#25067,#25068,
#25069,#25070,#25071,#25072,#25073,#25074,#25075,#25076,#25077,#25078,#25079,
#25080,#25081,#25082,#25083,#25084,#25085,#25086,#25087,#25088,#25089,#25090,
#25091,#25092,#25093,#25094,#25095,#25096,#25097,#25098,#25099,#25100,#25101,
#25102,#25103,#25104,#25105,#25106,#25107,#25108),.UNSPECIFIED.,.F.,.F.,
(4,3,3,3,3,3,3,3,3,3,3,3,3,3,3,3,3,3,3,3,3,3,4),(-7.28045043032899,-7.10146924891762,
-5.58665127078463,-5.3505385241117,-5.18292571340915,-4.93518995720784,
-4.59847254633886,-4.20592684642313,-3.6602578357137,-3.16635853522375,
-2.761384239933,-2.31987517752994,-2.01230406745978,-1.72292916434363,-1.60295645905542,
-1.18526991655219,-0.932600063385415,-0.806265136802025,-0.720980394296157,
-0.679930210218636,-0.615963294341316,-0.16431223136616,0.),
 .UNSPECIFIED.);
#3753=B_SPLINE_CURVE_WITH_KNOTS('',3,(#25112,#25113,#25114,#25115),
 .UNSPECIFIED.,.F.,.F.,(4,4),(-0.123320533354441,0.),.UNSPECIFIED.);
#3754=B_SPLINE_CURVE_WITH_KNOTS('',3,(#25117,#25118,#25119,#25120,#25121,
#25122),.UNSPECIFIED.,.F.,.F.,(4,2,4),(-1.35394250197628,-0.852961572903344,
-0.599740178024191),.UNSPECIFIED.);
#3755=B_SPLINE_CURVE_WITH_KNOTS('',3,(#25124,#25125,#25126,#25127),
 .UNSPECIFIED.,.F.,.F.,(4,4),(-0.12334511407174,0.),.UNSPECIFIED.);
#3756=B_SPLINE_CURVE_WITH_KNOTS('',3,(#25131,#25132,#25133,#25134,#25135,
#25136,#25137,#25138,#25139,#25140,#25141,#25142,#25143,#25144,#25145,#25146,
#25147,#25148,#25149,#25150,#25151,#25152,#25153,#25154,#25155,#25156,#25157,
#25158,#25159,#25160,#25161,#25162,#25163,#25164,#25165,#25166,#25167,#25168,
#25169,#25170,#25171,#25172,#25173,#25174,#25175,#25176,#25177,#25178,#25179,
#25180,#25181,#25182,#25183,#25184,#25185,#25186,#25187,#25188,#25189,#25190,
#25191,#25192,#25193,#25194,#25195,#25196,#25197,#25198,#25199,#25200,#25201,
#25202,#25203),.UNSPECIFIED.,.F.,.F.,(4,3,3,3,3,3,3,3,3,3,3,3,3,3,3,3,3,
3,3,3,3,3,3,3,4),(-12.8459375038567,-11.4794095705419,-10.7961456038845,
-10.3238102789195,-10.112881637227,-9.79002514266153,-7.1754644540322,-5.86818410971753,
-5.2145439375602,-4.88772385148153,-4.68535987651687,-4.56090376540287,
-4.42075804010368,-3.4847448928061,-2.76035534392402,-2.17493233269109,
-1.74712655325811,-1.70292711374465,-1.28137423833928,-0.996111179634543,
-0.765912925480012,-0.547442578207666,-0.286906424613349,-0.136326843594312,
-0.0501381164492891),.UNSPECIFIED.);
#3757=B_SPLINE_CURVE_WITH_KNOTS('',3,(#25205,#25206,#25207,#25208,#25209,
#25210),.UNSPECIFIED.,.F.,.F.,(4,2,4),(-0.59625459278609,-0.430840814871637,
-0.228304293786418),.UNSPECIFIED.);
#3758=B_SPLINE_CURVE_WITH_KNOTS('',3,(#25212,#25213,#25214,#25215,#25216,
#25217,#25218,#25219,#25220,#25221,#25222,#25223,#25224,#25225,#25226,#25227,
#25228,#25229,#25230,#25231,#25232,#25233,#25234,#25235,#25236,#25237,#25238,
#25239,#25240,#25241,#25242,#25243,#25244,#25245,#25246,#25247,#25248,#25249,
#25250,#25251,#25252,#25253,#25254,#25255,#25256,#25257,#25258,#25259,#25260,
#25261,#25262,#25263,#25264,#25265,#25266,#25267,#25268,#25269,#25270,#25271,
#25272,#25273,#25274,#25275,#25276,#25277,#25278),.UNSPECIFIED.,.F.,.F.,
(4,3,3,3,3,3,3,3,3,3,3,3,3,3,3,3,3,3,3,3,3,3,4),(-7.28045043166272,-7.10146925011317,
-5.58665127095826,-5.35053852414499,-5.18292571362894,-4.93518995732684,
-4.59847254636421,-4.2059268462769,-3.66025783539328,-3.16635853453117,
-2.76138423998915,-2.31987517746889,-2.01230406724825,-1.72292916446406,
-1.60295645919639,-1.18526991661974,-0.932600063420101,-0.806265136820283,
-0.72098039431399,-0.679930210220465,-0.615963294353296,-0.164312231344775,
0.),.UNSPECIFIED.);
#3759=B_SPLINE_CURVE_WITH_KNOTS('',3,(#25282,#25283,#25284,#25285),
 .UNSPECIFIED.,.F.,.F.,(4,4),(-0.123320533354419,0.),.UNSPECIFIED.);
#3760=B_SPLINE_CURVE_WITH_KNOTS('',3,(#25287,#25288,#25289,#25290,#25291,
#25292),.UNSPECIFIED.,.F.,.F.,(4,2,4),(-1.20932024771483,-0.985380063173395,
-0.454839283541961),.UNSPECIFIED.);
#3761=B_SPLINE_CURVE_WITH_KNOTS('',3,(#25294,#25295,#25296,#25297),
 .UNSPECIFIED.,.F.,.F.,(4,4),(-0.123345114071717,0.),.UNSPECIFIED.);
#3762=B_SPLINE_CURVE_WITH_KNOTS('',3,(#25301,#25302,#25303,#25304,#25305,
#25306,#25307,#25308,#25309,#25310,#25311,#25312,#25313,#25314,#25315,#25316,
#25317,#25318,#25319,#25320,#25321,#25322,#25323,#25324,#25325,#25326,#25327,
#25328,#25329,#25330,#25331,#25332,#25333,#25334,#25335,#25336,#25337,#25338,
#25339,#25340,#25341,#25342,#25343,#25344,#25345,#25346,#25347,#25348,#25349,
#25350,#25351,#25352,#25353,#25354,#25355,#25356,#25357,#25358,#25359,#25360,
#25361,#25362,#25363,#25364,#25365,#25366,#25367,#25368,#25369,#25370,#25371,
#25372,#25373),.UNSPECIFIED.,.F.,.F.,(4,3,3,3,3,3,3,3,3,3,3,3,3,3,3,3,3,
3,3,3,3,3,3,3,4),(-12.845937481397,-11.4794095526284,-10.7961455882441,
-10.3238102648368,-10.1128816238599,-9.79002513019444,-7.1754644477685,
-5.86818410655552,-5.21454393594904,-4.88772385064579,-4.68535987568061,
-4.56090376534255,-4.42075803979776,-3.48474489238989,-2.76035534391794,
-2.17493233268459,-1.7471265532667,-1.7029271137431,-1.28137423833835,-0.996111179633872,
-0.765912925479539,-0.547442578207378,-0.286906424613282,-0.136326843594111,
-0.0501381164492929),.UNSPECIFIED.);
#3763=B_SPLINE_CURVE_WITH_KNOTS('',3,(#25375,#25376,#25377,#25378,#25379,
#25380),.UNSPECIFIED.,.F.,.F.,(4,2,4),(-0.993618385713604,-0.861681629743274,
-0.625529516371081),.UNSPECIFIED.);
#3764=B_SPLINE_CURVE_WITH_KNOTS('',3,(#25382,#25383,#25384,#25385,#25386,
#25387,#25388,#25389,#25390,#25391,#25392,#25393,#25394,#25395,#25396,#25397,
#25398,#25399,#25400,#25401,#25402,#25403,#25404,#25405,#25406,#25407,#25408,
#25409,#25410,#25411,#25412,#25413,#25414,#25415,#25416,#25417,#25418,#25419,
#25420,#25421,#25422,#25423,#25424,#25425,#25426,#25427,#25428,#25429,#25430,
#25431,#25432,#25433,#25434,#25435,#25436,#25437,#25438,#25439,#25440,#25441,
#25442,#25443,#25444,#25445,#25446,#25447,#25448),.UNSPECIFIED.,.F.,.F.,
(4,3,3,3,3,3,3,3,3,3,3,3,3,3,3,3,3,3,3,3,3,3,4),(-7.28045042893884,-7.10146924747538,
-5.58665126903134,-5.35053852232403,-5.18292571185153,-4.93518995565818,
-4.59847254483662,-4.2059268449215,-3.66025783426991,-3.16635853364197,
-2.76138423916958,-2.31987517683752,-2.01230406676,-1.7229291640395,-1.60295645881592,
-1.18526991641048,-0.932600063313362,-0.806265136764801,-0.720980394288129,
-0.67993021021624,-0.615963294347702,-0.164312231346664,0.),
 .UNSPECIFIED.);
#3765=B_SPLINE_CURVE_WITH_KNOTS('',3,(#25452,#25453,#25454,#25455),
 .UNSPECIFIED.,.F.,.F.,(4,4),(-0.123320533354399,0.),.UNSPECIFIED.);
#3766=B_SPLINE_CURVE_WITH_KNOTS('',3,(#25457,#25458,#25459,#25460),
 .UNSPECIFIED.,.F.,.F.,(4,4),(-1.0626156692464,-0.306410932880038),
 .UNSPECIFIED.);
#3767=B_SPLINE_CURVE_WITH_KNOTS('',3,(#25462,#25463,#25464,#25465),
 .UNSPECIFIED.,.F.,.F.,(4,4),(-0.123345114071698,0.),.UNSPECIFIED.);
#3768=B_SPLINE_CURVE_WITH_KNOTS('',3,(#25469,#25470,#25471,#25472,#25473,
#25474,#25475,#25476,#25477,#25478,#25479,#25480,#25481,#25482,#25483,#25484,
#25485,#25486,#25487,#25488,#25489,#25490,#25491,#25492,#25493,#25494,#25495,
#25496,#25497,#25498,#25499,#25500,#25501,#25502,#25503,#25504,#25505,#25506,
#25507,#25508,#25509,#25510,#25511,#25512,#25513,#25514,#25515,#25516,#25517,
#25518,#25519,#25520,#25521,#25522,#25523,#25524,#25525,#25526,#25527,#25528,
#25529,#25530,#25531,#25532,#25533,#25534,#25535,#25536,#25537,#25538,#25539,
#25540,#25541),.UNSPECIFIED.,.F.,.F.,(4,3,3,3,3,3,3,3,3,3,3,3,3,3,3,3,3,
3,3,3,3,3,3,3,4),(-12.8459374966351,-11.47940956567,-10.7961456001875,-10.3238102760087,
-10.112881634705,-9.79002514042822,-7.17546445291215,-5.86818410915412,
-5.2145439372751,-4.88772385133559,-4.68535987628659,-4.56090376539608,
-4.42075803990238,-3.48474489262088,-2.76035534392035,-2.17493233268499,
-1.74712655327526,-1.70292711374321,-1.28137423833862,-0.996111179634085,
-0.765912925479667,-0.547442578207445,-0.286906424613299,-0.136326843594094,
-0.0501381164492935),.UNSPECIFIED.);
#3769=B_SPLINE_CURVE_WITH_KNOTS('',3,(#25543,#25544,#25545,#25546,#25547,
#25548),.UNSPECIFIED.,.F.,.F.,(4,2,4),(-0.562962425256162,-0.401675631762059,
-0.194993927866297),.UNSPECIFIED.);
#3770=B_SPLINE_CURVE_WITH_KNOTS('',3,(#25550,#25551,#25552,#25553,#25554,
#25555,#25556,#25557,#25558,#25559,#25560,#25561,#25562,#25563,#25564,#25565,
#25566,#25567,#25568,#25569,#25570,#25571,#25572,#25573,#25574,#25575,#25576,
#25577,#25578,#25579,#25580,#25581,#25582,#25583,#25584,#25585,#25586,#25587,
#25588,#25589,#25590,#25591,#25592,#25593,#25594,#25595,#25596,#25597,#25598,
#25599,#25600,#25601,#25602,#25603,#25604,#25605,#25606,#25607,#25608,#25609,
#25610,#25611,#25612,#25613,#25614,#25615,#25616),.UNSPECIFIED.,.F.,.F.,
(4,3,3,3,3,3,3,3,3,3,3,3,3,3,3,3,3,3,3,3,3,3,4),(-7.28045043082453,-7.10146924927971,
-5.58665127018918,-5.35053852339042,-5.18292571293016,-4.93518995664928,
-4.59847254572338,-4.20592684566866,-3.6602578348416,-3.16635853399249,
-2.76138423964393,-2.31987517718532,-2.01230406700153,-1.72292916430381,
-1.60295645905806,-1.18526991654249,-0.932600063380627,-0.806265136799696,
-0.720980394307554,-0.679930210218765,-0.615963294354504,-0.164312231365093,
0.),.UNSPECIFIED.);
#3771=B_SPLINE_CURVE_WITH_KNOTS('',3,(#25620,#25621,#25622,#25623),
 .UNSPECIFIED.,.F.,.F.,(4,4),(-0.123320533354414,0.),.UNSPECIFIED.);
#3772=B_SPLINE_CURVE_WITH_KNOTS('',3,(#25625,#25626,#25627,#25628,#25629,
#25630),.UNSPECIFIED.,.F.,.F.,(4,2,4),(-1.35394250197628,-0.852961572903346,
-0.59974017802419),.UNSPECIFIED.);
#3773=B_SPLINE_CURVE_WITH_KNOTS('',3,(#25632,#25633,#25634,#25635),
 .UNSPECIFIED.,.F.,.F.,(4,4),(-0.123345114071673,0.),.UNSPECIFIED.);
#3774=B_SPLINE_CURVE_WITH_KNOTS('',3,(#25639,#25640,#25641,#25642,#25643,
#25644,#25645,#25646,#25647,#25648,#25649,#25650,#25651,#25652,#25653,#25654,
#25655,#25656,#25657,#25658,#25659,#25660,#25661,#25662,#25663,#25664,#25665,
#25666,#25667,#25668,#25669,#25670,#25671,#25672,#25673,#25674,#25675,#25676,
#25677,#25678,#25679,#25680,#25681,#25682,#25683,#25684,#25685,#25686,#25687,
#25688,#25689,#25690,#25691,#25692,#25693,#25694,#25695,#25696,#25697,#25698,
#25699,#25700,#25701,#25702,#25703,#25704,#25705,#25706,#25707,#25708,#25709,
#25710,#25711),.UNSPECIFIED.,.F.,.F.,(4,3,3,3,3,3,3,3,3,3,3,3,3,3,3,3,3,
3,3,3,3,3,3,3,4),(-12.8459374941425,-11.4794095636326,-10.7961455983776,
-10.3238102743478,-10.1128816331227,-9.79002513892905,-7.17546445215169,
-5.86818410876301,-5.21454393706867,-4.8877238512215,-4.68535987616866,
-4.56090376537433,-4.42075803987497,-3.48474489239197,-2.76035534391279,
-2.17493233267342,-1.74712655332313,-1.70292711374052,-1.28137423833797,
-0.996111179633762,-0.765912925479437,-0.5474425782073,-0.286906424613261,
-0.136326843593853,-0.0501381164492956),.UNSPECIFIED.);
#3775=B_SPLINE_CURVE_WITH_KNOTS('',3,(#25713,#25714,#25715,#25716,#25717,
#25718),.UNSPECIFIED.,.F.,.F.,(4,2,4),(-0.59625459278609,-0.430840814871637,
-0.228304293786418),.UNSPECIFIED.);
#3776=B_SPLINE_CURVE_WITH_KNOTS('',3,(#25720,#25721,#25722,#25723,#25724,
#25725,#25726,#25727,#25728,#25729,#25730,#25731,#25732,#25733,#25734,#25735,
#25736,#25737,#25738,#25739,#25740,#25741,#25742,#25743,#25744,#25745,#25746,
#25747,#25748,#25749,#25750,#25751,#25752,#25753,#25754,#25755,#25756,#25757,
#25758,#25759,#25760,#25761,#25762,#25763,#25764,#25765,#25766,#25767,#25768,
#25769,#25770,#25771,#25772,#25773,#25774,#25775,#25776,#25777,#25778,#25779,
#25780,#25781,#25782,#25783,#25784,#25785,#25786),.UNSPECIFIED.,.F.,.F.,
(4,3,3,3,3,3,3,3,3,3,3,3,3,3,3,3,3,3,3,3,3,3,4),(-7.28045043046879,-7.10146924897955,
-5.5866512702956,-5.35053852355109,-5.18292571300685,-4.93518995676392,
-4.59847254587039,-4.20592684588041,-3.66025783511541,-3.16635853441469,
-2.7613842397294,-2.31987517727554,-2.01230406711462,-1.72292916430658,
-1.6029564590523,-1.18526991653489,-0.932600063375318,-0.806265136795533,
-0.72098039430825,-0.679930210215748,-0.615963294352945,-0.164312231215415,
0.),.UNSPECIFIED.);
#3777=B_SPLINE_CURVE_WITH_KNOTS('',3,(#25790,#25791,#25792,#25793),
 .UNSPECIFIED.,.F.,.F.,(4,4),(-0.123320533354419,0.),.UNSPECIFIED.);
#3778=B_SPLINE_CURVE_WITH_KNOTS('',3,(#25795,#25796,#25797,#25798,#25799,
#25800),.UNSPECIFIED.,.F.,.F.,(4,2,4),(-1.20932024771483,-0.985380063173395,
-0.454839283541961),.UNSPECIFIED.);
#3779=B_SPLINE_CURVE_WITH_KNOTS('',3,(#25802,#25803,#25804,#25805),
 .UNSPECIFIED.,.F.,.F.,(4,4),(-0.123345114071701,0.),.UNSPECIFIED.);
#3780=B_SPLINE_CURVE_WITH_KNOTS('',3,(#25809,#25810,#25811,#25812,#25813,
#25814,#25815,#25816,#25817,#25818,#25819,#25820,#25821,#25822,#25823,#25824,
#25825,#25826,#25827,#25828,#25829,#25830,#25831,#25832,#25833,#25834,#25835,
#25836,#25837,#25838,#25839,#25840,#25841,#25842,#25843,#25844,#25845,#25846,
#25847,#25848,#25849,#25850,#25851,#25852,#25853,#25854,#25855,#25856,#25857,
#25858,#25859,#25860,#25861,#25862,#25863,#25864,#25865,#25866,#25867,#25868,
#25869,#25870,#25871,#25872,#25873,#25874,#25875,#25876,#25877,#25878,#25879,
#25880,#25881),.UNSPECIFIED.,.F.,.F.,(4,3,3,3,3,3,3,3,3,3,3,3,3,3,3,3,3,
3,3,3,3,3,3,3,4),(-12.8459374808793,-11.4794095526363,-10.7961455885147,
-10.3238102652891,-10.1128816243932,-9.79002513076713,-7.17546444805649,
-5.86818410670117,-5.21454393602351,-4.88772385068468,-4.68535987570999,
-4.56090376534585,-4.42075803974874,-3.48474489224273,-2.7603553439125,
-2.1749323326753,-1.74712655331056,-1.70292711374082,-1.28137423833786,
-0.996111179633715,-0.765912925479485,-0.547442578207348,-0.286906424613266,
-0.136326843594045,-0.0501381164492935),.UNSPECIFIED.);
#3781=B_SPLINE_CURVE_WITH_KNOTS('',3,(#25883,#25884,#25885,#25886,#25887,
#25888),.UNSPECIFIED.,.F.,.F.,(4,2,4),(-0.993618385713603,-0.861681629743274,
-0.625529516371081),.UNSPECIFIED.);
#3782=B_SPLINE_CURVE_WITH_KNOTS('',3,(#25890,#25891,#25892,#25893,#25894,
#25895,#25896,#25897,#25898,#25899,#25900,#25901,#25902,#25903,#25904,#25905,
#25906,#25907,#25908,#25909,#25910,#25911,#25912,#25913,#25914,#25915,#25916,
#25917,#25918,#25919,#25920,#25921,#25922,#25923,#25924,#25925,#25926,#25927,
#25928,#25929,#25930,#25931,#25932,#25933,#25934,#25935,#25936,#25937,#25938,
#25939,#25940,#25941,#25942,#25943,#25944,#25945,#25946,#25947,#25948,#25949,
#25950,#25951,#25952,#25953,#25954,#25955,#25956),.UNSPECIFIED.,.F.,.F.,
(4,3,3,3,3,3,3,3,3,3,3,3,3,3,3,3,3,3,3,3,3,3,4),(-7.28045043064328,-7.10146924914703,
-5.58665127040606,-5.35053852365389,-5.18292571310771,-4.93518995685649,
-4.59847254595278,-4.20592684595026,-3.66025783517109,-3.16635853444291,
-2.76138423978034,-2.31987517731217,-2.01230406713492,-1.72292916433732,
-1.60295645908227,-1.18526991655821,-0.932600063388904,-0.806265136804252,
-0.72098039430321,-0.679930210219599,-0.615963294348663,-0.16431223133682,
0.),.UNSPECIFIED.);
#3783=B_SPLINE_CURVE_WITH_KNOTS('',3,(#25960,#25961,#25962,#25963),
 .UNSPECIFIED.,.F.,.F.,(4,4),(-0.123320533354419,0.),.UNSPECIFIED.);
#3784=B_SPLINE_CURVE_WITH_KNOTS('',3,(#25965,#25966,#25967,#25968),
 .UNSPECIFIED.,.F.,.F.,(4,4),(-1.0626156692464,-0.306410932880038),
 .UNSPECIFIED.);
#3785=B_SPLINE_CURVE_WITH_KNOTS('',3,(#25970,#25971,#25972,#25973),
 .UNSPECIFIED.,.F.,.F.,(4,4),(-0.123345114071741,0.),.UNSPECIFIED.);
#3786=B_SPLINE_CURVE_WITH_KNOTS('',3,(#25977,#25978,#25979,#25980,#25981,
#25982,#25983,#25984,#25985,#25986,#25987,#25988,#25989,#25990,#25991,#25992,
#25993,#25994,#25995,#25996,#25997,#25998,#25999,#26000,#26001,#26002,#26003,
#26004,#26005,#26006,#26007,#26008,#26009,#26010,#26011,#26012,#26013,#26014,
#26015,#26016,#26017,#26018,#26019,#26020,#26021,#26022,#26023,#26024,#26025,
#26026,#26027,#26028,#26029,#26030,#26031,#26032,#26033,#26034,#26035,#26036,
#26037,#26038,#26039,#26040,#26041,#26042,#26043,#26044,#26045,#26046,#26047,
#26048,#26049),.UNSPECIFIED.,.F.,.F.,(4,3,3,3,3,3,3,3,3,3,3,3,3,3,3,3,3,
3,3,3,3,3,3,3,4),(-12.8459374931962,-11.4794095622303,-10.7961455967474,
-10.3238102725535,-10.1128816312645,-9.79002513704445,-7.17546445119587,
-5.86818410827158,-5.21454393680944,-4.88772385107836,-4.68535987603764,
-4.56090376534729,-4.42075803988792,-3.4847448924849,-2.76035534391094,
-2.17493233266957,-1.74712655334424,-1.70292711374143,-1.28137423833914,
-0.996111179634701,-0.765912925480124,-0.54744257820773,-0.286906424613362,
-0.136326843594467,-0.0501381164492885),.UNSPECIFIED.);
#3787=B_SPLINE_CURVE_WITH_KNOTS('',3,(#26051,#26052,#26053,#26054,#26055,
#26056),.UNSPECIFIED.,.F.,.F.,(4,2,4),(-0.562962425256162,-0.401675631762059,
-0.194993927866297),.UNSPECIFIED.);
#3788=B_SPLINE_CURVE_WITH_KNOTS('',3,(#26058,#26059,#26060,#26061,#26062,
#26063,#26064,#26065,#26066,#26067,#26068,#26069,#26070,#26071,#26072,#26073,
#26074,#26075,#26076,#26077,#26078,#26079,#26080,#26081,#26082,#26083,#26084,
#26085,#26086,#26087,#26088,#26089,#26090,#26091,#26092,#26093,#26094,#26095,
#26096,#26097,#26098,#26099,#26100,#26101,#26102,#26103,#26104,#26105,#26106,
#26107,#26108,#26109,#26110,#26111,#26112,#26113,#26114,#26115,#26116,#26117,
#26118,#26119,#26120,#26121,#26122,#26123,#26124),.UNSPECIFIED.,.F.,.F.,
(4,3,3,3,3,3,3,3,3,3,3,3,3,3,3,3,3,3,3,3,3,3,4),(-7.28045043029337,-7.10146924879316,
-5.58665127003706,-5.35053852328322,-5.18292571277321,-4.93518995652797,
-4.59847254563688,-4.20592684564096,-3.66025783487647,-3.16635853414848,
-2.76138423958633,-2.31987517717087,-2.01230406703615,-1.72292916424559,
-1.60295645899705,-1.18526991650819,-0.932600063361394,-0.806265136787995,
-0.720980394298989,-0.679930210214595,-0.615963294349437,-0.164312231356818,
0.),.UNSPECIFIED.);
#3789=B_SPLINE_CURVE_WITH_KNOTS('',3,(#26128,#26129,#26130,#26131),
 .UNSPECIFIED.,.F.,.F.,(4,4),(-0.123320533354417,0.),.UNSPECIFIED.);
#3790=B_SPLINE_CURVE_WITH_KNOTS('',3,(#26133,#26134,#26135,#26136,#26137,
#26138),.UNSPECIFIED.,.F.,.F.,(4,2,4),(-1.35394250197628,-0.852961572903345,
-0.599740178024189),.UNSPECIFIED.);
#3791=B_SPLINE_CURVE_WITH_KNOTS('',3,(#26140,#26141,#26142,#26143),
 .UNSPECIFIED.,.F.,.F.,(4,4),(-0.123345114071735,0.),.UNSPECIFIED.);
#3792=B_SPLINE_CURVE_WITH_KNOTS('',3,(#26147,#26148,#26149,#26150,#26151,
#26152,#26153,#26154,#26155,#26156,#26157,#26158,#26159,#26160,#26161,#26162,
#26163,#26164,#26165,#26166,#26167,#26168,#26169,#26170,#26171,#26172,#26173,
#26174,#26175,#26176,#26177,#26178,#26179,#26180,#26181,#26182,#26183,#26184,
#26185,#26186,#26187,#26188,#26189,#26190,#26191,#26192,#26193,#26194,#26195,
#26196,#26197,#26198,#26199,#26200,#26201,#26202,#26203,#26204,#26205,#26206,
#26207,#26208,#26209,#26210,#26211,#26212,#26213,#26214,#26215,#26216,#26217,
#26218,#26219),.UNSPECIFIED.,.F.,.F.,(4,3,3,3,3,3,3,3,3,3,3,3,3,3,3,3,3,
3,3,3,3,3,3,3,4),(-12.8459375085894,-11.4794095748003,-10.7961456079058,
-10.3238102827373,-10.1128816410112,-9.79002514616695,-7.17546445577377,
-5.86818411057718,-5.21454393797889,-4.88772385167974,-4.68535987651592,
-4.56090376538059,-4.42075803995975,-3.4847448925491,-2.76035534390967,
-2.17493233266947,-1.7471265533345,-1.70292711373975,-1.28137423833773,
-0.996111179633625,-0.765912925479341,-0.547442578207242,-0.286906424613248,
-0.13632684359387,-0.0501381164492966),.UNSPECIFIED.);
#3793=B_SPLINE_CURVE_WITH_KNOTS('',3,(#26221,#26222,#26223,#26224,#26225,
#26226),.UNSPECIFIED.,.F.,.F.,(4,2,4),(-0.59625459278609,-0.430840814871637,
-0.228304293786418),.UNSPECIFIED.);
#3794=B_SPLINE_CURVE_WITH_KNOTS('',3,(#26228,#26229,#26230,#26231,#26232,
#26233,#26234,#26235,#26236,#26237,#26238,#26239,#26240,#26241,#26242,#26243,
#26244,#26245,#26246,#26247,#26248,#26249,#26250,#26251,#26252,#26253,#26254,
#26255,#26256,#26257,#26258,#26259,#26260,#26261,#26262,#26263,#26264,#26265,
#26266,#26267,#26268,#26269,#26270,#26271,#26272,#26273,#26274,#26275,#26276,
#26277,#26278,#26279,#26280,#26281,#26282,#26283,#26284,#26285,#26286,#26287,
#26288,#26289,#26290,#26291,#26292,#26293,#26294),.UNSPECIFIED.,.F.,.F.,
(4,3,3,3,3,3,3,3,3,3,3,3,3,3,3,3,3,3,3,3,3,3,4),(-7.2804504305595,-7.10146924906192,
-5.58665127031306,-5.35053852355854,-5.18292571301866,-4.93518995676791,
-4.59847254586487,-4.20592684586167,-3.6602578350825,-3.16635853435267,
-2.76138423970751,-2.31987517726742,-2.01229466833062,-1.72292721738687,
-1.60295645904427,-1.18526991653728,-0.932600063377868,-0.806265136798164,
-0.720980394308923,-0.679930210218459,-0.615963294355597,-0.164312231353533,
0.),.UNSPECIFIED.);
#3795=B_SPLINE_CURVE_WITH_KNOTS('',3,(#26298,#26299,#26300,#26301),
 .UNSPECIFIED.,.F.,.F.,(4,4),(-0.123320533354386,0.),.UNSPECIFIED.);
#3796=B_SPLINE_CURVE_WITH_KNOTS('',3,(#26303,#26304,#26305,#26306,#26307,
#26308),.UNSPECIFIED.,.F.,.F.,(4,2,4),(-1.20932024771483,-0.985380063173395,
-0.454839283541961),.UNSPECIFIED.);
#3797=B_SPLINE_CURVE_WITH_KNOTS('',3,(#26310,#26311,#26312,#26313),
 .UNSPECIFIED.,.F.,.F.,(4,4),(-0.12334511407169,0.),.UNSPECIFIED.);
#3798=B_SPLINE_CURVE_WITH_KNOTS('',3,(#26317,#26318,#26319,#26320,#26321,
#26322,#26323,#26324,#26325,#26326,#26327,#26328,#26329,#26330,#26331,#26332,
#26333,#26334,#26335,#26336,#26337,#26338,#26339,#26340,#26341,#26342,#26343,
#26344,#26345,#26346,#26347,#26348,#26349,#26350,#26351,#26352,#26353,#26354,
#26355,#26356,#26357,#26358,#26359,#26360,#26361,#26362,#26363,#26364,#26365,
#26366,#26367,#26368,#26369,#26370,#26371,#26372,#26373,#26374,#26375,#26376,
#26377,#26378,#26379,#26380,#26381,#26382,#26383,#26384,#26385,#26386,#26387,
#26388,#26389),.UNSPECIFIED.,.F.,.F.,(4,3,3,3,3,3,3,3,3,3,3,3,3,3,3,3,3,
3,3,3,3,3,3,3,4),(-12.8459374789857,-11.4794095507986,-10.796145586705,
-10.3238102635133,-10.1128816226115,-9.79002512908185,-7.17546444721137,
-5.86818410627612,-5.2145439358085,-4.88772385057469,-4.68535987579906,
-4.56090376534088,-4.42075803995232,-3.48474489272658,-2.76035534392023,
-2.17493233268704,-1.74712655326145,-1.70292711374347,-1.28137423833848,
-0.996111179633947,-0.765912925479577,-0.547442578207388,-0.286906424613283,
-0.136326843593936,-0.0501381164492949),.UNSPECIFIED.);
#3799=B_SPLINE_CURVE_WITH_KNOTS('',3,(#26391,#26392,#26393,#26394,#26395,
#26396),.UNSPECIFIED.,.F.,.F.,(4,2,4),(-0.993618385713603,-0.861681629743273,
-0.625529516371081),.UNSPECIFIED.);
#3800=B_SPLINE_CURVE_WITH_KNOTS('',3,(#26398,#26399,#26400,#26401,#26402,
#26403,#26404,#26405,#26406,#26407,#26408,#26409,#26410,#26411,#26412,#26413,
#26414,#26415,#26416,#26417,#26418,#26419,#26420,#26421,#26422,#26423,#26424,
#26425,#26426,#26427,#26428,#26429,#26430,#26431,#26432,#26433,#26434,#26435,
#26436,#26437,#26438,#26439,#26440,#26441,#26442,#26443,#26444,#26445,#26446,
#26447,#26448,#26449,#26450,#26451,#26452,#26453,#26454,#26455,#26456,#26457,
#26458,#26459,#26460,#26461,#26462,#26463,#26464),.UNSPECIFIED.,.F.,.F.,
(4,3,3,3,3,3,3,3,3,3,3,3,3,3,3,3,3,3,3,3,3,3,4),(-7.28045043097374,-7.10146924946984,
-5.58665127066262,-5.3505385238982,-5.18292571334222,-4.9351899570797,-4.5984725461592,
-4.20592684613719,-3.66025783532649,-3.1663585345898,-2.76138423986509,
-2.3198751773955,-2.01230406722963,-1.72292916437289,-1.60295645910747,
-1.18526991657213,-0.932600063393711,-0.806265136804503,-0.720980394315423,
-0.679930210215295,-0.615963294358323,-0.164312231362043,0.),
 .UNSPECIFIED.);
#3801=B_SPLINE_CURVE_WITH_KNOTS('',3,(#26468,#26469,#26470,#26471),
 .UNSPECIFIED.,.F.,.F.,(4,4),(-0.123320533354413,0.),.UNSPECIFIED.);
#3802=B_SPLINE_CURVE_WITH_KNOTS('',3,(#26473,#26474,#26475,#26476),
 .UNSPECIFIED.,.F.,.F.,(4,4),(-1.0626156692464,-0.306410932880038),
 .UNSPECIFIED.);
#3803=B_SPLINE_CURVE_WITH_KNOTS('',3,(#26478,#26479,#26480,#26481),
 .UNSPECIFIED.,.F.,.F.,(4,4),(-0.123345114071708,0.),.UNSPECIFIED.);
#3804=B_SPLINE_CURVE_WITH_KNOTS('',3,(#26485,#26486,#26487,#26488,#26489,
#26490,#26491,#26492,#26493,#26494,#26495,#26496,#26497,#26498,#26499,#26500,
#26501,#26502,#26503,#26504,#26505,#26506,#26507,#26508,#26509,#26510,#26511,
#26512,#26513,#26514,#26515,#26516,#26517,#26518,#26519,#26520,#26521,#26522,
#26523,#26524,#26525,#26526,#26527,#26528,#26529,#26530,#26531,#26532,#26533,
#26534,#26535,#26536,#26537,#26538,#26539,#26540,#26541,#26542,#26543,#26544,
#26545,#26546,#26547,#26548,#26549,#26550,#26551,#26552,#26553,#26554,#26555,
#26556,#26557),.UNSPECIFIED.,.F.,.F.,(4,3,3,3,3,3,3,3,3,3,3,3,3,3,3,3,3,
3,3,3,3,3,3,3,4),(-12.8459374978601,-11.4794095665157,-10.7961456008435,
-10.3238102765321,-10.1128816351713,-9.79002514084029,-7.17546445308554,
-5.86818410920817,-5.21454393726949,-4.88772385130015,-4.68535987641399,
-4.5609037653308,-4.42075804013772,-3.48474489292319,-2.76035534391119,
-2.1749323326717,-1.74712655332877,-1.70292711374094,-1.28137423833841,
-0.996111179634097,-0.765912925479675,-0.547442578207446,-0.286906424613297,
-0.13632684359409,-0.050138116449294),.UNSPECIFIED.);
#3805=B_SPLINE_CURVE_WITH_KNOTS('',3,(#26559,#26560,#26561,#26562,#26563,
#26564),.UNSPECIFIED.,.F.,.F.,(4,2,4),(-0.562962425256162,-0.401675631762059,
-0.194993927866297),.UNSPECIFIED.);
#3806=B_SPLINE_CURVE_WITH_KNOTS('',3,(#26565,#26566,#26567,#26568,#26569,
#26570,#26571,#26572,#26573,#26574,#26575,#26576,#26577,#26578,#26579,#26580,
#26581,#26582,#26583,#26584,#26585,#26586,#26587,#26588,#26589),
 .UNSPECIFIED.,.F.,.F.,(4,3,3,3,3,3,3,3,4),(-7.28045042871898,-7.10146924723026,
-5.58665126861639,-5.35053852188943,-5.18292571148688,-4.93518995528529,
-4.59847254446614,-4.20592684453517,-4.02394626436512),.UNSPECIFIED.);
#3807=B_SPLINE_CURVE_WITH_KNOTS('',3,(#26595,#26596,#26597,#26598,#26599,
#26600),.UNSPECIFIED.,.F.,.F.,(4,1,1,4),(109.955742875643,110.793237955343,
111.785020006418,112.692634884417),.UNSPECIFIED.);
#3808=B_SPLINE_CURVE_WITH_KNOTS('',3,(#26603,#26604,#26605,#26606,#26607),
 .UNSPECIFIED.,.F.,.F.,(4,1,4),(109.955742875643,110.461935712833,111.453717763908),
 .UNSPECIFIED.);
#3809=B_SPLINE_CURVE_WITH_KNOTS('',3,(#26612,#26613,#26614,#26615,#26616,
#26617,#26618,#26619,#26620,#26621,#26622),.UNSPECIFIED.,.F.,.F.,(4,1,1,
1,1,1,1,1,4),(103.672557568463,103.850763597816,104.842545648891,105.834327699966,
106.826109751042,107.817891802117,108.809673853192,109.801455904267,109.955742875643),
 .UNSPECIFIED.);
#3810=B_SPLINE_CURVE_WITH_KNOTS('',3,(#26623,#26624,#26625,#26626,#26627,
#26628,#26629,#26630,#26631,#26632),.UNSPECIFIED.,.F.,.F.,(4,1,1,1,1,1,
1,4),(103.672557568463,104.511243406382,105.503025457457,106.494807508532,
107.486589559607,108.478371610683,109.470153661758,109.955742875643),
 .UNSPECIFIED.);
#3811=B_SPLINE_CURVE_WITH_KNOTS('',3,(#26637,#26638,#26639,#26640,#26641,
#26642,#26643,#26644,#26645,#26646),.UNSPECIFIED.,.F.,.F.,(4,1,1,1,1,1,
1,4),(97.3893722612835,97.9000712913645,98.8918533424397,99.883635393515,
100.87541744459,101.867199495665,102.858981546741,103.672557568463),
 .UNSPECIFIED.);
#3812=B_SPLINE_CURVE_WITH_KNOTS('',3,(#26647,#26648,#26649,#26650,#26651,
#26652,#26653,#26654,#26655,#26656,#26657),.UNSPECIFIED.,.F.,.F.,(4,1,1,
1,1,1,1,1,4),(97.3893722612835,97.568769048855,98.5605510999303,99.5523331510055,
100.544115202081,101.535897253156,102.527679304231,103.519461355306,103.672557568463),
 .UNSPECIFIED.);
#3813=B_SPLINE_CURVE_WITH_KNOTS('',3,(#26662,#26663,#26664,#26665,#26666,
#26667,#26668,#26669,#26670,#26671),.UNSPECIFIED.,.F.,.F.,(4,1,1,1,1,1,
1,4),(91.106186954104,91.949378984913,92.9411610359883,93.9329430870635,
94.9247251381387,95.916507189214,96.9082892402892,97.3893722612835),
 .UNSPECIFIED.);
#3814=B_SPLINE_CURVE_WITH_KNOTS('',3,(#26672,#26673,#26674,#26675,#26676,
#26677,#26678,#26679,#26680,#26681),.UNSPECIFIED.,.F.,.F.,(4,1,1,1,1,1,
1,4),(91.106186954104,91.6180767424036,92.6098587934788,93.601640844554,
94.5934228956293,95.5852049467045,96.5769869977798,97.3893722612835),
 .UNSPECIFIED.);
#3815=B_SPLINE_CURVE_WITH_KNOTS('',3,(#26686,#26687,#26688,#26689,#26690,
#26691,#26692,#26693,#26694,#26695,#26696),.UNSPECIFIED.,.F.,.F.,(4,1,1,
1,1,1,1,1,4),(84.8230016469244,85.0069046273863,85.9986866784616,86.9904687295368,
87.9822507806121,88.9740328316873,89.9658148827625,90.9575969338378,91.106186954104),
 .UNSPECIFIED.);
#3816=B_SPLINE_CURVE_WITH_KNOTS('',3,(#26697,#26698,#26699,#26700,#26701,
#26702,#26703,#26704,#26705,#26706),.UNSPECIFIED.,.F.,.F.,(4,1,1,1,1,1,
1,4),(84.8230016469244,85.6673844359521,86.6591664870274,87.6509485381026,
88.6427305891778,89.6345126402531,90.6262946913283,91.106186954104),
 .UNSPECIFIED.);
#3817=B_SPLINE_CURVE_WITH_KNOTS('',3,(#26711,#26712,#26713,#26714,#26715,
#26716,#26717,#26718,#26719,#26720),.UNSPECIFIED.,.F.,.F.,(4,1,1,1,1,1,
1,4),(78.5398163397447,79.0562123209349,80.0479943720101,81.0397764230854,
82.0315584741606,83.0233405252359,84.0151225763111,84.8230016469244),
 .UNSPECIFIED.);
#3818=B_SPLINE_CURVE_WITH_KNOTS('',3,(#26721,#26722,#26723,#26724,#26725,
#26726,#26727,#26728,#26729,#26730,#26731),.UNSPECIFIED.,.F.,.F.,(4,1,1,
1,1,1,1,1,4),(78.5398163397447,78.7249100784254,79.7166921295007,80.7084741805759,
81.7002562316512,82.6920382827264,83.6838203338016,84.6756023848769,84.8230016469244),
 .UNSPECIFIED.);
#3819=B_SPLINE_CURVE_WITH_KNOTS('',3,(#26736,#26737,#26738,#26739,#26740,
#26741,#26742,#26743,#26744,#26745),.UNSPECIFIED.,.F.,.F.,(4,1,1,1,1,1,
1,4),(72.2566310325653,73.1055200144834,74.0973020655587,75.0890841166339,
76.0808661677092,77.0726482187844,78.0644302698597,78.5398163397447),
 .UNSPECIFIED.);
#3820=B_SPLINE_CURVE_WITH_KNOTS('',3,(#26746,#26747,#26748,#26749,#26750,
#26751,#26752,#26753,#26754,#26755),.UNSPECIFIED.,.F.,.F.,(4,1,1,1,1,1,
1,4),(72.2566310325653,72.774217771974,73.7659998230492,74.7577818741245,
75.7495639251997,76.741345976275,77.7331280273502,78.5398163397447),
 .UNSPECIFIED.);
#3821=B_SPLINE_CURVE_WITH_KNOTS('',3,(#26760,#26761,#26762,#26763,#26764,
#26765,#26766,#26767,#26768,#26769,#26770),.UNSPECIFIED.,.F.,.F.,(4,1,1,
1,1,1,1,1,4),(65.9734457253856,66.1630456569568,67.154827708032,68.1466097591072,
69.1383918101825,70.1301738612577,71.121955912333,72.1137379634082,72.2566310325653),
 .UNSPECIFIED.);
#3822=B_SPLINE_CURVE_WITH_KNOTS('',3,(#26771,#26772,#26773,#26774,#26775,
#26776,#26777,#26778,#26779,#26780),.UNSPECIFIED.,.F.,.F.,(4,1,1,1,1,1,
1,4),(65.9734457253856,66.8235254655226,67.8153075165978,68.807089567673,
69.7988716187483,70.7906536698235,71.7824357208987,72.2566310325653),
 .UNSPECIFIED.);
#3823=B_SPLINE_CURVE_WITH_KNOTS('',3,(#26785,#26786,#26787,#26788,#26789,
#26790,#26791,#26792,#26793,#26794),.UNSPECIFIED.,.F.,.F.,(4,1,1,1,1,1,
1,4),(59.6902604182061,60.2123533505053,61.2041354015806,62.1959174526558,
63.187699503731,64.1794815548063,65.1712636058815,65.9734457253856),
 .UNSPECIFIED.);
#3824=B_SPLINE_CURVE_WITH_KNOTS('',3,(#26795,#26796,#26797,#26798,#26799,
#26800,#26801,#26802,#26803,#26804,#26805),.UNSPECIFIED.,.F.,.F.,(4,1,1,
1,1,1,1,1,4),(59.6902604182059,59.8810511079959,60.8728331590711,61.8646152101463,
62.8563972612216,63.8481793122968,64.8399613633721,65.8317434144473,65.9734457253856),
 .UNSPECIFIED.);
#3825=B_SPLINE_CURVE_WITH_KNOTS('',3,(#26810,#26811,#26812,#26813,#26814,
#26815,#26816,#26817,#26818,#26819),.UNSPECIFIED.,.F.,.F.,(4,1,1,1,1,1,
1,4),(53.4070751110265,54.2616610440539,55.2534430951291,56.2452251462044,
57.2370071972796,58.2287892483548,59.2205712994301,59.6902604182061),
 .UNSPECIFIED.);
#3826=B_SPLINE_CURVE_WITH_KNOTS('',3,(#26820,#26821,#26822,#26823,#26824,
#26825,#26826,#26827,#26828,#26829),.UNSPECIFIED.,.F.,.F.,(4,1,1,1,1,1,
1,4),(53.4070751110265,53.9303588015444,54.9221408526197,55.9139229036949,
56.9057049547701,57.8974870058454,58.8892690569206,59.6902604182059),
 .UNSPECIFIED.);
#3827=B_SPLINE_CURVE_WITH_KNOTS('',3,(#26834,#26835,#26836,#26837,#26838,
#26839,#26840,#26841,#26842,#26843,#26844),.UNSPECIFIED.,.F.,.F.,(4,1,1,
1,1,1,1,1,4),(47.1238898038468,47.3191866865272,48.3109687376024,49.3027507886777,
50.2945328397529,51.2863148908282,52.2780969419034,53.2698789929786,53.4070751110265),
 .UNSPECIFIED.);
#3828=B_SPLINE_CURVE_WITH_KNOTS('',3,(#26845,#26846,#26847,#26848,#26849,
#26850,#26851,#26852,#26853,#26854),.UNSPECIFIED.,.F.,.F.,(4,1,1,1,1,1,
1,4),(47.1238898038468,47.979666495093,48.9714485461682,49.9632305972435,
50.9550126483187,51.9467946993939,52.9385767504692,53.4070751110265),
 .UNSPECIFIED.);
#3829=B_SPLINE_CURVE_WITH_KNOTS('',3,(#26859,#26860,#26861,#26862,#26863,
#26864,#26865,#26866,#26867,#26868),.UNSPECIFIED.,.F.,.F.,(4,1,1,1,1,1,
1,4),(40.8407044966673,41.3684943800758,42.360276431151,43.3520584822262,
44.3438405333015,45.3356225843767,46.327404635452,47.1238898038468),
 .UNSPECIFIED.);
#3830=B_SPLINE_CURVE_WITH_KNOTS('',3,(#26869,#26870,#26871,#26872,#26873,
#26874,#26875,#26876,#26877,#26878,#26879),.UNSPECIFIED.,.F.,.F.,(4,1,1,
1,1,1,1,1,4),(40.8407044966673,41.0371921375663,42.0289741886415,43.0207562397168,
44.012538290792,45.0043203418673,45.9961023929425,46.9878844440177,47.1238898038468),
 .UNSPECIFIED.);
#3831=B_SPLINE_CURVE_WITH_KNOTS('',3,(#26884,#26885,#26886,#26887,#26888,
#26889,#26890,#26891,#26892,#26893),.UNSPECIFIED.,.F.,.F.,(4,1,1,1,1,1,
1,4),(34.5575191894877,35.4178020736243,36.4095841246995,37.4013661757748,
38.39314822685,39.3849302779253,40.3767123290005,40.8407044966673),
 .UNSPECIFIED.);
#3832=B_SPLINE_CURVE_WITH_KNOTS('',3,(#26894,#26895,#26896,#26897,#26898,
#26899,#26900,#26901,#26902,#26903),.UNSPECIFIED.,.F.,.F.,(4,1,1,1,1,1,
1,4),(34.5575191894877,35.0864998311148,36.0782818821901,37.0700639332653,
38.0618459843406,39.0536280354158,40.0454100864911,40.8407044966673),
 .UNSPECIFIED.);
#3833=B_SPLINE_CURVE_WITH_KNOTS('',3,(#26908,#26909,#26910,#26911,#26912,
#26913,#26914,#26915,#26916,#26917,#26918),.UNSPECIFIED.,.F.,.F.,(4,1,1,
1,1,1,1,1,4),(28.2743338823081,28.4753277160976,29.4671097671729,30.4588918182481,
31.4506738693233,32.4424559203986,33.4342379714738,34.4260200225491,34.5575191894877),
 .UNSPECIFIED.);
#3834=B_SPLINE_CURVE_WITH_KNOTS('',3,(#26919,#26920,#26921,#26922,#26923,
#26924,#26925,#26926,#26927,#26928),.UNSPECIFIED.,.F.,.F.,(4,1,1,1,1,1,
1,4),(28.2743338823081,29.1358075246634,30.1275895757386,31.1193716268139,
32.1111536778891,33.1029357289644,34.0947177800396,34.5575191894877),
 .UNSPECIFIED.);
#3835=B_SPLINE_CURVE_WITH_KNOTS('',3,(#26933,#26934,#26935,#26936,#26937,
#26938,#26939,#26940,#26941,#26942),.UNSPECIFIED.,.F.,.F.,(4,1,1,1,1,1,
1,4),(21.9911485751285,22.5246354096462,23.5164174607214,24.5081995117967,
25.4999815628719,26.4917636139471,27.4835456650224,28.2743338823081),
 .UNSPECIFIED.);
#3836=B_SPLINE_CURVE_WITH_KNOTS('',3,(#26943,#26944,#26945,#26946,#26947,
#26948,#26949,#26950,#26951,#26952,#26953),.UNSPECIFIED.,.F.,.F.,(4,1,1,
1,1,1,1,1,4),(21.9911485751284,22.1933331671367,23.185115218212,24.1768972692872,
25.1686793203624,26.1604613714377,27.1522434225129,28.1440254735882,28.2743338823081),
 .UNSPECIFIED.);
#3837=B_SPLINE_CURVE_WITH_KNOTS('',3,(#26958,#26959,#26960,#26961,#26962,
#26963,#26964,#26965,#26966,#26967),.UNSPECIFIED.,.F.,.F.,(4,1,1,1,1,1,
1,4),(15.7079632679489,16.5739431031947,17.56572515427,18.5575072053452,
19.5492892564205,20.5410713074957,21.5328533585709,21.9911485751285),
 .UNSPECIFIED.);
#3838=B_SPLINE_CURVE_WITH_KNOTS('',3,(#26968,#26969,#26970,#26971,#26972,
#26973,#26974,#26975,#26976,#26977),.UNSPECIFIED.,.F.,.F.,(4,1,1,1,1,1,
1,4),(15.7079632679489,16.2426408606853,17.2344229117605,18.2262049628358,
19.217987013911,20.2097690649862,21.2015511160615,21.9911485751284),
 .UNSPECIFIED.);
#3839=B_SPLINE_CURVE_WITH_KNOTS('',3,(#27305,#27306,#27307,#27308),
 .UNSPECIFIED.,.F.,.F.,(4,4),(-0.0707400283740946,0.),.UNSPECIFIED.);
#3840=B_SPLINE_CURVE_WITH_KNOTS('',3,(#27312,#27313,#27314,#27315),
 .UNSPECIFIED.,.F.,.F.,(4,4),(-0.070743295445964,-3.34525766250426E-6),
 .UNSPECIFIED.);
#3841=B_SPLINE_CURVE_WITH_KNOTS('',3,(#27319,#27320,#27321,#27322,#27323,
#27324,#27325,#27326,#27327,#27328,#27329,#27330,#27331,#27332,#27333,#27334,
#27335,#27336,#27337,#27338,#27339,#27340,#27341,#27342,#27343,#27344,#27345,
#27346,#27347,#27348,#27349,#27350,#27351,#27352,#27353,#27354,#27355,#27356,
#27357,#27358,#27359,#27360,#27361,#27362,#27363,#27364,#27365,#27366,#27367,
#27368,#27369,#27370,#27371,#27372,#27373,#27374,#27375,#27376,#27377,#27378,
#27379,#27380,#27381,#27382,#27383,#27384,#27385,#27386,#27387,#27388,#27389,
#27390,#27391,#27392,#27393,#27394,#27395,#27396,#27397,#27398,#27399,#27400,
#27401,#27402,#27403,#27404,#27405,#27406,#27407,#27408,#27409,#27410,#27411,
#27412,#27413,#27414,#27415),.UNSPECIFIED.,.F.,.F.,(4,3,3,3,3,3,3,3,3,3,
3,3,3,3,3,3,3,3,3,3,3,3,3,3,3,3,3,3,3,3,3,3,4),(-0.461463988274541,-0.386087506167661,
-0.375299929924104,-0.372903671306323,-0.356077696752448,-0.352040116130794,
-0.339920267375323,-0.338448280177947,-0.326632246672126,-0.313204943761465,
-0.304885949019545,-0.29982124014814,-0.293952204614803,-0.287658393406508,
-0.282882239837598,-0.277507204165034,-0.271689255077659,-0.265572046854325,
-0.25886897335232,-0.254459737762025,-0.241918019250842,-0.227822266677633,
-0.212603244487136,-0.196183063900822,-0.178197554741815,-0.159751102176233,
-0.141758270371077,-0.134249918117004,-0.101233605562941,-0.0682193757072185,
-0.0525746845214139,-0.0245175806023845,0.),.UNSPECIFIED.);
#3842=B_SPLINE_CURVE_WITH_KNOTS('',3,(#27418,#27419,#27420,#27421,#27422,
#27423,#27424,#27425,#27426,#27427,#27428,#27429,#27430,#27431,#27432,#27433,
#27434,#27435,#27436,#27437,#27438,#27439,#27440,#27441,#27442,#27443,#27444,
#27445,#27446,#27447,#27448,#27449,#27450,#27451,#27452,#27453,#27454,#27455,
#27456,#27457,#27458,#27459,#27460,#27461,#27462,#27463,#27464,#27465,#27466,
#27467,#27468,#27469,#27470,#27471,#27472,#27473,#27474,#27475,#27476,#27477,
#27478,#27479,#27480,#27481),.UNSPECIFIED.,.F.,.F.,(4,3,3,3,3,3,3,3,3,3,
3,3,3,3,3,3,3,3,3,3,3,4),(-0.976443208995993,-0.95964177146371,-0.949661288965092,
-0.932500795758735,-0.914975318862148,-0.904644103415597,-0.893689140152817,
-0.881835075865292,-0.868593367676957,-0.854447019507673,-0.839440732702782,
-0.82369847533003,-0.808085046250858,-0.793464970995011,-0.790720555879271,
-0.779060485592236,-0.740625,-0.691250000000001,-0.5925,-0.543125,-0.395,
-0.049999999999998),.UNSPECIFIED.);
#3843=B_SPLINE_CURVE_WITH_KNOTS('',3,(#27693,#27694,#27695,#27696),
 .UNSPECIFIED.,.F.,.F.,(4,4),(-0.253410853624616,-0.103262412077185),
 .UNSPECIFIED.);
#3844=B_SPLINE_CURVE_WITH_KNOTS('',3,(#27698,#27699,#27700,#27701),
 .UNSPECIFIED.,.F.,.F.,(4,4),(0.,0.29),.UNSPECIFIED.);
#3845=B_SPLINE_CURVE_WITH_KNOTS('',3,(#27703,#27704,#27705,#27706),
 .UNSPECIFIED.,.F.,.F.,(4,4),(3.28350553677514,3.37607250270485),
 .UNSPECIFIED.);
#3846=B_SPLINE_CURVE_WITH_KNOTS('',3,(#27707,#27708,#27709,#27710,#27711,
#27712,#27713,#27714,#27715,#27716,#27717,#27718,#27719,#27720,#27721,#27722,
#27723,#27724,#27725,#27726,#27727,#27728,#27729,#27730,#27731,#27732,#27733,
#27734,#27735,#27736,#27737,#27738,#27739,#27740,#27741,#27742,#27743,#27744,
#27745,#27746,#27747,#27748,#27749,#27750,#27751,#27752),.UNSPECIFIED.,
 .F.,.F.,(4,3,3,3,3,3,3,3,3,3,3,3,3,3,3,4),(-4.02394626436512,-3.66025783388072,
-3.16634870316095,-2.76138423897494,-2.31987517666077,-2.01230406657675,
-1.72292916396621,-1.60295645875968,-1.18526991637693,-0.932600063295131,
-0.806265136754233,-0.720980394265897,-0.679930210213335,-0.615963294332911,
-0.164312231367537,0.),.UNSPECIFIED.);
#3847=B_SPLINE_CURVE_WITH_KNOTS('',3,(#27754,#27755,#27756,#27757,#27758,
#27759),.UNSPECIFIED.,.F.,.F.,(4,2,4),(-2.17700203273975,-1.38478587807843,
-0.288632999074765),.UNSPECIFIED.);
#3848=B_SPLINE_CURVE_WITH_KNOTS('',3,(#27761,#27762,#27763,#27764,#27765,
#27766,#27767,#27768,#27769,#27770,#27771,#27772,#27773,#27774,#27775,#27776,
#27777,#27778,#27779,#27780,#27781,#27782,#27783,#27784,#27785,#27786,#27787,
#27788,#27789,#27790,#27791),.UNSPECIFIED.,.F.,.F.,(4,3,3,3,3,3,3,3,3,3,
4),(0.664704897780732,0.688351938092992,0.78031723869645,0.810486879810963,
0.862717972416633,0.955520663501275,1.01466394039964,1.06038302616807,1.10529572457683,
1.13272802062135,1.20216888729732),.UNSPECIFIED.);
#3849=B_SPLINE_CURVE_WITH_KNOTS('',3,(#27792,#27793,#27794,#27795,#27796,
#27797,#27798,#27799,#27800,#27801,#27802,#27803,#27804,#27805,#27806,#27807,
#27808,#27809,#27810),.UNSPECIFIED.,.F.,.F.,(4,3,3,3,3,3,4),(0.,0.178790961538472,
0.350742859481108,0.449205432353047,0.513879914408645,0.522694757423744,
0.664704897780732),.UNSPECIFIED.);
#3850=B_SPLINE_CURVE_WITH_KNOTS('',3,(#27814,#27815,#27816,#27817),
 .UNSPECIFIED.,.F.,.F.,(4,4),(-0.0707400282910659,0.),.UNSPECIFIED.);
#3851=B_SPLINE_CURVE_WITH_KNOTS('',3,(#27821,#27822,#27823,#27824),
 .UNSPECIFIED.,.F.,.F.,(4,4),(-0.0707432948545235,-3.34525766380878E-6),
 .UNSPECIFIED.);
#3852=B_SPLINE_CURVE_WITH_KNOTS('',3,(#27828,#27829,#27830,#27831,#27832,
#27833,#27834,#27835,#27836,#27837,#27838,#27839,#27840,#27841,#27842,#27843,
#27844,#27845,#27846,#27847,#27848,#27849,#27850,#27851,#27852,#27853,#27854,
#27855,#27856,#27857,#27858,#27859,#27860,#27861,#27862,#27863,#27864,#27865,
#27866,#27867,#27868,#27869,#27870,#27871,#27872,#27873,#27874,#27875,#27876,
#27877,#27878,#27879,#27880,#27881,#27882,#27883,#27884,#27885,#27886,#27887,
#27888,#27889,#27890,#27891,#27892,#27893,#27894,#27895,#27896,#27897,#27898,
#27899,#27900,#27901,#27902,#27903,#27904,#27905,#27906,#27907,#27908,#27909,
#27910,#27911,#27912,#27913,#27914,#27915,#27916,#27917,#27918),
 .UNSPECIFIED.,.F.,.F.,(4,3,3,3,3,3,3,3,3,3,3,3,3,3,3,3,3,3,3,3,3,3,3,3,
3,3,3,3,3,3,4),(-0.461463988274541,-0.386087506167661,-0.372903671306323,
-0.36421409612757,-0.352528758081246,-0.339636892136157,-0.338448280177947,
-0.328074919236012,-0.316383789572668,-0.304885949019545,-0.297243973048271,
-0.288858567477107,-0.282882239837598,-0.277347677282806,-0.271340988166504,
-0.265007390818464,-0.258044852490757,-0.254459737762025,-0.242044020405013,
-0.228141105146501,-0.213185106576004,-0.197120884701682,-0.179636878474788,
-0.161760929349414,-0.144350238406641,-0.134249918117004,-0.102125955921634,
-0.0702664487997089,-0.0525746845214139,-0.02166066501539,0.),
 .UNSPECIFIED.);
#3853=B_SPLINE_CURVE_WITH_KNOTS('',3,(#27921,#27922,#27923,#27924,#27925,
#27926,#27927,#27928,#27929,#27930,#27931,#27932,#27933,#27934,#27935,#27936,
#27937,#27938,#27939,#27940,#27941,#27942,#27943,#27944,#27945,#27946,#27947,
#27948,#27949,#27950,#27951,#27952,#27953,#27954,#27955,#27956,#27957,#27958,
#27959,#27960,#27961,#27962,#27963,#27964,#27965,#27966,#27967,#27968,#27969,
#27970,#27971,#27972,#27973,#27974,#27975,#27976,#27977,#27978,#27979,#27980,
#27981,#27982,#27983,#27984),.UNSPECIFIED.,.F.,.F.,(4,3,3,3,3,3,3,3,3,3,
3,3,3,3,3,3,3,3,3,3,3,4),(-0.976443208995993,-0.960629666524146,-0.949661288965092,
-0.931972270488235,-0.914398186943459,-0.904644103415597,-0.893317754842137,
-0.880493104971779,-0.866940956882255,-0.85260546798694,-0.837134239960023,
-0.82157385570265,-0.80614720579096,-0.79187466047125,-0.790720555879271,
-0.779060485592236,-0.740625,-0.691250000000001,-0.5925,-0.49375,-0.394999999999999,
-0.0499999999999998),.UNSPECIFIED.);
#3854=B_SPLINE_CURVE_WITH_KNOTS('',3,(#28176,#28177,#28178,#28179),
 .UNSPECIFIED.,.F.,.F.,(4,4),(-0.253410853624616,-0.103262412077185),
 .UNSPECIFIED.);
#3855=B_SPLINE_CURVE_WITH_KNOTS('',3,(#28181,#28182,#28183,#28184),
 .UNSPECIFIED.,.F.,.F.,(4,4),(0.,0.29),.UNSPECIFIED.);
#3856=B_SPLINE_CURVE_WITH_KNOTS('',3,(#28185,#28186,#28187,#28188),
 .UNSPECIFIED.,.F.,.F.,(4,4),(3.28350553660553,3.37607250252489),
 .UNSPECIFIED.);
#3857=B_SPLINE_CURVE_WITH_KNOTS('',3,(#28190,#28191,#28192,#28193,#28194,
#28195),.UNSPECIFIED.,.F.,.F.,(4,2,4),(-2.17700203273975,-1.38478587807843,
-0.288632999074765),.UNSPECIFIED.);
#3858=B_SPLINE_CURVE_WITH_KNOTS('',3,(#28197,#28198,#28199,#28200,#28201,
#28202,#28203,#28204,#28205,#28206,#28207,#28208,#28209,#28210,#28211,#28212,
#28213,#28214,#28215,#28216,#28217,#28218,#28219,#28220,#28221,#28222,#28223,
#28224,#28225,#28226,#28227),.UNSPECIFIED.,.F.,.F.,(4,3,3,3,3,3,3,3,3,3,
4),(0.664704897780732,0.688351938092992,0.780317238696425,0.810486879810963,
0.862717972416611,0.955520663501275,1.01466394039954,1.06038302616807,1.10529572457683,
1.13272802062135,1.20216888729732),.UNSPECIFIED.);
#3859=B_SPLINE_CURVE_WITH_KNOTS('',3,(#28228,#28229,#28230,#28231,#28232,
#28233,#28234,#28235,#28236,#28237,#28238,#28239,#28240,#28241,#28242,#28243,
#28244,#28245,#28246),.UNSPECIFIED.,.F.,.F.,(4,3,3,3,3,3,4),(0.,0.178790961538472,
0.350742859481108,0.449205432353048,0.513879914408647,0.522694757423744,
0.664704897780732),.UNSPECIFIED.);
#3860=B_SPLINE_CURVE_WITH_KNOTS('',3,(#28250,#28251,#28252,#28253),
 .UNSPECIFIED.,.F.,.F.,(4,4),(-0.0707400285408625,0.),.UNSPECIFIED.);
#3861=B_SPLINE_CURVE_WITH_KNOTS('',3,(#28257,#28258,#28259,#28260),
 .UNSPECIFIED.,.F.,.F.,(4,4),(-0.0707432954689054,-3.34525766178262E-6),
 .UNSPECIFIED.);
#3862=B_SPLINE_CURVE_WITH_KNOTS('',3,(#28264,#28265,#28266,#28267,#28268,
#28269,#28270,#28271,#28272,#28273,#28274,#28275,#28276,#28277,#28278,#28279,
#28280,#28281,#28282,#28283,#28284,#28285,#28286,#28287,#28288,#28289,#28290,
#28291,#28292,#28293,#28294,#28295,#28296,#28297,#28298,#28299,#28300,#28301,
#28302,#28303,#28304,#28305,#28306,#28307,#28308,#28309,#28310,#28311,#28312,
#28313,#28314,#28315,#28316,#28317,#28318,#28319,#28320,#28321,#28322,#28323,
#28324,#28325,#28326,#28327,#28328,#28329,#28330,#28331,#28332,#28333,#28334,
#28335,#28336,#28337,#28338,#28339,#28340,#28341,#28342,#28343,#28344,#28345,
#28346,#28347,#28348,#28349,#28350,#28351,#28352,#28353,#28354,#28355,#28356,
#28357,#28358,#28359,#28360),.UNSPECIFIED.,.F.,.F.,(4,3,3,3,3,3,3,3,3,3,
3,3,3,3,3,3,3,3,3,3,3,3,3,3,3,3,3,3,3,3,3,3,4),(-0.461463988274541,-0.386087506167661,
-0.372903671306323,-0.36421409612757,-0.349922618618476,-0.338448280177947,
-0.328550793223587,-0.322977024945215,-0.314822638010309,-0.306007155782235,
-0.304885949019545,-0.297658439870379,-0.289754515056109,-0.282882239837598,
-0.277393071545031,-0.271439067306372,-0.265165133454002,-0.258272116803473,
-0.254459737762025,-0.242193625916565,-0.2284734588626,-0.213717473130501,
-0.197852099811634,-0.180468088683695,-0.162567602548416,-0.144906258984996,
-0.134249918117004,-0.102205018832853,-0.0696974934620852,-0.0525746845214139,
-0.0222228841287548,-0.000827460244363642,0.),.UNSPECIFIED.);
#3863=B_SPLINE_CURVE_WITH_KNOTS('',3,(#28363,#28364,#28365,#28366,#28367,
#28368,#28369,#28370,#28371,#28372,#28373,#28374,#28375,#28376,#28377,#28378,
#28379,#28380,#28381,#28382,#28383,#28384,#28385,#28386,#28387,#28388,#28389,
#28390,#28391,#28392,#28393,#28394,#28395,#28396,#28397,#28398,#28399,#28400,
#28401,#28402,#28403,#28404,#28405,#28406,#28407,#28408,#28409,#28410,#28411,
#28412,#28413,#28414,#28415,#28416,#28417,#28418,#28419,#28420,#28421,#28422,
#28423,#28424,#28425,#28426),.UNSPECIFIED.,.F.,.F.,(4,3,3,3,3,3,3,3,3,3,
3,3,3,3,3,3,3,3,3,3,3,4),(-0.976443208995993,-0.960628704721015,-0.949661288965092,
-0.931975105549615,-0.914400310860217,-0.904644103415597,-0.893320015681317,
-0.880495083206061,-0.866943636882904,-0.852607981525575,-0.837136125113999,
-0.821574066138986,-0.806147311009128,-0.791872999074624,-0.790720555879271,
-0.779060485592236,-0.740625,-0.691250000000001,-0.5925,-0.49375,-0.394999999999999,
-0.0499999999999998),.UNSPECIFIED.);
#3864=B_SPLINE_CURVE_WITH_KNOTS('',3,(#28648,#28649,#28650,#28651),
 .UNSPECIFIED.,.F.,.F.,(4,4),(-0.253410853624616,-0.103262412077186),
 .UNSPECIFIED.);
#3865=B_SPLINE_CURVE_WITH_KNOTS('',3,(#28653,#28654,#28655,#28656),
 .UNSPECIFIED.,.F.,.F.,(4,4),(0.,0.29),.UNSPECIFIED.);
#3866=B_SPLINE_CURVE_WITH_KNOTS('',3,(#28657,#28658,#28659,#28660),
 .UNSPECIFIED.,.F.,.F.,(4,4),(3.28350553660308,3.37607250251481),
 .UNSPECIFIED.);
#3867=B_SPLINE_CURVE_WITH_KNOTS('',3,(#28662,#28663,#28664,#28665,#28666,
#28667),.UNSPECIFIED.,.F.,.F.,(4,2,4),(-2.17700203273975,-1.38478587807843,
-0.288632999074765),.UNSPECIFIED.);
#3868=B_SPLINE_CURVE_WITH_KNOTS('',3,(#28669,#28670,#28671,#28672,#28673,
#28674,#28675,#28676,#28677,#28678,#28679,#28680,#28681,#28682,#28683,#28684,
#28685,#28686,#28687,#28688,#28689,#28690,#28691,#28692,#28693,#28694,#28695,
#28696,#28697,#28698,#28699),.UNSPECIFIED.,.F.,.F.,(4,3,3,3,3,3,3,3,3,3,
4),(0.664704897780732,0.688351938092992,0.780317238696443,0.810486879810963,
0.862717972416633,0.955520663501275,1.0146639403997,1.06038302616807,1.10529572457683,
1.13272802062135,1.20216888729732),.UNSPECIFIED.);
#3869=B_SPLINE_CURVE_WITH_KNOTS('',3,(#28700,#28701,#28702,#28703,#28704,
#28705,#28706,#28707,#28708,#28709,#28710,#28711,#28712,#28713,#28714,#28715,
#28716,#28717,#28718),.UNSPECIFIED.,.F.,.F.,(4,3,3,3,3,3,4),(0.,0.178790961538472,
0.350742859481108,0.449205432353048,0.513879914408647,0.522694757423744,
0.664704897780732),.UNSPECIFIED.);
#3870=B_SPLINE_CURVE_WITH_KNOTS('',3,(#28722,#28723,#28724,#28725),
 .UNSPECIFIED.,.F.,.F.,(4,4),(-0.0707400283740959,0.),.UNSPECIFIED.);
#3871=B_SPLINE_CURVE_WITH_KNOTS('',3,(#28729,#28730,#28731,#28732),
 .UNSPECIFIED.,.F.,.F.,(4,4),(-0.0707432954466584,-3.34525766253202E-6),
 .UNSPECIFIED.);
#3872=B_SPLINE_CURVE_WITH_KNOTS('',3,(#28736,#28737,#28738,#28739,#28740,
#28741,#28742,#28743,#28744,#28745,#28746,#28747,#28748,#28749,#28750,#28751,
#28752,#28753,#28754,#28755,#28756,#28757,#28758,#28759,#28760,#28761,#28762,
#28763,#28764,#28765,#28766,#28767,#28768,#28769,#28770,#28771,#28772,#28773,
#28774,#28775,#28776,#28777,#28778,#28779,#28780,#28781,#28782,#28783,#28784,
#28785,#28786,#28787,#28788,#28789,#28790,#28791,#28792,#28793,#28794,#28795,
#28796,#28797,#28798,#28799,#28800,#28801,#28802,#28803,#28804,#28805,#28806,
#28807,#28808,#28809,#28810,#28811,#28812,#28813,#28814,#28815,#28816,#28817,
#28818,#28819,#28820,#28821,#28822,#28823,#28824,#28825,#28826,#28827,#28828,
#28829,#28830,#28831,#28832),.UNSPECIFIED.,.F.,.F.,(4,3,3,3,3,3,3,3,3,3,
3,3,3,3,3,3,3,3,3,3,3,3,3,3,3,3,3,3,3,3,3,3,4),(-0.461463988274541,-0.386087506167661,
-0.375299929924104,-0.372903671306323,-0.356077696752448,-0.352040116130794,
-0.339920267375323,-0.338448280177947,-0.326632246672124,-0.313204943761436,
-0.304885949019545,-0.29982124014814,-0.293952204614803,-0.287658393406508,
-0.282882239837598,-0.277507204165034,-0.271689255077659,-0.265572046854325,
-0.258868973352318,-0.254459737762025,-0.241918019250842,-0.227822266677611,
-0.212603244487091,-0.196183063900774,-0.178197554741625,-0.159751102176005,
-0.141758270370875,-0.134249918117004,-0.10123360556295,-0.068219375707454,
-0.0525746845214139,-0.0245175806023862,0.),.UNSPECIFIED.);
#3873=B_SPLINE_CURVE_WITH_KNOTS('',3,(#28835,#28836,#28837,#28838,#28839,
#28840,#28841,#28842,#28843,#28844,#28845,#28846,#28847,#28848,#28849,#28850,
#28851,#28852,#28853,#28854,#28855,#28856,#28857,#28858,#28859,#28860,#28861,
#28862,#28863,#28864,#28865,#28866,#28867,#28868,#28869,#28870,#28871,#28872,
#28873,#28874,#28875,#28876,#28877,#28878,#28879,#28880,#28881,#28882,#28883,
#28884,#28885,#28886,#28887,#28888,#28889,#28890,#28891,#28892,#28893,#28894,
#28895,#28896,#28897,#28898),.UNSPECIFIED.,.F.,.F.,(4,3,3,3,3,3,3,3,3,3,
3,3,3,3,3,3,3,3,3,3,3,4),(-0.976443208995993,-0.959642323211355,-0.949661288965092,
-0.932497758133295,-0.914973156724424,-0.904644103415597,-0.893686857853989,
-0.881830566008639,-0.868587665962165,-0.854441220699773,-0.839436072992889,
-0.823696621722087,-0.808086574213453,-0.793469897333356,-0.790720555879271,
-0.779060485592236,-0.740625,-0.691250000000001,-0.5925,-0.543125,-0.394999999999999,
-0.0499999999999998),.UNSPECIFIED.);
#3874=B_SPLINE_CURVE_WITH_KNOTS('',3,(#29110,#29111,#29112,#29113),
 .UNSPECIFIED.,.F.,.F.,(4,4),(-0.253410853624616,-0.103262412077185),
 .UNSPECIFIED.);
#3875=B_SPLINE_CURVE_WITH_KNOTS('',3,(#29115,#29116,#29117,#29118),
 .UNSPECIFIED.,.F.,.F.,(4,4),(0.,0.29),.UNSPECIFIED.);
#3876=B_SPLINE_CURVE_WITH_KNOTS('',3,(#29119,#29120,#29121,#29122),
 .UNSPECIFIED.,.F.,.F.,(4,4),(3.28350553697936,3.37607250293456),
 .UNSPECIFIED.);
#3877=B_SPLINE_CURVE_WITH_KNOTS('',3,(#29124,#29125,#29126,#29127,#29128,
#29129),.UNSPECIFIED.,.F.,.F.,(4,2,4),(-2.17700203273975,-1.38478587807843,
-0.288632999074766),.UNSPECIFIED.);
#3878=B_SPLINE_CURVE_WITH_KNOTS('',3,(#29131,#29132,#29133,#29134,#29135,
#29136,#29137,#29138,#29139,#29140,#29141,#29142,#29143,#29144,#29145,#29146,
#29147,#29148,#29149,#29150,#29151,#29152,#29153,#29154,#29155,#29156,#29157,
#29158,#29159,#29160,#29161),.UNSPECIFIED.,.F.,.F.,(4,3,3,3,3,3,3,3,3,3,
4),(0.664704897780732,0.688351938092992,0.780317238696442,0.810486879810963,
0.862717972416637,0.955520663501275,1.01466394039962,1.06038302616807,1.10529572457683,
1.13272802062135,1.20216888729732),.UNSPECIFIED.);
#3879=B_SPLINE_CURVE_WITH_KNOTS('',3,(#29162,#29163,#29164,#29165,#29166,
#29167,#29168,#29169,#29170,#29171,#29172,#29173,#29174,#29175,#29176,#29177,
#29178,#29179,#29180),.UNSPECIFIED.,.F.,.F.,(4,3,3,3,3,3,4),(0.,0.178790961538472,
0.350742859481108,0.449205432353047,0.513879914408646,0.522694757423744,
0.664704897780732),.UNSPECIFIED.);
#3880=B_SPLINE_CURVE_WITH_KNOTS('',3,(#29184,#29185,#29186,#29187),
 .UNSPECIFIED.,.F.,.F.,(4,4),(-0.070740028353927,0.),.UNSPECIFIED.);
#3881=B_SPLINE_CURVE_WITH_KNOTS('',3,(#29191,#29192,#29193,#29194),
 .UNSPECIFIED.,.F.,.F.,(4,4),(-0.0707432948167915,-3.34525766403082E-6),
 .UNSPECIFIED.);
#3882=B_SPLINE_CURVE_WITH_KNOTS('',3,(#29198,#29199,#29200,#29201,#29202,
#29203,#29204,#29205,#29206,#29207,#29208,#29209,#29210,#29211,#29212,#29213,
#29214,#29215,#29216,#29217,#29218,#29219,#29220,#29221,#29222,#29223,#29224,
#29225,#29226,#29227,#29228,#29229,#29230,#29231,#29232,#29233,#29234,#29235,
#29236,#29237,#29238,#29239,#29240,#29241,#29242,#29243,#29244,#29245,#29246,
#29247,#29248,#29249,#29250,#29251,#29252,#29253,#29254,#29255,#29256,#29257,
#29258,#29259,#29260,#29261,#29262,#29263,#29264,#29265,#29266,#29267,#29268,
#29269,#29270,#29271,#29272,#29273,#29274,#29275,#29276,#29277,#29278,#29279,
#29280,#29281,#29282,#29283,#29284,#29285,#29286,#29287,#29288),
 .UNSPECIFIED.,.F.,.F.,(4,3,3,3,3,3,3,3,3,3,3,3,3,3,3,3,3,3,3,3,3,3,3,3,
3,3,3,3,3,3,4),(-0.461463988274541,-0.386087506167661,-0.372903671306323,
-0.36421409612757,-0.352528758081253,-0.339636892136,-0.338448280177947,
-0.328074919236012,-0.316383789572691,-0.304885949019545,-0.297243973048271,
-0.288858567477107,-0.282882239837598,-0.277347677282806,-0.271340988166504,
-0.265007390818464,-0.258044852490787,-0.254459737762025,-0.242044020405011,
-0.228141105146502,-0.213185106575989,-0.1971208847016,-0.179636878474718,
-0.161760929349413,-0.144350238406588,-0.134249918117004,-0.102125955921634,
-0.070266448799884,-0.0525746845214139,-0.0216606650153916,0.),
 .UNSPECIFIED.);
#3883=B_SPLINE_CURVE_WITH_KNOTS('',3,(#29291,#29292,#29293,#29294,#29295,
#29296,#29297,#29298,#29299,#29300,#29301,#29302,#29303,#29304,#29305,#29306,
#29307,#29308,#29309,#29310,#29311,#29312,#29313,#29314,#29315,#29316,#29317,
#29318,#29319,#29320,#29321,#29322,#29323,#29324,#29325,#29326,#29327,#29328,
#29329,#29330,#29331,#29332,#29333,#29334,#29335,#29336,#29337,#29338,#29339,
#29340,#29341,#29342,#29343,#29344,#29345,#29346,#29347,#29348,#29349,#29350,
#29351,#29352,#29353,#29354),.UNSPECIFIED.,.F.,.F.,(4,3,3,3,3,3,3,3,3,3,
3,3,3,3,3,3,3,3,3,3,3,4),(-0.976443208995993,-0.960629666524142,-0.949661288965092,
-0.931972270488239,-0.91439818694324,-0.904644103415597,-0.893317754842134,
-0.880493104971777,-0.866940956882277,-0.852605467987382,-0.837134239960354,
-0.821573855703088,-0.806147205791179,-0.791874660471442,-0.790720555879271,
-0.779060485592236,-0.740625,-0.691250000000001,-0.5925,-0.49375,-0.394999999999999,
-0.0499999999999998),.UNSPECIFIED.);
#3884=B_SPLINE_CURVE_WITH_KNOTS('',3,(#29546,#29547,#29548,#29549),
 .UNSPECIFIED.,.F.,.F.,(4,4),(-0.253410853624616,-0.103262412077186),
 .UNSPECIFIED.);
#3885=B_SPLINE_CURVE_WITH_KNOTS('',3,(#29551,#29552,#29553,#29554),
 .UNSPECIFIED.,.F.,.F.,(4,4),(0.,0.29),.UNSPECIFIED.);
#3886=B_SPLINE_CURVE_WITH_KNOTS('',3,(#29555,#29556,#29557,#29558),
 .UNSPECIFIED.,.F.,.F.,(4,4),(3.28350553753493,3.3760725035161),
 .UNSPECIFIED.);
#3887=B_SPLINE_CURVE_WITH_KNOTS('',3,(#29560,#29561,#29562,#29563,#29564,
#29565),.UNSPECIFIED.,.F.,.F.,(4,2,4),(-2.17700203273975,-1.38478587807843,
-0.288632999074765),.UNSPECIFIED.);
#3888=B_SPLINE_CURVE_WITH_KNOTS('',3,(#29567,#29568,#29569,#29570,#29571,
#29572,#29573,#29574,#29575,#29576,#29577,#29578,#29579,#29580,#29581,#29582,
#29583,#29584,#29585,#29586,#29587,#29588,#29589,#29590,#29591,#29592,#29593,
#29594,#29595,#29596,#29597),.UNSPECIFIED.,.F.,.F.,(4,3,3,3,3,3,3,3,3,3,
4),(0.664704897780732,0.688351938092992,0.780317238696427,0.810486879810963,
0.862717972416633,0.955520663501275,1.01466394039958,1.06038302616807,1.10529572457683,
1.13272802062135,1.20216888729732),.UNSPECIFIED.);
#3889=B_SPLINE_CURVE_WITH_KNOTS('',3,(#29598,#29599,#29600,#29601,#29602,
#29603,#29604,#29605,#29606,#29607,#29608,#29609,#29610,#29611,#29612,#29613,
#29614,#29615,#29616),.UNSPECIFIED.,.F.,.F.,(4,3,3,3,3,3,4),(0.,0.178790961538472,
0.350742859481108,0.449205432353047,0.513879914408645,0.522694757423744,
0.664704897780732),.UNSPECIFIED.);
#3890=B_SPLINE_CURVE_WITH_KNOTS('',3,(#29620,#29621,#29622,#29623),
 .UNSPECIFIED.,.F.,.F.,(4,4),(-0.0707400285050858,0.),.UNSPECIFIED.);
#3891=B_SPLINE_CURVE_WITH_KNOTS('',3,(#29627,#29628,#29629,#29630),
 .UNSPECIFIED.,.F.,.F.,(4,4),(-0.0707432949753092,-3.34525766367E-6),
 .UNSPECIFIED.);
#3892=B_SPLINE_CURVE_WITH_KNOTS('',3,(#29634,#29635,#29636,#29637,#29638,
#29639,#29640,#29641,#29642,#29643,#29644,#29645,#29646,#29647,#29648,#29649,
#29650,#29651,#29652,#29653,#29654,#29655,#29656,#29657,#29658,#29659,#29660,
#29661,#29662,#29663,#29664,#29665,#29666,#29667,#29668,#29669,#29670,#29671,
#29672,#29673,#29674,#29675,#29676,#29677,#29678,#29679,#29680,#29681,#29682,
#29683,#29684,#29685,#29686,#29687,#29688,#29689,#29690,#29691,#29692,#29693,
#29694,#29695,#29696,#29697,#29698,#29699,#29700,#29701,#29702,#29703,#29704,
#29705,#29706,#29707,#29708,#29709,#29710,#29711,#29712,#29713,#29714,#29715,
#29716,#29717,#29718,#29719,#29720,#29721,#29722,#29723,#29724,#29725,#29726,
#29727,#29728,#29729,#29730),.UNSPECIFIED.,.F.,.F.,(4,3,3,3,3,3,3,3,3,3,
3,3,3,3,3,3,3,3,3,3,3,3,3,3,3,3,3,3,3,3,3,3,4),(-0.461463988274541,-0.386087506167661,
-0.372903671306323,-0.36421409612757,-0.349922618627789,-0.338448280177947,
-0.328550793223787,-0.322977024945215,-0.314822638010135,-0.306007155781963,
-0.304885949019545,-0.297658439870205,-0.289754515055765,-0.282882239837598,
-0.277393071544922,-0.271439067306183,-0.265165133453763,-0.25827211680326,
-0.254459737762025,-0.242193625915918,-0.228473458861481,-0.213717473129083,
-0.197852099810681,-0.180468088688272,-0.162567602565291,-0.144906259020414,
-0.134249918117004,-0.102205019200819,-0.0696974945135463,-0.0525746845214139,
-0.0222228838221726,-0.000827460244363642,0.),.UNSPECIFIED.);
#3893=B_SPLINE_CURVE_WITH_KNOTS('',3,(#29733,#29734,#29735,#29736,#29737,
#29738,#29739,#29740,#29741,#29742,#29743,#29744,#29745,#29746,#29747,#29748,
#29749,#29750,#29751,#29752,#29753,#29754,#29755,#29756,#29757,#29758,#29759,
#29760,#29761,#29762,#29763,#29764,#29765,#29766,#29767,#29768,#29769,#29770,
#29771,#29772,#29773,#29774,#29775,#29776,#29777,#29778,#29779,#29780,#29781,
#29782,#29783,#29784,#29785,#29786,#29787,#29788,#29789,#29790,#29791,#29792,
#29793,#29794,#29795,#29796),.UNSPECIFIED.,.F.,.F.,(4,3,3,3,3,3,3,3,3,3,
3,3,3,3,3,3,3,3,3,3,3,4),(-0.976443208995993,-0.96062870472102,-0.949661288965092,
-0.931975105549613,-0.91440031086007,-0.904644103415597,-0.893320015681315,
-0.880495083206059,-0.866943636882815,-0.852607981525168,-0.837136125113694,
-0.821574066138705,-0.806147311008988,-0.791872999074437,-0.790720555879271,
-0.779060485592236,-0.740625,-0.691250000000001,-0.5925,-0.49375,-0.394999999999999,
-0.0499999999999998),.UNSPECIFIED.);
#3894=B_SPLINE_CURVE_WITH_KNOTS('',3,(#30018,#30019,#30020,#30021),
 .UNSPECIFIED.,.F.,.F.,(4,4),(-0.253410853624616,-0.103262412077185),
 .UNSPECIFIED.);
#3895=B_SPLINE_CURVE_WITH_KNOTS('',3,(#30023,#30024,#30025,#30026),
 .UNSPECIFIED.,.F.,.F.,(4,4),(0.,0.29),.UNSPECIFIED.);
#3896=B_SPLINE_CURVE_WITH_KNOTS('',3,(#30027,#30028,#30029,#30030),
 .UNSPECIFIED.,.F.,.F.,(4,4),(3.28350553820744,3.37607250422172),
 .UNSPECIFIED.);
#3897=B_SPLINE_CURVE_WITH_KNOTS('',3,(#30032,#30033,#30034,#30035,#30036,
#30037),.UNSPECIFIED.,.F.,.F.,(4,2,4),(-2.17700203273975,-1.38478587807843,
-0.288632999074765),.UNSPECIFIED.);
#3898=B_SPLINE_CURVE_WITH_KNOTS('',3,(#30039,#30040,#30041,#30042,#30043,
#30044,#30045,#30046,#30047,#30048,#30049,#30050,#30051,#30052,#30053,#30054,
#30055,#30056,#30057,#30058,#30059,#30060,#30061,#30062,#30063,#30064,#30065,
#30066,#30067,#30068,#30069),.UNSPECIFIED.,.F.,.F.,(4,3,3,3,3,3,3,3,3,3,
4),(0.664704897780732,0.688351938092992,0.780317238696421,0.810486879810963,
0.862717972416634,0.955520663501275,1.01466394039958,1.06038302616807,1.10529572457683,
1.13272802062135,1.20216888729732),.UNSPECIFIED.);
#3899=B_SPLINE_CURVE_WITH_KNOTS('',3,(#30070,#30071,#30072,#30073,#30074,
#30075,#30076,#30077,#30078,#30079,#30080,#30081,#30082,#30083,#30084,#30085,
#30086,#30087,#30088),.UNSPECIFIED.,.F.,.F.,(4,3,3,3,3,3,4),(0.,0.178790961538472,
0.350742859481108,0.449205432353047,0.513879914408646,0.522694757423744,
0.664704897780732),.UNSPECIFIED.);
#3900=B_SPLINE_CURVE_WITH_KNOTS('',3,(#30092,#30093,#30094,#30095),
 .UNSPECIFIED.,.F.,.F.,(4,4),(-0.0707400282391991,0.),.UNSPECIFIED.);
#3901=B_SPLINE_CURVE_WITH_KNOTS('',3,(#30099,#30100,#30101,#30102),
 .UNSPECIFIED.,.F.,.F.,(4,4),(-0.0707432951646884,-3.34525766250426E-6),
 .UNSPECIFIED.);
#3902=B_SPLINE_CURVE_WITH_KNOTS('',3,(#30106,#30107,#30108,#30109,#30110,
#30111,#30112,#30113,#30114,#30115,#30116,#30117,#30118,#30119,#30120,#30121,
#30122,#30123,#30124,#30125,#30126,#30127,#30128,#30129,#30130,#30131,#30132,
#30133,#30134,#30135,#30136,#30137,#30138,#30139,#30140,#30141,#30142,#30143,
#30144,#30145,#30146,#30147,#30148,#30149,#30150,#30151,#30152,#30153,#30154,
#30155,#30156,#30157,#30158,#30159,#30160,#30161,#30162,#30163,#30164,#30165,
#30166,#30167,#30168,#30169,#30170,#30171,#30172,#30173,#30174,#30175,#30176,
#30177,#30178,#30179,#30180,#30181,#30182,#30183,#30184,#30185,#30186,#30187,
#30188,#30189,#30190,#30191,#30192,#30193,#30194,#30195,#30196,#30197,#30198,
#30199,#30200,#30201,#30202),.UNSPECIFIED.,.F.,.F.,(4,3,3,3,3,3,3,3,3,3,
3,3,3,3,3,3,3,3,3,3,3,3,3,3,3,3,3,3,3,3,3,3,4),(-0.461463988274541,-0.386087506167661,
-0.375299929924104,-0.372903671306323,-0.356077696752447,-0.352040116130794,
-0.339920267375323,-0.338448280177947,-0.326632246672126,-0.313204943761465,
-0.304885949019545,-0.29982124014814,-0.293952204614803,-0.287658393406508,
-0.282882239837598,-0.277507204165034,-0.271689255077659,-0.265572046854315,
-0.25886897335229,-0.254459737762025,-0.241918019250842,-0.227822266677592,
-0.212603244487111,-0.196183063900843,-0.178197554741787,-0.159751102176188,
-0.141758270371022,-0.134249918117004,-0.10123360556295,-0.0682193757076537,
-0.0525746845214139,-0.0245175806023846,0.),.UNSPECIFIED.);
#3903=B_SPLINE_CURVE_WITH_KNOTS('',3,(#30205,#30206,#30207,#30208,#30209,
#30210,#30211,#30212,#30213,#30214,#30215,#30216,#30217,#30218,#30219,#30220,
#30221,#30222,#30223,#30224,#30225,#30226,#30227,#30228,#30229,#30230,#30231,
#30232,#30233,#30234,#30235,#30236,#30237,#30238,#30239,#30240,#30241,#30242,
#30243,#30244,#30245,#30246,#30247,#30248,#30249,#30250,#30251,#30252,#30253,
#30254,#30255,#30256,#30257,#30258,#30259,#30260,#30261,#30262,#30263,#30264,
#30265,#30266,#30267,#30268),.UNSPECIFIED.,.F.,.F.,(4,3,3,3,3,3,3,3,3,3,
3,3,3,3,3,3,3,3,3,3,3,4),(-0.976443208995993,-0.959641771463709,-0.949661288965092,
-0.932500795758733,-0.914975318861591,-0.904644103415597,-0.893689140152815,
-0.881835075865074,-0.86859336767674,-0.854447019507201,-0.83944073270216,
-0.82369847532938,-0.808085046249769,-0.793464970994094,-0.790720555879271,
-0.779060485592236,-0.740625,-0.691250000000001,-0.5925,-0.543125,-0.394999999999999,
-0.0499999999999998),.UNSPECIFIED.);
#3904=B_SPLINE_CURVE_WITH_KNOTS('',3,(#30480,#30481,#30482,#30483),
 .UNSPECIFIED.,.F.,.F.,(4,4),(-0.253410853624616,-0.103262412077185),
 .UNSPECIFIED.);
#3905=B_SPLINE_CURVE_WITH_KNOTS('',3,(#30485,#30486,#30487,#30488),
 .UNSPECIFIED.,.F.,.F.,(4,4),(0.,0.29),.UNSPECIFIED.);
#3906=B_SPLINE_CURVE_WITH_KNOTS('',3,(#30489,#30490,#30491,#30492),
 .UNSPECIFIED.,.F.,.F.,(4,4),(3.28350553686237,3.37607250280011),
 .UNSPECIFIED.);
#3907=B_SPLINE_CURVE_WITH_KNOTS('',3,(#30494,#30495,#30496,#30497,#30498,
#30499),.UNSPECIFIED.,.F.,.F.,(4,2,4),(-2.17700203273975,-1.38478587807843,
-0.288632999074765),.UNSPECIFIED.);
#3908=B_SPLINE_CURVE_WITH_KNOTS('',3,(#30501,#30502,#30503,#30504,#30505,
#30506,#30507,#30508,#30509,#30510,#30511,#30512,#30513,#30514,#30515,#30516,
#30517,#30518,#30519,#30520,#30521,#30522,#30523,#30524,#30525,#30526,#30527,
#30528,#30529,#30530,#30531),.UNSPECIFIED.,.F.,.F.,(4,3,3,3,3,3,3,3,3,3,
4),(0.664704897780732,0.688351938092992,0.78031723869643,0.810486879810963,
0.862717972416625,0.955520663501275,1.01466394039959,1.06038302616807,1.10529572457683,
1.13272802062135,1.20216888729732),.UNSPECIFIED.);
#3909=B_SPLINE_CURVE_WITH_KNOTS('',3,(#30532,#30533,#30534,#30535,#30536,
#30537,#30538,#30539,#30540,#30541,#30542,#30543,#30544,#30545,#30546,#30547,
#30548,#30549,#30550),.UNSPECIFIED.,.F.,.F.,(4,3,3,3,3,3,4),(0.,0.178790961538472,
0.350742859481108,0.449205432353047,0.513879914408646,0.522694757423744,
0.664704897780732),.UNSPECIFIED.);
#3910=B_SPLINE_CURVE_WITH_KNOTS('',3,(#30554,#30555,#30556,#30557),
 .UNSPECIFIED.,.F.,.F.,(4,4),(-0.0707400284125705,0.),.UNSPECIFIED.);
#3911=B_SPLINE_CURVE_WITH_KNOTS('',3,(#30561,#30562,#30563,#30564),
 .UNSPECIFIED.,.F.,.F.,(4,4),(-0.0707432947474667,-3.34525766357285E-6),
 .UNSPECIFIED.);
#3912=B_SPLINE_CURVE_WITH_KNOTS('',3,(#30568,#30569,#30570,#30571,#30572,
#30573,#30574,#30575,#30576,#30577,#30578,#30579,#30580,#30581,#30582,#30583,
#30584,#30585,#30586,#30587,#30588,#30589,#30590,#30591,#30592,#30593,#30594,
#30595,#30596,#30597,#30598,#30599,#30600,#30601,#30602,#30603,#30604,#30605,
#30606,#30607,#30608,#30609,#30610,#30611,#30612,#30613,#30614,#30615,#30616,
#30617,#30618,#30619,#30620,#30621,#30622,#30623,#30624,#30625,#30626,#30627,
#30628,#30629,#30630,#30631,#30632,#30633,#30634,#30635,#30636,#30637,#30638,
#30639,#30640,#30641,#30642,#30643,#30644,#30645,#30646,#30647,#30648,#30649,
#30650,#30651,#30652,#30653,#30654,#30655,#30656,#30657,#30658),
 .UNSPECIFIED.,.F.,.F.,(4,3,3,3,3,3,3,3,3,3,3,3,3,3,3,3,3,3,3,3,3,3,3,3,
3,3,3,3,3,3,4),(-0.461463988274541,-0.386087506167661,-0.372903671306323,
-0.36421409612757,-0.35252875808128,-0.339636892136031,-0.338448280177947,
-0.328074919236012,-0.316383789572668,-0.304885949019545,-0.297243973048271,
-0.288858567477107,-0.282882239837598,-0.277347677282808,-0.271340988166513,
-0.265007390818488,-0.258044852490789,-0.254459737762025,-0.242044020405011,
-0.228141105146501,-0.21318510657597,-0.197120884701618,-0.179636878474804,
-0.161760929349425,-0.144350238406565,-0.134249918117004,-0.102125955921629,
-0.0702664487999561,-0.0525746845214139,-0.021660665015393,0.),
 .UNSPECIFIED.);
#3913=B_SPLINE_CURVE_WITH_KNOTS('',3,(#30661,#30662,#30663,#30664,#30665,
#30666,#30667,#30668,#30669,#30670,#30671,#30672,#30673,#30674,#30675,#30676,
#30677,#30678,#30679,#30680,#30681,#30682,#30683,#30684,#30685,#30686,#30687,
#30688,#30689,#30690,#30691,#30692,#30693,#30694,#30695,#30696,#30697,#30698,
#30699,#30700,#30701,#30702,#30703,#30704,#30705,#30706,#30707,#30708,#30709,
#30710,#30711,#30712,#30713,#30714,#30715,#30716,#30717,#30718,#30719,#30720,
#30721,#30722,#30723,#30724),.UNSPECIFIED.,.F.,.F.,(4,3,3,3,3,3,3,3,3,3,
3,3,3,3,3,3,3,3,3,3,3,4),(-0.976443208995993,-0.960629666524145,-0.949661288965092,
-0.931972270488238,-0.914398186942953,-0.904644103415597,-0.893317754842134,
-0.880493104971776,-0.86694095688213,-0.852605467987035,-0.837134239960094,
-0.82157385570267,-0.80614720579097,-0.791874660471043,-0.790720555879271,
-0.779060485592236,-0.740625,-0.691250000000001,-0.5925,-0.49375,-0.394999999999999,
-0.0499999999999998),.UNSPECIFIED.);
#3914=B_SPLINE_CURVE_WITH_KNOTS('',3,(#30916,#30917,#30918,#30919),
 .UNSPECIFIED.,.F.,.F.,(4,4),(-0.253410853624616,-0.103262412077186),
 .UNSPECIFIED.);
#3915=B_SPLINE_CURVE_WITH_KNOTS('',3,(#30921,#30922,#30923,#30924),
 .UNSPECIFIED.,.F.,.F.,(4,4),(0.,0.29),.UNSPECIFIED.);
#3916=B_SPLINE_CURVE_WITH_KNOTS('',3,(#30925,#30926,#30927,#30928),
 .UNSPECIFIED.,.F.,.F.,(4,4),(3.28350553743639,3.37607250339859),
 .UNSPECIFIED.);
#3917=B_SPLINE_CURVE_WITH_KNOTS('',3,(#30930,#30931,#30932,#30933,#30934,
#30935),.UNSPECIFIED.,.F.,.F.,(4,2,4),(-2.17700203273975,-1.38478587807843,
-0.288632999074766),.UNSPECIFIED.);
#3918=B_SPLINE_CURVE_WITH_KNOTS('',3,(#30937,#30938,#30939,#30940,#30941,
#30942,#30943,#30944,#30945,#30946,#30947,#30948,#30949,#30950,#30951,#30952,
#30953,#30954,#30955,#30956,#30957,#30958,#30959,#30960,#30961,#30962,#30963,
#30964,#30965,#30966,#30967),.UNSPECIFIED.,.F.,.F.,(4,3,3,3,3,3,3,3,3,3,
4),(0.664704897780732,0.688351938092992,0.780317238696445,0.810486879810963,
0.862717972416636,0.955520663501275,1.01466394039967,1.06038302616807,1.10529572457683,
1.13272802062135,1.20216888729732),.UNSPECIFIED.);
#3919=B_SPLINE_CURVE_WITH_KNOTS('',3,(#30968,#30969,#30970,#30971,#30972,
#30973,#30974,#30975,#30976,#30977,#30978,#30979,#30980,#30981,#30982,#30983,
#30984,#30985,#30986),.UNSPECIFIED.,.F.,.F.,(4,3,3,3,3,3,4),(0.,0.178790961538472,
0.350742859481108,0.449205432353047,0.513879914408646,0.522694757423744,
0.664704897780732),.UNSPECIFIED.);
#3920=B_SPLINE_CURVE_WITH_KNOTS('',3,(#30990,#30991,#30992,#30993),
 .UNSPECIFIED.,.F.,.F.,(4,4),(-0.0707400283123018,0.),.UNSPECIFIED.);
#3921=B_SPLINE_CURVE_WITH_KNOTS('',3,(#30997,#30998,#30999,#31000),
 .UNSPECIFIED.,.F.,.F.,(4,4),(-0.0707432952234936,-3.34525766215732E-6),
 .UNSPECIFIED.);
#3922=B_SPLINE_CURVE_WITH_KNOTS('',3,(#31004,#31005,#31006,#31007,#31008,
#31009,#31010,#31011,#31012,#31013,#31014,#31015,#31016,#31017,#31018,#31019,
#31020,#31021,#31022,#31023,#31024,#31025,#31026,#31027,#31028,#31029,#31030,
#31031,#31032,#31033,#31034,#31035,#31036,#31037,#31038,#31039,#31040,#31041,
#31042,#31043,#31044,#31045,#31046,#31047,#31048,#31049,#31050,#31051,#31052,
#31053,#31054,#31055,#31056,#31057,#31058,#31059,#31060,#31061,#31062,#31063,
#31064,#31065,#31066,#31067,#31068,#31069,#31070,#31071,#31072,#31073,#31074,
#31075,#31076,#31077,#31078,#31079,#31080,#31081,#31082,#31083,#31084,#31085,
#31086,#31087,#31088,#31089,#31090,#31091,#31092,#31093,#31094,#31095,#31096,
#31097,#31098,#31099,#31100),.UNSPECIFIED.,.F.,.F.,(4,3,3,3,3,3,3,3,3,3,
3,3,3,3,3,3,3,3,3,3,3,3,3,3,3,3,3,3,3,3,3,3,4),(-0.461463988274541,-0.386087506167661,
-0.372903671306323,-0.36421409612757,-0.349922618618653,-0.338448280177947,
-0.328550793223542,-0.322977024945215,-0.314822638010335,-0.306007155782303,
-0.304885949019545,-0.297658439870374,-0.289754515056093,-0.282882239837598,
-0.277393071545029,-0.271439067306369,-0.265165133453971,-0.258272116803451,
-0.254459737762025,-0.242193625916564,-0.228473458862565,-0.21371747313048,
-0.197852099811482,-0.180468088683521,-0.162567602548332,-0.144906258985007,
-0.134249918117004,-0.102205018832849,-0.0696974934620405,-0.0525746845214139,
-0.0222228841287436,-0.000827460244363642,0.),.UNSPECIFIED.);
#3923=B_SPLINE_CURVE_WITH_KNOTS('',3,(#31103,#31104,#31105,#31106,#31107,
#31108,#31109,#31110,#31111,#31112,#31113,#31114,#31115,#31116,#31117,#31118,
#31119,#31120,#31121,#31122,#31123,#31124,#31125,#31126,#31127,#31128,#31129,
#31130,#31131,#31132,#31133,#31134,#31135,#31136,#31137,#31138,#31139,#31140,
#31141,#31142,#31143,#31144,#31145,#31146,#31147,#31148,#31149,#31150,#31151,
#31152,#31153,#31154,#31155,#31156,#31157,#31158,#31159,#31160,#31161,#31162,
#31163,#31164,#31165,#31166),.UNSPECIFIED.,.F.,.F.,(4,3,3,3,3,3,3,3,3,3,
3,3,3,3,3,3,3,3,3,3,3,4),(-0.976443208995993,-0.960628704721019,-0.949661288965092,
-0.931975105549617,-0.914400310860108,-0.904644103415597,-0.893320015681313,
-0.880495083206057,-0.866943636882841,-0.852607981525343,-0.837136125113825,
-0.821574066139019,-0.806147311009145,-0.791872999074882,-0.790720555879271,
-0.779060485592236,-0.740625,-0.691250000000001,-0.5925,-0.49375,-0.394999999999999,
-0.0499999999999998),.UNSPECIFIED.);
#3924=B_SPLINE_CURVE_WITH_KNOTS('',3,(#31388,#31389,#31390,#31391),
 .UNSPECIFIED.,.F.,.F.,(4,4),(-0.253410853624616,-0.103262412077186),
 .UNSPECIFIED.);
#3925=B_SPLINE_CURVE_WITH_KNOTS('',3,(#31393,#31394,#31395,#31396),
 .UNSPECIFIED.,.F.,.F.,(4,4),(0.,0.29),.UNSPECIFIED.);
#3926=B_SPLINE_CURVE_WITH_KNOTS('',3,(#31397,#31398,#31399,#31400),
 .UNSPECIFIED.,.F.,.F.,(4,4),(3.2835055364322,3.37607250233925),
 .UNSPECIFIED.);
#3927=B_SPLINE_CURVE_WITH_KNOTS('',3,(#31402,#31403,#31404,#31405,#31406,
#31407),.UNSPECIFIED.,.F.,.F.,(4,2,4),(-2.17700203273975,-1.38478587807843,
-0.288632999074765),.UNSPECIFIED.);
#3928=B_SPLINE_CURVE_WITH_KNOTS('',3,(#31409,#31410,#31411,#31412,#31413,
#31414,#31415,#31416,#31417,#31418,#31419,#31420,#31421,#31422,#31423,#31424,
#31425,#31426,#31427,#31428,#31429,#31430,#31431,#31432,#31433,#31434,#31435,
#31436,#31437,#31438,#31439),.UNSPECIFIED.,.F.,.F.,(4,3,3,3,3,3,3,3,3,3,
4),(0.664704897780732,0.688351938092992,0.780317238696455,0.810486879810963,
0.86271797241663,0.955520663501275,1.0146639403996,1.06038302616807,1.10529572457683,
1.13272802062135,1.20216888729732),.UNSPECIFIED.);
#3929=B_SPLINE_CURVE_WITH_KNOTS('',3,(#31440,#31441,#31442,#31443,#31444,
#31445,#31446,#31447,#31448,#31449,#31450,#31451,#31452,#31453,#31454,#31455,
#31456,#31457,#31458),.UNSPECIFIED.,.F.,.F.,(4,3,3,3,3,3,4),(0.,0.178790961538472,
0.350742859481108,0.449205432353048,0.513879914408647,0.522694757423744,
0.664704897780732),.UNSPECIFIED.);
#3930=B_SPLINE_CURVE_WITH_KNOTS('',3,(#31462,#31463,#31464,#31465),
 .UNSPECIFIED.,.F.,.F.,(4,4),(-0.070740028238931,0.),.UNSPECIFIED.);
#3931=B_SPLINE_CURVE_WITH_KNOTS('',3,(#31469,#31470,#31471,#31472),
 .UNSPECIFIED.,.F.,.F.,(4,4),(-0.0707432954463844,-3.34525766251814E-6),
 .UNSPECIFIED.);
#3932=B_SPLINE_CURVE_WITH_KNOTS('',3,(#31476,#31477,#31478,#31479,#31480,
#31481,#31482,#31483,#31484,#31485,#31486,#31487,#31488,#31489,#31490,#31491,
#31492,#31493,#31494,#31495,#31496,#31497,#31498,#31499,#31500,#31501,#31502,
#31503,#31504,#31505,#31506,#31507,#31508,#31509,#31510,#31511,#31512,#31513,
#31514,#31515,#31516,#31517,#31518,#31519,#31520,#31521,#31522,#31523,#31524,
#31525,#31526,#31527,#31528,#31529,#31530,#31531,#31532,#31533,#31534,#31535,
#31536,#31537,#31538,#31539,#31540,#31541,#31542,#31543,#31544,#31545,#31546,
#31547,#31548,#31549,#31550,#31551,#31552,#31553,#31554,#31555,#31556,#31557,
#31558,#31559,#31560,#31561,#31562,#31563,#31564,#31565,#31566,#31567,#31568,
#31569,#31570,#31571,#31572),.UNSPECIFIED.,.F.,.F.,(4,3,3,3,3,3,3,3,3,3,
3,3,3,3,3,3,3,3,3,3,3,3,3,3,3,3,3,3,3,3,3,3,4),(-0.461463988274541,-0.386087506167661,
-0.375299929924104,-0.372903671306323,-0.356067397506652,-0.352040116130794,
-0.339910821414875,-0.338448280177947,-0.326626118627217,-0.313191280956895,
-0.304885949019545,-0.29982124014814,-0.293951934878654,-0.287657824438721,
-0.282882239837598,-0.277506987555355,-0.271688793715204,-0.265571314353823,
-0.258867937821342,-0.254459737762025,-0.241918476962302,-0.227823327163533,
-0.21260498793569,-0.196185493994907,-0.178200253731108,-0.159753497644407,
-0.141759381819153,-0.134249918117004,-0.101233746097596,-0.0682163658997657,
-0.0525746845214139,-0.024519300953322,0.),.UNSPECIFIED.);
#3933=B_SPLINE_CURVE_WITH_KNOTS('',3,(#31575,#31576,#31577,#31578,#31579,
#31580,#31581,#31582,#31583,#31584,#31585,#31586,#31587,#31588,#31589,#31590,
#31591,#31592,#31593,#31594,#31595,#31596,#31597,#31598,#31599,#31600,#31601,
#31602,#31603,#31604,#31605,#31606,#31607,#31608,#31609,#31610,#31611,#31612,
#31613,#31614,#31615,#31616,#31617,#31618,#31619,#31620,#31621,#31622,#31623,
#31624,#31625,#31626,#31627,#31628,#31629,#31630,#31631,#31632,#31633,#31634,
#31635,#31636,#31637,#31638),.UNSPECIFIED.,.F.,.F.,(4,3,3,3,3,3,3,3,3,3,
3,3,3,3,3,3,3,3,3,3,3,4),(-0.976443208995993,-0.959641771463709,-0.949661288965092,
-0.932500795758733,-0.914975318861593,-0.904644103415597,-0.893689140152816,
-0.881835075865263,-0.86859336767701,-0.854447019507575,-0.839440732702475,
-0.823698475329622,-0.808085046250136,-0.793464970994181,-0.790720555879271,
-0.779060485592236,-0.740625,-0.691250000000001,-0.5925,-0.543125,-0.394999999999999,
-0.0499999999999998),.UNSPECIFIED.);
#3934=B_SPLINE_CURVE_WITH_KNOTS('',3,(#31850,#31851,#31852,#31853),
 .UNSPECIFIED.,.F.,.F.,(4,4),(-0.253410853624616,-0.103262412077185),
 .UNSPECIFIED.);
#3935=B_SPLINE_CURVE_WITH_KNOTS('',3,(#31855,#31856,#31857,#31858),
 .UNSPECIFIED.,.F.,.F.,(4,4),(0.,0.29),.UNSPECIFIED.);
#3936=B_SPLINE_CURVE_WITH_KNOTS('',3,(#31859,#31860,#31861,#31862),
 .UNSPECIFIED.,.F.,.F.,(4,4),(3.28350553681631,3.37607250273892),
 .UNSPECIFIED.);
#3937=B_SPLINE_CURVE_WITH_KNOTS('',3,(#31864,#31865,#31866,#31867,#31868,
#31869),.UNSPECIFIED.,.F.,.F.,(4,2,4),(-2.17700203273975,-1.38478587807843,
-0.288632999074765),.UNSPECIFIED.);
#3938=B_SPLINE_CURVE_WITH_KNOTS('',3,(#31871,#31872,#31873,#31874,#31875,
#31876,#31877,#31878,#31879,#31880,#31881,#31882,#31883,#31884,#31885,#31886,
#31887,#31888,#31889,#31890,#31891,#31892,#31893,#31894,#31895,#31896,#31897,
#31898,#31899,#31900,#31901),.UNSPECIFIED.,.F.,.F.,(4,3,3,3,3,3,3,3,3,3,
4),(0.664704897780732,0.688351938092992,0.780317238696435,0.810486879810963,
0.862717972416624,0.955520663501275,1.01466394039955,1.06038302616807,1.10529572457683,
1.13272802062135,1.20216888729732),.UNSPECIFIED.);
#3939=B_SPLINE_CURVE_WITH_KNOTS('',3,(#31902,#31903,#31904,#31905,#31906,
#31907,#31908,#31909,#31910,#31911,#31912,#31913,#31914,#31915,#31916,#31917,
#31918,#31919,#31920),.UNSPECIFIED.,.F.,.F.,(4,3,3,3,3,3,4),(0.,0.178790961538472,
0.350742859481108,0.449205432353047,0.513879914408646,0.522694757423744,
0.664704897780732),.UNSPECIFIED.);
#3940=B_SPLINE_CURVE_WITH_KNOTS('',3,(#31924,#31925,#31926,#31927),
 .UNSPECIFIED.,.F.,.F.,(4,4),(-0.0707400282745222,0.),.UNSPECIFIED.);
#3941=B_SPLINE_CURVE_WITH_KNOTS('',3,(#31931,#31932,#31933,#31934),
 .UNSPECIFIED.,.F.,.F.,(4,4),(-0.0707432948552679,-3.34525766382265E-6),
 .UNSPECIFIED.);
#3942=B_SPLINE_CURVE_WITH_KNOTS('',3,(#31938,#31939,#31940,#31941,#31942,
#31943,#31944,#31945,#31946,#31947,#31948,#31949,#31950,#31951,#31952,#31953,
#31954,#31955,#31956,#31957,#31958,#31959,#31960,#31961,#31962,#31963,#31964,
#31965,#31966,#31967,#31968,#31969,#31970,#31971,#31972,#31973,#31974,#31975,
#31976,#31977,#31978,#31979,#31980,#31981,#31982,#31983,#31984,#31985,#31986,
#31987,#31988,#31989,#31990,#31991,#31992,#31993,#31994,#31995,#31996,#31997,
#31998,#31999,#32000,#32001,#32002,#32003,#32004,#32005,#32006,#32007,#32008,
#32009,#32010,#32011,#32012,#32013,#32014,#32015,#32016,#32017,#32018,#32019,
#32020,#32021,#32022,#32023,#32024,#32025,#32026,#32027,#32028),
 .UNSPECIFIED.,.F.,.F.,(4,3,3,3,3,3,3,3,3,3,3,3,3,3,3,3,3,3,3,3,3,3,3,3,
3,3,3,3,3,3,4),(-0.461463988274541,-0.386087506167661,-0.372903671306323,
-0.36421409612757,-0.352528758081246,-0.339636892135942,-0.338448280177947,
-0.328074919236012,-0.316383789572667,-0.304885949019545,-0.297243973048271,
-0.288858567477107,-0.282882239837598,-0.277347677282806,-0.271340988166504,
-0.265007390818465,-0.25804485249077,-0.254459737762025,-0.242044020405011,
-0.228141105146492,-0.213185106576009,-0.197120884701566,-0.179636878474647,
-0.161760929349303,-0.144350238406463,-0.134249918117004,-0.102125955921642,
-0.0702664487997433,-0.0525746845214139,-0.0216606650153897,0.),
 .UNSPECIFIED.);
#3943=B_SPLINE_CURVE_WITH_KNOTS('',3,(#32031,#32032,#32033,#32034,#32035,
#32036,#32037,#32038,#32039,#32040,#32041,#32042,#32043,#32044,#32045,#32046,
#32047,#32048,#32049,#32050,#32051,#32052,#32053,#32054,#32055,#32056,#32057,
#32058,#32059,#32060,#32061,#32062,#32063,#32064,#32065,#32066,#32067,#32068,
#32069,#32070,#32071,#32072,#32073,#32074,#32075,#32076,#32077,#32078,#32079,
#32080,#32081,#32082,#32083,#32084,#32085,#32086,#32087,#32088,#32089,#32090,
#32091,#32092,#32093,#32094),.UNSPECIFIED.,.F.,.F.,(4,3,3,3,3,3,3,3,3,3,
3,3,3,3,3,3,3,3,3,3,3,4),(-0.976443208995993,-0.960629666524143,-0.949661288965092,
-0.931972270488239,-0.91439818694386,-0.904644103415597,-0.893317754842135,
-0.880493104971777,-0.866940956882102,-0.852605467987185,-0.837134239960207,
-0.821573855702639,-0.806147205790955,-0.791874660471242,-0.790720555879271,
-0.779060485592236,-0.740625,-0.691250000000001,-0.5925,-0.49375,-0.394999999999999,
-0.0499999999999998),.UNSPECIFIED.);
#3944=B_SPLINE_CURVE_WITH_KNOTS('',3,(#32286,#32287,#32288,#32289),
 .UNSPECIFIED.,.F.,.F.,(4,4),(-0.253410853624616,-0.103262412077186),
 .UNSPECIFIED.);
#3945=B_SPLINE_CURVE_WITH_KNOTS('',3,(#32291,#32292,#32293,#32294),
 .UNSPECIFIED.,.F.,.F.,(4,4),(0.,0.29),.UNSPECIFIED.);
#3946=B_SPLINE_CURVE_WITH_KNOTS('',3,(#32295,#32296,#32297,#32298),
 .UNSPECIFIED.,.F.,.F.,(4,4),(3.28350553629102,3.37607250219087),
 .UNSPECIFIED.);
#3947=B_SPLINE_CURVE_WITH_KNOTS('',3,(#32300,#32301,#32302,#32303,#32304,
#32305),.UNSPECIFIED.,.F.,.F.,(4,2,4),(-2.17700203273975,-1.38478587807843,
-0.288632999074765),.UNSPECIFIED.);
#3948=B_SPLINE_CURVE_WITH_KNOTS('',3,(#32307,#32308,#32309,#32310,#32311,
#32312,#32313,#32314,#32315,#32316,#32317,#32318,#32319,#32320,#32321,#32322,
#32323,#32324,#32325,#32326,#32327,#32328,#32329,#32330,#32331,#32332,#32333,
#32334,#32335,#32336,#32337),.UNSPECIFIED.,.F.,.F.,(4,3,3,3,3,3,3,3,3,3,
4),(0.664704897780732,0.688351938092992,0.780317238696413,0.810486879810963,
0.862717972416625,0.955520663501275,1.01466394039958,1.06038302616807,1.10529572457683,
1.13272802062135,1.20216888729732),.UNSPECIFIED.);
#3949=B_SPLINE_CURVE_WITH_KNOTS('',3,(#32338,#32339,#32340,#32341,#32342,
#32343,#32344,#32345,#32346,#32347,#32348,#32349,#32350,#32351,#32352,#32353,
#32354,#32355,#32356),.UNSPECIFIED.,.F.,.F.,(4,3,3,3,3,3,4),(0.,0.178790961538472,
0.350742859481108,0.449205432353047,0.513879914408646,0.522694757423744,
0.664704897780732),.UNSPECIFIED.);
#3950=B_SPLINE_CURVE_WITH_KNOTS('',3,(#32360,#32361,#32362,#32363),
 .UNSPECIFIED.,.F.,.F.,(4,4),(-0.0707400283126209,0.),.UNSPECIFIED.);
#3951=B_SPLINE_CURVE_WITH_KNOTS('',3,(#32367,#32368,#32369,#32370),
 .UNSPECIFIED.,.F.,.F.,(4,4),(-0.0707432952233519,-3.34525766214344E-6),
 .UNSPECIFIED.);
#3952=B_SPLINE_CURVE_WITH_KNOTS('',3,(#32374,#32375,#32376,#32377,#32378,
#32379,#32380,#32381,#32382,#32383,#32384,#32385,#32386,#32387,#32388,#32389,
#32390,#32391,#32392,#32393,#32394,#32395,#32396,#32397,#32398,#32399,#32400,
#32401,#32402,#32403,#32404,#32405,#32406,#32407,#32408,#32409,#32410,#32411,
#32412,#32413,#32414,#32415,#32416,#32417,#32418,#32419,#32420,#32421,#32422,
#32423,#32424,#32425,#32426,#32427,#32428,#32429,#32430,#32431,#32432,#32433,
#32434,#32435,#32436,#32437,#32438,#32439,#32440,#32441,#32442,#32443,#32444,
#32445,#32446,#32447,#32448,#32449,#32450,#32451,#32452,#32453,#32454,#32455,
#32456,#32457,#32458,#32459,#32460,#32461,#32462,#32463,#32464,#32465,#32466,
#32467,#32468,#32469,#32470),.UNSPECIFIED.,.F.,.F.,(4,3,3,3,3,3,3,3,3,3,
3,3,3,3,3,3,3,3,3,3,3,3,3,3,3,3,3,3,3,3,3,3,4),(-0.461463988274541,-0.386087506167661,
-0.372903671306323,-0.36421409612757,-0.349922618627965,-0.338448280177947,
-0.328550793223787,-0.322977024945215,-0.314822638010135,-0.306007155781965,
-0.304885949019545,-0.297658439870209,-0.289754515055766,-0.282882239837598,
-0.277393071544918,-0.271439067306178,-0.265165133453712,-0.258272116803191,
-0.254459737762025,-0.242193625915922,-0.228473458861454,-0.213717473128992,
-0.197852099810461,-0.180468088688012,-0.162567602565365,-0.144906259020509,
-0.134249918117004,-0.102205019200821,-0.069697494513509,-0.0525746845214139,
-0.0222228838221762,-0.000827460244363642,0.),.UNSPECIFIED.);
#3953=B_SPLINE_CURVE_WITH_KNOTS('',3,(#32473,#32474,#32475,#32476,#32477,
#32478,#32479,#32480,#32481,#32482,#32483,#32484,#32485,#32486,#32487,#32488,
#32489,#32490,#32491,#32492,#32493,#32494,#32495,#32496,#32497,#32498,#32499,
#32500,#32501,#32502,#32503,#32504,#32505,#32506,#32507,#32508,#32509,#32510,
#32511,#32512,#32513,#32514,#32515,#32516,#32517,#32518,#32519,#32520,#32521,
#32522,#32523,#32524,#32525,#32526,#32527,#32528,#32529,#32530,#32531,#32532,
#32533,#32534,#32535,#32536),.UNSPECIFIED.,.F.,.F.,(4,3,3,3,3,3,3,3,3,3,
3,3,3,3,3,3,3,3,3,3,3,4),(-0.976443208995993,-0.960628704721016,-0.949661288965092,
-0.931975105549621,-0.914400310859732,-0.904644103415597,-0.893320015681319,
-0.880495083206063,-0.866943636882833,-0.852607981525122,-0.837136125113659,
-0.821574066138669,-0.80614731100897,-0.791872999074531,-0.790720555879271,
-0.779060485592236,-0.740625,-0.691250000000001,-0.5925,-0.49375,-0.394999999999999,
-0.0499999999999998),.UNSPECIFIED.);
#3954=B_SPLINE_CURVE_WITH_KNOTS('',3,(#32758,#32759,#32760,#32761),
 .UNSPECIFIED.,.F.,.F.,(4,4),(-0.253410853624616,-0.103262412077186),
 .UNSPECIFIED.);
#3955=B_SPLINE_CURVE_WITH_KNOTS('',3,(#32763,#32764,#32765,#32766),
 .UNSPECIFIED.,.F.,.F.,(4,4),(0.,0.29),.UNSPECIFIED.);
#3956=B_SPLINE_CURVE_WITH_KNOTS('',3,(#32767,#32768,#32769,#32770),
 .UNSPECIFIED.,.F.,.F.,(4,4),(3.28350553791586,3.3760725039151),
 .UNSPECIFIED.);
#3957=B_SPLINE_CURVE_WITH_KNOTS('',3,(#32772,#32773,#32774,#32775,#32776,
#32777),.UNSPECIFIED.,.F.,.F.,(4,2,4),(-2.17700203273975,-1.38478587807843,
-0.288632999074766),.UNSPECIFIED.);
#3958=B_SPLINE_CURVE_WITH_KNOTS('',3,(#32779,#32780,#32781,#32782,#32783,
#32784,#32785,#32786,#32787,#32788,#32789,#32790,#32791,#32792,#32793,#32794,
#32795,#32796,#32797,#32798,#32799,#32800,#32801,#32802,#32803,#32804,#32805,
#32806,#32807,#32808,#32809),.UNSPECIFIED.,.F.,.F.,(4,3,3,3,3,3,3,3,3,3,
4),(0.664704897780732,0.688351938092992,0.780317238696449,0.810486879810963,
0.862717972416621,0.955520663501275,1.0146639403996,1.06038302616807,1.10529572457683,
1.13272802062135,1.20216888729732),.UNSPECIFIED.);
#3959=B_SPLINE_CURVE_WITH_KNOTS('',3,(#32810,#32811,#32812,#32813,#32814,
#32815,#32816,#32817,#32818,#32819,#32820,#32821,#32822,#32823,#32824,#32825,
#32826,#32827,#32828),.UNSPECIFIED.,.F.,.F.,(4,3,3,3,3,3,4),(0.,0.178790961538472,
0.350742859481108,0.449205432353048,0.513879914408647,0.522694757423744,
0.664704897780732),.UNSPECIFIED.);
#3960=B_SPLINE_CURVE_WITH_KNOTS('',3,(#32874,#32875,#32876,#32877),
 .UNSPECIFIED.,.F.,.F.,(4,4),(3.77373852169387,3.81785134154664),
 .UNSPECIFIED.);
#3961=B_SPLINE_CURVE_WITH_KNOTS('',3,(#32881,#32882,#32883,#32884),
 .UNSPECIFIED.,.F.,.F.,(4,4),(1.38212585516677,1.42567867406759),
 .UNSPECIFIED.);
#3962=B_SPLINE_CURVE_WITH_KNOTS('',3,(#32898,#32899,#32900,#32901),
 .UNSPECIFIED.,.F.,.F.,(4,4),(1.38212585516678,1.42567867432177),
 .UNSPECIFIED.);
#3963=B_SPLINE_CURVE_WITH_KNOTS('',3,(#32908,#32909,#32910,#32911),
 .UNSPECIFIED.,.F.,.F.,(4,4),(0.,0.29),.UNSPECIFIED.);
#3964=B_SPLINE_CURVE_WITH_KNOTS('',3,(#32933,#32934,#32935,#32936),
 .UNSPECIFIED.,.F.,.F.,(4,4),(3.77373852169387,3.81785134154665),
 .UNSPECIFIED.);
#3965=B_SPLINE_CURVE_WITH_KNOTS('',3,(#32958,#32959,#32960,#32961),
 .UNSPECIFIED.,.F.,.F.,(4,4),(1.38212585516677,1.42567867432177),
 .UNSPECIFIED.);
#3966=B_SPLINE_CURVE_WITH_KNOTS('',3,(#32968,#32969,#32970,#32971),
 .UNSPECIFIED.,.F.,.F.,(4,4),(0.,0.29),.UNSPECIFIED.);
#3967=B_SPLINE_CURVE_WITH_KNOTS('',3,(#32993,#32994,#32995,#32996),
 .UNSPECIFIED.,.F.,.F.,(4,4),(3.77373852169387,3.81785134154664),
 .UNSPECIFIED.);
#3968=B_SPLINE_CURVE_WITH_KNOTS('',3,(#33018,#33019,#33020,#33021),
 .UNSPECIFIED.,.F.,.F.,(4,4),(1.38212585516678,1.42567867432177),
 .UNSPECIFIED.);
#3969=B_SPLINE_CURVE_WITH_KNOTS('',3,(#33028,#33029,#33030,#33031),
 .UNSPECIFIED.,.F.,.F.,(4,4),(0.,0.29),.UNSPECIFIED.);
#3970=B_SPLINE_CURVE_WITH_KNOTS('',3,(#33053,#33054,#33055,#33056),
 .UNSPECIFIED.,.F.,.F.,(4,4),(3.77373852169387,3.81785134154664),
 .UNSPECIFIED.);
#3971=B_SPLINE_CURVE_WITH_KNOTS('',3,(#33078,#33079,#33080,#33081),
 .UNSPECIFIED.,.F.,.F.,(4,4),(1.38212585516677,1.42567867432177),
 .UNSPECIFIED.);
#3972=B_SPLINE_CURVE_WITH_KNOTS('',3,(#33088,#33089,#33090,#33091),
 .UNSPECIFIED.,.F.,.F.,(4,4),(0.,0.29),.UNSPECIFIED.);
#3973=B_SPLINE_CURVE_WITH_KNOTS('',3,(#33113,#33114,#33115,#33116),
 .UNSPECIFIED.,.F.,.F.,(4,4),(3.77373852169387,3.81785134154665),
 .UNSPECIFIED.);
#3974=B_SPLINE_CURVE_WITH_KNOTS('',3,(#33138,#33139,#33140,#33141),
 .UNSPECIFIED.,.F.,.F.,(4,4),(1.38212585516677,1.42567867432177),
 .UNSPECIFIED.);
#3975=B_SPLINE_CURVE_WITH_KNOTS('',3,(#33148,#33149,#33150,#33151),
 .UNSPECIFIED.,.F.,.F.,(4,4),(0.,0.29),.UNSPECIFIED.);
#3976=B_SPLINE_CURVE_WITH_KNOTS('',3,(#33173,#33174,#33175,#33176),
 .UNSPECIFIED.,.F.,.F.,(4,4),(3.77373866725656,3.81785134154664),
 .UNSPECIFIED.);
#3977=B_SPLINE_CURVE_WITH_KNOTS('',3,(#33217,#33218,#33219,#33220),
 .UNSPECIFIED.,.F.,.F.,(4,4),(1.38209974812346,1.42565252910459),
 .UNSPECIFIED.);
#3978=B_SPLINE_CURVE_WITH_KNOTS('',3,(#33230,#33231,#33232,#33233,#33234,
#33235),.UNSPECIFIED.,.F.,.F.,(4,2,4),(2.73646626801627,2.7475473717049,
2.77362936601305),.UNSPECIFIED.);
#3979=B_SPLINE_CURVE_WITH_KNOTS('',3,(#33237,#33238,#33239,#33240,#33241,
#33242),.UNSPECIFIED.,.F.,.F.,(4,2,4),(1.69951603755124,1.72559803185939,
1.73667913554802),.UNSPECIFIED.);
#3980=B_SPLINE_CURVE_WITH_KNOTS('',3,(#33246,#33247,#33248,#33249,#33250,
#33251),.UNSPECIFIED.,.F.,.F.,(4,2,4),(2.73646626800866,2.74754737169729,
2.77362936600545),.UNSPECIFIED.);
#3981=B_SPLINE_CURVE_WITH_KNOTS('',3,(#33253,#33254,#33255,#33256,#33257,
#33258),.UNSPECIFIED.,.F.,.F.,(4,2,4),(1.69951603754363,1.72559803185179,
1.73667913554042),.UNSPECIFIED.);
#3982=B_SPLINE_CURVE_WITH_KNOTS('',3,(#33274,#33275,#33276,#33277),
 .UNSPECIFIED.,.F.,.F.,(4,4),(0.,0.29),.UNSPECIFIED.);
#3983=B_SPLINE_CURVE_WITH_KNOTS('',3,(#33298,#33299,#33300,#33301),
 .UNSPECIFIED.,.F.,.F.,(4,4),(3.77373866725655,3.81785134154664),
 .UNSPECIFIED.);
#3984=B_SPLINE_CURVE_WITH_KNOTS('',3,(#33313,#33314,#33315,#33316),
 .UNSPECIFIED.,.F.,.F.,(4,4),(1.38209974812346,1.42565252910459),
 .UNSPECIFIED.);
#3985=B_SPLINE_CURVE_WITH_KNOTS('',3,(#33330,#33331,#33332,#33333),
 .UNSPECIFIED.,.F.,.F.,(4,4),(0.,0.29),.UNSPECIFIED.);
#3986=B_SPLINE_CURVE_WITH_KNOTS('',3,(#33354,#33355,#33356,#33357),
 .UNSPECIFIED.,.F.,.F.,(4,4),(3.77373866725655,3.81785134154664),
 .UNSPECIFIED.);
#3987=B_SPLINE_CURVE_WITH_KNOTS('',3,(#33369,#33370,#33371,#33372),
 .UNSPECIFIED.,.F.,.F.,(4,4),(1.38209974812346,1.42565252910459),
 .UNSPECIFIED.);
#3988=B_SPLINE_CURVE_WITH_KNOTS('',3,(#33386,#33387,#33388,#33389),
 .UNSPECIFIED.,.F.,.F.,(4,4),(0.,0.29),.UNSPECIFIED.);
#3989=B_SPLINE_CURVE_WITH_KNOTS('',3,(#33410,#33411,#33412,#33413),
 .UNSPECIFIED.,.F.,.F.,(4,4),(3.77373866725655,3.81785134154664),
 .UNSPECIFIED.);
#3990=B_SPLINE_CURVE_WITH_KNOTS('',3,(#33425,#33426,#33427,#33428),
 .UNSPECIFIED.,.F.,.F.,(4,4),(1.38209974812346,1.42565252910459),
 .UNSPECIFIED.);
#3991=B_SPLINE_CURVE_WITH_KNOTS('',3,(#33442,#33443,#33444,#33445),
 .UNSPECIFIED.,.F.,.F.,(4,4),(0.,0.29),.UNSPECIFIED.);
#3992=B_SPLINE_CURVE_WITH_KNOTS('',3,(#33466,#33467,#33468,#33469),
 .UNSPECIFIED.,.F.,.F.,(4,4),(3.77373866725655,3.81785134154664),
 .UNSPECIFIED.);
#3993=B_SPLINE_CURVE_WITH_KNOTS('',3,(#33481,#33482,#33483,#33484),
 .UNSPECIFIED.,.F.,.F.,(4,4),(1.38209974812346,1.42565252910459),
 .UNSPECIFIED.);
#3994=B_SPLINE_CURVE_WITH_KNOTS('',3,(#33498,#33499,#33500,#33501),
 .UNSPECIFIED.,.F.,.F.,(4,4),(0.,0.29),.UNSPECIFIED.);
#3995=B_SPLINE_CURVE_WITH_KNOTS('',3,(#33522,#33523,#33524,#33525),
 .UNSPECIFIED.,.F.,.F.,(4,4),(3.77373866725656,3.81785134154665),
 .UNSPECIFIED.);
#3996=B_SPLINE_CURVE_WITH_KNOTS('',3,(#33537,#33538,#33539,#33540),
 .UNSPECIFIED.,.F.,.F.,(4,4),(1.38209974812346,1.42565252910459),
 .UNSPECIFIED.);
#3997=B_SPLINE_CURVE_WITH_KNOTS('',3,(#33558,#33559,#33560,#33561),
 .UNSPECIFIED.,.F.,.F.,(4,4),(0.,0.29),.UNSPECIFIED.);
#3998=B_SPLINE_CURVE_WITH_KNOTS('',3,(#33565,#33566,#33567,#33568),
 .UNSPECIFIED.,.F.,.F.,(4,4),(3.77373866725655,3.81785134154664),
 .UNSPECIFIED.);
#3999=B_SPLINE_CURVE_WITH_KNOTS('',3,(#33577,#33578,#33579,#33580),
 .UNSPECIFIED.,.F.,.F.,(4,4),(0.,0.29),.UNSPECIFIED.);
#4000=B_SPLINE_CURVE_WITH_KNOTS('',3,(#33608,#33609,#33610,#33611,#33612,
#33613),.UNSPECIFIED.,.F.,.F.,(4,2,4),(1.69951603754749,1.72559803185564,
1.73667913554427),.UNSPECIFIED.);
#4001=B_SPLINE_CURVE_WITH_KNOTS('',3,(#33617,#33618,#33619,#33620,#33621,
#33622),.UNSPECIFIED.,.F.,.F.,(4,2,4),(2.73646626801252,2.74754737170115,
2.7736293660093),.UNSPECIFIED.);
#4002=B_SPLINE_CURVE_WITH_KNOTS('',3,(#33624,#33625,#33626,#33627),
 .UNSPECIFIED.,.F.,.F.,(4,4),(-0.123345114071782,0.),.UNSPECIFIED.);
#4003=B_SPLINE_CURVE_WITH_KNOTS('',3,(#33630,#33631,#33632,#33633),
 .UNSPECIFIED.,.F.,.F.,(4,4),(-0.123320533354397,0.),.UNSPECIFIED.);
#4004=B_SPLINE_CURVE_WITH_KNOTS('',3,(#33636,#33637,#33638,#33639,#33640,
#33641,#33642,#33643,#33644,#33645,#33646,#33647,#33648,#33649,#33650,#33651,
#33652,#33653,#33654,#33655,#33656,#33657,#33658,#33659,#33660,#33661,#33662,
#33663,#33664,#33665,#33666,#33667,#33668,#33669,#33670,#33671,#33672,#33673,
#33674,#33675,#33676,#33677,#33678,#33679,#33680,#33681,#33682,#33683,#33684,
#33685,#33686,#33687,#33688,#33689,#33690,#33691,#33692,#33693,#33694,#33695,
#33696,#33697,#33698,#33699,#33700,#33701,#33702,#33703,#33704,#33705,#33706,
#33707,#33708,#33709,#33710,#33711,#33712,#33713,#33714,#33715,#33716,#33717,
#33718,#33719,#33720,#33721,#33722,#33723,#33724,#33725,#33726,#33727,#33728,
#33729),.UNSPECIFIED.,.F.,.F.,(4,3,3,3,3,3,3,3,3,3,3,3,3,3,3,3,3,3,3,3,
3,3,3,3,3,3,3,3,3,3,3,4),(-0.658260979006731,-0.633773279162244,-0.605111071598155,
-0.587935823275639,-0.58215389072593,-0.576676348727153,-0.545880192440996,
-0.518933555690609,-0.50528736116522,-0.500250745725887,-0.469731699052497,
-0.438742337954577,-0.407896515574978,-0.388499161290708,-0.383813915666766,
-0.379411229252426,-0.347601178358055,-0.330307098437898,-0.29950598700594,
-0.268122067677042,-0.260223722040077,-0.255500332123237,-0.223562790607832,
-0.191212812564609,-0.158617534984855,-0.138790343111748,-0.132403685477666,
-0.127529513558128,-0.0941940108532412,-0.0608372923199841,-0.0281712614885087,
0.),.UNSPECIFIED.);
#4005=B_SPLINE_CURVE_WITH_KNOTS('',3,(#33734,#33735,#33736,#33737,#33738,
#33739,#33740,#33741,#33742,#33743,#33744,#33745,#33746,#33747,#33748,#33749,
#33750,#33751,#33752,#33753,#33754,#33755,#33756,#33757,#33758,#33759,#33760,
#33761,#33762,#33763,#33764,#33765,#33766,#33767,#33768,#33769,#33770,#33771,
#33772,#33773,#33774,#33775,#33776,#33777,#33778,#33779,#33780,#33781,#33782,
#33783,#33784,#33785,#33786,#33787,#33788,#33789,#33790,#33791,#33792,#33793,
#33794,#33795,#33796,#33797,#33798,#33799,#33800,#33801,#33802,#33803,#33804,
#33805,#33806,#33807,#33808,#33809,#33810,#33811,#33812,#33813,#33814,#33815,
#33816,#33817,#33818,#33819,#33820,#33821,#33822,#33823,#33824,#33825,#33826,
#33827,#33828,#33829,#33830),.UNSPECIFIED.,.F.,.F.,(4,3,3,3,3,3,3,3,3,3,
3,3,3,3,3,3,3,3,3,3,3,3,3,3,3,3,3,3,3,3,3,3,4),(-0.655752415918347,-0.626851741040676,
-0.59369504602698,-0.575358814455742,-0.568230237621974,-0.56261560332179,
-0.529721437610406,-0.501045675520003,-0.488500029605451,-0.480121961098349,
-0.475419822411446,-0.443204075940068,-0.411200944373518,-0.380156597583109,
-0.360196283409126,-0.353873717113103,-0.349018195039205,-0.318315352453775,
-0.300315340887177,-0.269060639454171,-0.237672628214141,-0.231826094134014,
-0.227181047726769,-0.196613620435523,-0.166002976183476,-0.135781765031655,
-0.118809044402698,-0.114031241820972,-0.109476336553635,-0.0799052018350452,
-0.0507571470011222,-0.022522284006719,0.),.UNSPECIFIED.);
#4006=B_SPLINE_CURVE_WITH_KNOTS('',3,(#34259,#34260,#34261,#34262,#34263,
#34264,#34265,#34266,#34267,#34268,#34269,#34270,#34271,#34272,#34273,#34274,
#34275,#34276,#34277),.UNSPECIFIED.,.F.,.F.,(4,3,3,3,3,3,4),(95.3641731163798,
96.2028589542983,97.1946410053736,98.1864230564488,99.1782051075241,100.169987158599,
101.077602036598),.UNSPECIFIED.);
#4007=B_SPLINE_CURVE_WITH_KNOTS('',3,(#34279,#34280,#34281,#34282,#34283,
#34284,#34285,#34286,#34287,#34288,#34289,#34290,#34291,#34292,#34293,#34294,
#34295,#34296,#34297,#34298,#34299,#34300,#34301,#34302,#34303,#34304,#34305,
#34306,#34307,#34308,#34309,#34310,#34311,#34312,#34313,#34314,#34315,#34316,
#34317,#34318,#34319,#34320,#34321,#34322,#34323,#34324,#34325,#34326,#34327,
#34328,#34329,#34330,#34331,#34332,#34333,#34334,#34335,#34336,#34337,#34338,
#34339,#34340,#34341,#34342,#34343,#34344,#34345,#34346,#34347,#34348,#34349,
#34350,#34351,#34352,#34353,#34354,#34355,#34356,#34357,#34358,#34359,#34360,
#34361,#34362,#34363,#34364,#34365,#34366,#34367,#34368,#34369,#34370,#34371,
#34372),.UNSPECIFIED.,.F.,.F.,(4,3,3,3,3,3,3,3,3,3,3,3,3,3,3,3,3,3,3,3,
3,3,3,3,3,3,3,3,3,3,3,4),(-0.658260979006784,-0.633773279162306,-0.60511106550004,
-0.587935817558656,-0.582153877533815,-0.576676345808561,-0.545880189887229,
-0.518933553456064,-0.505287355660679,-0.500250742991463,-0.469731693480689,
-0.438742332174745,-0.407896509549881,-0.388499156771889,-0.383813916281054,
-0.37941122894066,-0.347601178541539,-0.33030709843791,-0.299505983293081,
-0.268122059993525,-0.260224018962276,-0.25550038819645,-0.223562839671894,
-0.191212858654853,-0.158617580462045,-0.13879038290429,-0.132403785254111,
-0.127529529765003,-0.0941940254338511,-0.060837309314193,-0.0281712889870458,
0.),.UNSPECIFIED.);
#4008=B_SPLINE_CURVE_WITH_KNOTS('',3,(#34373,#34374,#34375,#34376,#34377,
#34378,#34379,#34380,#34381),.UNSPECIFIED.,.F.,.F.,(4,1,1,1,1,1,4),(10.3761157273103,
11.2837306053091,12.2755126563843,13.2672947074596,14.2590767585348,15.25085880961,
15.7079632679489),.UNSPECIFIED.);
#4009=B_SPLINE_CURVE_WITH_KNOTS('',3,(#34387,#34388,#34389,#34390,#34391,
#34392,#34393,#34394,#34395,#34396,#34397,#34398,#34399,#34400,#34401,#34402,
#34403,#34404,#34405,#34406,#34407,#34408,#34409,#34410,#34411,#34412,#34413,
#34414,#34415,#34416,#34417,#34418,#34419,#34420,#34421,#34422,#34423,#34424,
#34425,#34426,#34427,#34428,#34429,#34430,#34431,#34432,#34433,#34434,#34435,
#34436,#34437,#34438,#34439,#34440,#34441,#34442,#34443,#34444,#34445,#34446,
#34447,#34448,#34449,#34450,#34451,#34452,#34453,#34454,#34455,#34456,#34457,
#34458,#34459,#34460,#34461,#34462,#34463,#34464,#34465,#34466,#34467,#34468,
#34469,#34470,#34471,#34472,#34473,#34474,#34475,#34476,#34477,#34478,#34479,
#34480,#34481,#34482,#34483),.UNSPECIFIED.,.F.,.F.,(4,3,3,3,3,3,3,3,3,3,
3,3,3,3,3,3,3,3,3,3,3,3,3,3,3,3,3,3,3,3,3,3,4),(-0.655752415918265,-0.626851741040643,
-0.593695046194504,-0.575358814612795,-0.568230240534389,-0.562615606353527,
-0.529721440557959,-0.501045678099109,-0.488500032023362,-0.480121968529048,
-0.475419837506024,-0.44320409140917,-0.411200962660038,-0.380156623791134,
-0.36019630306514,-0.353875988306761,-0.349018404483483,-0.318315565766959,
-0.300315340887157,-0.269060643749347,-0.237672631000559,-0.231826095923608,
-0.227181047488589,-0.196613622754405,-0.166002975418797,-0.135781755587927,
-0.118809036139436,-0.114031227885311,-0.109476333948085,-0.0799051921969754,
-0.0507571266588613,-0.0225222496686074,0.),.UNSPECIFIED.);
#4010=B_SPLINE_CURVE_WITH_KNOTS('',3,(#34486,#34487,#34488,#34489,#34490,
#34491,#34492,#34493),.UNSPECIFIED.,.F.,.F.,(4,1,1,1,1,4),(11.6150328478185,
12.6068148988938,13.598596949969,14.5903790010443,15.5821610521195,15.7079632679489),
 .UNSPECIFIED.);
#4011=B_SPLINE_CURVE_WITH_KNOTS('',3,(#34922,#34923,#34924,#34925,#34926,
#34927,#34928,#34929,#34930,#34931,#34932,#34933,#34934,#34935,#34936,#34937),
 .UNSPECIFIED.,.F.,.F.,(4,3,3,3,3,4),(-103.145333311825,-102.15355126075,
-101.161769209675,-100.169987158599,-99.1782051075241,-98.3407100278241),
 .UNSPECIFIED.);
#4012=B_SPLINE_CURVE_WITH_KNOTS('',3,(#34939,#34940,#34941,#34942,#34943,
#34944),.UNSPECIFIED.,.F.,.F.,(4,2,4),(-1.35394250197628,-0.852961572903344,
-0.599740178024191),.UNSPECIFIED.);
#4013=B_SPLINE_CURVE_WITH_KNOTS('',3,(#35217,#35218,#35219,#35220,#35221,
#35222,#35223,#35224,#35225,#35226,#35227,#35228,#35229,#35230,#35231,#35232,
#35233,#35234,#35235,#35236,#35237,#35238,#35239,#35240,#35241,#35242,#35243,
#35244,#35245,#35246,#35247,#35248,#35249,#35250,#35251,#35252,#35253,#35254,
#35255,#35256,#35257,#35258,#35259,#35260,#35261,#35262,#35263,#35264,#35265,
#35266,#35267,#35268,#35269,#35270,#35271,#35272,#35273,#35274,#35275,#35276,
#35277,#35278,#35279,#35280),.UNSPECIFIED.,.F.,.F.,(4,3,3,3,3,3,3,3,3,3,
3,3,3,3,3,3,3,3,3,3,3,4),(-12.8459374819259,-11.4794095531645,-10.7961455887838,
-10.3238102653841,-10.1128816244031,-9.79002513073258,-7.17546444804456,
-5.86818410670054,-5.21454393602854,-4.88772385069253,-4.68535987578927,
-4.56090376535653,-4.4207580398687,-3.48474489248014,-2.76035534391825,
-2.17493233268475,-1.74712655327371,-1.70292711374287,-1.28137423833841,
-0.996111179633922,-0.765912925479548,-0.621212683296683),.UNSPECIFIED.);
#4014=B_SPLINE_CURVE_WITH_KNOTS('',3,(#35282,#35283,#35284,#35285),
 .UNSPECIFIED.,.F.,.F.,(4,4),(0.258432097335974,0.335446700888131),
 .UNSPECIFIED.);
#4015=B_SPLINE_CURVE_WITH_KNOTS('',3,(#35289,#35290,#35291,#35292,#35293,
#35294),.UNSPECIFIED.,.F.,.F.,(4,2,4),(2.73646626800883,2.74754737169745,
2.77362936600561),.UNSPECIFIED.);
#4016=B_SPLINE_CURVE_WITH_KNOTS('',3,(#35295,#35296,#35297,#35298,#35299,
#35300),.UNSPECIFIED.,.F.,.F.,(4,2,4),(1.69951603754379,1.72559803185195,
1.73667913554058),.UNSPECIFIED.);
#4017=B_SPLINE_CURVE_WITH_KNOTS('',3,(#35302,#35303,#35304,#35305),
 .UNSPECIFIED.,.F.,.F.,(4,4),(0.258432097334697,0.335446700886078),
 .UNSPECIFIED.);
#4018=B_SPLINE_CURVE_WITH_KNOTS('',3,(#35310,#35311,#35312,#35313,#35314,
#35315),.UNSPECIFIED.,.F.,.F.,(4,2,4),(2.73646626801231,2.74754737170094,
2.77362936600909),.UNSPECIFIED.);
#4019=B_SPLINE_CURVE_WITH_KNOTS('',3,(#35316,#35317,#35318,#35319,#35320,
#35321),.UNSPECIFIED.,.F.,.F.,(4,2,4),(1.69951603754727,1.72559803185543,
1.73667913554406),.UNSPECIFIED.);
#4020=B_SPLINE_CURVE_WITH_KNOTS('',3,(#35323,#35324,#35325,#35326),
 .UNSPECIFIED.,.F.,.F.,(4,4),(0.258432097333565,0.335446700884273),
 .UNSPECIFIED.);
#4021=B_SPLINE_CURVE_WITH_KNOTS('',3,(#35331,#35332,#35333,#35334,#35335,
#35336),.UNSPECIFIED.,.F.,.F.,(4,2,4),(2.73646626800806,2.74754737169669,
2.77362936600484),.UNSPECIFIED.);
#4022=B_SPLINE_CURVE_WITH_KNOTS('',3,(#35337,#35338,#35339,#35340,#35341,
#35342),.UNSPECIFIED.,.F.,.F.,(4,2,4),(1.69951603754303,1.72559803185118,
1.73667913553981),.UNSPECIFIED.);
#4023=B_SPLINE_CURVE_WITH_KNOTS('',3,(#35344,#35345,#35346,#35347),
 .UNSPECIFIED.,.F.,.F.,(4,4),(0.258432097337429,0.335446700890448),
 .UNSPECIFIED.);
#4024=B_SPLINE_CURVE_WITH_KNOTS('',3,(#35352,#35353,#35354,#35355,#35356,
#35357),.UNSPECIFIED.,.F.,.F.,(4,2,4),(2.73646626800755,2.74754737169618,
2.77362936600433),.UNSPECIFIED.);
#4025=B_SPLINE_CURVE_WITH_KNOTS('',3,(#35358,#35359,#35360,#35361,#35362,
#35363),.UNSPECIFIED.,.F.,.F.,(4,2,4),(1.69951603754252,1.72559803185067,
1.7366791355393),.UNSPECIFIED.);
#4026=B_SPLINE_CURVE_WITH_KNOTS('',3,(#35365,#35366,#35367,#35368),
 .UNSPECIFIED.,.F.,.F.,(4,4),(0.258432097333234,0.335446700883742),
 .UNSPECIFIED.);
#4027=B_SPLINE_CURVE_WITH_KNOTS('',3,(#35373,#35374,#35375,#35376,#35377,
#35378),.UNSPECIFIED.,.F.,.F.,(4,2,4),(2.73646626801512,2.74754737170375,
2.77362936601191),.UNSPECIFIED.);
#4028=B_SPLINE_CURVE_WITH_KNOTS('',3,(#35379,#35380,#35381,#35382,#35383,
#35384),.UNSPECIFIED.,.F.,.F.,(4,2,4),(1.69951603755009,1.72559803185825,
1.73667913554687),.UNSPECIFIED.);
#4029=B_SPLINE_CURVE_WITH_KNOTS('',3,(#35386,#35387,#35388,#35389),
 .UNSPECIFIED.,.F.,.F.,(4,4),(0.258432097341974,0.335446700897715),
 .UNSPECIFIED.);
#4030=B_SPLINE_CURVE_WITH_KNOTS('',3,(#35394,#35395,#35396,#35397,#35398,
#35399),.UNSPECIFIED.,.F.,.F.,(4,2,4),(2.73646626801742,2.74754737170605,
2.7736293660142),.UNSPECIFIED.);
#4031=B_SPLINE_CURVE_WITH_KNOTS('',3,(#35400,#35401,#35402,#35403,#35404,
#35405),.UNSPECIFIED.,.F.,.F.,(4,2,4),(1.69951603755239,1.72559803186054,
1.73667913554917),.UNSPECIFIED.);
#4032=B_SPLINE_CURVE_WITH_KNOTS('',3,(#35407,#35408,#35409,#35410),
 .UNSPECIFIED.,.F.,.F.,(4,4),(0.258432097341738,0.335446700897338),
 .UNSPECIFIED.);
#4033=B_SPLINE_CURVE_WITH_KNOTS('',3,(#35415,#35416,#35417,#35418,#35419,
#35420),.UNSPECIFIED.,.F.,.F.,(4,2,4),(2.7364662680157,2.74754737170433,
2.77362936601248),.UNSPECIFIED.);
#4034=B_SPLINE_CURVE_WITH_KNOTS('',3,(#35421,#35422,#35423,#35424,#35425,
#35426),.UNSPECIFIED.,.F.,.F.,(4,2,4),(1.69951603755067,1.72559803185882,
1.73667913554745),.UNSPECIFIED.);
#4035=B_SPLINE_CURVE_WITH_KNOTS('',3,(#35428,#35429,#35430,#35431),
 .UNSPECIFIED.,.F.,.F.,(4,4),(0.258432097339649,0.335446700893994),
 .UNSPECIFIED.);
#4036=B_SPLINE_CURVE_WITH_KNOTS('',3,(#35436,#35437,#35438,#35439,#35440,
#35441),.UNSPECIFIED.,.F.,.F.,(4,2,4),(2.73646626801472,2.74754737170335,
2.7736293660115),.UNSPECIFIED.);
#4037=B_SPLINE_CURVE_WITH_KNOTS('',3,(#35442,#35443,#35444,#35445,#35446,
#35447),.UNSPECIFIED.,.F.,.F.,(4,2,4),(1.69951603754969,1.72559803185784,
1.73667913554647),.UNSPECIFIED.);
#4038=B_SPLINE_CURVE_WITH_KNOTS('',3,(#35449,#35450,#35451,#35452),
 .UNSPECIFIED.,.F.,.F.,(4,4),(0.258432097340253,0.335446700894965),
 .UNSPECIFIED.);
#4039=B_SPLINE_CURVE_WITH_KNOTS('',3,(#35457,#35458,#35459,#35460,#35461,
#35462),.UNSPECIFIED.,.F.,.F.,(4,2,4),(2.7364662680108,2.74754737169943,
2.77362936600758),.UNSPECIFIED.);
#4040=B_SPLINE_CURVE_WITH_KNOTS('',3,(#35463,#35464,#35465,#35466,#35467,
#35468),.UNSPECIFIED.,.F.,.F.,(4,2,4),(1.69951603754577,1.72559803185392,
1.73667913554255),.UNSPECIFIED.);
#4041=B_SPLINE_CURVE_WITH_KNOTS('',3,(#35470,#35471,#35472,#35473),
 .UNSPECIFIED.,.F.,.F.,(4,4),(0.258432097337265,0.33544670089019),
 .UNSPECIFIED.);
#4042=B_SPLINE_CURVE_WITH_KNOTS('',3,(#35477,#35478,#35479,#35480),
 .UNSPECIFIED.,.F.,.F.,(4,4),(0.258432097338423,0.335446700892038),
 .UNSPECIFIED.);
#4043=B_SPLINE_CURVE_WITH_KNOTS('',3,(#35484,#35485,#35486,#35487),
 .UNSPECIFIED.,.F.,.F.,(4,4),(0.258432097338034,0.335446700891419),
 .UNSPECIFIED.);
#4044=B_SPLINE_CURVE_WITH_KNOTS('',3,(#35507,#35508,#35509,#35510,#35511,
#35512),.UNSPECIFIED.,.F.,.F.,(4,2,4),(-2.32216477286167,-1.3409543646706,
-0.618253846678096),.UNSPECIFIED.);
#4045=B_SPLINE_CURVE_WITH_KNOTS('',3,(#35515,#35516,#35517,#35518),
 .UNSPECIFIED.,.F.,.F.,(4,4),(-2.64673758792282,-2.49658914637539),
 .UNSPECIFIED.);
#4046=B_SPLINE_CURVE_WITH_KNOTS('',3,(#35794,#35795,#35796,#35797,#35798,
#35799,#35800,#35801,#35802,#35803,#35804,#35805,#35806,#35807,#35808,#35809,
#35810,#35811,#35812,#35813),.UNSPECIFIED.,.F.,.F.,(4,2,2,2,2,2,2,2,2,4),
(0.,0.658822881651553,1.04966242800916,1.12777860787417,1.6152043752719,
2.27666472044823,2.65447358681698,2.96850721180304,2.98700678447604,3.25371381595271),
 .UNSPECIFIED.);
#4047=B_SPLINE_CURVE_WITH_KNOTS('',3,(#36016,#36017,#36018,#36019,#36020,
#36021),.UNSPECIFIED.,.F.,.F.,(4,2,4),(-2.32216477286167,-1.3409543646706,
-0.618253846678096),.UNSPECIFIED.);
#4048=B_SPLINE_CURVE_WITH_KNOTS('',3,(#36024,#36025,#36026,#36027),
 .UNSPECIFIED.,.F.,.F.,(4,4),(-2.64673758792282,-2.49658914637539),
 .UNSPECIFIED.);
#4049=B_SPLINE_CURVE_WITH_KNOTS('',3,(#36303,#36304,#36305,#36306,#36307,
#36308,#36309,#36310,#36311,#36312,#36313,#36314,#36315,#36316,#36317,#36318,
#36319,#36320,#36321,#36322),.UNSPECIFIED.,.F.,.F.,(4,2,2,2,2,2,2,2,2,4),
(0.,0.658822881651553,1.04966242800916,1.12777860787417,1.6152043752719,
2.27666472044823,2.65447358681698,2.96850721180304,2.98700678447604,3.25371381595271),
 .UNSPECIFIED.);
#4050=B_SPLINE_CURVE_WITH_KNOTS('',3,(#36535,#36536,#36537,#36538,#36539,
#36540),.UNSPECIFIED.,.F.,.F.,(4,2,4),(-2.32216477286167,-1.3409543646706,
-0.618253846678096),.UNSPECIFIED.);
#4051=B_SPLINE_CURVE_WITH_KNOTS('',3,(#36543,#36544,#36545,#36546),
 .UNSPECIFIED.,.F.,.F.,(4,4),(-2.64673758792282,-2.49658914637539),
 .UNSPECIFIED.);
#4052=B_SPLINE_CURVE_WITH_KNOTS('',3,(#36822,#36823,#36824,#36825,#36826,
#36827,#36828,#36829,#36830,#36831,#36832,#36833,#36834,#36835,#36836,#36837,
#36838,#36839,#36840,#36841),.UNSPECIFIED.,.F.,.F.,(4,2,2,2,2,2,2,2,2,4),
(0.,0.658822881651553,1.04966242800916,1.12777860787417,1.6152043752719,
2.27666472044823,2.65447358681698,2.96850721180304,2.98700678447604,3.25371381595271),
 .UNSPECIFIED.);
#4053=B_SPLINE_CURVE_WITH_KNOTS('',3,(#37034,#37035,#37036,#37037,#37038,
#37039),.UNSPECIFIED.,.F.,.F.,(4,2,4),(-2.32216477286167,-1.3409543646706,
-0.618253846678096),.UNSPECIFIED.);
#4054=B_SPLINE_CURVE_WITH_KNOTS('',3,(#37042,#37043,#37044,#37045),
 .UNSPECIFIED.,.F.,.F.,(4,4),(-2.64673758792282,-2.49658914637539),
 .UNSPECIFIED.);
#4055=B_SPLINE_CURVE_WITH_KNOTS('',3,(#37321,#37322,#37323,#37324,#37325,
#37326,#37327,#37328,#37329,#37330,#37331,#37332,#37333,#37334,#37335,#37336,
#37337,#37338,#37339,#37340),.UNSPECIFIED.,.F.,.F.,(4,2,2,2,2,2,2,2,2,4),
(0.,0.658822881651553,1.04966242800916,1.12777860787417,1.6152043752719,
2.27666472044823,2.65447358681698,2.96850721180304,2.98700678447604,3.25371381595271),
 .UNSPECIFIED.);
#4056=B_SPLINE_CURVE_WITH_KNOTS('',3,(#37543,#37544,#37545,#37546,#37547,
#37548),.UNSPECIFIED.,.F.,.F.,(4,2,4),(-2.32216477286167,-1.3409543646706,
-0.618253846678096),.UNSPECIFIED.);
#4057=B_SPLINE_CURVE_WITH_KNOTS('',3,(#37551,#37552,#37553,#37554),
 .UNSPECIFIED.,.F.,.F.,(4,4),(-2.64673758792282,-2.49658914637539),
 .UNSPECIFIED.);
#4058=B_SPLINE_CURVE_WITH_KNOTS('',3,(#37830,#37831,#37832,#37833,#37834,
#37835,#37836,#37837,#37838,#37839,#37840,#37841,#37842,#37843,#37844,#37845,
#37846,#37847,#37848,#37849),.UNSPECIFIED.,.F.,.F.,(4,2,2,2,2,2,2,2,2,4),
(0.,0.658822881651553,1.04966242800916,1.12777860787417,1.6152043752719,
2.27666472044823,2.65447358681698,2.96850721180304,2.98700678447604,3.25371381595271),
 .UNSPECIFIED.);
#4059=B_SPLINE_CURVE_WITH_KNOTS('',3,(#38062,#38063,#38064,#38065,#38066,
#38067),.UNSPECIFIED.,.F.,.F.,(4,2,4),(-2.32216477286167,-1.3409543646706,
-0.618253846678096),.UNSPECIFIED.);
#4060=B_SPLINE_CURVE_WITH_KNOTS('',3,(#38070,#38071,#38072,#38073),
 .UNSPECIFIED.,.F.,.F.,(4,4),(-2.64673758792282,-2.49658914637539),
 .UNSPECIFIED.);
#4061=B_SPLINE_CURVE_WITH_KNOTS('',3,(#38349,#38350,#38351,#38352,#38353,
#38354,#38355,#38356,#38357,#38358,#38359,#38360,#38361,#38362,#38363,#38364,
#38365,#38366,#38367,#38368),.UNSPECIFIED.,.F.,.F.,(4,2,2,2,2,2,2,2,2,4),
(0.,0.658822881651553,1.04966242800916,1.12777860787417,1.6152043752719,
2.27666472044823,2.65447358681698,2.96850721180304,2.98700678447604,3.25371381595271),
 .UNSPECIFIED.);
#4062=B_SPLINE_CURVE_WITH_KNOTS('',3,(#38561,#38562,#38563,#38564,#38565,
#38566),.UNSPECIFIED.,.F.,.F.,(4,2,4),(-2.32216477286167,-1.3409543646706,
-0.618253846678096),.UNSPECIFIED.);
#4063=B_SPLINE_CURVE_WITH_KNOTS('',3,(#38569,#38570,#38571,#38572),
 .UNSPECIFIED.,.F.,.F.,(4,4),(-2.64673758792282,-2.49658914637539),
 .UNSPECIFIED.);
#4064=B_SPLINE_CURVE_WITH_KNOTS('',3,(#38848,#38849,#38850,#38851,#38852,
#38853,#38854,#38855,#38856,#38857,#38858,#38859,#38860,#38861,#38862,#38863,
#38864,#38865,#38866,#38867),.UNSPECIFIED.,.F.,.F.,(4,2,2,2,2,2,2,2,2,4),
(0.,0.658822881651553,1.04966242800916,1.12777860787417,1.6152043752719,
2.27666472044823,2.65447358681698,2.96850721180304,2.98700678447604,3.25371381595271),
 .UNSPECIFIED.);
#4065=B_SPLINE_CURVE_WITH_KNOTS('',3,(#39070,#39071,#39072,#39073,#39074,
#39075),.UNSPECIFIED.,.F.,.F.,(4,2,4),(-2.32216477286167,-1.3409543646706,
-0.618253846678096),.UNSPECIFIED.);
#4066=B_SPLINE_CURVE_WITH_KNOTS('',3,(#39078,#39079,#39080,#39081),
 .UNSPECIFIED.,.F.,.F.,(4,4),(-2.64673758792282,-2.49658914637539),
 .UNSPECIFIED.);
#4067=B_SPLINE_CURVE_WITH_KNOTS('',3,(#39357,#39358,#39359,#39360,#39361,
#39362,#39363,#39364,#39365,#39366,#39367,#39368,#39369,#39370,#39371,#39372,
#39373,#39374,#39375,#39376),.UNSPECIFIED.,.F.,.F.,(4,2,2,2,2,2,2,2,2,4),
(0.,0.658822881651553,1.04966242800916,1.12777860787417,1.6152043752719,
2.27666472044823,2.65447358681698,2.96850721180304,2.98700678447604,3.25371381595271),
 .UNSPECIFIED.);
#4068=B_SPLINE_CURVE_WITH_KNOTS('',3,(#39589,#39590,#39591,#39592,#39593,
#39594),.UNSPECIFIED.,.F.,.F.,(4,2,4),(-2.32216477286167,-1.3409543646706,
-0.618253846678096),.UNSPECIFIED.);
#4069=B_SPLINE_CURVE_WITH_KNOTS('',3,(#39597,#39598,#39599,#39600),
 .UNSPECIFIED.,.F.,.F.,(4,4),(-2.64673758792282,-2.49658914637539),
 .UNSPECIFIED.);
#4070=B_SPLINE_CURVE_WITH_KNOTS('',3,(#39876,#39877,#39878,#39879,#39880,
#39881,#39882,#39883,#39884,#39885,#39886,#39887,#39888,#39889,#39890,#39891,
#39892,#39893,#39894,#39895),.UNSPECIFIED.,.F.,.F.,(4,2,2,2,2,2,2,2,2,4),
(0.,0.658822881651553,1.04966242800916,1.12777860787417,1.6152043752719,
2.27666472044823,2.65447358681698,2.96850721180304,2.98700678447604,3.25371381595271),
 .UNSPECIFIED.);
#4071=B_SPLINE_CURVE_WITH_KNOTS('',3,(#40098,#40099,#40100,#40101,#40102,
#40103),.UNSPECIFIED.,.F.,.F.,(4,2,4),(-2.32216477286167,-1.3409543646706,
-0.618253846678096),.UNSPECIFIED.);
#4072=B_SPLINE_CURVE_WITH_KNOTS('',3,(#40106,#40107,#40108,#40109),
 .UNSPECIFIED.,.F.,.F.,(4,4),(-2.64673758792282,-2.49658914637539),
 .UNSPECIFIED.);
#4073=B_SPLINE_CURVE_WITH_KNOTS('',3,(#40385,#40386,#40387,#40388,#40389,
#40390,#40391,#40392,#40393,#40394,#40395,#40396,#40397,#40398,#40399,#40400,
#40401,#40402,#40403,#40404),.UNSPECIFIED.,.F.,.F.,(4,2,2,2,2,2,2,2,2,4),
(0.,0.658822881651553,1.04966242800916,1.12777860787417,1.6152043752719,
2.27666472044823,2.65447358681698,2.96850721180304,2.98700678447604,3.25371381595271),
 .UNSPECIFIED.);
#4074=B_SPLINE_CURVE_WITH_KNOTS('',3,(#40607,#40608,#40609,#40610,#40611,
#40612),.UNSPECIFIED.,.F.,.F.,(4,2,4),(-2.32216477286167,-1.3409543646706,
-0.618253846678096),.UNSPECIFIED.);
#4075=B_SPLINE_CURVE_WITH_KNOTS('',3,(#40615,#40616,#40617,#40618),
 .UNSPECIFIED.,.F.,.F.,(4,4),(-2.64673758792282,-2.49658914637539),
 .UNSPECIFIED.);
#4076=B_SPLINE_CURVE_WITH_KNOTS('',3,(#40894,#40895,#40896,#40897,#40898,
#40899,#40900,#40901,#40902,#40903,#40904,#40905,#40906,#40907,#40908,#40909,
#40910,#40911,#40912,#40913),.UNSPECIFIED.,.F.,.F.,(4,2,2,2,2,2,2,2,2,4),
(0.,0.658822881651553,1.04966242800916,1.12777860787417,1.6152043752719,
2.27666472044823,2.65447358681698,2.96850721180304,2.98700678447604,3.25371381595271),
 .UNSPECIFIED.);
#4077=B_SPLINE_CURVE_WITH_KNOTS('',3,(#41126,#41127,#41128,#41129,#41130,
#41131),.UNSPECIFIED.,.F.,.F.,(4,2,4),(-2.32216477286167,-1.3409543646706,
-0.618253846678096),.UNSPECIFIED.);
#4078=B_SPLINE_CURVE_WITH_KNOTS('',3,(#41134,#41135,#41136,#41137),
 .UNSPECIFIED.,.F.,.F.,(4,4),(-2.64673758792282,-2.49658914637539),
 .UNSPECIFIED.);
#4079=B_SPLINE_CURVE_WITH_KNOTS('',3,(#41413,#41414,#41415,#41416,#41417,
#41418,#41419,#41420,#41421,#41422,#41423,#41424,#41425,#41426,#41427,#41428,
#41429,#41430,#41431,#41432),.UNSPECIFIED.,.F.,.F.,(4,2,2,2,2,2,2,2,2,4),
(0.,0.658822881651553,1.04966242800916,1.12777860787417,1.6152043752719,
2.27666472044823,2.65447358681698,2.96850721180304,2.98700678447604,3.25371381595271),
 .UNSPECIFIED.);
#4500=LINE('',#23615,#5912);
#4501=LINE('',#23639,#5913);
#4502=LINE('',#23687,#5914);
#4503=LINE('',#23735,#5915);
#4504=LINE('',#23789,#5916);
#4505=LINE('',#23837,#5917);
#4506=LINE('',#23885,#5918);
#4507=LINE('',#23939,#5919);
#4508=LINE('',#23987,#5920);
#4509=LINE('',#24035,#5921);
#4510=LINE('',#24089,#5922);
#4511=LINE('',#24137,#5923);
#4512=LINE('',#24185,#5924);
#4513=LINE('',#24239,#5925);
#4514=LINE('',#24287,#5926);
#4515=LINE('',#24335,#5927);
#4516=LINE('',#26593,#5928);
#4517=LINE('',#26611,#5929);
#4518=LINE('',#26636,#5930);
#4519=LINE('',#26661,#5931);
#4520=LINE('',#26685,#5932);
#4521=LINE('',#26710,#5933);
#4522=LINE('',#26735,#5934);
#4523=LINE('',#26759,#5935);
#4524=LINE('',#26784,#5936);
#4525=LINE('',#26809,#5937);
#4526=LINE('',#26833,#5938);
#4527=LINE('',#26858,#5939);
#4528=LINE('',#26883,#5940);
#4529=LINE('',#26907,#5941);
#4530=LINE('',#26932,#5942);
#4531=LINE('',#26957,#5943);
#4532=LINE('',#26982,#5944);
#4533=LINE('',#26988,#5945);
#4534=LINE('',#26996,#5946);
#4535=LINE('',#26998,#5947);
#4536=LINE('',#27000,#5948);
#4537=LINE('',#27002,#5949);
#4538=LINE('',#27003,#5950);
#4539=LINE('',#27006,#5951);
#4540=LINE('',#27008,#5952);
#4541=LINE('',#27009,#5953);
#4542=LINE('',#27012,#5954);
#4543=LINE('',#27014,#5955);
#4544=LINE('',#27015,#5956);
#4545=LINE('',#27018,#5957);
#4546=LINE('',#27020,#5958);
#4547=LINE('',#27021,#5959);
#4548=LINE('',#27025,#5960);
#4549=LINE('',#27027,#5961);
#4550=LINE('',#27029,#5962);
#4551=LINE('',#27031,#5963);
#4552=LINE('',#27032,#5964);
#4553=LINE('',#27035,#5965);
#4554=LINE('',#27037,#5966);
#4555=LINE('',#27038,#5967);
#4556=LINE('',#27041,#5968);
#4557=LINE('',#27043,#5969);
#4558=LINE('',#27044,#5970);
#4559=LINE('',#27046,#5971);
#4560=LINE('',#27047,#5972);
#4561=LINE('',#27051,#5973);
#4562=LINE('',#27053,#5974);
#4563=LINE('',#27055,#5975);
#4564=LINE('',#27057,#5976);
#4565=LINE('',#27058,#5977);
#4566=LINE('',#27061,#5978);
#4567=LINE('',#27063,#5979);
#4568=LINE('',#27064,#5980);
#4569=LINE('',#27067,#5981);
#4570=LINE('',#27069,#5982);
#4571=LINE('',#27070,#5983);
#4572=LINE('',#27072,#5984);
#4573=LINE('',#27073,#5985);
#4574=LINE('',#27077,#5986);
#4575=LINE('',#27079,#5987);
#4576=LINE('',#27081,#5988);
#4577=LINE('',#27083,#5989);
#4578=LINE('',#27084,#5990);
#4579=LINE('',#27087,#5991);
#4580=LINE('',#27089,#5992);
#4581=LINE('',#27090,#5993);
#4582=LINE('',#27093,#5994);
#4583=LINE('',#27095,#5995);
#4584=LINE('',#27096,#5996);
#4585=LINE('',#27098,#5997);
#4586=LINE('',#27099,#5998);
#4587=LINE('',#27103,#5999);
#4588=LINE('',#27105,#6000);
#4589=LINE('',#27107,#6001);
#4590=LINE('',#27109,#6002);
#4591=LINE('',#27110,#6003);
#4592=LINE('',#27113,#6004);
#4593=LINE('',#27115,#6005);
#4594=LINE('',#27116,#6006);
#4595=LINE('',#27119,#6007);
#4596=LINE('',#27121,#6008);
#4597=LINE('',#27122,#6009);
#4598=LINE('',#27124,#6010);
#4599=LINE('',#27125,#6011);
#4600=LINE('',#27129,#6012);
#4601=LINE('',#27131,#6013);
#4602=LINE('',#27133,#6014);
#4603=LINE('',#27135,#6015);
#4604=LINE('',#27136,#6016);
#4605=LINE('',#27138,#6017);
#4606=LINE('',#27140,#6018);
#4607=LINE('',#27141,#6019);
#4608=LINE('',#27144,#6020);
#4609=LINE('',#27145,#6021);
#4610=LINE('',#27148,#6022);
#4611=LINE('',#27150,#6023);
#4612=LINE('',#27151,#6024);
#4613=LINE('',#27155,#6025);
#4614=LINE('',#27157,#6026);
#4615=LINE('',#27159,#6027);
#4616=LINE('',#27161,#6028);
#4617=LINE('',#27162,#6029);
#4618=LINE('',#27164,#6030);
#4619=LINE('',#27166,#6031);
#4620=LINE('',#27167,#6032);
#4621=LINE('',#27170,#6033);
#4622=LINE('',#27171,#6034);
#4623=LINE('',#27175,#6035);
#4624=LINE('',#27177,#6036);
#4625=LINE('',#27179,#6037);
#4626=LINE('',#27181,#6038);
#4627=LINE('',#27182,#6039);
#4628=LINE('',#27185,#6040);
#4629=LINE('',#27187,#6041);
#4630=LINE('',#27188,#6042);
#4631=LINE('',#27191,#6043);
#4632=LINE('',#27193,#6044);
#4633=LINE('',#27194,#6045);
#4634=LINE('',#27197,#6046);
#4635=LINE('',#27199,#6047);
#4636=LINE('',#27200,#6048);
#4637=LINE('',#27204,#6049);
#4638=LINE('',#27206,#6050);
#4639=LINE('',#27208,#6051);
#4640=LINE('',#27210,#6052);
#4641=LINE('',#27211,#6053);
#4642=LINE('',#27213,#6054);
#4643=LINE('',#27215,#6055);
#4644=LINE('',#27216,#6056);
#4645=LINE('',#27219,#6057);
#4646=LINE('',#27220,#6058);
#4647=LINE('',#27223,#6059);
#4648=LINE('',#27225,#6060);
#4649=LINE('',#27226,#6061);
#4650=LINE('',#27230,#6062);
#4651=LINE('',#27232,#6063);
#4652=LINE('',#27234,#6064);
#4653=LINE('',#27236,#6065);
#4654=LINE('',#27237,#6066);
#4655=LINE('',#27239,#6067);
#4656=LINE('',#27241,#6068);
#4657=LINE('',#27242,#6069);
#4658=LINE('',#27245,#6070);
#4659=LINE('',#27246,#6071);
#4660=LINE('',#27249,#6072);
#4661=LINE('',#27251,#6073);
#4662=LINE('',#27252,#6074);
#4663=LINE('',#27256,#6075);
#4664=LINE('',#27258,#6076);
#4665=LINE('',#27260,#6077);
#4666=LINE('',#27262,#6078);
#4667=LINE('',#27263,#6079);
#4668=LINE('',#27265,#6080);
#4669=LINE('',#27267,#6081);
#4670=LINE('',#27268,#6082);
#4671=LINE('',#27271,#6083);
#4672=LINE('',#27272,#6084);
#4673=LINE('',#27275,#6085);
#4674=LINE('',#27277,#6086);
#4675=LINE('',#27278,#6087);
#4676=LINE('',#27282,#6088);
#4677=LINE('',#27284,#6089);
#4678=LINE('',#27286,#6090);
#4679=LINE('',#27288,#6091);
#4680=LINE('',#27289,#6092);
#4681=LINE('',#27291,#6093);
#4682=LINE('',#27293,#6094);
#4683=LINE('',#27294,#6095);
#4684=LINE('',#27297,#6096);
#4685=LINE('',#27298,#6097);
#4686=LINE('',#27300,#6098);
#4687=LINE('',#27301,#6099);
#4688=LINE('',#32833,#6100);
#4689=LINE('',#32841,#6101);
#4690=LINE('',#32846,#6102);
#4691=LINE('',#32853,#6103);
#4692=LINE('',#32862,#6104);
#4693=LINE('',#32871,#6105);
#4694=LINE('',#32914,#6106);
#4695=LINE('',#32921,#6107);
#4696=LINE('',#32945,#6108);
#4697=LINE('',#32949,#6109);
#4698=LINE('',#32974,#6110);
#4699=LINE('',#32981,#6111);
#4700=LINE('',#33005,#6112);
#4701=LINE('',#33009,#6113);
#4702=LINE('',#33034,#6114);
#4703=LINE('',#33041,#6115);
#4704=LINE('',#33065,#6116);
#4705=LINE('',#33069,#6117);
#4706=LINE('',#33094,#6118);
#4707=LINE('',#33101,#6119);
#4708=LINE('',#33125,#6120);
#4709=LINE('',#33129,#6121);
#4710=LINE('',#33154,#6122);
#4711=LINE('',#33161,#6123);
#4712=LINE('',#33223,#6124);
#4713=LINE('',#33228,#6125);
#4714=LINE('',#33245,#6126);
#4715=LINE('',#33265,#6127);
#4716=LINE('',#33280,#6128);
#4717=LINE('',#33287,#6129);
#4718=LINE('',#33319,#6130);
#4719=LINE('',#33324,#6131);
#4720=LINE('',#33336,#6132);
#4721=LINE('',#33343,#6133);
#4722=LINE('',#33375,#6134);
#4723=LINE('',#33380,#6135);
#4724=LINE('',#33392,#6136);
#4725=LINE('',#33399,#6137);
#4726=LINE('',#33431,#6138);
#4727=LINE('',#33436,#6139);
#4728=LINE('',#33448,#6140);
#4729=LINE('',#33455,#6141);
#4730=LINE('',#33487,#6142);
#4731=LINE('',#33492,#6143);
#4732=LINE('',#33504,#6144);
#4733=LINE('',#33511,#6145);
#4734=LINE('',#33543,#6146);
#4735=LINE('',#33548,#6147);
#4736=LINE('',#33553,#6148);
#4737=LINE('',#33583,#6149);
#4738=LINE('',#33590,#6150);
#4739=LINE('',#33602,#6151);
#4740=LINE('',#35493,#6152);
#4741=LINE('',#35502,#6153);
#4742=LINE('',#35504,#6154);
#4743=LINE('',#41624,#6155);
#4744=LINE('',#41625,#6156);
#4745=LINE('',#41627,#6157);
#4746=LINE('',#41629,#6158);
#4747=LINE('',#41631,#6159);
#4748=LINE('',#41633,#6160);
#4749=LINE('',#41635,#6161);
#4750=LINE('',#41637,#6162);
#4751=LINE('',#41640,#6163);
#4752=LINE('',#41642,#6164);
#4753=LINE('',#41644,#6165);
#4754=LINE('',#41646,#6166);
#4755=LINE('',#41648,#6167);
#4756=LINE('',#41650,#6168);
#4757=LINE('',#41655,#6169);
#4758=LINE('',#41657,#6170);
#4759=LINE('',#41659,#6171);
#4760=LINE('',#41663,#6172);
#4761=LINE('',#41670,#6173);
#4762=LINE('',#41674,#6174);
#4763=LINE('',#41678,#6175);
#4764=LINE('',#41682,#6176);
#4765=LINE('',#41689,#6177);
#4766=LINE('',#41693,#6178);
#4767=LINE('',#41697,#6179);
#4768=LINE('',#41701,#6180);
#4769=LINE('',#41705,#6181);
#4770=LINE('',#41707,#6182);
#4771=LINE('',#41713,#6183);
#5912=VECTOR('',#19684,3.5);
#5913=VECTOR('',#19689,3.5);
#5914=VECTOR('',#19692,3.5);
#5915=VECTOR('',#19695,3.5);
#5916=VECTOR('',#19698,3.5);
#5917=VECTOR('',#19701,3.5);
#5918=VECTOR('',#19704,3.5);
#5919=VECTOR('',#19707,3.5);
#5920=VECTOR('',#19710,3.5);
#5921=VECTOR('',#19713,3.5);
#5922=VECTOR('',#19716,3.5);
#5923=VECTOR('',#19719,3.5);
#5924=VECTOR('',#19722,3.5);
#5925=VECTOR('',#19725,3.5);
#5926=VECTOR('',#19728,3.5);
#5927=VECTOR('',#19731,3.5);
#5928=VECTOR('',#19780,2.872);
#5929=VECTOR('',#19785,2.872);
#5930=VECTOR('',#19788,2.872);
#5931=VECTOR('',#19791,2.872);
#5932=VECTOR('',#19794,2.872);
#5933=VECTOR('',#19797,2.872);
#5934=VECTOR('',#19800,2.872);
#5935=VECTOR('',#19803,2.872);
#5936=VECTOR('',#19806,2.872);
#5937=VECTOR('',#19809,2.872);
#5938=VECTOR('',#19812,2.872);
#5939=VECTOR('',#19815,2.872);
#5940=VECTOR('',#19818,2.872);
#5941=VECTOR('',#19821,2.872);
#5942=VECTOR('',#19824,2.872);
#5943=VECTOR('',#19827,2.872);
#5944=VECTOR('',#19832,9.87862393885688);
#5945=VECTOR('',#19839,10.3);
#5946=VECTOR('',#19848,10.);
#5947=VECTOR('',#19849,10.);
#5948=VECTOR('',#19850,10.);
#5949=VECTOR('',#19851,10.);
#5950=VECTOR('',#19852,10.);
#5951=VECTOR('',#19855,10.);
#5952=VECTOR('',#19856,10.);
#5953=VECTOR('',#19857,10.);
#5954=VECTOR('',#19860,10.);
#5955=VECTOR('',#19861,10.);
#5956=VECTOR('',#19862,10.);
#5957=VECTOR('',#19865,10.);
#5958=VECTOR('',#19866,10.);
#5959=VECTOR('',#19867,10.);
#5960=VECTOR('',#19870,10.);
#5961=VECTOR('',#19871,10.);
#5962=VECTOR('',#19872,10.);
#5963=VECTOR('',#19873,10.);
#5964=VECTOR('',#19874,10.);
#5965=VECTOR('',#19877,10.);
#5966=VECTOR('',#19878,10.);
#5967=VECTOR('',#19879,10.);
#5968=VECTOR('',#19882,10.);
#5969=VECTOR('',#19883,10.);
#5970=VECTOR('',#19884,10.);
#5971=VECTOR('',#19887,10.);
#5972=VECTOR('',#19888,10.);
#5973=VECTOR('',#19891,10.);
#5974=VECTOR('',#19892,10.);
#5975=VECTOR('',#19893,10.);
#5976=VECTOR('',#19894,10.);
#5977=VECTOR('',#19895,10.);
#5978=VECTOR('',#19898,10.);
#5979=VECTOR('',#19899,10.);
#5980=VECTOR('',#19900,10.);
#5981=VECTOR('',#19903,10.);
#5982=VECTOR('',#19904,10.);
#5983=VECTOR('',#19905,10.);
#5984=VECTOR('',#19908,10.);
#5985=VECTOR('',#19909,10.);
#5986=VECTOR('',#19912,10.);
#5987=VECTOR('',#19913,10.);
#5988=VECTOR('',#19914,10.);
#5989=VECTOR('',#19915,10.);
#5990=VECTOR('',#19916,10.);
#5991=VECTOR('',#19919,10.);
#5992=VECTOR('',#19920,10.);
#5993=VECTOR('',#19921,10.);
#5994=VECTOR('',#19924,10.);
#5995=VECTOR('',#19925,10.);
#5996=VECTOR('',#19926,10.);
#5997=VECTOR('',#19929,10.);
#5998=VECTOR('',#19930,10.);
#5999=VECTOR('',#19933,10.);
#6000=VECTOR('',#19934,10.);
#6001=VECTOR('',#19935,10.);
#6002=VECTOR('',#19936,10.);
#6003=VECTOR('',#19937,10.);
#6004=VECTOR('',#19940,10.);
#6005=VECTOR('',#19941,10.);
#6006=VECTOR('',#19942,10.);
#6007=VECTOR('',#19945,10.);
#6008=VECTOR('',#19946,10.);
#6009=VECTOR('',#19947,10.);
#6010=VECTOR('',#19950,10.);
#6011=VECTOR('',#19951,10.);
#6012=VECTOR('',#19954,10.);
#6013=VECTOR('',#19955,10.);
#6014=VECTOR('',#19956,10.);
#6015=VECTOR('',#19957,10.);
#6016=VECTOR('',#19958,10.);
#6017=VECTOR('',#19961,10.);
#6018=VECTOR('',#19962,10.);
#6019=VECTOR('',#19963,10.);
#6020=VECTOR('',#19966,10.);
#6021=VECTOR('',#19967,10.);
#6022=VECTOR('',#19970,10.);
#6023=VECTOR('',#19971,10.);
#6024=VECTOR('',#19972,10.);
#6025=VECTOR('',#19975,10.);
#6026=VECTOR('',#19976,10.);
#6027=VECTOR('',#19977,10.);
#6028=VECTOR('',#19978,10.);
#6029=VECTOR('',#19979,10.);
#6030=VECTOR('',#19982,10.);
#6031=VECTOR('',#19983,10.);
#6032=VECTOR('',#19984,10.);
#6033=VECTOR('',#19987,10.);
#6034=VECTOR('',#19988,10.);
#6035=VECTOR('',#19991,10.);
#6036=VECTOR('',#19992,10.);
#6037=VECTOR('',#19993,10.);
#6038=VECTOR('',#19994,10.);
#6039=VECTOR('',#19995,10.);
#6040=VECTOR('',#19998,10.);
#6041=VECTOR('',#19999,10.);
#6042=VECTOR('',#20000,10.);
#6043=VECTOR('',#20003,10.);
#6044=VECTOR('',#20004,10.);
#6045=VECTOR('',#20005,10.);
#6046=VECTOR('',#20008,10.);
#6047=VECTOR('',#20009,10.);
#6048=VECTOR('',#20010,10.);
#6049=VECTOR('',#20013,10.);
#6050=VECTOR('',#20014,10.);
#6051=VECTOR('',#20015,10.);
#6052=VECTOR('',#20016,10.);
#6053=VECTOR('',#20017,10.);
#6054=VECTOR('',#20020,10.);
#6055=VECTOR('',#20021,10.);
#6056=VECTOR('',#20022,10.);
#6057=VECTOR('',#20025,10.);
#6058=VECTOR('',#20026,10.);
#6059=VECTOR('',#20029,10.);
#6060=VECTOR('',#20030,10.);
#6061=VECTOR('',#20031,10.);
#6062=VECTOR('',#20034,10.);
#6063=VECTOR('',#20035,10.);
#6064=VECTOR('',#20036,10.);
#6065=VECTOR('',#20037,10.);
#6066=VECTOR('',#20038,10.);
#6067=VECTOR('',#20041,10.);
#6068=VECTOR('',#20042,10.);
#6069=VECTOR('',#20043,10.);
#6070=VECTOR('',#20046,10.);
#6071=VECTOR('',#20047,10.);
#6072=VECTOR('',#20050,10.);
#6073=VECTOR('',#20051,10.);
#6074=VECTOR('',#20052,10.);
#6075=VECTOR('',#20055,10.);
#6076=VECTOR('',#20056,10.);
#6077=VECTOR('',#20057,10.);
#6078=VECTOR('',#20058,10.);
#6079=VECTOR('',#20059,10.);
#6080=VECTOR('',#20062,10.);
#6081=VECTOR('',#20063,10.);
#6082=VECTOR('',#20064,10.);
#6083=VECTOR('',#20067,10.);
#6084=VECTOR('',#20068,10.);
#6085=VECTOR('',#20071,10.);
#6086=VECTOR('',#20072,10.);
#6087=VECTOR('',#20073,10.);
#6088=VECTOR('',#20076,10.);
#6089=VECTOR('',#20077,10.);
#6090=VECTOR('',#20078,10.);
#6091=VECTOR('',#20079,10.);
#6092=VECTOR('',#20080,10.);
#6093=VECTOR('',#20083,10.);
#6094=VECTOR('',#20084,10.);
#6095=VECTOR('',#20085,10.);
#6096=VECTOR('',#20088,10.);
#6097=VECTOR('',#20089,10.);
#6098=VECTOR('',#20092,10.);
#6099=VECTOR('',#20093,10.);
#6100=VECTOR('',#20218,8.95);
#6101=VECTOR('',#20229,9.2);
#6102=VECTOR('',#20234,8.95);
#6103=VECTOR('',#20243,9.2);
#6104=VECTOR('',#20248,10.);
#6105=VECTOR('',#20249,10.);
#6106=VECTOR('',#20270,10.);
#6107=VECTOR('',#20273,10.);
#6108=VECTOR('',#20282,10.);
#6109=VECTOR('',#20283,10.);
#6110=VECTOR('',#20298,10.);
#6111=VECTOR('',#20301,10.);
#6112=VECTOR('',#20310,10.);
#6113=VECTOR('',#20311,10.);
#6114=VECTOR('',#20326,10.);
#6115=VECTOR('',#20329,10.);
#6116=VECTOR('',#20338,10.);
#6117=VECTOR('',#20339,10.);
#6118=VECTOR('',#20354,10.);
#6119=VECTOR('',#20357,10.);
#6120=VECTOR('',#20366,10.);
#6121=VECTOR('',#20367,10.);
#6122=VECTOR('',#20382,10.);
#6123=VECTOR('',#20385,10.);
#6124=VECTOR('',#20428,10.);
#6125=VECTOR('',#20429,10.);
#6126=VECTOR('',#20436,10.);
#6127=VECTOR('',#20441,10.);
#6128=VECTOR('',#20450,10.);
#6129=VECTOR('',#20453,10.);
#6130=VECTOR('',#20464,10.);
#6131=VECTOR('',#20465,10.);
#6132=VECTOR('',#20474,10.);
#6133=VECTOR('',#20477,10.);
#6134=VECTOR('',#20488,10.);
#6135=VECTOR('',#20489,10.);
#6136=VECTOR('',#20498,10.);
#6137=VECTOR('',#20501,10.);
#6138=VECTOR('',#20512,10.);
#6139=VECTOR('',#20513,10.);
#6140=VECTOR('',#20522,10.);
#6141=VECTOR('',#20525,10.);
#6142=VECTOR('',#20536,10.);
#6143=VECTOR('',#20537,10.);
#6144=VECTOR('',#20546,10.);
#6145=VECTOR('',#20549,10.);
#6146=VECTOR('',#20560,10.);
#6147=VECTOR('',#20561,10.);
#6148=VECTOR('',#20566,10.);
#6149=VECTOR('',#20583,10.);
#6150=VECTOR('',#20586,10.);
#6151=VECTOR('',#20593,10.);
#6152=VECTOR('',#20730,8.5);
#6153=VECTOR('',#20743,9.2);
#6154=VECTOR('',#20746,7.7);
#6155=VECTOR('',#20821,10.);
#6156=VECTOR('',#20822,10.);
#6157=VECTOR('',#20825,10.);
#6158=VECTOR('',#20828,10.);
#6159=VECTOR('',#20831,10.);
#6160=VECTOR('',#20834,10.);
#6161=VECTOR('',#20837,10.);
#6162=VECTOR('',#20840,10.);
#6163=VECTOR('',#20845,10.);
#6164=VECTOR('',#20848,10.);
#6165=VECTOR('',#20851,10.);
#6166=VECTOR('',#20854,10.);
#6167=VECTOR('',#20857,10.);
#6168=VECTOR('',#20860,10.);
#6169=VECTOR('',#20867,13.);
#6170=VECTOR('',#20870,11.3);
#6171=VECTOR('',#20873,9.);
#6172=VECTOR('',#20878,9.);
#6173=VECTOR('',#20887,6.7);
#6174=VECTOR('',#20892,5.85);
#6175=VECTOR('',#20897,5.5);
#6176=VECTOR('',#20902,5.35);
#6177=VECTOR('',#20911,3.3);
#6178=VECTOR('',#20916,3.4);
#6179=VECTOR('',#20921,3.5);
#6180=VECTOR('',#20926,3.2);
#6181=VECTOR('',#20931,2.9);
#6182=VECTOR('',#20934,3.2);
#6183=VECTOR('',#20943,3.25);
#7324=VERTEX_POINT('',#23613);
#7325=VERTEX_POINT('',#23614);
#7326=VERTEX_POINT('',#23616);
#7327=VERTEX_POINT('',#23627);
#7328=VERTEX_POINT('',#23637);
#7329=VERTEX_POINT('',#23638);
#7330=VERTEX_POINT('',#23685);
#7331=VERTEX_POINT('',#23686);
#7332=VERTEX_POINT('',#23733);
#7333=VERTEX_POINT('',#23734);
#7334=VERTEX_POINT('',#23787);
#7335=VERTEX_POINT('',#23788);
#7336=VERTEX_POINT('',#23835);
#7337=VERTEX_POINT('',#23836);
#7338=VERTEX_POINT('',#23883);
#7339=VERTEX_POINT('',#23884);
#7340=VERTEX_POINT('',#23937);
#7341=VERTEX_POINT('',#23938);
#7342=VERTEX_POINT('',#23985);
#7343=VERTEX_POINT('',#23986);
#7344=VERTEX_POINT('',#24033);
#7345=VERTEX_POINT('',#24034);
#7346=VERTEX_POINT('',#24087);
#7347=VERTEX_POINT('',#24088);
#7348=VERTEX_POINT('',#24135);
#7349=VERTEX_POINT('',#24136);
#7350=VERTEX_POINT('',#24183);
#7351=VERTEX_POINT('',#24184);
#7352=VERTEX_POINT('',#24237);
#7353=VERTEX_POINT('',#24238);
#7354=VERTEX_POINT('',#24285);
#7355=VERTEX_POINT('',#24286);
#7356=VERTEX_POINT('',#24333);
#7357=VERTEX_POINT('',#24334);
#7358=VERTEX_POINT('',#24656);
#7359=VERTEX_POINT('',#24657);
#7360=VERTEX_POINT('',#24669);
#7361=VERTEX_POINT('',#24683);
#7362=VERTEX_POINT('',#24690);
#7363=VERTEX_POINT('',#24695);
#7364=VERTEX_POINT('',#24703);
#7365=VERTEX_POINT('',#24771);
#7366=VERTEX_POINT('',#24773);
#7367=VERTEX_POINT('',#24778);
#7368=VERTEX_POINT('',#24785);
#7369=VERTEX_POINT('',#24790);
#7370=VERTEX_POINT('',#24792);
#7371=VERTEX_POINT('',#24866);
#7372=VERTEX_POINT('',#24873);
#7373=VERTEX_POINT('',#24941);
#7374=VERTEX_POINT('',#24943);
#7375=VERTEX_POINT('',#24948);
#7376=VERTEX_POINT('',#24953);
#7377=VERTEX_POINT('',#24958);
#7378=VERTEX_POINT('',#24960);
#7379=VERTEX_POINT('',#25034);
#7380=VERTEX_POINT('',#25041);
#7381=VERTEX_POINT('',#25109);
#7382=VERTEX_POINT('',#25111);
#7383=VERTEX_POINT('',#25116);
#7384=VERTEX_POINT('',#25123);
#7385=VERTEX_POINT('',#25128);
#7386=VERTEX_POINT('',#25130);
#7387=VERTEX_POINT('',#25204);
#7388=VERTEX_POINT('',#25211);
#7389=VERTEX_POINT('',#25279);
#7390=VERTEX_POINT('',#25281);
#7391=VERTEX_POINT('',#25286);
#7392=VERTEX_POINT('',#25293);
#7393=VERTEX_POINT('',#25298);
#7394=VERTEX_POINT('',#25300);
#7395=VERTEX_POINT('',#25374);
#7396=VERTEX_POINT('',#25381);
#7397=VERTEX_POINT('',#25449);
#7398=VERTEX_POINT('',#25451);
#7399=VERTEX_POINT('',#25456);
#7400=VERTEX_POINT('',#25461);
#7401=VERTEX_POINT('',#25466);
#7402=VERTEX_POINT('',#25468);
#7403=VERTEX_POINT('',#25542);
#7404=VERTEX_POINT('',#25549);
#7405=VERTEX_POINT('',#25617);
#7406=VERTEX_POINT('',#25619);
#7407=VERTEX_POINT('',#25624);
#7408=VERTEX_POINT('',#25631);
#7409=VERTEX_POINT('',#25636);
#7410=VERTEX_POINT('',#25638);
#7411=VERTEX_POINT('',#25712);
#7412=VERTEX_POINT('',#25719);
#7413=VERTEX_POINT('',#25787);
#7414=VERTEX_POINT('',#25789);
#7415=VERTEX_POINT('',#25794);
#7416=VERTEX_POINT('',#25801);
#7417=VERTEX_POINT('',#25806);
#7418=VERTEX_POINT('',#25808);
#7419=VERTEX_POINT('',#25882);
#7420=VERTEX_POINT('',#25889);
#7421=VERTEX_POINT('',#25957);
#7422=VERTEX_POINT('',#25959);
#7423=VERTEX_POINT('',#25964);
#7424=VERTEX_POINT('',#25969);
#7425=VERTEX_POINT('',#25974);
#7426=VERTEX_POINT('',#25976);
#7427=VERTEX_POINT('',#26050);
#7428=VERTEX_POINT('',#26057);
#7429=VERTEX_POINT('',#26125);
#7430=VERTEX_POINT('',#26127);
#7431=VERTEX_POINT('',#26132);
#7432=VERTEX_POINT('',#26139);
#7433=VERTEX_POINT('',#26144);
#7434=VERTEX_POINT('',#26146);
#7435=VERTEX_POINT('',#26220);
#7436=VERTEX_POINT('',#26227);
#7437=VERTEX_POINT('',#26295);
#7438=VERTEX_POINT('',#26297);
#7439=VERTEX_POINT('',#26302);
#7440=VERTEX_POINT('',#26309);
#7441=VERTEX_POINT('',#26314);
#7442=VERTEX_POINT('',#26316);
#7443=VERTEX_POINT('',#26390);
#7444=VERTEX_POINT('',#26397);
#7445=VERTEX_POINT('',#26465);
#7446=VERTEX_POINT('',#26467);
#7447=VERTEX_POINT('',#26472);
#7448=VERTEX_POINT('',#26477);
#7449=VERTEX_POINT('',#26482);
#7450=VERTEX_POINT('',#26484);
#7451=VERTEX_POINT('',#26558);
#7452=VERTEX_POINT('',#26591);
#7453=VERTEX_POINT('',#26592);
#7454=VERTEX_POINT('',#26594);
#7455=VERTEX_POINT('',#26601);
#7456=VERTEX_POINT('',#26609);
#7457=VERTEX_POINT('',#26610);
#7458=VERTEX_POINT('',#26634);
#7459=VERTEX_POINT('',#26635);
#7460=VERTEX_POINT('',#26659);
#7461=VERTEX_POINT('',#26660);
#7462=VERTEX_POINT('',#26683);
#7463=VERTEX_POINT('',#26684);
#7464=VERTEX_POINT('',#26708);
#7465=VERTEX_POINT('',#26709);
#7466=VERTEX_POINT('',#26733);
#7467=VERTEX_POINT('',#26734);
#7468=VERTEX_POINT('',#26757);
#7469=VERTEX_POINT('',#26758);
#7470=VERTEX_POINT('',#26782);
#7471=VERTEX_POINT('',#26783);
#7472=VERTEX_POINT('',#26807);
#7473=VERTEX_POINT('',#26808);
#7474=VERTEX_POINT('',#26831);
#7475=VERTEX_POINT('',#26832);
#7476=VERTEX_POINT('',#26856);
#7477=VERTEX_POINT('',#26857);
#7478=VERTEX_POINT('',#26881);
#7479=VERTEX_POINT('',#26882);
#7480=VERTEX_POINT('',#26905);
#7481=VERTEX_POINT('',#26906);
#7482=VERTEX_POINT('',#26930);
#7483=VERTEX_POINT('',#26931);
#7484=VERTEX_POINT('',#26955);
#7485=VERTEX_POINT('',#26956);
#7486=VERTEX_POINT('',#26979);
#7487=VERTEX_POINT('',#26981);
#7488=VERTEX_POINT('',#26983);
#7489=VERTEX_POINT('',#26987);
#7490=VERTEX_POINT('',#26991);
#7491=VERTEX_POINT('',#26994);
#7492=VERTEX_POINT('',#26995);
#7493=VERTEX_POINT('',#26997);
#7494=VERTEX_POINT('',#26999);
#7495=VERTEX_POINT('',#27001);
#7496=VERTEX_POINT('',#27005);
#7497=VERTEX_POINT('',#27007);
#7498=VERTEX_POINT('',#27011);
#7499=VERTEX_POINT('',#27013);
#7500=VERTEX_POINT('',#27017);
#7501=VERTEX_POINT('',#27019);
#7502=VERTEX_POINT('',#27023);
#7503=VERTEX_POINT('',#27024);
#7504=VERTEX_POINT('',#27026);
#7505=VERTEX_POINT('',#27028);
#7506=VERTEX_POINT('',#27030);
#7507=VERTEX_POINT('',#27034);
#7508=VERTEX_POINT('',#27036);
#7509=VERTEX_POINT('',#27040);
#7510=VERTEX_POINT('',#27042);
#7511=VERTEX_POINT('',#27049);
#7512=VERTEX_POINT('',#27050);
#7513=VERTEX_POINT('',#27052);
#7514=VERTEX_POINT('',#27054);
#7515=VERTEX_POINT('',#27056);
#7516=VERTEX_POINT('',#27060);
#7517=VERTEX_POINT('',#27062);
#7518=VERTEX_POINT('',#27066);
#7519=VERTEX_POINT('',#27068);
#7520=VERTEX_POINT('',#27075);
#7521=VERTEX_POINT('',#27076);
#7522=VERTEX_POINT('',#27078);
#7523=VERTEX_POINT('',#27080);
#7524=VERTEX_POINT('',#27082);
#7525=VERTEX_POINT('',#27086);
#7526=VERTEX_POINT('',#27088);
#7527=VERTEX_POINT('',#27092);
#7528=VERTEX_POINT('',#27094);
#7529=VERTEX_POINT('',#27101);
#7530=VERTEX_POINT('',#27102);
#7531=VERTEX_POINT('',#27104);
#7532=VERTEX_POINT('',#27106);
#7533=VERTEX_POINT('',#27108);
#7534=VERTEX_POINT('',#27112);
#7535=VERTEX_POINT('',#27114);
#7536=VERTEX_POINT('',#27118);
#7537=VERTEX_POINT('',#27120);
#7538=VERTEX_POINT('',#27127);
#7539=VERTEX_POINT('',#27128);
#7540=VERTEX_POINT('',#27130);
#7541=VERTEX_POINT('',#27132);
#7542=VERTEX_POINT('',#27134);
#7543=VERTEX_POINT('',#27139);
#7544=VERTEX_POINT('',#27143);
#7545=VERTEX_POINT('',#27147);
#7546=VERTEX_POINT('',#27149);
#7547=VERTEX_POINT('',#27153);
#7548=VERTEX_POINT('',#27154);
#7549=VERTEX_POINT('',#27156);
#7550=VERTEX_POINT('',#27158);
#7551=VERTEX_POINT('',#27160);
#7552=VERTEX_POINT('',#27165);
#7553=VERTEX_POINT('',#27169);
#7554=VERTEX_POINT('',#27173);
#7555=VERTEX_POINT('',#27174);
#7556=VERTEX_POINT('',#27176);
#7557=VERTEX_POINT('',#27178);
#7558=VERTEX_POINT('',#27180);
#7559=VERTEX_POINT('',#27184);
#7560=VERTEX_POINT('',#27186);
#7561=VERTEX_POINT('',#27190);
#7562=VERTEX_POINT('',#27192);
#7563=VERTEX_POINT('',#27196);
#7564=VERTEX_POINT('',#27198);
#7565=VERTEX_POINT('',#27202);
#7566=VERTEX_POINT('',#27203);
#7567=VERTEX_POINT('',#27205);
#7568=VERTEX_POINT('',#27207);
#7569=VERTEX_POINT('',#27209);
#7570=VERTEX_POINT('',#27214);
#7571=VERTEX_POINT('',#27218);
#7572=VERTEX_POINT('',#27222);
#7573=VERTEX_POINT('',#27224);
#7574=VERTEX_POINT('',#27228);
#7575=VERTEX_POINT('',#27229);
#7576=VERTEX_POINT('',#27231);
#7577=VERTEX_POINT('',#27233);
#7578=VERTEX_POINT('',#27235);
#7579=VERTEX_POINT('',#27240);
#7580=VERTEX_POINT('',#27244);
#7581=VERTEX_POINT('',#27248);
#7582=VERTEX_POINT('',#27250);
#7583=VERTEX_POINT('',#27254);
#7584=VERTEX_POINT('',#27255);
#7585=VERTEX_POINT('',#27257);
#7586=VERTEX_POINT('',#27259);
#7587=VERTEX_POINT('',#27261);
#7588=VERTEX_POINT('',#27266);
#7589=VERTEX_POINT('',#27270);
#7590=VERTEX_POINT('',#27274);
#7591=VERTEX_POINT('',#27276);
#7592=VERTEX_POINT('',#27280);
#7593=VERTEX_POINT('',#27281);
#7594=VERTEX_POINT('',#27283);
#7595=VERTEX_POINT('',#27285);
#7596=VERTEX_POINT('',#27287);
#7597=VERTEX_POINT('',#27292);
#7598=VERTEX_POINT('',#27296);
#7599=VERTEX_POINT('',#27303);
#7600=VERTEX_POINT('',#27304);
#7601=VERTEX_POINT('',#27309);
#7602=VERTEX_POINT('',#27311);
#7603=VERTEX_POINT('',#27318);
#7604=VERTEX_POINT('',#27416);
#7605=VERTEX_POINT('',#27692);
#7606=VERTEX_POINT('',#27697);
#7607=VERTEX_POINT('',#27702);
#7608=VERTEX_POINT('',#27753);
#7609=VERTEX_POINT('',#27760);
#7610=VERTEX_POINT('',#27812);
#7611=VERTEX_POINT('',#27813);
#7612=VERTEX_POINT('',#27818);
#7613=VERTEX_POINT('',#27820);
#7614=VERTEX_POINT('',#27827);
#7615=VERTEX_POINT('',#27919);
#7616=VERTEX_POINT('',#28175);
#7617=VERTEX_POINT('',#28180);
#7618=VERTEX_POINT('',#28189);
#7619=VERTEX_POINT('',#28196);
#7620=VERTEX_POINT('',#28248);
#7621=VERTEX_POINT('',#28249);
#7622=VERTEX_POINT('',#28254);
#7623=VERTEX_POINT('',#28256);
#7624=VERTEX_POINT('',#28263);
#7625=VERTEX_POINT('',#28361);
#7626=VERTEX_POINT('',#28647);
#7627=VERTEX_POINT('',#28652);
#7628=VERTEX_POINT('',#28661);
#7629=VERTEX_POINT('',#28668);
#7630=VERTEX_POINT('',#28720);
#7631=VERTEX_POINT('',#28721);
#7632=VERTEX_POINT('',#28726);
#7633=VERTEX_POINT('',#28728);
#7634=VERTEX_POINT('',#28735);
#7635=VERTEX_POINT('',#28833);
#7636=VERTEX_POINT('',#29109);
#7637=VERTEX_POINT('',#29114);
#7638=VERTEX_POINT('',#29123);
#7639=VERTEX_POINT('',#29130);
#7640=VERTEX_POINT('',#29182);
#7641=VERTEX_POINT('',#29183);
#7642=VERTEX_POINT('',#29188);
#7643=VERTEX_POINT('',#29190);
#7644=VERTEX_POINT('',#29197);
#7645=VERTEX_POINT('',#29289);
#7646=VERTEX_POINT('',#29545);
#7647=VERTEX_POINT('',#29550);
#7648=VERTEX_POINT('',#29559);
#7649=VERTEX_POINT('',#29566);
#7650=VERTEX_POINT('',#29618);
#7651=VERTEX_POINT('',#29619);
#7652=VERTEX_POINT('',#29624);
#7653=VERTEX_POINT('',#29626);
#7654=VERTEX_POINT('',#29633);
#7655=VERTEX_POINT('',#29731);
#7656=VERTEX_POINT('',#30017);
#7657=VERTEX_POINT('',#30022);
#7658=VERTEX_POINT('',#30031);
#7659=VERTEX_POINT('',#30038);
#7660=VERTEX_POINT('',#30090);
#7661=VERTEX_POINT('',#30091);
#7662=VERTEX_POINT('',#30096);
#7663=VERTEX_POINT('',#30098);
#7664=VERTEX_POINT('',#30105);
#7665=VERTEX_POINT('',#30203);
#7666=VERTEX_POINT('',#30479);
#7667=VERTEX_POINT('',#30484);
#7668=VERTEX_POINT('',#30493);
#7669=VERTEX_POINT('',#30500);
#7670=VERTEX_POINT('',#30552);
#7671=VERTEX_POINT('',#30553);
#7672=VERTEX_POINT('',#30558);
#7673=VERTEX_POINT('',#30560);
#7674=VERTEX_POINT('',#30567);
#7675=VERTEX_POINT('',#30659);
#7676=VERTEX_POINT('',#30915);
#7677=VERTEX_POINT('',#30920);
#7678=VERTEX_POINT('',#30929);
#7679=VERTEX_POINT('',#30936);
#7680=VERTEX_POINT('',#30988);
#7681=VERTEX_POINT('',#30989);
#7682=VERTEX_POINT('',#30994);
#7683=VERTEX_POINT('',#30996);
#7684=VERTEX_POINT('',#31003);
#7685=VERTEX_POINT('',#31101);
#7686=VERTEX_POINT('',#31387);
#7687=VERTEX_POINT('',#31392);
#7688=VERTEX_POINT('',#31401);
#7689=VERTEX_POINT('',#31408);
#7690=VERTEX_POINT('',#31460);
#7691=VERTEX_POINT('',#31461);
#7692=VERTEX_POINT('',#31466);
#7693=VERTEX_POINT('',#31468);
#7694=VERTEX_POINT('',#31475);
#7695=VERTEX_POINT('',#31573);
#7696=VERTEX_POINT('',#31849);
#7697=VERTEX_POINT('',#31854);
#7698=VERTEX_POINT('',#31863);
#7699=VERTEX_POINT('',#31870);
#7700=VERTEX_POINT('',#31922);
#7701=VERTEX_POINT('',#31923);
#7702=VERTEX_POINT('',#31928);
#7703=VERTEX_POINT('',#31930);
#7704=VERTEX_POINT('',#31937);
#7705=VERTEX_POINT('',#32029);
#7706=VERTEX_POINT('',#32285);
#7707=VERTEX_POINT('',#32290);
#7708=VERTEX_POINT('',#32299);
#7709=VERTEX_POINT('',#32306);
#7710=VERTEX_POINT('',#32358);
#7711=VERTEX_POINT('',#32359);
#7712=VERTEX_POINT('',#32364);
#7713=VERTEX_POINT('',#32366);
#7714=VERTEX_POINT('',#32373);
#7715=VERTEX_POINT('',#32471);
#7716=VERTEX_POINT('',#32757);
#7717=VERTEX_POINT('',#32762);
#7718=VERTEX_POINT('',#32771);
#7719=VERTEX_POINT('',#32778);
#7720=VERTEX_POINT('',#32830);
#7721=VERTEX_POINT('',#32832);
#7722=VERTEX_POINT('',#32836);
#7723=VERTEX_POINT('',#32839);
#7724=VERTEX_POINT('',#32843);
#7725=VERTEX_POINT('',#32845);
#7726=VERTEX_POINT('',#32849);
#7727=VERTEX_POINT('',#32852);
#7728=VERTEX_POINT('',#32856);
#7729=VERTEX_POINT('',#32857);
#7730=VERTEX_POINT('',#32861);
#7731=VERTEX_POINT('',#32863);
#7732=VERTEX_POINT('',#32867);
#7733=VERTEX_POINT('',#32873);
#7734=VERTEX_POINT('',#32878);
#7735=VERTEX_POINT('',#32880);
#7736=VERTEX_POINT('',#32885);
#7737=VERTEX_POINT('',#32891);
#7738=VERTEX_POINT('',#32893);
#7739=VERTEX_POINT('',#32897);
#7740=VERTEX_POINT('',#32905);
#7741=VERTEX_POINT('',#32907);
#7742=VERTEX_POINT('',#32912);
#7743=VERTEX_POINT('',#32916);
#7744=VERTEX_POINT('',#32920);
#7745=VERTEX_POINT('',#32926);
#7746=VERTEX_POINT('',#32928);
#7747=VERTEX_POINT('',#32932);
#7748=VERTEX_POINT('',#32939);
#7749=VERTEX_POINT('',#32940);
#7750=VERTEX_POINT('',#32944);
#7751=VERTEX_POINT('',#32951);
#7752=VERTEX_POINT('',#32953);
#7753=VERTEX_POINT('',#32957);
#7754=VERTEX_POINT('',#32965);
#7755=VERTEX_POINT('',#32967);
#7756=VERTEX_POINT('',#32972);
#7757=VERTEX_POINT('',#32976);
#7758=VERTEX_POINT('',#32980);
#7759=VERTEX_POINT('',#32986);
#7760=VERTEX_POINT('',#32988);
#7761=VERTEX_POINT('',#32992);
#7762=VERTEX_POINT('',#32999);
#7763=VERTEX_POINT('',#33000);
#7764=VERTEX_POINT('',#33004);
#7765=VERTEX_POINT('',#33011);
#7766=VERTEX_POINT('',#33013);
#7767=VERTEX_POINT('',#33017);
#7768=VERTEX_POINT('',#33025);
#7769=VERTEX_POINT('',#33027);
#7770=VERTEX_POINT('',#33032);
#7771=VERTEX_POINT('',#33036);
#7772=VERTEX_POINT('',#33040);
#7773=VERTEX_POINT('',#33046);
#7774=VERTEX_POINT('',#33048);
#7775=VERTEX_POINT('',#33052);
#7776=VERTEX_POINT('',#33059);
#7777=VERTEX_POINT('',#33060);
#7778=VERTEX_POINT('',#33064);
#7779=VERTEX_POINT('',#33071);
#7780=VERTEX_POINT('',#33073);
#7781=VERTEX_POINT('',#33077);
#7782=VERTEX_POINT('',#33085);
#7783=VERTEX_POINT('',#33087);
#7784=VERTEX_POINT('',#33092);
#7785=VERTEX_POINT('',#33096);
#7786=VERTEX_POINT('',#33100);
#7787=VERTEX_POINT('',#33106);
#7788=VERTEX_POINT('',#33108);
#7789=VERTEX_POINT('',#33112);
#7790=VERTEX_POINT('',#33119);
#7791=VERTEX_POINT('',#33120);
#7792=VERTEX_POINT('',#33124);
#7793=VERTEX_POINT('',#33131);
#7794=VERTEX_POINT('',#33133);
#7795=VERTEX_POINT('',#33137);
#7796=VERTEX_POINT('',#33145);
#7797=VERTEX_POINT('',#33147);
#7798=VERTEX_POINT('',#33152);
#7799=VERTEX_POINT('',#33156);
#7800=VERTEX_POINT('',#33160);
#7801=VERTEX_POINT('',#33166);
#7802=VERTEX_POINT('',#33168);
#7803=VERTEX_POINT('',#33172);
#7804=VERTEX_POINT('',#33179);
#7805=VERTEX_POINT('',#33181);
#7806=VERTEX_POINT('',#33183);
#7807=VERTEX_POINT('',#33185);
#7808=VERTEX_POINT('',#33187);
#7809=VERTEX_POINT('',#33189);
#7810=VERTEX_POINT('',#33191);
#7811=VERTEX_POINT('',#33193);
#7812=VERTEX_POINT('',#33195);
#7813=VERTEX_POINT('',#33197);
#7814=VERTEX_POINT('',#33199);
#7815=VERTEX_POINT('',#33201);
#7816=VERTEX_POINT('',#33204);
#7817=VERTEX_POINT('',#33207);
#7818=VERTEX_POINT('',#33211);
#7819=VERTEX_POINT('',#33213);
#7820=VERTEX_POINT('',#33222);
#7821=VERTEX_POINT('',#33224);
#7822=VERTEX_POINT('',#33244);
#7823=VERTEX_POINT('',#33260);
#7824=VERTEX_POINT('',#33264);
#7825=VERTEX_POINT('',#33271);
#7826=VERTEX_POINT('',#33273);
#7827=VERTEX_POINT('',#33278);
#7828=VERTEX_POINT('',#33282);
#7829=VERTEX_POINT('',#33286);
#7830=VERTEX_POINT('',#33292);
#7831=VERTEX_POINT('',#33294);
#7832=VERTEX_POINT('',#33303);
#7833=VERTEX_POINT('',#33307);
#7834=VERTEX_POINT('',#33309);
#7835=VERTEX_POINT('',#33318);
#7836=VERTEX_POINT('',#33320);
#7837=VERTEX_POINT('',#33327);
#7838=VERTEX_POINT('',#33329);
#7839=VERTEX_POINT('',#33334);
#7840=VERTEX_POINT('',#33338);
#7841=VERTEX_POINT('',#33342);
#7842=VERTEX_POINT('',#33348);
#7843=VERTEX_POINT('',#33350);
#7844=VERTEX_POINT('',#33359);
#7845=VERTEX_POINT('',#33363);
#7846=VERTEX_POINT('',#33365);
#7847=VERTEX_POINT('',#33374);
#7848=VERTEX_POINT('',#33376);
#7849=VERTEX_POINT('',#33383);
#7850=VERTEX_POINT('',#33385);
#7851=VERTEX_POINT('',#33390);
#7852=VERTEX_POINT('',#33394);
#7853=VERTEX_POINT('',#33398);
#7854=VERTEX_POINT('',#33404);
#7855=VERTEX_POINT('',#33406);
#7856=VERTEX_POINT('',#33415);
#7857=VERTEX_POINT('',#33419);
#7858=VERTEX_POINT('',#33421);
#7859=VERTEX_POINT('',#33430);
#7860=VERTEX_POINT('',#33432);
#7861=VERTEX_POINT('',#33439);
#7862=VERTEX_POINT('',#33441);
#7863=VERTEX_POINT('',#33446);
#7864=VERTEX_POINT('',#33450);
#7865=VERTEX_POINT('',#33454);
#7866=VERTEX_POINT('',#33460);
#7867=VERTEX_POINT('',#33462);
#7868=VERTEX_POINT('',#33471);
#7869=VERTEX_POINT('',#33475);
#7870=VERTEX_POINT('',#33477);
#7871=VERTEX_POINT('',#33486);
#7872=VERTEX_POINT('',#33488);
#7873=VERTEX_POINT('',#33495);
#7874=VERTEX_POINT('',#33497);
#7875=VERTEX_POINT('',#33502);
#7876=VERTEX_POINT('',#33506);
#7877=VERTEX_POINT('',#33510);
#7878=VERTEX_POINT('',#33516);
#7879=VERTEX_POINT('',#33518);
#7880=VERTEX_POINT('',#33527);
#7881=VERTEX_POINT('',#33531);
#7882=VERTEX_POINT('',#33533);
#7883=VERTEX_POINT('',#33542);
#7884=VERTEX_POINT('',#33544);
#7885=VERTEX_POINT('',#33550);
#7886=VERTEX_POINT('',#33552);
#7887=VERTEX_POINT('',#33555);
#7888=VERTEX_POINT('',#33557);
#7889=VERTEX_POINT('',#33564);
#7890=VERTEX_POINT('',#33574);
#7891=VERTEX_POINT('',#33576);
#7892=VERTEX_POINT('',#33581);
#7893=VERTEX_POINT('',#33585);
#7894=VERTEX_POINT('',#33589);
#7895=VERTEX_POINT('',#33595);
#7896=VERTEX_POINT('',#33601);
#7897=VERTEX_POINT('',#33607);
#7898=VERTEX_POINT('',#33616);
#7899=VERTEX_POINT('',#33623);
#7900=VERTEX_POINT('',#33628);
#7901=VERTEX_POINT('',#33635);
#7902=VERTEX_POINT('',#33730);
#7903=VERTEX_POINT('',#33732);
#7904=VERTEX_POINT('',#34278);
#7905=VERTEX_POINT('',#34383);
#7906=VERTEX_POINT('',#34386);
#7907=VERTEX_POINT('',#35215);
#7908=VERTEX_POINT('',#35490);
#7909=VERTEX_POINT('',#35492);
#7910=VERTEX_POINT('',#35497);
#7911=VERTEX_POINT('',#35500);
#7912=VERTEX_POINT('',#35506);
#7913=VERTEX_POINT('',#36015);
#7914=VERTEX_POINT('',#36534);
#7915=VERTEX_POINT('',#37033);
#7916=VERTEX_POINT('',#37542);
#7917=VERTEX_POINT('',#38061);
#7918=VERTEX_POINT('',#38560);
#7919=VERTEX_POINT('',#39069);
#7920=VERTEX_POINT('',#39588);
#7921=VERTEX_POINT('',#40097);
#7922=VERTEX_POINT('',#40606);
#7923=VERTEX_POINT('',#41125);
#7924=VERTEX_POINT('',#41653);
#7925=VERTEX_POINT('',#41661);
#7926=VERTEX_POINT('',#41665);
#7927=VERTEX_POINT('',#41668);
#7928=VERTEX_POINT('',#41672);
#7929=VERTEX_POINT('',#41676);
#7930=VERTEX_POINT('',#41680);
#7931=VERTEX_POINT('',#41684);
#7932=VERTEX_POINT('',#41687);
#7933=VERTEX_POINT('',#41691);
#7934=VERTEX_POINT('',#41695);
#7935=VERTEX_POINT('',#41699);
#7936=VERTEX_POINT('',#41703);
#7937=VERTEX_POINT('',#41711);
#9115=EDGE_CURVE('',#7324,#7325,#4500,.T.);
#9116=EDGE_CURVE('',#7324,#7326,#3705,.T.);
#9117=EDGE_CURVE('',#7326,#7327,#3300,.T.);
#9118=EDGE_CURVE('',#7327,#7325,#3706,.T.);
#9119=EDGE_CURVE('',#7328,#7329,#4501,.T.);
#9120=EDGE_CURVE('',#7328,#7324,#3707,.T.);
#9121=EDGE_CURVE('',#7325,#7329,#3708,.T.);
#9122=EDGE_CURVE('',#7330,#7331,#4502,.T.);
#9123=EDGE_CURVE('',#7330,#7328,#3709,.T.);
#9124=EDGE_CURVE('',#7329,#7331,#3710,.T.);
#9125=EDGE_CURVE('',#7332,#7333,#4503,.T.);
#9126=EDGE_CURVE('',#7332,#7330,#3711,.T.);
#9127=EDGE_CURVE('',#7331,#7333,#3712,.T.);
#9128=EDGE_CURVE('',#7334,#7335,#4504,.T.);
#9129=EDGE_CURVE('',#7334,#7332,#3713,.T.);
#9130=EDGE_CURVE('',#7333,#7335,#3714,.T.);
#9131=EDGE_CURVE('',#7336,#7337,#4505,.T.);
#9132=EDGE_CURVE('',#7336,#7334,#3715,.T.);
#9133=EDGE_CURVE('',#7335,#7337,#3716,.T.);
#9134=EDGE_CURVE('',#7338,#7339,#4506,.T.);
#9135=EDGE_CURVE('',#7338,#7336,#3717,.T.);
#9136=EDGE_CURVE('',#7337,#7339,#3718,.T.);
#9137=EDGE_CURVE('',#7340,#7341,#4507,.T.);
#9138=EDGE_CURVE('',#7340,#7338,#3719,.T.);
#9139=EDGE_CURVE('',#7339,#7341,#3720,.T.);
#9140=EDGE_CURVE('',#7342,#7343,#4508,.T.);
#9141=EDGE_CURVE('',#7342,#7340,#3721,.T.);
#9142=EDGE_CURVE('',#7341,#7343,#3722,.T.);
#9143=EDGE_CURVE('',#7344,#7345,#4509,.T.);
#9144=EDGE_CURVE('',#7344,#7342,#3723,.T.);
#9145=EDGE_CURVE('',#7343,#7345,#3724,.T.);
#9146=EDGE_CURVE('',#7346,#7347,#4510,.T.);
#9147=EDGE_CURVE('',#7346,#7344,#3725,.T.);
#9148=EDGE_CURVE('',#7345,#7347,#3726,.T.);
#9149=EDGE_CURVE('',#7348,#7349,#4511,.T.);
#9150=EDGE_CURVE('',#7348,#7346,#3727,.T.);
#9151=EDGE_CURVE('',#7347,#7349,#3728,.T.);
#9152=EDGE_CURVE('',#7350,#7351,#4512,.T.);
#9153=EDGE_CURVE('',#7350,#7348,#3729,.T.);
#9154=EDGE_CURVE('',#7349,#7351,#3730,.T.);
#9155=EDGE_CURVE('',#7352,#7353,#4513,.T.);
#9156=EDGE_CURVE('',#7352,#7350,#3731,.T.);
#9157=EDGE_CURVE('',#7351,#7353,#3732,.T.);
#9158=EDGE_CURVE('',#7354,#7355,#4514,.T.);
#9159=EDGE_CURVE('',#7354,#7352,#3733,.T.);
#9160=EDGE_CURVE('',#7353,#7355,#3734,.T.);
#9161=EDGE_CURVE('',#7356,#7357,#4515,.T.);
#9162=EDGE_CURVE('',#7356,#7354,#3735,.T.);
#9163=EDGE_CURVE('',#7355,#7357,#3736,.T.);
#9164=EDGE_CURVE('',#7358,#7359,#976,.T.);
#9165=EDGE_CURVE('',#7358,#7360,#3737,.T.);
#9166=EDGE_CURVE('',#7360,#7361,#3738,.T.);
#9167=EDGE_CURVE('',#7361,#7362,#3739,.T.);
#9168=EDGE_CURVE('',#7363,#7362,#977,.T.);
#9169=EDGE_CURVE('',#7363,#7363,#3301,.T.);
#9170=EDGE_CURVE('',#7362,#7364,#3740,.T.);
#9171=EDGE_CURVE('',#7365,#7364,#3302,.T.);
#9172=EDGE_CURVE('',#7365,#7366,#3741,.T.);
#9173=EDGE_CURVE('',#7366,#7367,#3742,.T.);
#9174=EDGE_CURVE('',#7367,#7368,#3743,.T.);
#9175=EDGE_CURVE('',#7369,#7368,#3303,.T.);
#9176=EDGE_CURVE('',#7369,#7370,#3744,.T.);
#9177=EDGE_CURVE('',#7370,#7371,#3745,.T.);
#9178=EDGE_CURVE('',#7371,#7372,#3746,.T.);
#9179=EDGE_CURVE('',#7373,#7372,#3304,.T.);
#9180=EDGE_CURVE('',#7373,#7374,#3747,.T.);
#9181=EDGE_CURVE('',#7374,#7375,#3748,.T.);
#9182=EDGE_CURVE('',#7375,#7376,#3749,.T.);
#9183=EDGE_CURVE('',#7377,#7376,#3305,.T.);
#9184=EDGE_CURVE('',#7377,#7378,#3750,.T.);
#9185=EDGE_CURVE('',#7378,#7379,#3751,.T.);
#9186=EDGE_CURVE('',#7379,#7380,#3752,.T.);
#9187=EDGE_CURVE('',#7381,#7380,#3306,.T.);
#9188=EDGE_CURVE('',#7381,#7382,#3753,.T.);
#9189=EDGE_CURVE('',#7382,#7383,#3754,.T.);
#9190=EDGE_CURVE('',#7383,#7384,#3755,.T.);
#9191=EDGE_CURVE('',#7385,#7384,#3307,.T.);
#9192=EDGE_CURVE('',#7385,#7386,#3756,.T.);
#9193=EDGE_CURVE('',#7386,#7387,#3757,.T.);
#9194=EDGE_CURVE('',#7387,#7388,#3758,.T.);
#9195=EDGE_CURVE('',#7389,#7388,#3308,.T.);
#9196=EDGE_CURVE('',#7389,#7390,#3759,.T.);
#9197=EDGE_CURVE('',#7390,#7391,#3760,.T.);
#9198=EDGE_CURVE('',#7391,#7392,#3761,.T.);
#9199=EDGE_CURVE('',#7393,#7392,#3309,.T.);
#9200=EDGE_CURVE('',#7393,#7394,#3762,.T.);
#9201=EDGE_CURVE('',#7394,#7395,#3763,.T.);
#9202=EDGE_CURVE('',#7395,#7396,#3764,.T.);
#9203=EDGE_CURVE('',#7397,#7396,#3310,.T.);
#9204=EDGE_CURVE('',#7397,#7398,#3765,.T.);
#9205=EDGE_CURVE('',#7398,#7399,#3766,.T.);
#9206=EDGE_CURVE('',#7399,#7400,#3767,.T.);
#9207=EDGE_CURVE('',#7401,#7400,#3311,.T.);
#9208=EDGE_CURVE('',#7401,#7402,#3768,.T.);
#9209=EDGE_CURVE('',#7402,#7403,#3769,.T.);
#9210=EDGE_CURVE('',#7403,#7404,#3770,.T.);
#9211=EDGE_CURVE('',#7405,#7404,#3312,.T.);
#9212=EDGE_CURVE('',#7405,#7406,#3771,.T.);
#9213=EDGE_CURVE('',#7406,#7407,#3772,.T.);
#9214=EDGE_CURVE('',#7407,#7408,#3773,.T.);
#9215=EDGE_CURVE('',#7409,#7408,#3313,.T.);
#9216=EDGE_CURVE('',#7409,#7410,#3774,.T.);
#9217=EDGE_CURVE('',#7410,#7411,#3775,.T.);
#9218=EDGE_CURVE('',#7411,#7412,#3776,.T.);
#9219=EDGE_CURVE('',#7413,#7412,#3314,.T.);
#9220=EDGE_CURVE('',#7413,#7414,#3777,.T.);
#9221=EDGE_CURVE('',#7414,#7415,#3778,.T.);
#9222=EDGE_CURVE('',#7415,#7416,#3779,.T.);
#9223=EDGE_CURVE('',#7417,#7416,#3315,.T.);
#9224=EDGE_CURVE('',#7417,#7418,#3780,.T.);
#9225=EDGE_CURVE('',#7418,#7419,#3781,.T.);
#9226=EDGE_CURVE('',#7419,#7420,#3782,.T.);
#9227=EDGE_CURVE('',#7421,#7420,#3316,.T.);
#9228=EDGE_CURVE('',#7421,#7422,#3783,.T.);
#9229=EDGE_CURVE('',#7422,#7423,#3784,.T.);
#9230=EDGE_CURVE('',#7423,#7424,#3785,.T.);
#9231=EDGE_CURVE('',#7425,#7424,#3317,.T.);
#9232=EDGE_CURVE('',#7425,#7426,#3786,.T.);
#9233=EDGE_CURVE('',#7426,#7427,#3787,.T.);
#9234=EDGE_CURVE('',#7427,#7428,#3788,.T.);
#9235=EDGE_CURVE('',#7429,#7428,#3318,.T.);
#9236=EDGE_CURVE('',#7429,#7430,#3789,.T.);
#9237=EDGE_CURVE('',#7430,#7431,#3790,.T.);
#9238=EDGE_CURVE('',#7431,#7432,#3791,.T.);
#9239=EDGE_CURVE('',#7433,#7432,#3319,.T.);
#9240=EDGE_CURVE('',#7433,#7434,#3792,.T.);
#9241=EDGE_CURVE('',#7434,#7435,#3793,.T.);
#9242=EDGE_CURVE('',#7435,#7436,#3794,.T.);
#9243=EDGE_CURVE('',#7437,#7436,#3320,.T.);
#9244=EDGE_CURVE('',#7437,#7438,#3795,.T.);
#9245=EDGE_CURVE('',#7438,#7439,#3796,.T.);
#9246=EDGE_CURVE('',#7439,#7440,#3797,.T.);
#9247=EDGE_CURVE('',#7441,#7440,#3321,.T.);
#9248=EDGE_CURVE('',#7441,#7442,#3798,.T.);
#9249=EDGE_CURVE('',#7442,#7443,#3799,.T.);
#9250=EDGE_CURVE('',#7443,#7444,#3800,.T.);
#9251=EDGE_CURVE('',#7445,#7444,#3322,.T.);
#9252=EDGE_CURVE('',#7445,#7446,#3801,.T.);
#9253=EDGE_CURVE('',#7446,#7447,#3802,.T.);
#9254=EDGE_CURVE('',#7447,#7448,#3803,.T.);
#9255=EDGE_CURVE('',#7449,#7448,#3323,.T.);
#9256=EDGE_CURVE('',#7449,#7450,#3804,.T.);
#9257=EDGE_CURVE('',#7450,#7451,#3805,.T.);
#9258=EDGE_CURVE('',#7451,#7359,#3806,.T.);
#9259=EDGE_CURVE('',#7452,#7453,#4516,.T.);
#9260=EDGE_CURVE('',#7452,#7454,#3807,.T.);
#9261=EDGE_CURVE('',#7455,#7454,#3324,.T.);
#9262=EDGE_CURVE('',#7453,#7455,#3808,.T.);
#9263=EDGE_CURVE('',#7456,#7457,#4517,.T.);
#9264=EDGE_CURVE('',#7456,#7452,#3809,.T.);
#9265=EDGE_CURVE('',#7457,#7453,#3810,.T.);
#9266=EDGE_CURVE('',#7458,#7459,#4518,.T.);
#9267=EDGE_CURVE('',#7458,#7456,#3811,.T.);
#9268=EDGE_CURVE('',#7459,#7457,#3812,.T.);
#9269=EDGE_CURVE('',#7460,#7461,#4519,.T.);
#9270=EDGE_CURVE('',#7460,#7458,#3813,.T.);
#9271=EDGE_CURVE('',#7461,#7459,#3814,.T.);
#9272=EDGE_CURVE('',#7462,#7463,#4520,.T.);
#9273=EDGE_CURVE('',#7462,#7460,#3815,.T.);
#9274=EDGE_CURVE('',#7463,#7461,#3816,.T.);
#9275=EDGE_CURVE('',#7464,#7465,#4521,.T.);
#9276=EDGE_CURVE('',#7464,#7462,#3817,.T.);
#9277=EDGE_CURVE('',#7465,#7463,#3818,.T.);
#9278=EDGE_CURVE('',#7466,#7467,#4522,.T.);
#9279=EDGE_CURVE('',#7466,#7464,#3819,.T.);
#9280=EDGE_CURVE('',#7467,#7465,#3820,.T.);
#9281=EDGE_CURVE('',#7468,#7469,#4523,.T.);
#9282=EDGE_CURVE('',#7468,#7466,#3821,.T.);
#9283=EDGE_CURVE('',#7469,#7467,#3822,.T.);
#9284=EDGE_CURVE('',#7470,#7471,#4524,.T.);
#9285=EDGE_CURVE('',#7470,#7468,#3823,.T.);
#9286=EDGE_CURVE('',#7471,#7469,#3824,.T.);
#9287=EDGE_CURVE('',#7472,#7473,#4525,.T.);
#9288=EDGE_CURVE('',#7472,#7470,#3825,.T.);
#9289=EDGE_CURVE('',#7473,#7471,#3826,.T.);
#9290=EDGE_CURVE('',#7474,#7475,#4526,.T.);
#9291=EDGE_CURVE('',#7474,#7472,#3827,.T.);
#9292=EDGE_CURVE('',#7475,#7473,#3828,.T.);
#9293=EDGE_CURVE('',#7476,#7477,#4527,.T.);
#9294=EDGE_CURVE('',#7476,#7474,#3829,.T.);
#9295=EDGE_CURVE('',#7477,#7475,#3830,.T.);
#9296=EDGE_CURVE('',#7478,#7479,#4528,.T.);
#9297=EDGE_CURVE('',#7478,#7476,#3831,.T.);
#9298=EDGE_CURVE('',#7479,#7477,#3832,.T.);
#9299=EDGE_CURVE('',#7480,#7481,#4529,.T.);
#9300=EDGE_CURVE('',#7480,#7478,#3833,.T.);
#9301=EDGE_CURVE('',#7481,#7479,#3834,.T.);
#9302=EDGE_CURVE('',#7482,#7483,#4530,.T.);
#9303=EDGE_CURVE('',#7482,#7480,#3835,.T.);
#9304=EDGE_CURVE('',#7483,#7481,#3836,.T.);
#9305=EDGE_CURVE('',#7484,#7485,#4531,.T.);
#9306=EDGE_CURVE('',#7484,#7482,#3837,.T.);
#9307=EDGE_CURVE('',#7485,#7483,#3838,.T.);
#9308=EDGE_CURVE('',#7486,#7486,#3325,.T.);
#9309=EDGE_CURVE('',#7486,#7487,#4532,.T.);
#9310=EDGE_CURVE('',#7487,#7488,#3326,.T.);
#9311=EDGE_CURVE('',#7488,#7487,#3327,.T.);
#9312=EDGE_CURVE('',#7488,#7489,#4533,.T.);
#9313=EDGE_CURVE('',#7489,#7489,#3328,.T.);
#9314=EDGE_CURVE('',#7490,#7490,#3329,.T.);
#9315=EDGE_CURVE('',#7491,#7492,#4534,.T.);
#9316=EDGE_CURVE('',#7492,#7493,#4535,.T.);
#9317=EDGE_CURVE('',#7493,#7494,#4536,.F.);
#9318=EDGE_CURVE('',#7494,#7495,#4537,.T.);
#9319=EDGE_CURVE('',#7495,#7491,#4538,.T.);
#9320=EDGE_CURVE('',#7496,#7492,#4539,.T.);
#9321=EDGE_CURVE('',#7496,#7497,#4540,.T.);
#9322=EDGE_CURVE('',#7493,#7497,#4541,.T.);
#9323=EDGE_CURVE('',#7498,#7491,#4542,.T.);
#9324=EDGE_CURVE('',#7498,#7499,#4543,.T.);
#9325=EDGE_CURVE('',#7499,#7496,#4544,.T.);
#9326=EDGE_CURVE('',#7495,#7500,#4545,.T.);
#9327=EDGE_CURVE('',#7501,#7500,#4546,.T.);
#9328=EDGE_CURVE('',#7501,#7498,#4547,.T.);
#9329=EDGE_CURVE('',#7502,#7503,#4548,.T.);
#9330=EDGE_CURVE('',#7503,#7504,#4549,.T.);
#9331=EDGE_CURVE('',#7504,#7505,#4550,.F.);
#9332=EDGE_CURVE('',#7505,#7506,#4551,.T.);
#9333=EDGE_CURVE('',#7506,#7502,#4552,.T.);
#9334=EDGE_CURVE('',#7507,#7503,#4553,.T.);
#9335=EDGE_CURVE('',#7507,#7508,#4554,.T.);
#9336=EDGE_CURVE('',#7504,#7508,#4555,.T.);
#9337=EDGE_CURVE('',#7509,#7502,#4556,.T.);
#9338=EDGE_CURVE('',#7509,#7510,#4557,.T.);
#9339=EDGE_CURVE('',#7510,#7507,#4558,.T.);
#9340=EDGE_CURVE('',#7506,#7496,#4559,.T.);
#9341=EDGE_CURVE('',#7499,#7509,#4560,.T.);
#9342=EDGE_CURVE('',#7511,#7512,#4561,.T.);
#9343=EDGE_CURVE('',#7512,#7513,#4562,.T.);
#9344=EDGE_CURVE('',#7513,#7514,#4563,.F.);
#9345=EDGE_CURVE('',#7514,#7515,#4564,.T.);
#9346=EDGE_CURVE('',#7515,#7511,#4565,.T.);
#9347=EDGE_CURVE('',#7516,#7512,#4566,.T.);
#9348=EDGE_CURVE('',#7516,#7517,#4567,.T.);
#9349=EDGE_CURVE('',#7513,#7517,#4568,.T.);
#9350=EDGE_CURVE('',#7518,#7511,#4569,.T.);
#9351=EDGE_CURVE('',#7518,#7519,#4570,.T.);
#9352=EDGE_CURVE('',#7519,#7516,#4571,.T.);
#9353=EDGE_CURVE('',#7515,#7507,#4572,.T.);
#9354=EDGE_CURVE('',#7510,#7518,#4573,.T.);
#9355=EDGE_CURVE('',#7520,#7521,#4574,.T.);
#9356=EDGE_CURVE('',#7521,#7522,#4575,.T.);
#9357=EDGE_CURVE('',#7522,#7523,#4576,.F.);
#9358=EDGE_CURVE('',#7523,#7524,#4577,.T.);
#9359=EDGE_CURVE('',#7524,#7520,#4578,.T.);
#9360=EDGE_CURVE('',#7525,#7521,#4579,.T.);
#9361=EDGE_CURVE('',#7525,#7526,#4580,.T.);
#9362=EDGE_CURVE('',#7522,#7526,#4581,.T.);
#9363=EDGE_CURVE('',#7527,#7520,#4582,.T.);
#9364=EDGE_CURVE('',#7527,#7528,#4583,.T.);
#9365=EDGE_CURVE('',#7528,#7525,#4584,.T.);
#9366=EDGE_CURVE('',#7524,#7516,#4585,.T.);
#9367=EDGE_CURVE('',#7519,#7527,#4586,.T.);
#9368=EDGE_CURVE('',#7529,#7530,#4587,.T.);
#9369=EDGE_CURVE('',#7530,#7531,#4588,.T.);
#9370=EDGE_CURVE('',#7531,#7532,#4589,.F.);
#9371=EDGE_CURVE('',#7532,#7533,#4590,.T.);
#9372=EDGE_CURVE('',#7533,#7529,#4591,.T.);
#9373=EDGE_CURVE('',#7534,#7530,#4592,.T.);
#9374=EDGE_CURVE('',#7534,#7535,#4593,.T.);
#9375=EDGE_CURVE('',#7531,#7535,#4594,.T.);
#9376=EDGE_CURVE('',#7536,#7529,#4595,.T.);
#9377=EDGE_CURVE('',#7536,#7537,#4596,.T.);
#9378=EDGE_CURVE('',#7537,#7534,#4597,.T.);
#9379=EDGE_CURVE('',#7533,#7525,#4598,.T.);
#9380=EDGE_CURVE('',#7528,#7536,#4599,.T.);
#9381=EDGE_CURVE('',#7538,#7539,#4600,.T.);
#9382=EDGE_CURVE('',#7539,#7540,#4601,.T.);
#9383=EDGE_CURVE('',#7540,#7541,#4602,.F.);
#9384=EDGE_CURVE('',#7541,#7542,#4603,.T.);
#9385=EDGE_CURVE('',#7542,#7538,#4604,.T.);
#9386=EDGE_CURVE('',#7500,#7539,#4605,.T.);
#9387=EDGE_CURVE('',#7500,#7543,#4606,.T.);
#9388=EDGE_CURVE('',#7540,#7543,#4607,.T.);
#9389=EDGE_CURVE('',#7544,#7538,#4608,.T.);
#9390=EDGE_CURVE('',#7544,#7501,#4609,.T.);
#9391=EDGE_CURVE('',#7542,#7545,#4610,.T.);
#9392=EDGE_CURVE('',#7545,#7546,#4611,.T.);
#9393=EDGE_CURVE('',#7546,#7544,#4612,.T.);
#9394=EDGE_CURVE('',#7547,#7548,#4613,.T.);
#9395=EDGE_CURVE('',#7548,#7549,#4614,.T.);
#9396=EDGE_CURVE('',#7549,#7550,#4615,.F.);
#9397=EDGE_CURVE('',#7550,#7551,#4616,.T.);
#9398=EDGE_CURVE('',#7551,#7547,#4617,.T.);
#9399=EDGE_CURVE('',#7545,#7548,#4618,.T.);
#9400=EDGE_CURVE('',#7545,#7552,#4619,.T.);
#9401=EDGE_CURVE('',#7549,#7552,#4620,.T.);
#9402=EDGE_CURVE('',#7553,#7547,#4621,.T.);
#9403=EDGE_CURVE('',#7553,#7546,#4622,.T.);
#9404=EDGE_CURVE('',#7554,#7555,#4623,.T.);
#9405=EDGE_CURVE('',#7555,#7556,#4624,.T.);
#9406=EDGE_CURVE('',#7556,#7557,#4625,.F.);
#9407=EDGE_CURVE('',#7557,#7558,#4626,.T.);
#9408=EDGE_CURVE('',#7558,#7554,#4627,.T.);
#9409=EDGE_CURVE('',#7559,#7555,#4628,.T.);
#9410=EDGE_CURVE('',#7559,#7560,#4629,.T.);
#9411=EDGE_CURVE('',#7556,#7560,#4630,.T.);
#9412=EDGE_CURVE('',#7561,#7554,#4631,.T.);
#9413=EDGE_CURVE('',#7561,#7562,#4632,.T.);
#9414=EDGE_CURVE('',#7562,#7559,#4633,.T.);
#9415=EDGE_CURVE('',#7558,#7563,#4634,.T.);
#9416=EDGE_CURVE('',#7564,#7563,#4635,.T.);
#9417=EDGE_CURVE('',#7564,#7561,#4636,.T.);
#9418=EDGE_CURVE('',#7565,#7566,#4637,.T.);
#9419=EDGE_CURVE('',#7566,#7567,#4638,.T.);
#9420=EDGE_CURVE('',#7567,#7568,#4639,.F.);
#9421=EDGE_CURVE('',#7568,#7569,#4640,.T.);
#9422=EDGE_CURVE('',#7569,#7565,#4641,.T.);
#9423=EDGE_CURVE('',#7563,#7566,#4642,.T.);
#9424=EDGE_CURVE('',#7563,#7570,#4643,.T.);
#9425=EDGE_CURVE('',#7567,#7570,#4644,.T.);
#9426=EDGE_CURVE('',#7571,#7565,#4645,.T.);
#9427=EDGE_CURVE('',#7571,#7564,#4646,.T.);
#9428=EDGE_CURVE('',#7569,#7572,#4647,.T.);
#9429=EDGE_CURVE('',#7573,#7572,#4648,.T.);
#9430=EDGE_CURVE('',#7573,#7571,#4649,.T.);
#9431=EDGE_CURVE('',#7574,#7575,#4650,.T.);
#9432=EDGE_CURVE('',#7575,#7576,#4651,.T.);
#9433=EDGE_CURVE('',#7576,#7577,#4652,.F.);
#9434=EDGE_CURVE('',#7577,#7578,#4653,.T.);
#9435=EDGE_CURVE('',#7578,#7574,#4654,.T.);
#9436=EDGE_CURVE('',#7572,#7575,#4655,.T.);
#9437=EDGE_CURVE('',#7572,#7579,#4656,.T.);
#9438=EDGE_CURVE('',#7576,#7579,#4657,.T.);
#9439=EDGE_CURVE('',#7580,#7574,#4658,.T.);
#9440=EDGE_CURVE('',#7580,#7573,#4659,.T.);
#9441=EDGE_CURVE('',#7578,#7581,#4660,.T.);
#9442=EDGE_CURVE('',#7582,#7581,#4661,.T.);
#9443=EDGE_CURVE('',#7582,#7580,#4662,.T.);
#9444=EDGE_CURVE('',#7583,#7584,#4663,.T.);
#9445=EDGE_CURVE('',#7584,#7585,#4664,.T.);
#9446=EDGE_CURVE('',#7585,#7586,#4665,.F.);
#9447=EDGE_CURVE('',#7586,#7587,#4666,.T.);
#9448=EDGE_CURVE('',#7587,#7583,#4667,.T.);
#9449=EDGE_CURVE('',#7581,#7584,#4668,.T.);
#9450=EDGE_CURVE('',#7581,#7588,#4669,.T.);
#9451=EDGE_CURVE('',#7585,#7588,#4670,.T.);
#9452=EDGE_CURVE('',#7589,#7583,#4671,.T.);
#9453=EDGE_CURVE('',#7589,#7582,#4672,.T.);
#9454=EDGE_CURVE('',#7587,#7590,#4673,.T.);
#9455=EDGE_CURVE('',#7591,#7590,#4674,.T.);
#9456=EDGE_CURVE('',#7591,#7589,#4675,.T.);
#9457=EDGE_CURVE('',#7592,#7593,#4676,.T.);
#9458=EDGE_CURVE('',#7593,#7594,#4677,.T.);
#9459=EDGE_CURVE('',#7594,#7595,#4678,.F.);
#9460=EDGE_CURVE('',#7595,#7596,#4679,.T.);
#9461=EDGE_CURVE('',#7596,#7592,#4680,.T.);
#9462=EDGE_CURVE('',#7590,#7593,#4681,.T.);
#9463=EDGE_CURVE('',#7590,#7597,#4682,.T.);
#9464=EDGE_CURVE('',#7594,#7597,#4683,.T.);
#9465=EDGE_CURVE('',#7598,#7592,#4684,.T.);
#9466=EDGE_CURVE('',#7598,#7591,#4685,.T.);
#9467=EDGE_CURVE('',#7596,#7534,#4686,.T.);
#9468=EDGE_CURVE('',#7537,#7598,#4687,.T.);
#9469=EDGE_CURVE('',#7599,#7600,#3839,.T.);
#9470=EDGE_CURVE('',#7600,#7601,#3330,.T.);
#9471=EDGE_CURVE('',#7601,#7602,#3840,.T.);
#9472=EDGE_CURVE('',#7602,#7599,#3331,.T.);
#9473=EDGE_CURVE('',#7602,#7603,#3841,.T.);
#9474=EDGE_CURVE('',#7603,#7604,#3332,.T.);
#9475=EDGE_CURVE('',#7604,#7599,#3842,.T.);
#9476=EDGE_CURVE('',#7605,#7601,#3843,.T.);
#9477=EDGE_CURVE('',#7606,#7605,#3844,.T.);
#9478=EDGE_CURVE('',#7607,#7606,#3845,.T.);
#9479=EDGE_CURVE('',#7359,#7607,#3846,.T.);
#9480=EDGE_CURVE('',#7608,#7451,#3847,.T.);
#9481=EDGE_CURVE('',#7609,#7608,#3848,.T.);
#9482=EDGE_CURVE('',#7603,#7609,#3849,.T.);
#9483=EDGE_CURVE('',#7610,#7611,#3850,.T.);
#9484=EDGE_CURVE('',#7611,#7612,#3333,.T.);
#9485=EDGE_CURVE('',#7612,#7613,#3851,.T.);
#9486=EDGE_CURVE('',#7613,#7610,#3334,.T.);
#9487=EDGE_CURVE('',#7613,#7614,#3852,.T.);
#9488=EDGE_CURVE('',#7614,#7615,#3335,.T.);
#9489=EDGE_CURVE('',#7615,#7610,#3853,.T.);
#9490=EDGE_CURVE('',#7616,#7612,#3854,.T.);
#9491=EDGE_CURVE('',#7617,#7616,#3855,.T.);
#9492=EDGE_CURVE('',#7444,#7617,#3856,.T.);
#9493=EDGE_CURVE('',#7618,#7443,#3857,.T.);
#9494=EDGE_CURVE('',#7619,#7618,#3858,.T.);
#9495=EDGE_CURVE('',#7614,#7619,#3859,.T.);
#9496=EDGE_CURVE('',#7620,#7621,#3860,.T.);
#9497=EDGE_CURVE('',#7621,#7622,#3336,.T.);
#9498=EDGE_CURVE('',#7622,#7623,#3861,.T.);
#9499=EDGE_CURVE('',#7623,#7620,#3337,.T.);
#9500=EDGE_CURVE('',#7623,#7624,#3862,.T.);
#9501=EDGE_CURVE('',#7624,#7625,#3338,.T.);
#9502=EDGE_CURVE('',#7625,#7620,#3863,.T.);
#9503=EDGE_CURVE('',#7626,#7622,#3864,.T.);
#9504=EDGE_CURVE('',#7627,#7626,#3865,.T.);
#9505=EDGE_CURVE('',#7436,#7627,#3866,.T.);
#9506=EDGE_CURVE('',#7628,#7435,#3867,.T.);
#9507=EDGE_CURVE('',#7629,#7628,#3868,.T.);
#9508=EDGE_CURVE('',#7624,#7629,#3869,.T.);
#9509=EDGE_CURVE('',#7630,#7631,#3870,.T.);
#9510=EDGE_CURVE('',#7631,#7632,#3339,.T.);
#9511=EDGE_CURVE('',#7632,#7633,#3871,.T.);
#9512=EDGE_CURVE('',#7633,#7630,#3340,.T.);
#9513=EDGE_CURVE('',#7633,#7634,#3872,.T.);
#9514=EDGE_CURVE('',#7634,#7635,#3341,.T.);
#9515=EDGE_CURVE('',#7635,#7630,#3873,.T.);
#9516=EDGE_CURVE('',#7636,#7632,#3874,.T.);
#9517=EDGE_CURVE('',#7637,#7636,#3875,.T.);
#9518=EDGE_CURVE('',#7428,#7637,#3876,.T.);
#9519=EDGE_CURVE('',#7638,#7427,#3877,.T.);
#9520=EDGE_CURVE('',#7639,#7638,#3878,.T.);
#9521=EDGE_CURVE('',#7634,#7639,#3879,.T.);
#9522=EDGE_CURVE('',#7640,#7641,#3880,.T.);
#9523=EDGE_CURVE('',#7641,#7642,#3342,.T.);
#9524=EDGE_CURVE('',#7642,#7643,#3881,.T.);
#9525=EDGE_CURVE('',#7643,#7640,#3343,.T.);
#9526=EDGE_CURVE('',#7643,#7644,#3882,.T.);
#9527=EDGE_CURVE('',#7644,#7645,#3344,.T.);
#9528=EDGE_CURVE('',#7645,#7640,#3883,.T.);
#9529=EDGE_CURVE('',#7646,#7642,#3884,.T.);
#9530=EDGE_CURVE('',#7647,#7646,#3885,.T.);
#9531=EDGE_CURVE('',#7420,#7647,#3886,.T.);
#9532=EDGE_CURVE('',#7648,#7419,#3887,.T.);
#9533=EDGE_CURVE('',#7649,#7648,#3888,.T.);
#9534=EDGE_CURVE('',#7644,#7649,#3889,.T.);
#9535=EDGE_CURVE('',#7650,#7651,#3890,.T.);
#9536=EDGE_CURVE('',#7651,#7652,#3345,.T.);
#9537=EDGE_CURVE('',#7652,#7653,#3891,.T.);
#9538=EDGE_CURVE('',#7653,#7650,#3346,.T.);
#9539=EDGE_CURVE('',#7653,#7654,#3892,.T.);
#9540=EDGE_CURVE('',#7654,#7655,#3347,.T.);
#9541=EDGE_CURVE('',#7655,#7650,#3893,.T.);
#9542=EDGE_CURVE('',#7656,#7652,#3894,.T.);
#9543=EDGE_CURVE('',#7657,#7656,#3895,.T.);
#9544=EDGE_CURVE('',#7412,#7657,#3896,.T.);
#9545=EDGE_CURVE('',#7658,#7411,#3897,.T.);
#9546=EDGE_CURVE('',#7659,#7658,#3898,.T.);
#9547=EDGE_CURVE('',#7654,#7659,#3899,.T.);
#9548=EDGE_CURVE('',#7660,#7661,#3900,.T.);
#9549=EDGE_CURVE('',#7661,#7662,#3348,.T.);
#9550=EDGE_CURVE('',#7662,#7663,#3901,.T.);
#9551=EDGE_CURVE('',#7663,#7660,#3349,.T.);
#9552=EDGE_CURVE('',#7663,#7664,#3902,.T.);
#9553=EDGE_CURVE('',#7664,#7665,#3350,.T.);
#9554=EDGE_CURVE('',#7665,#7660,#3903,.T.);
#9555=EDGE_CURVE('',#7666,#7662,#3904,.T.);
#9556=EDGE_CURVE('',#7667,#7666,#3905,.T.);
#9557=EDGE_CURVE('',#7404,#7667,#3906,.T.);
#9558=EDGE_CURVE('',#7668,#7403,#3907,.T.);
#9559=EDGE_CURVE('',#7669,#7668,#3908,.T.);
#9560=EDGE_CURVE('',#7664,#7669,#3909,.T.);
#9561=EDGE_CURVE('',#7670,#7671,#3910,.T.);
#9562=EDGE_CURVE('',#7671,#7672,#3351,.T.);
#9563=EDGE_CURVE('',#7672,#7673,#3911,.T.);
#9564=EDGE_CURVE('',#7673,#7670,#3352,.T.);
#9565=EDGE_CURVE('',#7673,#7674,#3912,.T.);
#9566=EDGE_CURVE('',#7674,#7675,#3353,.T.);
#9567=EDGE_CURVE('',#7675,#7670,#3913,.T.);
#9568=EDGE_CURVE('',#7676,#7672,#3914,.T.);
#9569=EDGE_CURVE('',#7677,#7676,#3915,.T.);
#9570=EDGE_CURVE('',#7396,#7677,#3916,.T.);
#9571=EDGE_CURVE('',#7678,#7395,#3917,.T.);
#9572=EDGE_CURVE('',#7679,#7678,#3918,.T.);
#9573=EDGE_CURVE('',#7674,#7679,#3919,.T.);
#9574=EDGE_CURVE('',#7680,#7681,#3920,.T.);
#9575=EDGE_CURVE('',#7681,#7682,#3354,.T.);
#9576=EDGE_CURVE('',#7682,#7683,#3921,.T.);
#9577=EDGE_CURVE('',#7683,#7680,#3355,.T.);
#9578=EDGE_CURVE('',#7683,#7684,#3922,.T.);
#9579=EDGE_CURVE('',#7684,#7685,#3356,.T.);
#9580=EDGE_CURVE('',#7685,#7680,#3923,.T.);
#9581=EDGE_CURVE('',#7686,#7682,#3924,.T.);
#9582=EDGE_CURVE('',#7687,#7686,#3925,.T.);
#9583=EDGE_CURVE('',#7388,#7687,#3926,.T.);
#9584=EDGE_CURVE('',#7688,#7387,#3927,.T.);
#9585=EDGE_CURVE('',#7689,#7688,#3928,.T.);
#9586=EDGE_CURVE('',#7684,#7689,#3929,.T.);
#9587=EDGE_CURVE('',#7690,#7691,#3930,.T.);
#9588=EDGE_CURVE('',#7691,#7692,#3357,.T.);
#9589=EDGE_CURVE('',#7692,#7693,#3931,.T.);
#9590=EDGE_CURVE('',#7693,#7690,#3358,.T.);
#9591=EDGE_CURVE('',#7693,#7694,#3932,.T.);
#9592=EDGE_CURVE('',#7694,#7695,#3359,.T.);
#9593=EDGE_CURVE('',#7695,#7690,#3933,.T.);
#9594=EDGE_CURVE('',#7696,#7692,#3934,.T.);
#9595=EDGE_CURVE('',#7697,#7696,#3935,.T.);
#9596=EDGE_CURVE('',#7380,#7697,#3936,.T.);
#9597=EDGE_CURVE('',#7698,#7379,#3937,.T.);
#9598=EDGE_CURVE('',#7699,#7698,#3938,.T.);
#9599=EDGE_CURVE('',#7694,#7699,#3939,.T.);
#9600=EDGE_CURVE('',#7700,#7701,#3940,.T.);
#9601=EDGE_CURVE('',#7701,#7702,#3360,.T.);
#9602=EDGE_CURVE('',#7702,#7703,#3941,.T.);
#9603=EDGE_CURVE('',#7703,#7700,#3361,.T.);
#9604=EDGE_CURVE('',#7703,#7704,#3942,.T.);
#9605=EDGE_CURVE('',#7704,#7705,#3362,.T.);
#9606=EDGE_CURVE('',#7705,#7700,#3943,.T.);
#9607=EDGE_CURVE('',#7706,#7702,#3944,.T.);
#9608=EDGE_CURVE('',#7707,#7706,#3945,.T.);
#9609=EDGE_CURVE('',#7372,#7707,#3946,.T.);
#9610=EDGE_CURVE('',#7708,#7371,#3947,.T.);
#9611=EDGE_CURVE('',#7709,#7708,#3948,.T.);
#9612=EDGE_CURVE('',#7704,#7709,#3949,.T.);
#9613=EDGE_CURVE('',#7710,#7711,#3950,.T.);
#9614=EDGE_CURVE('',#7711,#7712,#3363,.T.);
#9615=EDGE_CURVE('',#7712,#7713,#3951,.T.);
#9616=EDGE_CURVE('',#7713,#7710,#3364,.T.);
#9617=EDGE_CURVE('',#7713,#7714,#3952,.T.);
#9618=EDGE_CURVE('',#7714,#7715,#3365,.T.);
#9619=EDGE_CURVE('',#7715,#7710,#3953,.T.);
#9620=EDGE_CURVE('',#7716,#7712,#3954,.T.);
#9621=EDGE_CURVE('',#7717,#7716,#3955,.T.);
#9622=EDGE_CURVE('',#7364,#7717,#3956,.T.);
#9623=EDGE_CURVE('',#7718,#7361,#3957,.T.);
#9624=EDGE_CURVE('',#7719,#7718,#3958,.T.);
#9625=EDGE_CURVE('',#7714,#7719,#3959,.T.);
#9626=EDGE_CURVE('',#7720,#7720,#3366,.T.);
#9627=EDGE_CURVE('',#7720,#7721,#4688,.T.);
#9628=EDGE_CURVE('',#7721,#7721,#3367,.T.);
#9629=EDGE_CURVE('',#7722,#7722,#3368,.T.);
#9630=EDGE_CURVE('',#7723,#7723,#3369,.T.);
#9631=EDGE_CURVE('',#7723,#7720,#4689,.T.);
#9632=EDGE_CURVE('',#7724,#7724,#3370,.T.);
#9633=EDGE_CURVE('',#7724,#7725,#4690,.T.);
#9634=EDGE_CURVE('',#7725,#7725,#3371,.T.);
#9635=EDGE_CURVE('',#7726,#7726,#3372,.T.);
#9636=EDGE_CURVE('',#7724,#7727,#4691,.T.);
#9637=EDGE_CURVE('',#7727,#7727,#3373,.T.);
#9638=EDGE_CURVE('',#7728,#7729,#978,.T.);
#9639=EDGE_CURVE('',#7729,#7730,#4692,.T.);
#9640=EDGE_CURVE('',#7730,#7731,#979,.T.);
#9641=EDGE_CURVE('',#7731,#7732,#980,.T.);
#9642=EDGE_CURVE('',#7732,#7728,#4693,.T.);
#9643=EDGE_CURVE('',#7731,#7733,#3960,.T.);
#9644=EDGE_CURVE('',#7733,#7734,#3374,.T.);
#9645=EDGE_CURVE('',#7734,#7735,#3961,.T.);
#9646=EDGE_CURVE('',#7735,#7736,#981,.T.);
#9647=EDGE_CURVE('',#7736,#7732,#3375,.T.);
#9648=EDGE_CURVE('',#7730,#7737,#3376,.T.);
#9649=EDGE_CURVE('',#7738,#7737,#982,.T.);
#9650=EDGE_CURVE('',#7739,#7738,#3962,.T.);
#9651=EDGE_CURVE('',#7733,#7739,#3377,.T.);
#9652=EDGE_CURVE('',#7729,#7617,#3378,.T.);
#9653=EDGE_CURVE('',#7616,#7740,#3379,.T.);
#9654=EDGE_CURVE('',#7740,#7741,#3963,.T.);
#9655=EDGE_CURVE('',#7741,#7742,#3380,.T.);
#9656=EDGE_CURVE('',#7737,#7742,#4694,.T.);
#9657=EDGE_CURVE('',#7742,#7743,#983,.T.);
#9658=EDGE_CURVE('',#7743,#7744,#4695,.T.);
#9659=EDGE_CURVE('',#7744,#7738,#984,.T.);
#9660=EDGE_CURVE('',#7744,#7745,#3381,.T.);
#9661=EDGE_CURVE('',#7746,#7745,#985,.T.);
#9662=EDGE_CURVE('',#7746,#7747,#3964,.T.);
#9663=EDGE_CURVE('',#7747,#7739,#3382,.T.);
#9664=EDGE_CURVE('',#7748,#7749,#986,.T.);
#9665=EDGE_CURVE('',#7749,#7750,#4696,.T.);
#9666=EDGE_CURVE('',#7750,#7746,#987,.T.);
#9667=EDGE_CURVE('',#7745,#7748,#4697,.T.);
#9668=EDGE_CURVE('',#7750,#7751,#3383,.T.);
#9669=EDGE_CURVE('',#7752,#7751,#988,.T.);
#9670=EDGE_CURVE('',#7753,#7752,#3965,.T.);
#9671=EDGE_CURVE('',#7747,#7753,#3384,.T.);
#9672=EDGE_CURVE('',#7749,#7627,#3385,.T.);
#9673=EDGE_CURVE('',#7626,#7754,#3386,.T.);
#9674=EDGE_CURVE('',#7754,#7755,#3966,.T.);
#9675=EDGE_CURVE('',#7755,#7756,#3387,.T.);
#9676=EDGE_CURVE('',#7751,#7756,#4698,.T.);
#9677=EDGE_CURVE('',#7756,#7757,#989,.T.);
#9678=EDGE_CURVE('',#7757,#7758,#4699,.T.);
#9679=EDGE_CURVE('',#7758,#7752,#990,.T.);
#9680=EDGE_CURVE('',#7758,#7759,#3388,.T.);
#9681=EDGE_CURVE('',#7760,#7759,#991,.T.);
#9682=EDGE_CURVE('',#7760,#7761,#3967,.T.);
#9683=EDGE_CURVE('',#7761,#7753,#3389,.T.);
#9684=EDGE_CURVE('',#7762,#7763,#992,.T.);
#9685=EDGE_CURVE('',#7763,#7764,#4700,.T.);
#9686=EDGE_CURVE('',#7764,#7760,#993,.T.);
#9687=EDGE_CURVE('',#7759,#7762,#4701,.T.);
#9688=EDGE_CURVE('',#7764,#7765,#3390,.T.);
#9689=EDGE_CURVE('',#7766,#7765,#994,.T.);
#9690=EDGE_CURVE('',#7767,#7766,#3968,.T.);
#9691=EDGE_CURVE('',#7761,#7767,#3391,.T.);
#9692=EDGE_CURVE('',#7763,#7637,#3392,.T.);
#9693=EDGE_CURVE('',#7636,#7768,#3393,.T.);
#9694=EDGE_CURVE('',#7768,#7769,#3969,.T.);
#9695=EDGE_CURVE('',#7769,#7770,#3394,.T.);
#9696=EDGE_CURVE('',#7765,#7770,#4702,.T.);
#9697=EDGE_CURVE('',#7770,#7771,#995,.T.);
#9698=EDGE_CURVE('',#7771,#7772,#4703,.T.);
#9699=EDGE_CURVE('',#7772,#7766,#996,.T.);
#9700=EDGE_CURVE('',#7772,#7773,#3395,.T.);
#9701=EDGE_CURVE('',#7774,#7773,#997,.T.);
#9702=EDGE_CURVE('',#7774,#7775,#3970,.T.);
#9703=EDGE_CURVE('',#7775,#7767,#3396,.T.);
#9704=EDGE_CURVE('',#7776,#7777,#998,.T.);
#9705=EDGE_CURVE('',#7777,#7778,#4704,.T.);
#9706=EDGE_CURVE('',#7778,#7774,#999,.T.);
#9707=EDGE_CURVE('',#7773,#7776,#4705,.T.);
#9708=EDGE_CURVE('',#7778,#7779,#3397,.T.);
#9709=EDGE_CURVE('',#7780,#7779,#1000,.T.);
#9710=EDGE_CURVE('',#7781,#7780,#3971,.T.);
#9711=EDGE_CURVE('',#7775,#7781,#3398,.T.);
#9712=EDGE_CURVE('',#7777,#7647,#3399,.T.);
#9713=EDGE_CURVE('',#7646,#7782,#3400,.T.);
#9714=EDGE_CURVE('',#7782,#7783,#3972,.T.);
#9715=EDGE_CURVE('',#7783,#7784,#3401,.T.);
#9716=EDGE_CURVE('',#7779,#7784,#4706,.T.);
#9717=EDGE_CURVE('',#7784,#7785,#1001,.T.);
#9718=EDGE_CURVE('',#7785,#7786,#4707,.T.);
#9719=EDGE_CURVE('',#7786,#7780,#1002,.T.);
#9720=EDGE_CURVE('',#7786,#7787,#3402,.T.);
#9721=EDGE_CURVE('',#7788,#7787,#1003,.T.);
#9722=EDGE_CURVE('',#7788,#7789,#3973,.T.);
#9723=EDGE_CURVE('',#7789,#7781,#3403,.T.);
#9724=EDGE_CURVE('',#7790,#7791,#1004,.T.);
#9725=EDGE_CURVE('',#7791,#7792,#4708,.T.);
#9726=EDGE_CURVE('',#7792,#7788,#1005,.T.);
#9727=EDGE_CURVE('',#7787,#7790,#4709,.T.);
#9728=EDGE_CURVE('',#7792,#7793,#3404,.T.);
#9729=EDGE_CURVE('',#7794,#7793,#1006,.T.);
#9730=EDGE_CURVE('',#7795,#7794,#3974,.T.);
#9731=EDGE_CURVE('',#7789,#7795,#3405,.T.);
#9732=EDGE_CURVE('',#7791,#7657,#3406,.T.);
#9733=EDGE_CURVE('',#7656,#7796,#3407,.T.);
#9734=EDGE_CURVE('',#7796,#7797,#3975,.T.);
#9735=EDGE_CURVE('',#7797,#7798,#3408,.T.);
#9736=EDGE_CURVE('',#7793,#7798,#4710,.T.);
#9737=EDGE_CURVE('',#7798,#7799,#1007,.T.);
#9738=EDGE_CURVE('',#7799,#7800,#4711,.T.);
#9739=EDGE_CURVE('',#7800,#7794,#1008,.T.);
#9740=EDGE_CURVE('',#7800,#7801,#3409,.T.);
#9741=EDGE_CURVE('',#7801,#7802,#1009,.T.);
#9742=EDGE_CURVE('',#7802,#7803,#3976,.T.);
#9743=EDGE_CURVE('',#7803,#7795,#3410,.T.);
#9744=EDGE_CURVE('',#7803,#7804,#3411,.T.);
#9745=EDGE_CURVE('',#7805,#7804,#3412,.T.);
#9746=EDGE_CURVE('',#7805,#7806,#3413,.T.);
#9747=EDGE_CURVE('',#7807,#7806,#3414,.T.);
#9748=EDGE_CURVE('',#7807,#7808,#3415,.T.);
#9749=EDGE_CURVE('',#7809,#7808,#3416,.T.);
#9750=EDGE_CURVE('',#7809,#7810,#3417,.T.);
#9751=EDGE_CURVE('',#7811,#7810,#3418,.T.);
#9752=EDGE_CURVE('',#7811,#7812,#3419,.T.);
#9753=EDGE_CURVE('',#7813,#7812,#3420,.T.);
#9754=EDGE_CURVE('',#7813,#7814,#3421,.T.);
#9755=EDGE_CURVE('',#7815,#7814,#3422,.T.);
#9756=EDGE_CURVE('',#7815,#7734,#3423,.T.);
#9757=EDGE_CURVE('',#7816,#7816,#3424,.T.);
#9758=EDGE_CURVE('',#7817,#7802,#1010,.T.);
#9759=EDGE_CURVE('',#7817,#7818,#3425,.T.);
#9760=EDGE_CURVE('',#7819,#7818,#1011,.T.);
#9761=EDGE_CURVE('',#7804,#7819,#3977,.T.);
#9762=EDGE_CURVE('',#7801,#7820,#4712,.T.);
#9763=EDGE_CURVE('',#7820,#7821,#1012,.T.);
#9764=EDGE_CURVE('',#7821,#7817,#4713,.T.);
#9765=EDGE_CURVE('',#7440,#7743,#3978,.T.);
#9766=EDGE_CURVE('',#7438,#7439,#3426,.T.);
#9767=EDGE_CURVE('',#7748,#7437,#3979,.T.);
#9768=EDGE_CURVE('',#7822,#7736,#4714,.T.);
#9769=EDGE_CURVE('',#7448,#7822,#3980,.T.);
#9770=EDGE_CURVE('',#7446,#7447,#3427,.T.);
#9771=EDGE_CURVE('',#7728,#7445,#3981,.T.);
#9772=EDGE_CURVE('',#7735,#7823,#1013,.T.);
#9773=EDGE_CURVE('',#7823,#7824,#4715,.T.);
#9774=EDGE_CURVE('',#7824,#7822,#1014,.T.);
#9775=EDGE_CURVE('',#7821,#7667,#3428,.T.);
#9776=EDGE_CURVE('',#7666,#7825,#3429,.T.);
#9777=EDGE_CURVE('',#7825,#7826,#3982,.T.);
#9778=EDGE_CURVE('',#7826,#7827,#3430,.T.);
#9779=EDGE_CURVE('',#7818,#7827,#4716,.T.);
#9780=EDGE_CURVE('',#7827,#7828,#1015,.T.);
#9781=EDGE_CURVE('',#7828,#7829,#4717,.T.);
#9782=EDGE_CURVE('',#7829,#7819,#1016,.T.);
#9783=EDGE_CURVE('',#7829,#7830,#3431,.T.);
#9784=EDGE_CURVE('',#7830,#7831,#1017,.T.);
#9785=EDGE_CURVE('',#7831,#7805,#3983,.T.);
#9786=EDGE_CURVE('',#7832,#7831,#1018,.T.);
#9787=EDGE_CURVE('',#7832,#7833,#3432,.T.);
#9788=EDGE_CURVE('',#7834,#7833,#1019,.T.);
#9789=EDGE_CURVE('',#7806,#7834,#3984,.T.);
#9790=EDGE_CURVE('',#7830,#7835,#4718,.T.);
#9791=EDGE_CURVE('',#7835,#7836,#1020,.T.);
#9792=EDGE_CURVE('',#7836,#7832,#4719,.T.);
#9793=EDGE_CURVE('',#7836,#7677,#3433,.T.);
#9794=EDGE_CURVE('',#7676,#7837,#3434,.T.);
#9795=EDGE_CURVE('',#7837,#7838,#3985,.T.);
#9796=EDGE_CURVE('',#7838,#7839,#3435,.T.);
#9797=EDGE_CURVE('',#7833,#7839,#4720,.T.);
#9798=EDGE_CURVE('',#7839,#7840,#1021,.T.);
#9799=EDGE_CURVE('',#7840,#7841,#4721,.T.);
#9800=EDGE_CURVE('',#7841,#7834,#1022,.T.);
#9801=EDGE_CURVE('',#7841,#7842,#3436,.T.);
#9802=EDGE_CURVE('',#7842,#7843,#1023,.T.);
#9803=EDGE_CURVE('',#7843,#7807,#3986,.T.);
#9804=EDGE_CURVE('',#7844,#7843,#1024,.T.);
#9805=EDGE_CURVE('',#7844,#7845,#3437,.T.);
#9806=EDGE_CURVE('',#7846,#7845,#1025,.T.);
#9807=EDGE_CURVE('',#7808,#7846,#3987,.T.);
#9808=EDGE_CURVE('',#7842,#7847,#4722,.T.);
#9809=EDGE_CURVE('',#7847,#7848,#1026,.T.);
#9810=EDGE_CURVE('',#7848,#7844,#4723,.T.);
#9811=EDGE_CURVE('',#7848,#7687,#3438,.T.);
#9812=EDGE_CURVE('',#7686,#7849,#3439,.T.);
#9813=EDGE_CURVE('',#7849,#7850,#3988,.T.);
#9814=EDGE_CURVE('',#7850,#7851,#3440,.T.);
#9815=EDGE_CURVE('',#7845,#7851,#4724,.T.);
#9816=EDGE_CURVE('',#7851,#7852,#1027,.T.);
#9817=EDGE_CURVE('',#7852,#7853,#4725,.T.);
#9818=EDGE_CURVE('',#7853,#7846,#1028,.T.);
#9819=EDGE_CURVE('',#7853,#7854,#3441,.T.);
#9820=EDGE_CURVE('',#7854,#7855,#1029,.T.);
#9821=EDGE_CURVE('',#7855,#7809,#3989,.T.);
#9822=EDGE_CURVE('',#7856,#7855,#1030,.T.);
#9823=EDGE_CURVE('',#7856,#7857,#3442,.T.);
#9824=EDGE_CURVE('',#7858,#7857,#1031,.T.);
#9825=EDGE_CURVE('',#7810,#7858,#3990,.T.);
#9826=EDGE_CURVE('',#7854,#7859,#4726,.T.);
#9827=EDGE_CURVE('',#7859,#7860,#1032,.T.);
#9828=EDGE_CURVE('',#7860,#7856,#4727,.T.);
#9829=EDGE_CURVE('',#7860,#7697,#3443,.T.);
#9830=EDGE_CURVE('',#7696,#7861,#3444,.T.);
#9831=EDGE_CURVE('',#7861,#7862,#3991,.T.);
#9832=EDGE_CURVE('',#7862,#7863,#3445,.T.);
#9833=EDGE_CURVE('',#7857,#7863,#4728,.T.);
#9834=EDGE_CURVE('',#7863,#7864,#1033,.T.);
#9835=EDGE_CURVE('',#7864,#7865,#4729,.T.);
#9836=EDGE_CURVE('',#7865,#7858,#1034,.T.);
#9837=EDGE_CURVE('',#7865,#7866,#3446,.T.);
#9838=EDGE_CURVE('',#7866,#7867,#1035,.T.);
#9839=EDGE_CURVE('',#7867,#7811,#3992,.T.);
#9840=EDGE_CURVE('',#7868,#7867,#1036,.T.);
#9841=EDGE_CURVE('',#7868,#7869,#3447,.T.);
#9842=EDGE_CURVE('',#7870,#7869,#1037,.T.);
#9843=EDGE_CURVE('',#7812,#7870,#3993,.T.);
#9844=EDGE_CURVE('',#7866,#7871,#4730,.T.);
#9845=EDGE_CURVE('',#7871,#7872,#1038,.T.);
#9846=EDGE_CURVE('',#7872,#7868,#4731,.T.);
#9847=EDGE_CURVE('',#7872,#7707,#3448,.T.);
#9848=EDGE_CURVE('',#7706,#7873,#3449,.T.);
#9849=EDGE_CURVE('',#7873,#7874,#3994,.T.);
#9850=EDGE_CURVE('',#7874,#7875,#3450,.T.);
#9851=EDGE_CURVE('',#7869,#7875,#4732,.T.);
#9852=EDGE_CURVE('',#7875,#7876,#1039,.T.);
#9853=EDGE_CURVE('',#7876,#7877,#4733,.T.);
#9854=EDGE_CURVE('',#7877,#7870,#1040,.T.);
#9855=EDGE_CURVE('',#7877,#7878,#3451,.T.);
#9856=EDGE_CURVE('',#7878,#7879,#1041,.T.);
#9857=EDGE_CURVE('',#7879,#7813,#3995,.T.);
#9858=EDGE_CURVE('',#7880,#7879,#1042,.T.);
#9859=EDGE_CURVE('',#7880,#7881,#3452,.T.);
#9860=EDGE_CURVE('',#7882,#7881,#1043,.T.);
#9861=EDGE_CURVE('',#7814,#7882,#3996,.T.);
#9862=EDGE_CURVE('',#7878,#7883,#4734,.T.);
#9863=EDGE_CURVE('',#7883,#7884,#1044,.T.);
#9864=EDGE_CURVE('',#7884,#7880,#4735,.T.);
#9865=EDGE_CURVE('',#7885,#7823,#3453,.T.);
#9866=EDGE_CURVE('',#7886,#7885,#4736,.T.);
#9867=EDGE_CURVE('',#7886,#7606,#3454,.T.);
#9868=EDGE_CURVE('',#7605,#7887,#3455,.T.);
#9869=EDGE_CURVE('',#7887,#7888,#3997,.T.);
#9870=EDGE_CURVE('',#7888,#7824,#3456,.T.);
#9871=EDGE_CURVE('',#7889,#7815,#3998,.T.);
#9872=EDGE_CURVE('',#7885,#7889,#1045,.T.);
#9873=EDGE_CURVE('',#7884,#7717,#3457,.T.);
#9874=EDGE_CURVE('',#7716,#7890,#3458,.T.);
#9875=EDGE_CURVE('',#7890,#7891,#3999,.T.);
#9876=EDGE_CURVE('',#7891,#7892,#3459,.T.);
#9877=EDGE_CURVE('',#7881,#7892,#4737,.T.);
#9878=EDGE_CURVE('',#7892,#7893,#1046,.T.);
#9879=EDGE_CURVE('',#7893,#7894,#4738,.T.);
#9880=EDGE_CURVE('',#7894,#7882,#1047,.T.);
#9881=EDGE_CURVE('',#7894,#7895,#3460,.T.);
#9882=EDGE_CURVE('',#7895,#7889,#1048,.T.);
#9883=EDGE_CURVE('',#7895,#7896,#4739,.T.);
#9884=EDGE_CURVE('',#7896,#7886,#1049,.T.);
#9885=EDGE_CURVE('',#7896,#7897,#4000,.T.);
#9886=EDGE_CURVE('',#7897,#7607,#3461,.T.);
#9887=EDGE_CURVE('',#7898,#7893,#4001,.T.);
#9888=EDGE_CURVE('',#7899,#7898,#4002,.T.);
#9889=EDGE_CURVE('',#7900,#7899,#3462,.T.);
#9890=EDGE_CURVE('',#7897,#7900,#4003,.T.);
#9891=EDGE_CURVE('',#7454,#7901,#4004,.T.);
#9892=EDGE_CURVE('',#7902,#7901,#3463,.F.);
#9893=EDGE_CURVE('',#7903,#7902,#3464,.F.);
#9894=EDGE_CURVE('',#7903,#7455,#4005,.T.);
#9895=EDGE_CURVE('',#7357,#7903,#4006,.T.);
#9896=EDGE_CURVE('',#7904,#7327,#4007,.T.);
#9897=EDGE_CURVE('',#7904,#7485,#4008,.T.);
#9898=EDGE_CURVE('',#7327,#7905,#3465,.T.);
#9899=EDGE_CURVE('',#7905,#7326,#3466,.T.);
#9900=EDGE_CURVE('',#7326,#7906,#4009,.T.);
#9901=EDGE_CURVE('',#7906,#7904,#3467,.T.);
#9902=EDGE_CURVE('',#7906,#7484,#4010,.T.);
#9903=EDGE_CURVE('',#7901,#7356,#4011,.T.);
#9904=EDGE_CURVE('',#7900,#7899,#4012,.T.);
#9905=EDGE_CURVE('',#7907,#7898,#3468,.T.);
#9906=EDGE_CURVE('',#7907,#7358,#4013,.T.);
#9907=EDGE_CURVE('',#7891,#7907,#4014,.T.);
#9908=EDGE_CURVE('',#7366,#7367,#3469,.T.);
#9909=EDGE_CURVE('',#7368,#7876,#4015,.T.);
#9910=EDGE_CURVE('',#7883,#7365,#4016,.T.);
#9911=EDGE_CURVE('',#7874,#7369,#4017,.T.);
#9912=EDGE_CURVE('',#7374,#7375,#3470,.T.);
#9913=EDGE_CURVE('',#7376,#7864,#4018,.T.);
#9914=EDGE_CURVE('',#7871,#7373,#4019,.T.);
#9915=EDGE_CURVE('',#7862,#7377,#4020,.T.);
#9916=EDGE_CURVE('',#7382,#7383,#3471,.T.);
#9917=EDGE_CURVE('',#7384,#7852,#4021,.T.);
#9918=EDGE_CURVE('',#7859,#7381,#4022,.T.);
#9919=EDGE_CURVE('',#7850,#7385,#4023,.T.);
#9920=EDGE_CURVE('',#7390,#7391,#3472,.T.);
#9921=EDGE_CURVE('',#7392,#7840,#4024,.T.);
#9922=EDGE_CURVE('',#7847,#7389,#4025,.T.);
#9923=EDGE_CURVE('',#7838,#7393,#4026,.T.);
#9924=EDGE_CURVE('',#7398,#7399,#3473,.T.);
#9925=EDGE_CURVE('',#7400,#7828,#4027,.T.);
#9926=EDGE_CURVE('',#7835,#7397,#4028,.T.);
#9927=EDGE_CURVE('',#7826,#7401,#4029,.T.);
#9928=EDGE_CURVE('',#7406,#7407,#3474,.T.);
#9929=EDGE_CURVE('',#7408,#7799,#4030,.T.);
#9930=EDGE_CURVE('',#7820,#7405,#4031,.T.);
#9931=EDGE_CURVE('',#7797,#7409,#4032,.T.);
#9932=EDGE_CURVE('',#7414,#7415,#3475,.T.);
#9933=EDGE_CURVE('',#7416,#7785,#4033,.T.);
#9934=EDGE_CURVE('',#7790,#7413,#4034,.T.);
#9935=EDGE_CURVE('',#7783,#7417,#4035,.T.);
#9936=EDGE_CURVE('',#7422,#7423,#3476,.T.);
#9937=EDGE_CURVE('',#7424,#7771,#4036,.T.);
#9938=EDGE_CURVE('',#7776,#7421,#4037,.T.);
#9939=EDGE_CURVE('',#7769,#7425,#4038,.T.);
#9940=EDGE_CURVE('',#7430,#7431,#3477,.T.);
#9941=EDGE_CURVE('',#7432,#7757,#4039,.T.);
#9942=EDGE_CURVE('',#7762,#7429,#4040,.T.);
#9943=EDGE_CURVE('',#7755,#7433,#4041,.T.);
#9944=EDGE_CURVE('',#7741,#7441,#4042,.T.);
#9945=EDGE_CURVE('',#7888,#7449,#4043,.T.);
#9946=EDGE_CURVE('',#7908,#7908,#3478,.T.);
#9947=EDGE_CURVE('',#7908,#7909,#4740,.T.);
#9948=EDGE_CURVE('',#7909,#7909,#3479,.T.);
#9949=EDGE_CURVE('',#7910,#7910,#3480,.T.);
#9950=EDGE_CURVE('',#7911,#7911,#3481,.T.);
#9951=EDGE_CURVE('',#7911,#7910,#4741,.T.);
#9952=EDGE_CURVE('',#7726,#7722,#4742,.T.);
#9953=EDGE_CURVE('',#7360,#7912,#4044,.T.);
#9954=EDGE_CURVE('',#7718,#7912,#3482,.T.);
#9955=EDGE_CURVE('',#7711,#7890,#4045,.T.);
#9956=EDGE_CURVE('',#7912,#7715,#4046,.T.);
#9957=EDGE_CURVE('',#7370,#7913,#4047,.T.);
#9958=EDGE_CURVE('',#7708,#7913,#3483,.T.);
#9959=EDGE_CURVE('',#7701,#7873,#4048,.T.);
#9960=EDGE_CURVE('',#7913,#7705,#4049,.T.);
#9961=EDGE_CURVE('',#7378,#7914,#4050,.T.);
#9962=EDGE_CURVE('',#7698,#7914,#3484,.T.);
#9963=EDGE_CURVE('',#7691,#7861,#4051,.T.);
#9964=EDGE_CURVE('',#7914,#7695,#4052,.T.);
#9965=EDGE_CURVE('',#7386,#7915,#4053,.T.);
#9966=EDGE_CURVE('',#7688,#7915,#3485,.T.);
#9967=EDGE_CURVE('',#7681,#7849,#4054,.T.);
#9968=EDGE_CURVE('',#7915,#7685,#4055,.T.);
#9969=EDGE_CURVE('',#7394,#7916,#4056,.T.);
#9970=EDGE_CURVE('',#7678,#7916,#3486,.T.);
#9971=EDGE_CURVE('',#7671,#7837,#4057,.T.);
#9972=EDGE_CURVE('',#7916,#7675,#4058,.T.);
#9973=EDGE_CURVE('',#7402,#7917,#4059,.T.);
#9974=EDGE_CURVE('',#7668,#7917,#3487,.T.);
#9975=EDGE_CURVE('',#7661,#7825,#4060,.T.);
#9976=EDGE_CURVE('',#7917,#7665,#4061,.T.);
#9977=EDGE_CURVE('',#7410,#7918,#4062,.T.);
#9978=EDGE_CURVE('',#7658,#7918,#3488,.T.);
#9979=EDGE_CURVE('',#7651,#7796,#4063,.T.);
#9980=EDGE_CURVE('',#7918,#7655,#4064,.T.);
#9981=EDGE_CURVE('',#7418,#7919,#4065,.T.);
#9982=EDGE_CURVE('',#7648,#7919,#3489,.T.);
#9983=EDGE_CURVE('',#7641,#7782,#4066,.T.);
#9984=EDGE_CURVE('',#7919,#7645,#4067,.T.);
#9985=EDGE_CURVE('',#7426,#7920,#4068,.T.);
#9986=EDGE_CURVE('',#7638,#7920,#3490,.T.);
#9987=EDGE_CURVE('',#7631,#7768,#4069,.T.);
#9988=EDGE_CURVE('',#7920,#7635,#4070,.T.);
#9989=EDGE_CURVE('',#7434,#7921,#4071,.T.);
#9990=EDGE_CURVE('',#7628,#7921,#3491,.T.);
#9991=EDGE_CURVE('',#7621,#7754,#4072,.T.);
#9992=EDGE_CURVE('',#7921,#7625,#4073,.T.);
#9993=EDGE_CURVE('',#7442,#7922,#4074,.T.);
#9994=EDGE_CURVE('',#7618,#7922,#3492,.T.);
#9995=EDGE_CURVE('',#7611,#7740,#4075,.T.);
#9996=EDGE_CURVE('',#7922,#7615,#4076,.T.);
#9997=EDGE_CURVE('',#7450,#7923,#4077,.T.);
#9998=EDGE_CURVE('',#7608,#7923,#3493,.T.);
#9999=EDGE_CURVE('',#7600,#7887,#4078,.T.);
#10000=EDGE_CURVE('',#7923,#7604,#4079,.T.);
#10001=EDGE_CURVE('',#7551,#7559,#4743,.T.);
#10002=EDGE_CURVE('',#7562,#7553,#4744,.T.);
#10003=EDGE_CURVE('',#7597,#7586,#4745,.T.);
#10004=EDGE_CURVE('',#7588,#7577,#4746,.T.);
#10005=EDGE_CURVE('',#7579,#7568,#4747,.T.);
#10006=EDGE_CURVE('',#7570,#7557,#4748,.T.);
#10007=EDGE_CURVE('',#7560,#7550,#4749,.T.);
#10008=EDGE_CURVE('',#7552,#7541,#4750,.T.);
#10009=EDGE_CURVE('',#7526,#7532,#4751,.T.);
#10010=EDGE_CURVE('',#7517,#7523,#4752,.T.);
#10011=EDGE_CURVE('',#7508,#7514,#4753,.T.);
#10012=EDGE_CURVE('',#7497,#7505,#4754,.T.);
#10013=EDGE_CURVE('',#7543,#7494,#4755,.T.);
#10014=EDGE_CURVE('',#7535,#7595,#4756,.T.);
#10015=EDGE_CURVE('',#7924,#7924,#3494,.T.);
#10016=EDGE_CURVE('',#7924,#7816,#4757,.T.);
#10017=EDGE_CURVE('',#7489,#7924,#4758,.T.);
#10018=EDGE_CURVE('',#7727,#7490,#4759,.T.);
#10019=EDGE_CURVE('',#7925,#7925,#3495,.T.);
#10020=EDGE_CURVE('',#7925,#7911,#4760,.T.);
#10021=EDGE_CURVE('',#7926,#7926,#3496,.T.);
#10022=EDGE_CURVE('',#7927,#7927,#3497,.T.);
#10023=EDGE_CURVE('',#7927,#7926,#4761,.T.);
#10024=EDGE_CURVE('',#7928,#7928,#3498,.T.);
#10025=EDGE_CURVE('',#7928,#7927,#4762,.T.);
#10026=EDGE_CURVE('',#7929,#7929,#3499,.T.);
#10027=EDGE_CURVE('',#7929,#7928,#4763,.T.);
#10028=EDGE_CURVE('',#7930,#7930,#3500,.T.);
#10029=EDGE_CURVE('',#7930,#7929,#4764,.T.);
#10030=EDGE_CURVE('',#7931,#7931,#3501,.T.);
#10031=EDGE_CURVE('',#7932,#7932,#3502,.T.);
#10032=EDGE_CURVE('',#7932,#7931,#4765,.T.);
#10033=EDGE_CURVE('',#7933,#7933,#3503,.T.);
#10034=EDGE_CURVE('',#7933,#7932,#4766,.T.);
#10035=EDGE_CURVE('',#7934,#7934,#3504,.T.);
#10036=EDGE_CURVE('',#7934,#7933,#4767,.T.);
#10037=EDGE_CURVE('',#7935,#7935,#3505,.T.);
#10038=EDGE_CURVE('',#7935,#7934,#4768,.T.);
#10039=EDGE_CURVE('',#7936,#7936,#3506,.T.);
#10040=EDGE_CURVE('',#7936,#7935,#4769,.T.);
#10041=EDGE_CURVE('',#7905,#7936,#4770,.T.);
#10042=EDGE_CURVE('',#7901,#7903,#3507,.F.);
#10043=EDGE_CURVE('',#7937,#7937,#3508,.T.);
#10044=EDGE_CURVE('',#7937,#7902,#4771,.T.);
#11815=ORIENTED_EDGE('',*,*,#9115,.F.);
#11816=ORIENTED_EDGE('',*,*,#9116,.T.);
#11817=ORIENTED_EDGE('',*,*,#9117,.T.);
#11818=ORIENTED_EDGE('',*,*,#9118,.T.);
#11819=ORIENTED_EDGE('',*,*,#9119,.F.);
#11820=ORIENTED_EDGE('',*,*,#9120,.T.);
#11821=ORIENTED_EDGE('',*,*,#9115,.T.);
#11822=ORIENTED_EDGE('',*,*,#9121,.T.);
#11823=ORIENTED_EDGE('',*,*,#9122,.F.);
#11824=ORIENTED_EDGE('',*,*,#9123,.T.);
#11825=ORIENTED_EDGE('',*,*,#9119,.T.);
#11826=ORIENTED_EDGE('',*,*,#9124,.T.);
#11827=ORIENTED_EDGE('',*,*,#9125,.F.);
#11828=ORIENTED_EDGE('',*,*,#9126,.T.);
#11829=ORIENTED_EDGE('',*,*,#9122,.T.);
#11830=ORIENTED_EDGE('',*,*,#9127,.T.);
#11831=ORIENTED_EDGE('',*,*,#9128,.F.);
#11832=ORIENTED_EDGE('',*,*,#9129,.T.);
#11833=ORIENTED_EDGE('',*,*,#9125,.T.);
#11834=ORIENTED_EDGE('',*,*,#9130,.T.);
#11835=ORIENTED_EDGE('',*,*,#9131,.F.);
#11836=ORIENTED_EDGE('',*,*,#9132,.T.);
#11837=ORIENTED_EDGE('',*,*,#9128,.T.);
#11838=ORIENTED_EDGE('',*,*,#9133,.T.);
#11839=ORIENTED_EDGE('',*,*,#9134,.F.);
#11840=ORIENTED_EDGE('',*,*,#9135,.T.);
#11841=ORIENTED_EDGE('',*,*,#9131,.T.);
#11842=ORIENTED_EDGE('',*,*,#9136,.T.);
#11843=ORIENTED_EDGE('',*,*,#9137,.F.);
#11844=ORIENTED_EDGE('',*,*,#9138,.T.);
#11845=ORIENTED_EDGE('',*,*,#9134,.T.);
#11846=ORIENTED_EDGE('',*,*,#9139,.T.);
#11847=ORIENTED_EDGE('',*,*,#9140,.F.);
#11848=ORIENTED_EDGE('',*,*,#9141,.T.);
#11849=ORIENTED_EDGE('',*,*,#9137,.T.);
#11850=ORIENTED_EDGE('',*,*,#9142,.T.);
#11851=ORIENTED_EDGE('',*,*,#9143,.F.);
#11852=ORIENTED_EDGE('',*,*,#9144,.T.);
#11853=ORIENTED_EDGE('',*,*,#9140,.T.);
#11854=ORIENTED_EDGE('',*,*,#9145,.T.);
#11855=ORIENTED_EDGE('',*,*,#9146,.F.);
#11856=ORIENTED_EDGE('',*,*,#9147,.T.);
#11857=ORIENTED_EDGE('',*,*,#9143,.T.);
#11858=ORIENTED_EDGE('',*,*,#9148,.T.);
#11859=ORIENTED_EDGE('',*,*,#9149,.F.);
#11860=ORIENTED_EDGE('',*,*,#9150,.T.);
#11861=ORIENTED_EDGE('',*,*,#9146,.T.);
#11862=ORIENTED_EDGE('',*,*,#9151,.T.);
#11863=ORIENTED_EDGE('',*,*,#9152,.F.);
#11864=ORIENTED_EDGE('',*,*,#9153,.T.);
#11865=ORIENTED_EDGE('',*,*,#9149,.T.);
#11866=ORIENTED_EDGE('',*,*,#9154,.T.);
#11867=ORIENTED_EDGE('',*,*,#9155,.F.);
#11868=ORIENTED_EDGE('',*,*,#9156,.T.);
#11869=ORIENTED_EDGE('',*,*,#9152,.T.);
#11870=ORIENTED_EDGE('',*,*,#9157,.T.);
#11871=ORIENTED_EDGE('',*,*,#9158,.F.);
#11872=ORIENTED_EDGE('',*,*,#9159,.T.);
#11873=ORIENTED_EDGE('',*,*,#9155,.T.);
#11874=ORIENTED_EDGE('',*,*,#9160,.T.);
#11875=ORIENTED_EDGE('',*,*,#9161,.F.);
#11876=ORIENTED_EDGE('',*,*,#9162,.T.);
#11877=ORIENTED_EDGE('',*,*,#9158,.T.);
#11878=ORIENTED_EDGE('',*,*,#9163,.T.);
#11879=ORIENTED_EDGE('',*,*,#9164,.F.);
#11880=ORIENTED_EDGE('',*,*,#9165,.T.);
#11881=ORIENTED_EDGE('',*,*,#9166,.T.);
#11882=ORIENTED_EDGE('',*,*,#9167,.T.);
#11883=ORIENTED_EDGE('',*,*,#9168,.F.);
#11884=ORIENTED_EDGE('',*,*,#9169,.T.);
#11885=ORIENTED_EDGE('',*,*,#9168,.T.);
#11886=ORIENTED_EDGE('',*,*,#9170,.T.);
#11887=ORIENTED_EDGE('',*,*,#9171,.F.);
#11888=ORIENTED_EDGE('',*,*,#9172,.T.);
#11889=ORIENTED_EDGE('',*,*,#9173,.T.);
#11890=ORIENTED_EDGE('',*,*,#9174,.T.);
#11891=ORIENTED_EDGE('',*,*,#9175,.F.);
#11892=ORIENTED_EDGE('',*,*,#9176,.T.);
#11893=ORIENTED_EDGE('',*,*,#9177,.T.);
#11894=ORIENTED_EDGE('',*,*,#9178,.T.);
#11895=ORIENTED_EDGE('',*,*,#9179,.F.);
#11896=ORIENTED_EDGE('',*,*,#9180,.T.);
#11897=ORIENTED_EDGE('',*,*,#9181,.T.);
#11898=ORIENTED_EDGE('',*,*,#9182,.T.);
#11899=ORIENTED_EDGE('',*,*,#9183,.F.);
#11900=ORIENTED_EDGE('',*,*,#9184,.T.);
#11901=ORIENTED_EDGE('',*,*,#9185,.T.);
#11902=ORIENTED_EDGE('',*,*,#9186,.T.);
#11903=ORIENTED_EDGE('',*,*,#9187,.F.);
#11904=ORIENTED_EDGE('',*,*,#9188,.T.);
#11905=ORIENTED_EDGE('',*,*,#9189,.T.);
#11906=ORIENTED_EDGE('',*,*,#9190,.T.);
#11907=ORIENTED_EDGE('',*,*,#9191,.F.);
#11908=ORIENTED_EDGE('',*,*,#9192,.T.);
#11909=ORIENTED_EDGE('',*,*,#9193,.T.);
#11910=ORIENTED_EDGE('',*,*,#9194,.T.);
#11911=ORIENTED_EDGE('',*,*,#9195,.F.);
#11912=ORIENTED_EDGE('',*,*,#9196,.T.);
#11913=ORIENTED_EDGE('',*,*,#9197,.T.);
#11914=ORIENTED_EDGE('',*,*,#9198,.T.);
#11915=ORIENTED_EDGE('',*,*,#9199,.F.);
#11916=ORIENTED_EDGE('',*,*,#9200,.T.);
#11917=ORIENTED_EDGE('',*,*,#9201,.T.);
#11918=ORIENTED_EDGE('',*,*,#9202,.T.);
#11919=ORIENTED_EDGE('',*,*,#9203,.F.);
#11920=ORIENTED_EDGE('',*,*,#9204,.T.);
#11921=ORIENTED_EDGE('',*,*,#9205,.T.);
#11922=ORIENTED_EDGE('',*,*,#9206,.T.);
#11923=ORIENTED_EDGE('',*,*,#9207,.F.);
#11924=ORIENTED_EDGE('',*,*,#9208,.T.);
#11925=ORIENTED_EDGE('',*,*,#9209,.T.);
#11926=ORIENTED_EDGE('',*,*,#9210,.T.);
#11927=ORIENTED_EDGE('',*,*,#9211,.F.);
#11928=ORIENTED_EDGE('',*,*,#9212,.T.);
#11929=ORIENTED_EDGE('',*,*,#9213,.T.);
#11930=ORIENTED_EDGE('',*,*,#9214,.T.);
#11931=ORIENTED_EDGE('',*,*,#9215,.F.);
#11932=ORIENTED_EDGE('',*,*,#9216,.T.);
#11933=ORIENTED_EDGE('',*,*,#9217,.T.);
#11934=ORIENTED_EDGE('',*,*,#9218,.T.);
#11935=ORIENTED_EDGE('',*,*,#9219,.F.);
#11936=ORIENTED_EDGE('',*,*,#9220,.T.);
#11937=ORIENTED_EDGE('',*,*,#9221,.T.);
#11938=ORIENTED_EDGE('',*,*,#9222,.T.);
#11939=ORIENTED_EDGE('',*,*,#9223,.F.);
#11940=ORIENTED_EDGE('',*,*,#9224,.T.);
#11941=ORIENTED_EDGE('',*,*,#9225,.T.);
#11942=ORIENTED_EDGE('',*,*,#9226,.T.);
#11943=ORIENTED_EDGE('',*,*,#9227,.F.);
#11944=ORIENTED_EDGE('',*,*,#9228,.T.);
#11945=ORIENTED_EDGE('',*,*,#9229,.T.);
#11946=ORIENTED_EDGE('',*,*,#9230,.T.);
#11947=ORIENTED_EDGE('',*,*,#9231,.F.);
#11948=ORIENTED_EDGE('',*,*,#9232,.T.);
#11949=ORIENTED_EDGE('',*,*,#9233,.T.);
#11950=ORIENTED_EDGE('',*,*,#9234,.T.);
#11951=ORIENTED_EDGE('',*,*,#9235,.F.);
#11952=ORIENTED_EDGE('',*,*,#9236,.T.);
#11953=ORIENTED_EDGE('',*,*,#9237,.T.);
#11954=ORIENTED_EDGE('',*,*,#9238,.T.);
#11955=ORIENTED_EDGE('',*,*,#9239,.F.);
#11956=ORIENTED_EDGE('',*,*,#9240,.T.);
#11957=ORIENTED_EDGE('',*,*,#9241,.T.);
#11958=ORIENTED_EDGE('',*,*,#9242,.T.);
#11959=ORIENTED_EDGE('',*,*,#9243,.F.);
#11960=ORIENTED_EDGE('',*,*,#9244,.T.);
#11961=ORIENTED_EDGE('',*,*,#9245,.T.);
#11962=ORIENTED_EDGE('',*,*,#9246,.T.);
#11963=ORIENTED_EDGE('',*,*,#9247,.F.);
#11964=ORIENTED_EDGE('',*,*,#9248,.T.);
#11965=ORIENTED_EDGE('',*,*,#9249,.T.);
#11966=ORIENTED_EDGE('',*,*,#9250,.T.);
#11967=ORIENTED_EDGE('',*,*,#9251,.F.);
#11968=ORIENTED_EDGE('',*,*,#9252,.T.);
#11969=ORIENTED_EDGE('',*,*,#9253,.T.);
#11970=ORIENTED_EDGE('',*,*,#9254,.T.);
#11971=ORIENTED_EDGE('',*,*,#9255,.F.);
#11972=ORIENTED_EDGE('',*,*,#9256,.T.);
#11973=ORIENTED_EDGE('',*,*,#9257,.T.);
#11974=ORIENTED_EDGE('',*,*,#9258,.T.);
#11975=ORIENTED_EDGE('',*,*,#9259,.F.);
#11976=ORIENTED_EDGE('',*,*,#9260,.T.);
#11977=ORIENTED_EDGE('',*,*,#9261,.F.);
#11978=ORIENTED_EDGE('',*,*,#9262,.F.);
#11979=ORIENTED_EDGE('',*,*,#9263,.F.);
#11980=ORIENTED_EDGE('',*,*,#9264,.T.);
#11981=ORIENTED_EDGE('',*,*,#9259,.T.);
#11982=ORIENTED_EDGE('',*,*,#9265,.F.);
#11983=ORIENTED_EDGE('',*,*,#9266,.F.);
#11984=ORIENTED_EDGE('',*,*,#9267,.T.);
#11985=ORIENTED_EDGE('',*,*,#9263,.T.);
#11986=ORIENTED_EDGE('',*,*,#9268,.F.);
#11987=ORIENTED_EDGE('',*,*,#9269,.F.);
#11988=ORIENTED_EDGE('',*,*,#9270,.T.);
#11989=ORIENTED_EDGE('',*,*,#9266,.T.);
#11990=ORIENTED_EDGE('',*,*,#9271,.F.);
#11991=ORIENTED_EDGE('',*,*,#9272,.F.);
#11992=ORIENTED_EDGE('',*,*,#9273,.T.);
#11993=ORIENTED_EDGE('',*,*,#9269,.T.);
#11994=ORIENTED_EDGE('',*,*,#9274,.F.);
#11995=ORIENTED_EDGE('',*,*,#9275,.F.);
#11996=ORIENTED_EDGE('',*,*,#9276,.T.);
#11997=ORIENTED_EDGE('',*,*,#9272,.T.);
#11998=ORIENTED_EDGE('',*,*,#9277,.F.);
#11999=ORIENTED_EDGE('',*,*,#9278,.F.);
#12000=ORIENTED_EDGE('',*,*,#9279,.T.);
#12001=ORIENTED_EDGE('',*,*,#9275,.T.);
#12002=ORIENTED_EDGE('',*,*,#9280,.F.);
#12003=ORIENTED_EDGE('',*,*,#9281,.F.);
#12004=ORIENTED_EDGE('',*,*,#9282,.T.);
#12005=ORIENTED_EDGE('',*,*,#9278,.T.);
#12006=ORIENTED_EDGE('',*,*,#9283,.F.);
#12007=ORIENTED_EDGE('',*,*,#9284,.F.);
#12008=ORIENTED_EDGE('',*,*,#9285,.T.);
#12009=ORIENTED_EDGE('',*,*,#9281,.T.);
#12010=ORIENTED_EDGE('',*,*,#9286,.F.);
#12011=ORIENTED_EDGE('',*,*,#9287,.F.);
#12012=ORIENTED_EDGE('',*,*,#9288,.T.);
#12013=ORIENTED_EDGE('',*,*,#9284,.T.);
#12014=ORIENTED_EDGE('',*,*,#9289,.F.);
#12015=ORIENTED_EDGE('',*,*,#9290,.F.);
#12016=ORIENTED_EDGE('',*,*,#9291,.T.);
#12017=ORIENTED_EDGE('',*,*,#9287,.T.);
#12018=ORIENTED_EDGE('',*,*,#9292,.F.);
#12019=ORIENTED_EDGE('',*,*,#9293,.F.);
#12020=ORIENTED_EDGE('',*,*,#9294,.T.);
#12021=ORIENTED_EDGE('',*,*,#9290,.T.);
#12022=ORIENTED_EDGE('',*,*,#9295,.F.);
#12023=ORIENTED_EDGE('',*,*,#9296,.F.);
#12024=ORIENTED_EDGE('',*,*,#9297,.T.);
#12025=ORIENTED_EDGE('',*,*,#9293,.T.);
#12026=ORIENTED_EDGE('',*,*,#9298,.F.);
#12027=ORIENTED_EDGE('',*,*,#9299,.F.);
#12028=ORIENTED_EDGE('',*,*,#9300,.T.);
#12029=ORIENTED_EDGE('',*,*,#9296,.T.);
#12030=ORIENTED_EDGE('',*,*,#9301,.F.);
#12031=ORIENTED_EDGE('',*,*,#9302,.F.);
#12032=ORIENTED_EDGE('',*,*,#9303,.T.);
#12033=ORIENTED_EDGE('',*,*,#9299,.T.);
#12034=ORIENTED_EDGE('',*,*,#9304,.F.);
#12035=ORIENTED_EDGE('',*,*,#9305,.F.);
#12036=ORIENTED_EDGE('',*,*,#9306,.T.);
#12037=ORIENTED_EDGE('',*,*,#9302,.T.);
#12038=ORIENTED_EDGE('',*,*,#9307,.F.);
#12039=ORIENTED_EDGE('',*,*,#9308,.T.);
#12040=ORIENTED_EDGE('',*,*,#9309,.T.);
#12041=ORIENTED_EDGE('',*,*,#9310,.T.);
#12042=ORIENTED_EDGE('',*,*,#9311,.T.);
#12043=ORIENTED_EDGE('',*,*,#9309,.F.);
#12044=ORIENTED_EDGE('',*,*,#9310,.F.);
#12045=ORIENTED_EDGE('',*,*,#9311,.F.);
#12046=ORIENTED_EDGE('',*,*,#9312,.T.);
#12047=ORIENTED_EDGE('',*,*,#9313,.T.);
#12048=ORIENTED_EDGE('',*,*,#9312,.F.);
#12049=ORIENTED_EDGE('',*,*,#9308,.F.);
#12050=ORIENTED_EDGE('',*,*,#9314,.F.);
#12051=ORIENTED_EDGE('',*,*,#9315,.T.);
#12052=ORIENTED_EDGE('',*,*,#9316,.T.);
#12053=ORIENTED_EDGE('',*,*,#9317,.T.);
#12054=ORIENTED_EDGE('',*,*,#9318,.T.);
#12055=ORIENTED_EDGE('',*,*,#9319,.T.);
#12056=ORIENTED_EDGE('',*,*,#9316,.F.);
#12057=ORIENTED_EDGE('',*,*,#9320,.F.);
#12058=ORIENTED_EDGE('',*,*,#9321,.T.);
#12059=ORIENTED_EDGE('',*,*,#9322,.F.);
#12060=ORIENTED_EDGE('',*,*,#9315,.F.);
#12061=ORIENTED_EDGE('',*,*,#9323,.F.);
#12062=ORIENTED_EDGE('',*,*,#9324,.T.);
#12063=ORIENTED_EDGE('',*,*,#9325,.T.);
#12064=ORIENTED_EDGE('',*,*,#9320,.T.);
#12065=ORIENTED_EDGE('',*,*,#9319,.F.);
#12066=ORIENTED_EDGE('',*,*,#9326,.T.);
#12067=ORIENTED_EDGE('',*,*,#9327,.F.);
#12068=ORIENTED_EDGE('',*,*,#9328,.T.);
#12069=ORIENTED_EDGE('',*,*,#9323,.T.);
#12070=ORIENTED_EDGE('',*,*,#9329,.T.);
#12071=ORIENTED_EDGE('',*,*,#9330,.T.);
#12072=ORIENTED_EDGE('',*,*,#9331,.T.);
#12073=ORIENTED_EDGE('',*,*,#9332,.T.);
#12074=ORIENTED_EDGE('',*,*,#9333,.T.);
#12075=ORIENTED_EDGE('',*,*,#9330,.F.);
#12076=ORIENTED_EDGE('',*,*,#9334,.F.);
#12077=ORIENTED_EDGE('',*,*,#9335,.T.);
#12078=ORIENTED_EDGE('',*,*,#9336,.F.);
#12079=ORIENTED_EDGE('',*,*,#9329,.F.);
#12080=ORIENTED_EDGE('',*,*,#9337,.F.);
#12081=ORIENTED_EDGE('',*,*,#9338,.T.);
#12082=ORIENTED_EDGE('',*,*,#9339,.T.);
#12083=ORIENTED_EDGE('',*,*,#9334,.T.);
#12084=ORIENTED_EDGE('',*,*,#9333,.F.);
#12085=ORIENTED_EDGE('',*,*,#9340,.T.);
#12086=ORIENTED_EDGE('',*,*,#9325,.F.);
#12087=ORIENTED_EDGE('',*,*,#9341,.T.);
#12088=ORIENTED_EDGE('',*,*,#9337,.T.);
#12089=ORIENTED_EDGE('',*,*,#9342,.T.);
#12090=ORIENTED_EDGE('',*,*,#9343,.T.);
#12091=ORIENTED_EDGE('',*,*,#9344,.T.);
#12092=ORIENTED_EDGE('',*,*,#9345,.T.);
#12093=ORIENTED_EDGE('',*,*,#9346,.T.);
#12094=ORIENTED_EDGE('',*,*,#9343,.F.);
#12095=ORIENTED_EDGE('',*,*,#9347,.F.);
#12096=ORIENTED_EDGE('',*,*,#9348,.T.);
#12097=ORIENTED_EDGE('',*,*,#9349,.F.);
#12098=ORIENTED_EDGE('',*,*,#9342,.F.);
#12099=ORIENTED_EDGE('',*,*,#9350,.F.);
#12100=ORIENTED_EDGE('',*,*,#9351,.T.);
#12101=ORIENTED_EDGE('',*,*,#9352,.T.);
#12102=ORIENTED_EDGE('',*,*,#9347,.T.);
#12103=ORIENTED_EDGE('',*,*,#9346,.F.);
#12104=ORIENTED_EDGE('',*,*,#9353,.T.);
#12105=ORIENTED_EDGE('',*,*,#9339,.F.);
#12106=ORIENTED_EDGE('',*,*,#9354,.T.);
#12107=ORIENTED_EDGE('',*,*,#9350,.T.);
#12108=ORIENTED_EDGE('',*,*,#9355,.T.);
#12109=ORIENTED_EDGE('',*,*,#9356,.T.);
#12110=ORIENTED_EDGE('',*,*,#9357,.T.);
#12111=ORIENTED_EDGE('',*,*,#9358,.T.);
#12112=ORIENTED_EDGE('',*,*,#9359,.T.);
#12113=ORIENTED_EDGE('',*,*,#9356,.F.);
#12114=ORIENTED_EDGE('',*,*,#9360,.F.);
#12115=ORIENTED_EDGE('',*,*,#9361,.T.);
#12116=ORIENTED_EDGE('',*,*,#9362,.F.);
#12117=ORIENTED_EDGE('',*,*,#9355,.F.);
#12118=ORIENTED_EDGE('',*,*,#9363,.F.);
#12119=ORIENTED_EDGE('',*,*,#9364,.T.);
#12120=ORIENTED_EDGE('',*,*,#9365,.T.);
#12121=ORIENTED_EDGE('',*,*,#9360,.T.);
#12122=ORIENTED_EDGE('',*,*,#9359,.F.);
#12123=ORIENTED_EDGE('',*,*,#9366,.T.);
#12124=ORIENTED_EDGE('',*,*,#9352,.F.);
#12125=ORIENTED_EDGE('',*,*,#9367,.T.);
#12126=ORIENTED_EDGE('',*,*,#9363,.T.);
#12127=ORIENTED_EDGE('',*,*,#9368,.T.);
#12128=ORIENTED_EDGE('',*,*,#9369,.T.);
#12129=ORIENTED_EDGE('',*,*,#9370,.T.);
#12130=ORIENTED_EDGE('',*,*,#9371,.T.);
#12131=ORIENTED_EDGE('',*,*,#9372,.T.);
#12132=ORIENTED_EDGE('',*,*,#9369,.F.);
#12133=ORIENTED_EDGE('',*,*,#9373,.F.);
#12134=ORIENTED_EDGE('',*,*,#9374,.T.);
#12135=ORIENTED_EDGE('',*,*,#9375,.F.);
#12136=ORIENTED_EDGE('',*,*,#9368,.F.);
#12137=ORIENTED_EDGE('',*,*,#9376,.F.);
#12138=ORIENTED_EDGE('',*,*,#9377,.T.);
#12139=ORIENTED_EDGE('',*,*,#9378,.T.);
#12140=ORIENTED_EDGE('',*,*,#9373,.T.);
#12141=ORIENTED_EDGE('',*,*,#9372,.F.);
#12142=ORIENTED_EDGE('',*,*,#9379,.T.);
#12143=ORIENTED_EDGE('',*,*,#9365,.F.);
#12144=ORIENTED_EDGE('',*,*,#9380,.T.);
#12145=ORIENTED_EDGE('',*,*,#9376,.T.);
#12146=ORIENTED_EDGE('',*,*,#9381,.T.);
#12147=ORIENTED_EDGE('',*,*,#9382,.T.);
#12148=ORIENTED_EDGE('',*,*,#9383,.T.);
#12149=ORIENTED_EDGE('',*,*,#9384,.T.);
#12150=ORIENTED_EDGE('',*,*,#9385,.T.);
#12151=ORIENTED_EDGE('',*,*,#9382,.F.);
#12152=ORIENTED_EDGE('',*,*,#9386,.F.);
#12153=ORIENTED_EDGE('',*,*,#9387,.T.);
#12154=ORIENTED_EDGE('',*,*,#9388,.F.);
#12155=ORIENTED_EDGE('',*,*,#9381,.F.);
#12156=ORIENTED_EDGE('',*,*,#9389,.F.);
#12157=ORIENTED_EDGE('',*,*,#9390,.T.);
#12158=ORIENTED_EDGE('',*,*,#9327,.T.);
#12159=ORIENTED_EDGE('',*,*,#9386,.T.);
#12160=ORIENTED_EDGE('',*,*,#9385,.F.);
#12161=ORIENTED_EDGE('',*,*,#9391,.T.);
#12162=ORIENTED_EDGE('',*,*,#9392,.T.);
#12163=ORIENTED_EDGE('',*,*,#9393,.T.);
#12164=ORIENTED_EDGE('',*,*,#9389,.T.);
#12165=ORIENTED_EDGE('',*,*,#9394,.T.);
#12166=ORIENTED_EDGE('',*,*,#9395,.T.);
#12167=ORIENTED_EDGE('',*,*,#9396,.T.);
#12168=ORIENTED_EDGE('',*,*,#9397,.T.);
#12169=ORIENTED_EDGE('',*,*,#9398,.T.);
#12170=ORIENTED_EDGE('',*,*,#9395,.F.);
#12171=ORIENTED_EDGE('',*,*,#9399,.F.);
#12172=ORIENTED_EDGE('',*,*,#9400,.T.);
#12173=ORIENTED_EDGE('',*,*,#9401,.F.);
#12174=ORIENTED_EDGE('',*,*,#9394,.F.);
#12175=ORIENTED_EDGE('',*,*,#9402,.F.);
#12176=ORIENTED_EDGE('',*,*,#9403,.T.);
#12177=ORIENTED_EDGE('',*,*,#9392,.F.);
#12178=ORIENTED_EDGE('',*,*,#9399,.T.);
#12179=ORIENTED_EDGE('',*,*,#9404,.T.);
#12180=ORIENTED_EDGE('',*,*,#9405,.T.);
#12181=ORIENTED_EDGE('',*,*,#9406,.T.);
#12182=ORIENTED_EDGE('',*,*,#9407,.T.);
#12183=ORIENTED_EDGE('',*,*,#9408,.T.);
#12184=ORIENTED_EDGE('',*,*,#9405,.F.);
#12185=ORIENTED_EDGE('',*,*,#9409,.F.);
#12186=ORIENTED_EDGE('',*,*,#9410,.T.);
#12187=ORIENTED_EDGE('',*,*,#9411,.F.);
#12188=ORIENTED_EDGE('',*,*,#9404,.F.);
#12189=ORIENTED_EDGE('',*,*,#9412,.F.);
#12190=ORIENTED_EDGE('',*,*,#9413,.T.);
#12191=ORIENTED_EDGE('',*,*,#9414,.T.);
#12192=ORIENTED_EDGE('',*,*,#9409,.T.);
#12193=ORIENTED_EDGE('',*,*,#9408,.F.);
#12194=ORIENTED_EDGE('',*,*,#9415,.T.);
#12195=ORIENTED_EDGE('',*,*,#9416,.F.);
#12196=ORIENTED_EDGE('',*,*,#9417,.T.);
#12197=ORIENTED_EDGE('',*,*,#9412,.T.);
#12198=ORIENTED_EDGE('',*,*,#9418,.T.);
#12199=ORIENTED_EDGE('',*,*,#9419,.T.);
#12200=ORIENTED_EDGE('',*,*,#9420,.T.);
#12201=ORIENTED_EDGE('',*,*,#9421,.T.);
#12202=ORIENTED_EDGE('',*,*,#9422,.T.);
#12203=ORIENTED_EDGE('',*,*,#9419,.F.);
#12204=ORIENTED_EDGE('',*,*,#9423,.F.);
#12205=ORIENTED_EDGE('',*,*,#9424,.T.);
#12206=ORIENTED_EDGE('',*,*,#9425,.F.);
#12207=ORIENTED_EDGE('',*,*,#9418,.F.);
#12208=ORIENTED_EDGE('',*,*,#9426,.F.);
#12209=ORIENTED_EDGE('',*,*,#9427,.T.);
#12210=ORIENTED_EDGE('',*,*,#9416,.T.);
#12211=ORIENTED_EDGE('',*,*,#9423,.T.);
#12212=ORIENTED_EDGE('',*,*,#9422,.F.);
#12213=ORIENTED_EDGE('',*,*,#9428,.T.);
#12214=ORIENTED_EDGE('',*,*,#9429,.F.);
#12215=ORIENTED_EDGE('',*,*,#9430,.T.);
#12216=ORIENTED_EDGE('',*,*,#9426,.T.);
#12217=ORIENTED_EDGE('',*,*,#9431,.T.);
#12218=ORIENTED_EDGE('',*,*,#9432,.T.);
#12219=ORIENTED_EDGE('',*,*,#9433,.T.);
#12220=ORIENTED_EDGE('',*,*,#9434,.T.);
#12221=ORIENTED_EDGE('',*,*,#9435,.T.);
#12222=ORIENTED_EDGE('',*,*,#9432,.F.);
#12223=ORIENTED_EDGE('',*,*,#9436,.F.);
#12224=ORIENTED_EDGE('',*,*,#9437,.T.);
#12225=ORIENTED_EDGE('',*,*,#9438,.F.);
#12226=ORIENTED_EDGE('',*,*,#9431,.F.);
#12227=ORIENTED_EDGE('',*,*,#9439,.F.);
#12228=ORIENTED_EDGE('',*,*,#9440,.T.);
#12229=ORIENTED_EDGE('',*,*,#9429,.T.);
#12230=ORIENTED_EDGE('',*,*,#9436,.T.);
#12231=ORIENTED_EDGE('',*,*,#9435,.F.);
#12232=ORIENTED_EDGE('',*,*,#9441,.T.);
#12233=ORIENTED_EDGE('',*,*,#9442,.F.);
#12234=ORIENTED_EDGE('',*,*,#9443,.T.);
#12235=ORIENTED_EDGE('',*,*,#9439,.T.);
#12236=ORIENTED_EDGE('',*,*,#9444,.T.);
#12237=ORIENTED_EDGE('',*,*,#9445,.T.);
#12238=ORIENTED_EDGE('',*,*,#9446,.T.);
#12239=ORIENTED_EDGE('',*,*,#9447,.T.);
#12240=ORIENTED_EDGE('',*,*,#9448,.T.);
#12241=ORIENTED_EDGE('',*,*,#9445,.F.);
#12242=ORIENTED_EDGE('',*,*,#9449,.F.);
#12243=ORIENTED_EDGE('',*,*,#9450,.T.);
#12244=ORIENTED_EDGE('',*,*,#9451,.F.);
#12245=ORIENTED_EDGE('',*,*,#9444,.F.);
#12246=ORIENTED_EDGE('',*,*,#9452,.F.);
#12247=ORIENTED_EDGE('',*,*,#9453,.T.);
#12248=ORIENTED_EDGE('',*,*,#9442,.T.);
#12249=ORIENTED_EDGE('',*,*,#9449,.T.);
#12250=ORIENTED_EDGE('',*,*,#9448,.F.);
#12251=ORIENTED_EDGE('',*,*,#9454,.T.);
#12252=ORIENTED_EDGE('',*,*,#9455,.F.);
#12253=ORIENTED_EDGE('',*,*,#9456,.T.);
#12254=ORIENTED_EDGE('',*,*,#9452,.T.);
#12255=ORIENTED_EDGE('',*,*,#9457,.T.);
#12256=ORIENTED_EDGE('',*,*,#9458,.T.);
#12257=ORIENTED_EDGE('',*,*,#9459,.T.);
#12258=ORIENTED_EDGE('',*,*,#9460,.T.);
#12259=ORIENTED_EDGE('',*,*,#9461,.T.);
#12260=ORIENTED_EDGE('',*,*,#9458,.F.);
#12261=ORIENTED_EDGE('',*,*,#9462,.F.);
#12262=ORIENTED_EDGE('',*,*,#9463,.T.);
#12263=ORIENTED_EDGE('',*,*,#9464,.F.);
#12264=ORIENTED_EDGE('',*,*,#9457,.F.);
#12265=ORIENTED_EDGE('',*,*,#9465,.F.);
#12266=ORIENTED_EDGE('',*,*,#9466,.T.);
#12267=ORIENTED_EDGE('',*,*,#9455,.T.);
#12268=ORIENTED_EDGE('',*,*,#9462,.T.);
#12269=ORIENTED_EDGE('',*,*,#9461,.F.);
#12270=ORIENTED_EDGE('',*,*,#9467,.T.);
#12271=ORIENTED_EDGE('',*,*,#9378,.F.);
#12272=ORIENTED_EDGE('',*,*,#9468,.T.);
#12273=ORIENTED_EDGE('',*,*,#9465,.T.);
#12274=ORIENTED_EDGE('',*,*,#9469,.T.);
#12275=ORIENTED_EDGE('',*,*,#9470,.T.);
#12276=ORIENTED_EDGE('',*,*,#9471,.T.);
#12277=ORIENTED_EDGE('',*,*,#9472,.T.);
#12278=ORIENTED_EDGE('',*,*,#9472,.F.);
#12279=ORIENTED_EDGE('',*,*,#9473,.T.);
#12280=ORIENTED_EDGE('',*,*,#9474,.T.);
#12281=ORIENTED_EDGE('',*,*,#9475,.T.);
#12282=ORIENTED_EDGE('',*,*,#9471,.F.);
#12283=ORIENTED_EDGE('',*,*,#9476,.F.);
#12284=ORIENTED_EDGE('',*,*,#9477,.F.);
#12285=ORIENTED_EDGE('',*,*,#9478,.F.);
#12286=ORIENTED_EDGE('',*,*,#9479,.F.);
#12287=ORIENTED_EDGE('',*,*,#9258,.F.);
#12288=ORIENTED_EDGE('',*,*,#9480,.F.);
#12289=ORIENTED_EDGE('',*,*,#9481,.F.);
#12290=ORIENTED_EDGE('',*,*,#9482,.F.);
#12291=ORIENTED_EDGE('',*,*,#9473,.F.);
#12292=ORIENTED_EDGE('',*,*,#9483,.T.);
#12293=ORIENTED_EDGE('',*,*,#9484,.T.);
#12294=ORIENTED_EDGE('',*,*,#9485,.T.);
#12295=ORIENTED_EDGE('',*,*,#9486,.T.);
#12296=ORIENTED_EDGE('',*,*,#9486,.F.);
#12297=ORIENTED_EDGE('',*,*,#9487,.T.);
#12298=ORIENTED_EDGE('',*,*,#9488,.T.);
#12299=ORIENTED_EDGE('',*,*,#9489,.T.);
#12300=ORIENTED_EDGE('',*,*,#9485,.F.);
#12301=ORIENTED_EDGE('',*,*,#9490,.F.);
#12302=ORIENTED_EDGE('',*,*,#9491,.F.);
#12303=ORIENTED_EDGE('',*,*,#9492,.F.);
#12304=ORIENTED_EDGE('',*,*,#9250,.F.);
#12305=ORIENTED_EDGE('',*,*,#9493,.F.);
#12306=ORIENTED_EDGE('',*,*,#9494,.F.);
#12307=ORIENTED_EDGE('',*,*,#9495,.F.);
#12308=ORIENTED_EDGE('',*,*,#9487,.F.);
#12309=ORIENTED_EDGE('',*,*,#9496,.T.);
#12310=ORIENTED_EDGE('',*,*,#9497,.T.);
#12311=ORIENTED_EDGE('',*,*,#9498,.T.);
#12312=ORIENTED_EDGE('',*,*,#9499,.T.);
#12313=ORIENTED_EDGE('',*,*,#9499,.F.);
#12314=ORIENTED_EDGE('',*,*,#9500,.T.);
#12315=ORIENTED_EDGE('',*,*,#9501,.T.);
#12316=ORIENTED_EDGE('',*,*,#9502,.T.);
#12317=ORIENTED_EDGE('',*,*,#9498,.F.);
#12318=ORIENTED_EDGE('',*,*,#9503,.F.);
#12319=ORIENTED_EDGE('',*,*,#9504,.F.);
#12320=ORIENTED_EDGE('',*,*,#9505,.F.);
#12321=ORIENTED_EDGE('',*,*,#9242,.F.);
#12322=ORIENTED_EDGE('',*,*,#9506,.F.);
#12323=ORIENTED_EDGE('',*,*,#9507,.F.);
#12324=ORIENTED_EDGE('',*,*,#9508,.F.);
#12325=ORIENTED_EDGE('',*,*,#9500,.F.);
#12326=ORIENTED_EDGE('',*,*,#9509,.T.);
#12327=ORIENTED_EDGE('',*,*,#9510,.T.);
#12328=ORIENTED_EDGE('',*,*,#9511,.T.);
#12329=ORIENTED_EDGE('',*,*,#9512,.T.);
#12330=ORIENTED_EDGE('',*,*,#9512,.F.);
#12331=ORIENTED_EDGE('',*,*,#9513,.T.);
#12332=ORIENTED_EDGE('',*,*,#9514,.T.);
#12333=ORIENTED_EDGE('',*,*,#9515,.T.);
#12334=ORIENTED_EDGE('',*,*,#9511,.F.);
#12335=ORIENTED_EDGE('',*,*,#9516,.F.);
#12336=ORIENTED_EDGE('',*,*,#9517,.F.);
#12337=ORIENTED_EDGE('',*,*,#9518,.F.);
#12338=ORIENTED_EDGE('',*,*,#9234,.F.);
#12339=ORIENTED_EDGE('',*,*,#9519,.F.);
#12340=ORIENTED_EDGE('',*,*,#9520,.F.);
#12341=ORIENTED_EDGE('',*,*,#9521,.F.);
#12342=ORIENTED_EDGE('',*,*,#9513,.F.);
#12343=ORIENTED_EDGE('',*,*,#9522,.T.);
#12344=ORIENTED_EDGE('',*,*,#9523,.T.);
#12345=ORIENTED_EDGE('',*,*,#9524,.T.);
#12346=ORIENTED_EDGE('',*,*,#9525,.T.);
#12347=ORIENTED_EDGE('',*,*,#9525,.F.);
#12348=ORIENTED_EDGE('',*,*,#9526,.T.);
#12349=ORIENTED_EDGE('',*,*,#9527,.T.);
#12350=ORIENTED_EDGE('',*,*,#9528,.T.);
#12351=ORIENTED_EDGE('',*,*,#9524,.F.);
#12352=ORIENTED_EDGE('',*,*,#9529,.F.);
#12353=ORIENTED_EDGE('',*,*,#9530,.F.);
#12354=ORIENTED_EDGE('',*,*,#9531,.F.);
#12355=ORIENTED_EDGE('',*,*,#9226,.F.);
#12356=ORIENTED_EDGE('',*,*,#9532,.F.);
#12357=ORIENTED_EDGE('',*,*,#9533,.F.);
#12358=ORIENTED_EDGE('',*,*,#9534,.F.);
#12359=ORIENTED_EDGE('',*,*,#9526,.F.);
#12360=ORIENTED_EDGE('',*,*,#9535,.T.);
#12361=ORIENTED_EDGE('',*,*,#9536,.T.);
#12362=ORIENTED_EDGE('',*,*,#9537,.T.);
#12363=ORIENTED_EDGE('',*,*,#9538,.T.);
#12364=ORIENTED_EDGE('',*,*,#9538,.F.);
#12365=ORIENTED_EDGE('',*,*,#9539,.T.);
#12366=ORIENTED_EDGE('',*,*,#9540,.T.);
#12367=ORIENTED_EDGE('',*,*,#9541,.T.);
#12368=ORIENTED_EDGE('',*,*,#9537,.F.);
#12369=ORIENTED_EDGE('',*,*,#9542,.F.);
#12370=ORIENTED_EDGE('',*,*,#9543,.F.);
#12371=ORIENTED_EDGE('',*,*,#9544,.F.);
#12372=ORIENTED_EDGE('',*,*,#9218,.F.);
#12373=ORIENTED_EDGE('',*,*,#9545,.F.);
#12374=ORIENTED_EDGE('',*,*,#9546,.F.);
#12375=ORIENTED_EDGE('',*,*,#9547,.F.);
#12376=ORIENTED_EDGE('',*,*,#9539,.F.);
#12377=ORIENTED_EDGE('',*,*,#9548,.T.);
#12378=ORIENTED_EDGE('',*,*,#9549,.T.);
#12379=ORIENTED_EDGE('',*,*,#9550,.T.);
#12380=ORIENTED_EDGE('',*,*,#9551,.T.);
#12381=ORIENTED_EDGE('',*,*,#9551,.F.);
#12382=ORIENTED_EDGE('',*,*,#9552,.T.);
#12383=ORIENTED_EDGE('',*,*,#9553,.T.);
#12384=ORIENTED_EDGE('',*,*,#9554,.T.);
#12385=ORIENTED_EDGE('',*,*,#9550,.F.);
#12386=ORIENTED_EDGE('',*,*,#9555,.F.);
#12387=ORIENTED_EDGE('',*,*,#9556,.F.);
#12388=ORIENTED_EDGE('',*,*,#9557,.F.);
#12389=ORIENTED_EDGE('',*,*,#9210,.F.);
#12390=ORIENTED_EDGE('',*,*,#9558,.F.);
#12391=ORIENTED_EDGE('',*,*,#9559,.F.);
#12392=ORIENTED_EDGE('',*,*,#9560,.F.);
#12393=ORIENTED_EDGE('',*,*,#9552,.F.);
#12394=ORIENTED_EDGE('',*,*,#9561,.T.);
#12395=ORIENTED_EDGE('',*,*,#9562,.T.);
#12396=ORIENTED_EDGE('',*,*,#9563,.T.);
#12397=ORIENTED_EDGE('',*,*,#9564,.T.);
#12398=ORIENTED_EDGE('',*,*,#9564,.F.);
#12399=ORIENTED_EDGE('',*,*,#9565,.T.);
#12400=ORIENTED_EDGE('',*,*,#9566,.T.);
#12401=ORIENTED_EDGE('',*,*,#9567,.T.);
#12402=ORIENTED_EDGE('',*,*,#9563,.F.);
#12403=ORIENTED_EDGE('',*,*,#9568,.F.);
#12404=ORIENTED_EDGE('',*,*,#9569,.F.);
#12405=ORIENTED_EDGE('',*,*,#9570,.F.);
#12406=ORIENTED_EDGE('',*,*,#9202,.F.);
#12407=ORIENTED_EDGE('',*,*,#9571,.F.);
#12408=ORIENTED_EDGE('',*,*,#9572,.F.);
#12409=ORIENTED_EDGE('',*,*,#9573,.F.);
#12410=ORIENTED_EDGE('',*,*,#9565,.F.);
#12411=ORIENTED_EDGE('',*,*,#9574,.T.);
#12412=ORIENTED_EDGE('',*,*,#9575,.T.);
#12413=ORIENTED_EDGE('',*,*,#9576,.T.);
#12414=ORIENTED_EDGE('',*,*,#9577,.T.);
#12415=ORIENTED_EDGE('',*,*,#9577,.F.);
#12416=ORIENTED_EDGE('',*,*,#9578,.T.);
#12417=ORIENTED_EDGE('',*,*,#9579,.T.);
#12418=ORIENTED_EDGE('',*,*,#9580,.T.);
#12419=ORIENTED_EDGE('',*,*,#9576,.F.);
#12420=ORIENTED_EDGE('',*,*,#9581,.F.);
#12421=ORIENTED_EDGE('',*,*,#9582,.F.);
#12422=ORIENTED_EDGE('',*,*,#9583,.F.);
#12423=ORIENTED_EDGE('',*,*,#9194,.F.);
#12424=ORIENTED_EDGE('',*,*,#9584,.F.);
#12425=ORIENTED_EDGE('',*,*,#9585,.F.);
#12426=ORIENTED_EDGE('',*,*,#9586,.F.);
#12427=ORIENTED_EDGE('',*,*,#9578,.F.);
#12428=ORIENTED_EDGE('',*,*,#9587,.T.);
#12429=ORIENTED_EDGE('',*,*,#9588,.T.);
#12430=ORIENTED_EDGE('',*,*,#9589,.T.);
#12431=ORIENTED_EDGE('',*,*,#9590,.T.);
#12432=ORIENTED_EDGE('',*,*,#9590,.F.);
#12433=ORIENTED_EDGE('',*,*,#9591,.T.);
#12434=ORIENTED_EDGE('',*,*,#9592,.T.);
#12435=ORIENTED_EDGE('',*,*,#9593,.T.);
#12436=ORIENTED_EDGE('',*,*,#9589,.F.);
#12437=ORIENTED_EDGE('',*,*,#9594,.F.);
#12438=ORIENTED_EDGE('',*,*,#9595,.F.);
#12439=ORIENTED_EDGE('',*,*,#9596,.F.);
#12440=ORIENTED_EDGE('',*,*,#9186,.F.);
#12441=ORIENTED_EDGE('',*,*,#9597,.F.);
#12442=ORIENTED_EDGE('',*,*,#9598,.F.);
#12443=ORIENTED_EDGE('',*,*,#9599,.F.);
#12444=ORIENTED_EDGE('',*,*,#9591,.F.);
#12445=ORIENTED_EDGE('',*,*,#9600,.T.);
#12446=ORIENTED_EDGE('',*,*,#9601,.T.);
#12447=ORIENTED_EDGE('',*,*,#9602,.T.);
#12448=ORIENTED_EDGE('',*,*,#9603,.T.);
#12449=ORIENTED_EDGE('',*,*,#9603,.F.);
#12450=ORIENTED_EDGE('',*,*,#9604,.T.);
#12451=ORIENTED_EDGE('',*,*,#9605,.T.);
#12452=ORIENTED_EDGE('',*,*,#9606,.T.);
#12453=ORIENTED_EDGE('',*,*,#9602,.F.);
#12454=ORIENTED_EDGE('',*,*,#9607,.F.);
#12455=ORIENTED_EDGE('',*,*,#9608,.F.);
#12456=ORIENTED_EDGE('',*,*,#9609,.F.);
#12457=ORIENTED_EDGE('',*,*,#9178,.F.);
#12458=ORIENTED_EDGE('',*,*,#9610,.F.);
#12459=ORIENTED_EDGE('',*,*,#9611,.F.);
#12460=ORIENTED_EDGE('',*,*,#9612,.F.);
#12461=ORIENTED_EDGE('',*,*,#9604,.F.);
#12462=ORIENTED_EDGE('',*,*,#9613,.T.);
#12463=ORIENTED_EDGE('',*,*,#9614,.T.);
#12464=ORIENTED_EDGE('',*,*,#9615,.T.);
#12465=ORIENTED_EDGE('',*,*,#9616,.T.);
#12466=ORIENTED_EDGE('',*,*,#9616,.F.);
#12467=ORIENTED_EDGE('',*,*,#9617,.T.);
#12468=ORIENTED_EDGE('',*,*,#9618,.T.);
#12469=ORIENTED_EDGE('',*,*,#9619,.T.);
#12470=ORIENTED_EDGE('',*,*,#9615,.F.);
#12471=ORIENTED_EDGE('',*,*,#9620,.F.);
#12472=ORIENTED_EDGE('',*,*,#9621,.F.);
#12473=ORIENTED_EDGE('',*,*,#9622,.F.);
#12474=ORIENTED_EDGE('',*,*,#9170,.F.);
#12475=ORIENTED_EDGE('',*,*,#9167,.F.);
#12476=ORIENTED_EDGE('',*,*,#9623,.F.);
#12477=ORIENTED_EDGE('',*,*,#9624,.F.);
#12478=ORIENTED_EDGE('',*,*,#9625,.F.);
#12479=ORIENTED_EDGE('',*,*,#9617,.F.);
#12480=ORIENTED_EDGE('',*,*,#9626,.T.);
#12481=ORIENTED_EDGE('',*,*,#9627,.T.);
#12482=ORIENTED_EDGE('',*,*,#9628,.T.);
#12483=ORIENTED_EDGE('',*,*,#9627,.F.);
#12484=ORIENTED_EDGE('',*,*,#9628,.F.);
#12485=ORIENTED_EDGE('',*,*,#9629,.T.);
#12486=ORIENTED_EDGE('',*,*,#9630,.T.);
#12487=ORIENTED_EDGE('',*,*,#9631,.T.);
#12488=ORIENTED_EDGE('',*,*,#9626,.F.);
#12489=ORIENTED_EDGE('',*,*,#9631,.F.);
#12490=ORIENTED_EDGE('',*,*,#9632,.T.);
#12491=ORIENTED_EDGE('',*,*,#9633,.T.);
#12492=ORIENTED_EDGE('',*,*,#9634,.T.);
#12493=ORIENTED_EDGE('',*,*,#9633,.F.);
#12494=ORIENTED_EDGE('',*,*,#9634,.F.);
#12495=ORIENTED_EDGE('',*,*,#9635,.F.);
#12496=ORIENTED_EDGE('',*,*,#9632,.F.);
#12497=ORIENTED_EDGE('',*,*,#9636,.T.);
#12498=ORIENTED_EDGE('',*,*,#9637,.T.);
#12499=ORIENTED_EDGE('',*,*,#9636,.F.);
#12500=ORIENTED_EDGE('',*,*,#9638,.T.);
#12501=ORIENTED_EDGE('',*,*,#9639,.T.);
#12502=ORIENTED_EDGE('',*,*,#9640,.T.);
#12503=ORIENTED_EDGE('',*,*,#9641,.T.);
#12504=ORIENTED_EDGE('',*,*,#9642,.T.);
#12505=ORIENTED_EDGE('',*,*,#9641,.F.);
#12506=ORIENTED_EDGE('',*,*,#9643,.T.);
#12507=ORIENTED_EDGE('',*,*,#9644,.T.);
#12508=ORIENTED_EDGE('',*,*,#9645,.T.);
#12509=ORIENTED_EDGE('',*,*,#9646,.T.);
#12510=ORIENTED_EDGE('',*,*,#9647,.T.);
#12511=ORIENTED_EDGE('',*,*,#9640,.F.);
#12512=ORIENTED_EDGE('',*,*,#9648,.T.);
#12513=ORIENTED_EDGE('',*,*,#9649,.F.);
#12514=ORIENTED_EDGE('',*,*,#9650,.F.);
#12515=ORIENTED_EDGE('',*,*,#9651,.F.);
#12516=ORIENTED_EDGE('',*,*,#9643,.F.);
#12517=ORIENTED_EDGE('',*,*,#9639,.F.);
#12518=ORIENTED_EDGE('',*,*,#9652,.T.);
#12519=ORIENTED_EDGE('',*,*,#9491,.T.);
#12520=ORIENTED_EDGE('',*,*,#9653,.T.);
#12521=ORIENTED_EDGE('',*,*,#9654,.T.);
#12522=ORIENTED_EDGE('',*,*,#9655,.T.);
#12523=ORIENTED_EDGE('',*,*,#9656,.F.);
#12524=ORIENTED_EDGE('',*,*,#9648,.F.);
#12525=ORIENTED_EDGE('',*,*,#9649,.T.);
#12526=ORIENTED_EDGE('',*,*,#9656,.T.);
#12527=ORIENTED_EDGE('',*,*,#9657,.T.);
#12528=ORIENTED_EDGE('',*,*,#9658,.T.);
#12529=ORIENTED_EDGE('',*,*,#9659,.T.);
#12530=ORIENTED_EDGE('',*,*,#9659,.F.);
#12531=ORIENTED_EDGE('',*,*,#9660,.T.);
#12532=ORIENTED_EDGE('',*,*,#9661,.F.);
#12533=ORIENTED_EDGE('',*,*,#9662,.T.);
#12534=ORIENTED_EDGE('',*,*,#9663,.T.);
#12535=ORIENTED_EDGE('',*,*,#9650,.T.);
#12536=ORIENTED_EDGE('',*,*,#9664,.T.);
#12537=ORIENTED_EDGE('',*,*,#9665,.T.);
#12538=ORIENTED_EDGE('',*,*,#9666,.T.);
#12539=ORIENTED_EDGE('',*,*,#9661,.T.);
#12540=ORIENTED_EDGE('',*,*,#9667,.T.);
#12541=ORIENTED_EDGE('',*,*,#9666,.F.);
#12542=ORIENTED_EDGE('',*,*,#9668,.T.);
#12543=ORIENTED_EDGE('',*,*,#9669,.F.);
#12544=ORIENTED_EDGE('',*,*,#9670,.F.);
#12545=ORIENTED_EDGE('',*,*,#9671,.F.);
#12546=ORIENTED_EDGE('',*,*,#9662,.F.);
#12547=ORIENTED_EDGE('',*,*,#9665,.F.);
#12548=ORIENTED_EDGE('',*,*,#9672,.T.);
#12549=ORIENTED_EDGE('',*,*,#9504,.T.);
#12550=ORIENTED_EDGE('',*,*,#9673,.T.);
#12551=ORIENTED_EDGE('',*,*,#9674,.T.);
#12552=ORIENTED_EDGE('',*,*,#9675,.T.);
#12553=ORIENTED_EDGE('',*,*,#9676,.F.);
#12554=ORIENTED_EDGE('',*,*,#9668,.F.);
#12555=ORIENTED_EDGE('',*,*,#9669,.T.);
#12556=ORIENTED_EDGE('',*,*,#9676,.T.);
#12557=ORIENTED_EDGE('',*,*,#9677,.T.);
#12558=ORIENTED_EDGE('',*,*,#9678,.T.);
#12559=ORIENTED_EDGE('',*,*,#9679,.T.);
#12560=ORIENTED_EDGE('',*,*,#9679,.F.);
#12561=ORIENTED_EDGE('',*,*,#9680,.T.);
#12562=ORIENTED_EDGE('',*,*,#9681,.F.);
#12563=ORIENTED_EDGE('',*,*,#9682,.T.);
#12564=ORIENTED_EDGE('',*,*,#9683,.T.);
#12565=ORIENTED_EDGE('',*,*,#9670,.T.);
#12566=ORIENTED_EDGE('',*,*,#9684,.T.);
#12567=ORIENTED_EDGE('',*,*,#9685,.T.);
#12568=ORIENTED_EDGE('',*,*,#9686,.T.);
#12569=ORIENTED_EDGE('',*,*,#9681,.T.);
#12570=ORIENTED_EDGE('',*,*,#9687,.T.);
#12571=ORIENTED_EDGE('',*,*,#9686,.F.);
#12572=ORIENTED_EDGE('',*,*,#9688,.T.);
#12573=ORIENTED_EDGE('',*,*,#9689,.F.);
#12574=ORIENTED_EDGE('',*,*,#9690,.F.);
#12575=ORIENTED_EDGE('',*,*,#9691,.F.);
#12576=ORIENTED_EDGE('',*,*,#9682,.F.);
#12577=ORIENTED_EDGE('',*,*,#9685,.F.);
#12578=ORIENTED_EDGE('',*,*,#9692,.T.);
#12579=ORIENTED_EDGE('',*,*,#9517,.T.);
#12580=ORIENTED_EDGE('',*,*,#9693,.T.);
#12581=ORIENTED_EDGE('',*,*,#9694,.T.);
#12582=ORIENTED_EDGE('',*,*,#9695,.T.);
#12583=ORIENTED_EDGE('',*,*,#9696,.F.);
#12584=ORIENTED_EDGE('',*,*,#9688,.F.);
#12585=ORIENTED_EDGE('',*,*,#9689,.T.);
#12586=ORIENTED_EDGE('',*,*,#9696,.T.);
#12587=ORIENTED_EDGE('',*,*,#9697,.T.);
#12588=ORIENTED_EDGE('',*,*,#9698,.T.);
#12589=ORIENTED_EDGE('',*,*,#9699,.T.);
#12590=ORIENTED_EDGE('',*,*,#9699,.F.);
#12591=ORIENTED_EDGE('',*,*,#9700,.T.);
#12592=ORIENTED_EDGE('',*,*,#9701,.F.);
#12593=ORIENTED_EDGE('',*,*,#9702,.T.);
#12594=ORIENTED_EDGE('',*,*,#9703,.T.);
#12595=ORIENTED_EDGE('',*,*,#9690,.T.);
#12596=ORIENTED_EDGE('',*,*,#9704,.T.);
#12597=ORIENTED_EDGE('',*,*,#9705,.T.);
#12598=ORIENTED_EDGE('',*,*,#9706,.T.);
#12599=ORIENTED_EDGE('',*,*,#9701,.T.);
#12600=ORIENTED_EDGE('',*,*,#9707,.T.);
#12601=ORIENTED_EDGE('',*,*,#9706,.F.);
#12602=ORIENTED_EDGE('',*,*,#9708,.T.);
#12603=ORIENTED_EDGE('',*,*,#9709,.F.);
#12604=ORIENTED_EDGE('',*,*,#9710,.F.);
#12605=ORIENTED_EDGE('',*,*,#9711,.F.);
#12606=ORIENTED_EDGE('',*,*,#9702,.F.);
#12607=ORIENTED_EDGE('',*,*,#9705,.F.);
#12608=ORIENTED_EDGE('',*,*,#9712,.T.);
#12609=ORIENTED_EDGE('',*,*,#9530,.T.);
#12610=ORIENTED_EDGE('',*,*,#9713,.T.);
#12611=ORIENTED_EDGE('',*,*,#9714,.T.);
#12612=ORIENTED_EDGE('',*,*,#9715,.T.);
#12613=ORIENTED_EDGE('',*,*,#9716,.F.);
#12614=ORIENTED_EDGE('',*,*,#9708,.F.);
#12615=ORIENTED_EDGE('',*,*,#9709,.T.);
#12616=ORIENTED_EDGE('',*,*,#9716,.T.);
#12617=ORIENTED_EDGE('',*,*,#9717,.T.);
#12618=ORIENTED_EDGE('',*,*,#9718,.T.);
#12619=ORIENTED_EDGE('',*,*,#9719,.T.);
#12620=ORIENTED_EDGE('',*,*,#9719,.F.);
#12621=ORIENTED_EDGE('',*,*,#9720,.T.);
#12622=ORIENTED_EDGE('',*,*,#9721,.F.);
#12623=ORIENTED_EDGE('',*,*,#9722,.T.);
#12624=ORIENTED_EDGE('',*,*,#9723,.T.);
#12625=ORIENTED_EDGE('',*,*,#9710,.T.);
#12626=ORIENTED_EDGE('',*,*,#9724,.T.);
#12627=ORIENTED_EDGE('',*,*,#9725,.T.);
#12628=ORIENTED_EDGE('',*,*,#9726,.T.);
#12629=ORIENTED_EDGE('',*,*,#9721,.T.);
#12630=ORIENTED_EDGE('',*,*,#9727,.T.);
#12631=ORIENTED_EDGE('',*,*,#9726,.F.);
#12632=ORIENTED_EDGE('',*,*,#9728,.T.);
#12633=ORIENTED_EDGE('',*,*,#9729,.F.);
#12634=ORIENTED_EDGE('',*,*,#9730,.F.);
#12635=ORIENTED_EDGE('',*,*,#9731,.F.);
#12636=ORIENTED_EDGE('',*,*,#9722,.F.);
#12637=ORIENTED_EDGE('',*,*,#9725,.F.);
#12638=ORIENTED_EDGE('',*,*,#9732,.T.);
#12639=ORIENTED_EDGE('',*,*,#9543,.T.);
#12640=ORIENTED_EDGE('',*,*,#9733,.T.);
#12641=ORIENTED_EDGE('',*,*,#9734,.T.);
#12642=ORIENTED_EDGE('',*,*,#9735,.T.);
#12643=ORIENTED_EDGE('',*,*,#9736,.F.);
#12644=ORIENTED_EDGE('',*,*,#9728,.F.);
#12645=ORIENTED_EDGE('',*,*,#9729,.T.);
#12646=ORIENTED_EDGE('',*,*,#9736,.T.);
#12647=ORIENTED_EDGE('',*,*,#9737,.T.);
#12648=ORIENTED_EDGE('',*,*,#9738,.T.);
#12649=ORIENTED_EDGE('',*,*,#9739,.T.);
#12650=ORIENTED_EDGE('',*,*,#9739,.F.);
#12651=ORIENTED_EDGE('',*,*,#9740,.T.);
#12652=ORIENTED_EDGE('',*,*,#9741,.T.);
#12653=ORIENTED_EDGE('',*,*,#9742,.T.);
#12654=ORIENTED_EDGE('',*,*,#9743,.T.);
#12655=ORIENTED_EDGE('',*,*,#9730,.T.);
#12656=ORIENTED_EDGE('',*,*,#9743,.F.);
#12657=ORIENTED_EDGE('',*,*,#9744,.T.);
#12658=ORIENTED_EDGE('',*,*,#9745,.F.);
#12659=ORIENTED_EDGE('',*,*,#9746,.T.);
#12660=ORIENTED_EDGE('',*,*,#9747,.F.);
#12661=ORIENTED_EDGE('',*,*,#9748,.T.);
#12662=ORIENTED_EDGE('',*,*,#9749,.F.);
#12663=ORIENTED_EDGE('',*,*,#9750,.T.);
#12664=ORIENTED_EDGE('',*,*,#9751,.F.);
#12665=ORIENTED_EDGE('',*,*,#9752,.T.);
#12666=ORIENTED_EDGE('',*,*,#9753,.F.);
#12667=ORIENTED_EDGE('',*,*,#9754,.T.);
#12668=ORIENTED_EDGE('',*,*,#9755,.F.);
#12669=ORIENTED_EDGE('',*,*,#9756,.T.);
#12670=ORIENTED_EDGE('',*,*,#9644,.F.);
#12671=ORIENTED_EDGE('',*,*,#9651,.T.);
#12672=ORIENTED_EDGE('',*,*,#9663,.F.);
#12673=ORIENTED_EDGE('',*,*,#9671,.T.);
#12674=ORIENTED_EDGE('',*,*,#9683,.F.);
#12675=ORIENTED_EDGE('',*,*,#9691,.T.);
#12676=ORIENTED_EDGE('',*,*,#9703,.F.);
#12677=ORIENTED_EDGE('',*,*,#9711,.T.);
#12678=ORIENTED_EDGE('',*,*,#9723,.F.);
#12679=ORIENTED_EDGE('',*,*,#9731,.T.);
#12680=ORIENTED_EDGE('',*,*,#9757,.F.);
#12681=ORIENTED_EDGE('',*,*,#9742,.F.);
#12682=ORIENTED_EDGE('',*,*,#9758,.F.);
#12683=ORIENTED_EDGE('',*,*,#9759,.T.);
#12684=ORIENTED_EDGE('',*,*,#9760,.F.);
#12685=ORIENTED_EDGE('',*,*,#9761,.F.);
#12686=ORIENTED_EDGE('',*,*,#9744,.F.);
#12687=ORIENTED_EDGE('',*,*,#9741,.F.);
#12688=ORIENTED_EDGE('',*,*,#9762,.T.);
#12689=ORIENTED_EDGE('',*,*,#9763,.T.);
#12690=ORIENTED_EDGE('',*,*,#9764,.T.);
#12691=ORIENTED_EDGE('',*,*,#9758,.T.);
#12692=ORIENTED_EDGE('',*,*,#9658,.F.);
#12693=ORIENTED_EDGE('',*,*,#9765,.F.);
#12694=ORIENTED_EDGE('',*,*,#9246,.F.);
#12695=ORIENTED_EDGE('',*,*,#9766,.F.);
#12696=ORIENTED_EDGE('',*,*,#9244,.F.);
#12697=ORIENTED_EDGE('',*,*,#9767,.F.);
#12698=ORIENTED_EDGE('',*,*,#9667,.F.);
#12699=ORIENTED_EDGE('',*,*,#9660,.F.);
#12700=ORIENTED_EDGE('',*,*,#9642,.F.);
#12701=ORIENTED_EDGE('',*,*,#9647,.F.);
#12702=ORIENTED_EDGE('',*,*,#9768,.F.);
#12703=ORIENTED_EDGE('',*,*,#9769,.F.);
#12704=ORIENTED_EDGE('',*,*,#9254,.F.);
#12705=ORIENTED_EDGE('',*,*,#9770,.F.);
#12706=ORIENTED_EDGE('',*,*,#9252,.F.);
#12707=ORIENTED_EDGE('',*,*,#9771,.F.);
#12708=ORIENTED_EDGE('',*,*,#9646,.F.);
#12709=ORIENTED_EDGE('',*,*,#9772,.T.);
#12710=ORIENTED_EDGE('',*,*,#9773,.T.);
#12711=ORIENTED_EDGE('',*,*,#9774,.T.);
#12712=ORIENTED_EDGE('',*,*,#9768,.T.);
#12713=ORIENTED_EDGE('',*,*,#9764,.F.);
#12714=ORIENTED_EDGE('',*,*,#9775,.T.);
#12715=ORIENTED_EDGE('',*,*,#9556,.T.);
#12716=ORIENTED_EDGE('',*,*,#9776,.T.);
#12717=ORIENTED_EDGE('',*,*,#9777,.T.);
#12718=ORIENTED_EDGE('',*,*,#9778,.T.);
#12719=ORIENTED_EDGE('',*,*,#9779,.F.);
#12720=ORIENTED_EDGE('',*,*,#9759,.F.);
#12721=ORIENTED_EDGE('',*,*,#9760,.T.);
#12722=ORIENTED_EDGE('',*,*,#9779,.T.);
#12723=ORIENTED_EDGE('',*,*,#9780,.T.);
#12724=ORIENTED_EDGE('',*,*,#9781,.T.);
#12725=ORIENTED_EDGE('',*,*,#9782,.T.);
#12726=ORIENTED_EDGE('',*,*,#9782,.F.);
#12727=ORIENTED_EDGE('',*,*,#9783,.T.);
#12728=ORIENTED_EDGE('',*,*,#9784,.T.);
#12729=ORIENTED_EDGE('',*,*,#9785,.T.);
#12730=ORIENTED_EDGE('',*,*,#9745,.T.);
#12731=ORIENTED_EDGE('',*,*,#9761,.T.);
#12732=ORIENTED_EDGE('',*,*,#9785,.F.);
#12733=ORIENTED_EDGE('',*,*,#9786,.F.);
#12734=ORIENTED_EDGE('',*,*,#9787,.T.);
#12735=ORIENTED_EDGE('',*,*,#9788,.F.);
#12736=ORIENTED_EDGE('',*,*,#9789,.F.);
#12737=ORIENTED_EDGE('',*,*,#9746,.F.);
#12738=ORIENTED_EDGE('',*,*,#9784,.F.);
#12739=ORIENTED_EDGE('',*,*,#9790,.T.);
#12740=ORIENTED_EDGE('',*,*,#9791,.T.);
#12741=ORIENTED_EDGE('',*,*,#9792,.T.);
#12742=ORIENTED_EDGE('',*,*,#9786,.T.);
#12743=ORIENTED_EDGE('',*,*,#9792,.F.);
#12744=ORIENTED_EDGE('',*,*,#9793,.T.);
#12745=ORIENTED_EDGE('',*,*,#9569,.T.);
#12746=ORIENTED_EDGE('',*,*,#9794,.T.);
#12747=ORIENTED_EDGE('',*,*,#9795,.T.);
#12748=ORIENTED_EDGE('',*,*,#9796,.T.);
#12749=ORIENTED_EDGE('',*,*,#9797,.F.);
#12750=ORIENTED_EDGE('',*,*,#9787,.F.);
#12751=ORIENTED_EDGE('',*,*,#9788,.T.);
#12752=ORIENTED_EDGE('',*,*,#9797,.T.);
#12753=ORIENTED_EDGE('',*,*,#9798,.T.);
#12754=ORIENTED_EDGE('',*,*,#9799,.T.);
#12755=ORIENTED_EDGE('',*,*,#9800,.T.);
#12756=ORIENTED_EDGE('',*,*,#9800,.F.);
#12757=ORIENTED_EDGE('',*,*,#9801,.T.);
#12758=ORIENTED_EDGE('',*,*,#9802,.T.);
#12759=ORIENTED_EDGE('',*,*,#9803,.T.);
#12760=ORIENTED_EDGE('',*,*,#9747,.T.);
#12761=ORIENTED_EDGE('',*,*,#9789,.T.);
#12762=ORIENTED_EDGE('',*,*,#9803,.F.);
#12763=ORIENTED_EDGE('',*,*,#9804,.F.);
#12764=ORIENTED_EDGE('',*,*,#9805,.T.);
#12765=ORIENTED_EDGE('',*,*,#9806,.F.);
#12766=ORIENTED_EDGE('',*,*,#9807,.F.);
#12767=ORIENTED_EDGE('',*,*,#9748,.F.);
#12768=ORIENTED_EDGE('',*,*,#9802,.F.);
#12769=ORIENTED_EDGE('',*,*,#9808,.T.);
#12770=ORIENTED_EDGE('',*,*,#9809,.T.);
#12771=ORIENTED_EDGE('',*,*,#9810,.T.);
#12772=ORIENTED_EDGE('',*,*,#9804,.T.);
#12773=ORIENTED_EDGE('',*,*,#9810,.F.);
#12774=ORIENTED_EDGE('',*,*,#9811,.T.);
#12775=ORIENTED_EDGE('',*,*,#9582,.T.);
#12776=ORIENTED_EDGE('',*,*,#9812,.T.);
#12777=ORIENTED_EDGE('',*,*,#9813,.T.);
#12778=ORIENTED_EDGE('',*,*,#9814,.T.);
#12779=ORIENTED_EDGE('',*,*,#9815,.F.);
#12780=ORIENTED_EDGE('',*,*,#9805,.F.);
#12781=ORIENTED_EDGE('',*,*,#9806,.T.);
#12782=ORIENTED_EDGE('',*,*,#9815,.T.);
#12783=ORIENTED_EDGE('',*,*,#9816,.T.);
#12784=ORIENTED_EDGE('',*,*,#9817,.T.);
#12785=ORIENTED_EDGE('',*,*,#9818,.T.);
#12786=ORIENTED_EDGE('',*,*,#9818,.F.);
#12787=ORIENTED_EDGE('',*,*,#9819,.T.);
#12788=ORIENTED_EDGE('',*,*,#9820,.T.);
#12789=ORIENTED_EDGE('',*,*,#9821,.T.);
#12790=ORIENTED_EDGE('',*,*,#9749,.T.);
#12791=ORIENTED_EDGE('',*,*,#9807,.T.);
#12792=ORIENTED_EDGE('',*,*,#9821,.F.);
#12793=ORIENTED_EDGE('',*,*,#9822,.F.);
#12794=ORIENTED_EDGE('',*,*,#9823,.T.);
#12795=ORIENTED_EDGE('',*,*,#9824,.F.);
#12796=ORIENTED_EDGE('',*,*,#9825,.F.);
#12797=ORIENTED_EDGE('',*,*,#9750,.F.);
#12798=ORIENTED_EDGE('',*,*,#9820,.F.);
#12799=ORIENTED_EDGE('',*,*,#9826,.T.);
#12800=ORIENTED_EDGE('',*,*,#9827,.T.);
#12801=ORIENTED_EDGE('',*,*,#9828,.T.);
#12802=ORIENTED_EDGE('',*,*,#9822,.T.);
#12803=ORIENTED_EDGE('',*,*,#9828,.F.);
#12804=ORIENTED_EDGE('',*,*,#9829,.T.);
#12805=ORIENTED_EDGE('',*,*,#9595,.T.);
#12806=ORIENTED_EDGE('',*,*,#9830,.T.);
#12807=ORIENTED_EDGE('',*,*,#9831,.T.);
#12808=ORIENTED_EDGE('',*,*,#9832,.T.);
#12809=ORIENTED_EDGE('',*,*,#9833,.F.);
#12810=ORIENTED_EDGE('',*,*,#9823,.F.);
#12811=ORIENTED_EDGE('',*,*,#9824,.T.);
#12812=ORIENTED_EDGE('',*,*,#9833,.T.);
#12813=ORIENTED_EDGE('',*,*,#9834,.T.);
#12814=ORIENTED_EDGE('',*,*,#9835,.T.);
#12815=ORIENTED_EDGE('',*,*,#9836,.T.);
#12816=ORIENTED_EDGE('',*,*,#9836,.F.);
#12817=ORIENTED_EDGE('',*,*,#9837,.T.);
#12818=ORIENTED_EDGE('',*,*,#9838,.T.);
#12819=ORIENTED_EDGE('',*,*,#9839,.T.);
#12820=ORIENTED_EDGE('',*,*,#9751,.T.);
#12821=ORIENTED_EDGE('',*,*,#9825,.T.);
#12822=ORIENTED_EDGE('',*,*,#9839,.F.);
#12823=ORIENTED_EDGE('',*,*,#9840,.F.);
#12824=ORIENTED_EDGE('',*,*,#9841,.T.);
#12825=ORIENTED_EDGE('',*,*,#9842,.F.);
#12826=ORIENTED_EDGE('',*,*,#9843,.F.);
#12827=ORIENTED_EDGE('',*,*,#9752,.F.);
#12828=ORIENTED_EDGE('',*,*,#9838,.F.);
#12829=ORIENTED_EDGE('',*,*,#9844,.T.);
#12830=ORIENTED_EDGE('',*,*,#9845,.T.);
#12831=ORIENTED_EDGE('',*,*,#9846,.T.);
#12832=ORIENTED_EDGE('',*,*,#9840,.T.);
#12833=ORIENTED_EDGE('',*,*,#9846,.F.);
#12834=ORIENTED_EDGE('',*,*,#9847,.T.);
#12835=ORIENTED_EDGE('',*,*,#9608,.T.);
#12836=ORIENTED_EDGE('',*,*,#9848,.T.);
#12837=ORIENTED_EDGE('',*,*,#9849,.T.);
#12838=ORIENTED_EDGE('',*,*,#9850,.T.);
#12839=ORIENTED_EDGE('',*,*,#9851,.F.);
#12840=ORIENTED_EDGE('',*,*,#9841,.F.);
#12841=ORIENTED_EDGE('',*,*,#9842,.T.);
#12842=ORIENTED_EDGE('',*,*,#9851,.T.);
#12843=ORIENTED_EDGE('',*,*,#9852,.T.);
#12844=ORIENTED_EDGE('',*,*,#9853,.T.);
#12845=ORIENTED_EDGE('',*,*,#9854,.T.);
#12846=ORIENTED_EDGE('',*,*,#9854,.F.);
#12847=ORIENTED_EDGE('',*,*,#9855,.T.);
#12848=ORIENTED_EDGE('',*,*,#9856,.T.);
#12849=ORIENTED_EDGE('',*,*,#9857,.T.);
#12850=ORIENTED_EDGE('',*,*,#9753,.T.);
#12851=ORIENTED_EDGE('',*,*,#9843,.T.);
#12852=ORIENTED_EDGE('',*,*,#9857,.F.);
#12853=ORIENTED_EDGE('',*,*,#9858,.F.);
#12854=ORIENTED_EDGE('',*,*,#9859,.T.);
#12855=ORIENTED_EDGE('',*,*,#9860,.F.);
#12856=ORIENTED_EDGE('',*,*,#9861,.F.);
#12857=ORIENTED_EDGE('',*,*,#9754,.F.);
#12858=ORIENTED_EDGE('',*,*,#9856,.F.);
#12859=ORIENTED_EDGE('',*,*,#9862,.T.);
#12860=ORIENTED_EDGE('',*,*,#9863,.T.);
#12861=ORIENTED_EDGE('',*,*,#9864,.T.);
#12862=ORIENTED_EDGE('',*,*,#9858,.T.);
#12863=ORIENTED_EDGE('',*,*,#9773,.F.);
#12864=ORIENTED_EDGE('',*,*,#9865,.F.);
#12865=ORIENTED_EDGE('',*,*,#9866,.F.);
#12866=ORIENTED_EDGE('',*,*,#9867,.T.);
#12867=ORIENTED_EDGE('',*,*,#9477,.T.);
#12868=ORIENTED_EDGE('',*,*,#9868,.T.);
#12869=ORIENTED_EDGE('',*,*,#9869,.T.);
#12870=ORIENTED_EDGE('',*,*,#9870,.T.);
#12871=ORIENTED_EDGE('',*,*,#9645,.F.);
#12872=ORIENTED_EDGE('',*,*,#9756,.F.);
#12873=ORIENTED_EDGE('',*,*,#9871,.F.);
#12874=ORIENTED_EDGE('',*,*,#9872,.F.);
#12875=ORIENTED_EDGE('',*,*,#9865,.T.);
#12876=ORIENTED_EDGE('',*,*,#9772,.F.);
#12877=ORIENTED_EDGE('',*,*,#9864,.F.);
#12878=ORIENTED_EDGE('',*,*,#9873,.T.);
#12879=ORIENTED_EDGE('',*,*,#9621,.T.);
#12880=ORIENTED_EDGE('',*,*,#9874,.T.);
#12881=ORIENTED_EDGE('',*,*,#9875,.T.);
#12882=ORIENTED_EDGE('',*,*,#9876,.T.);
#12883=ORIENTED_EDGE('',*,*,#9877,.F.);
#12884=ORIENTED_EDGE('',*,*,#9859,.F.);
#12885=ORIENTED_EDGE('',*,*,#9860,.T.);
#12886=ORIENTED_EDGE('',*,*,#9877,.T.);
#12887=ORIENTED_EDGE('',*,*,#9878,.T.);
#12888=ORIENTED_EDGE('',*,*,#9879,.T.);
#12889=ORIENTED_EDGE('',*,*,#9880,.T.);
#12890=ORIENTED_EDGE('',*,*,#9880,.F.);
#12891=ORIENTED_EDGE('',*,*,#9881,.T.);
#12892=ORIENTED_EDGE('',*,*,#9882,.T.);
#12893=ORIENTED_EDGE('',*,*,#9871,.T.);
#12894=ORIENTED_EDGE('',*,*,#9755,.T.);
#12895=ORIENTED_EDGE('',*,*,#9861,.T.);
#12896=ORIENTED_EDGE('',*,*,#9882,.F.);
#12897=ORIENTED_EDGE('',*,*,#9883,.T.);
#12898=ORIENTED_EDGE('',*,*,#9884,.T.);
#12899=ORIENTED_EDGE('',*,*,#9866,.T.);
#12900=ORIENTED_EDGE('',*,*,#9872,.T.);
#12901=ORIENTED_EDGE('',*,*,#9884,.F.);
#12902=ORIENTED_EDGE('',*,*,#9885,.T.);
#12903=ORIENTED_EDGE('',*,*,#9886,.T.);
#12904=ORIENTED_EDGE('',*,*,#9478,.T.);
#12905=ORIENTED_EDGE('',*,*,#9867,.F.);
#12906=ORIENTED_EDGE('',*,*,#9879,.F.);
#12907=ORIENTED_EDGE('',*,*,#9887,.F.);
#12908=ORIENTED_EDGE('',*,*,#9888,.F.);
#12909=ORIENTED_EDGE('',*,*,#9889,.F.);
#12910=ORIENTED_EDGE('',*,*,#9890,.F.);
#12911=ORIENTED_EDGE('',*,*,#9885,.F.);
#12912=ORIENTED_EDGE('',*,*,#9883,.F.);
#12913=ORIENTED_EDGE('',*,*,#9881,.F.);
#12914=ORIENTED_EDGE('',*,*,#9261,.T.);
#12915=ORIENTED_EDGE('',*,*,#9891,.T.);
#12916=ORIENTED_EDGE('',*,*,#9892,.F.);
#12917=ORIENTED_EDGE('',*,*,#9893,.F.);
#12918=ORIENTED_EDGE('',*,*,#9894,.T.);
#12919=ORIENTED_EDGE('',*,*,#9894,.F.);
#12920=ORIENTED_EDGE('',*,*,#9895,.F.);
#12921=ORIENTED_EDGE('',*,*,#9163,.F.);
#12922=ORIENTED_EDGE('',*,*,#9160,.F.);
#12923=ORIENTED_EDGE('',*,*,#9157,.F.);
#12924=ORIENTED_EDGE('',*,*,#9154,.F.);
#12925=ORIENTED_EDGE('',*,*,#9151,.F.);
#12926=ORIENTED_EDGE('',*,*,#9148,.F.);
#12927=ORIENTED_EDGE('',*,*,#9145,.F.);
#12928=ORIENTED_EDGE('',*,*,#9142,.F.);
#12929=ORIENTED_EDGE('',*,*,#9139,.F.);
#12930=ORIENTED_EDGE('',*,*,#9136,.F.);
#12931=ORIENTED_EDGE('',*,*,#9133,.F.);
#12932=ORIENTED_EDGE('',*,*,#9130,.F.);
#12933=ORIENTED_EDGE('',*,*,#9127,.F.);
#12934=ORIENTED_EDGE('',*,*,#9124,.F.);
#12935=ORIENTED_EDGE('',*,*,#9121,.F.);
#12936=ORIENTED_EDGE('',*,*,#9118,.F.);
#12937=ORIENTED_EDGE('',*,*,#9896,.F.);
#12938=ORIENTED_EDGE('',*,*,#9897,.T.);
#12939=ORIENTED_EDGE('',*,*,#9307,.T.);
#12940=ORIENTED_EDGE('',*,*,#9304,.T.);
#12941=ORIENTED_EDGE('',*,*,#9301,.T.);
#12942=ORIENTED_EDGE('',*,*,#9298,.T.);
#12943=ORIENTED_EDGE('',*,*,#9295,.T.);
#12944=ORIENTED_EDGE('',*,*,#9292,.T.);
#12945=ORIENTED_EDGE('',*,*,#9289,.T.);
#12946=ORIENTED_EDGE('',*,*,#9286,.T.);
#12947=ORIENTED_EDGE('',*,*,#9283,.T.);
#12948=ORIENTED_EDGE('',*,*,#9280,.T.);
#12949=ORIENTED_EDGE('',*,*,#9277,.T.);
#12950=ORIENTED_EDGE('',*,*,#9274,.T.);
#12951=ORIENTED_EDGE('',*,*,#9271,.T.);
#12952=ORIENTED_EDGE('',*,*,#9268,.T.);
#12953=ORIENTED_EDGE('',*,*,#9265,.T.);
#12954=ORIENTED_EDGE('',*,*,#9262,.T.);
#12955=ORIENTED_EDGE('',*,*,#9898,.T.);
#12956=ORIENTED_EDGE('',*,*,#9899,.T.);
#12957=ORIENTED_EDGE('',*,*,#9900,.T.);
#12958=ORIENTED_EDGE('',*,*,#9901,.T.);
#12959=ORIENTED_EDGE('',*,*,#9896,.T.);
#12960=ORIENTED_EDGE('',*,*,#9305,.T.);
#12961=ORIENTED_EDGE('',*,*,#9897,.F.);
#12962=ORIENTED_EDGE('',*,*,#9901,.F.);
#12963=ORIENTED_EDGE('',*,*,#9902,.T.);
#12964=ORIENTED_EDGE('',*,*,#9891,.F.);
#12965=ORIENTED_EDGE('',*,*,#9260,.F.);
#12966=ORIENTED_EDGE('',*,*,#9264,.F.);
#12967=ORIENTED_EDGE('',*,*,#9267,.F.);
#12968=ORIENTED_EDGE('',*,*,#9270,.F.);
#12969=ORIENTED_EDGE('',*,*,#9273,.F.);
#12970=ORIENTED_EDGE('',*,*,#9276,.F.);
#12971=ORIENTED_EDGE('',*,*,#9279,.F.);
#12972=ORIENTED_EDGE('',*,*,#9282,.F.);
#12973=ORIENTED_EDGE('',*,*,#9285,.F.);
#12974=ORIENTED_EDGE('',*,*,#9288,.F.);
#12975=ORIENTED_EDGE('',*,*,#9291,.F.);
#12976=ORIENTED_EDGE('',*,*,#9294,.F.);
#12977=ORIENTED_EDGE('',*,*,#9297,.F.);
#12978=ORIENTED_EDGE('',*,*,#9300,.F.);
#12979=ORIENTED_EDGE('',*,*,#9303,.F.);
#12980=ORIENTED_EDGE('',*,*,#9306,.F.);
#12981=ORIENTED_EDGE('',*,*,#9902,.F.);
#12982=ORIENTED_EDGE('',*,*,#9900,.F.);
#12983=ORIENTED_EDGE('',*,*,#9116,.F.);
#12984=ORIENTED_EDGE('',*,*,#9120,.F.);
#12985=ORIENTED_EDGE('',*,*,#9123,.F.);
#12986=ORIENTED_EDGE('',*,*,#9126,.F.);
#12987=ORIENTED_EDGE('',*,*,#9129,.F.);
#12988=ORIENTED_EDGE('',*,*,#9132,.F.);
#12989=ORIENTED_EDGE('',*,*,#9135,.F.);
#12990=ORIENTED_EDGE('',*,*,#9138,.F.);
#12991=ORIENTED_EDGE('',*,*,#9141,.F.);
#12992=ORIENTED_EDGE('',*,*,#9144,.F.);
#12993=ORIENTED_EDGE('',*,*,#9147,.F.);
#12994=ORIENTED_EDGE('',*,*,#9150,.F.);
#12995=ORIENTED_EDGE('',*,*,#9153,.F.);
#12996=ORIENTED_EDGE('',*,*,#9156,.F.);
#12997=ORIENTED_EDGE('',*,*,#9159,.F.);
#12998=ORIENTED_EDGE('',*,*,#9162,.F.);
#12999=ORIENTED_EDGE('',*,*,#9903,.F.);
#13000=ORIENTED_EDGE('',*,*,#9904,.F.);
#13001=ORIENTED_EDGE('',*,*,#9889,.T.);
#13002=ORIENTED_EDGE('',*,*,#9164,.T.);
#13003=ORIENTED_EDGE('',*,*,#9479,.T.);
#13004=ORIENTED_EDGE('',*,*,#9886,.F.);
#13005=ORIENTED_EDGE('',*,*,#9890,.T.);
#13006=ORIENTED_EDGE('',*,*,#9904,.T.);
#13007=ORIENTED_EDGE('',*,*,#9888,.T.);
#13008=ORIENTED_EDGE('',*,*,#9905,.F.);
#13009=ORIENTED_EDGE('',*,*,#9906,.T.);
#13010=ORIENTED_EDGE('',*,*,#9878,.F.);
#13011=ORIENTED_EDGE('',*,*,#9876,.F.);
#13012=ORIENTED_EDGE('',*,*,#9907,.T.);
#13013=ORIENTED_EDGE('',*,*,#9905,.T.);
#13014=ORIENTED_EDGE('',*,*,#9887,.T.);
#13015=ORIENTED_EDGE('',*,*,#9173,.F.);
#13016=ORIENTED_EDGE('',*,*,#9908,.T.);
#13017=ORIENTED_EDGE('',*,*,#9853,.F.);
#13018=ORIENTED_EDGE('',*,*,#9909,.F.);
#13019=ORIENTED_EDGE('',*,*,#9174,.F.);
#13020=ORIENTED_EDGE('',*,*,#9908,.F.);
#13021=ORIENTED_EDGE('',*,*,#9172,.F.);
#13022=ORIENTED_EDGE('',*,*,#9910,.F.);
#13023=ORIENTED_EDGE('',*,*,#9862,.F.);
#13024=ORIENTED_EDGE('',*,*,#9855,.F.);
#13025=ORIENTED_EDGE('',*,*,#9852,.F.);
#13026=ORIENTED_EDGE('',*,*,#9850,.F.);
#13027=ORIENTED_EDGE('',*,*,#9911,.T.);
#13028=ORIENTED_EDGE('',*,*,#9175,.T.);
#13029=ORIENTED_EDGE('',*,*,#9909,.T.);
#13030=ORIENTED_EDGE('',*,*,#9863,.F.);
#13031=ORIENTED_EDGE('',*,*,#9910,.T.);
#13032=ORIENTED_EDGE('',*,*,#9171,.T.);
#13033=ORIENTED_EDGE('',*,*,#9622,.T.);
#13034=ORIENTED_EDGE('',*,*,#9873,.F.);
#13035=ORIENTED_EDGE('',*,*,#9181,.F.);
#13036=ORIENTED_EDGE('',*,*,#9912,.T.);
#13037=ORIENTED_EDGE('',*,*,#9835,.F.);
#13038=ORIENTED_EDGE('',*,*,#9913,.F.);
#13039=ORIENTED_EDGE('',*,*,#9182,.F.);
#13040=ORIENTED_EDGE('',*,*,#9912,.F.);
#13041=ORIENTED_EDGE('',*,*,#9180,.F.);
#13042=ORIENTED_EDGE('',*,*,#9914,.F.);
#13043=ORIENTED_EDGE('',*,*,#9844,.F.);
#13044=ORIENTED_EDGE('',*,*,#9837,.F.);
#13045=ORIENTED_EDGE('',*,*,#9834,.F.);
#13046=ORIENTED_EDGE('',*,*,#9832,.F.);
#13047=ORIENTED_EDGE('',*,*,#9915,.T.);
#13048=ORIENTED_EDGE('',*,*,#9183,.T.);
#13049=ORIENTED_EDGE('',*,*,#9913,.T.);
#13050=ORIENTED_EDGE('',*,*,#9845,.F.);
#13051=ORIENTED_EDGE('',*,*,#9914,.T.);
#13052=ORIENTED_EDGE('',*,*,#9179,.T.);
#13053=ORIENTED_EDGE('',*,*,#9609,.T.);
#13054=ORIENTED_EDGE('',*,*,#9847,.F.);
#13055=ORIENTED_EDGE('',*,*,#9189,.F.);
#13056=ORIENTED_EDGE('',*,*,#9916,.T.);
#13057=ORIENTED_EDGE('',*,*,#9817,.F.);
#13058=ORIENTED_EDGE('',*,*,#9917,.F.);
#13059=ORIENTED_EDGE('',*,*,#9190,.F.);
#13060=ORIENTED_EDGE('',*,*,#9916,.F.);
#13061=ORIENTED_EDGE('',*,*,#9188,.F.);
#13062=ORIENTED_EDGE('',*,*,#9918,.F.);
#13063=ORIENTED_EDGE('',*,*,#9826,.F.);
#13064=ORIENTED_EDGE('',*,*,#9819,.F.);
#13065=ORIENTED_EDGE('',*,*,#9816,.F.);
#13066=ORIENTED_EDGE('',*,*,#9814,.F.);
#13067=ORIENTED_EDGE('',*,*,#9919,.T.);
#13068=ORIENTED_EDGE('',*,*,#9191,.T.);
#13069=ORIENTED_EDGE('',*,*,#9917,.T.);
#13070=ORIENTED_EDGE('',*,*,#9827,.F.);
#13071=ORIENTED_EDGE('',*,*,#9918,.T.);
#13072=ORIENTED_EDGE('',*,*,#9187,.T.);
#13073=ORIENTED_EDGE('',*,*,#9596,.T.);
#13074=ORIENTED_EDGE('',*,*,#9829,.F.);
#13075=ORIENTED_EDGE('',*,*,#9197,.F.);
#13076=ORIENTED_EDGE('',*,*,#9920,.T.);
#13077=ORIENTED_EDGE('',*,*,#9799,.F.);
#13078=ORIENTED_EDGE('',*,*,#9921,.F.);
#13079=ORIENTED_EDGE('',*,*,#9198,.F.);
#13080=ORIENTED_EDGE('',*,*,#9920,.F.);
#13081=ORIENTED_EDGE('',*,*,#9196,.F.);
#13082=ORIENTED_EDGE('',*,*,#9922,.F.);
#13083=ORIENTED_EDGE('',*,*,#9808,.F.);
#13084=ORIENTED_EDGE('',*,*,#9801,.F.);
#13085=ORIENTED_EDGE('',*,*,#9798,.F.);
#13086=ORIENTED_EDGE('',*,*,#9796,.F.);
#13087=ORIENTED_EDGE('',*,*,#9923,.T.);
#13088=ORIENTED_EDGE('',*,*,#9199,.T.);
#13089=ORIENTED_EDGE('',*,*,#9921,.T.);
#13090=ORIENTED_EDGE('',*,*,#9809,.F.);
#13091=ORIENTED_EDGE('',*,*,#9922,.T.);
#13092=ORIENTED_EDGE('',*,*,#9195,.T.);
#13093=ORIENTED_EDGE('',*,*,#9583,.T.);
#13094=ORIENTED_EDGE('',*,*,#9811,.F.);
#13095=ORIENTED_EDGE('',*,*,#9205,.F.);
#13096=ORIENTED_EDGE('',*,*,#9924,.T.);
#13097=ORIENTED_EDGE('',*,*,#9781,.F.);
#13098=ORIENTED_EDGE('',*,*,#9925,.F.);
#13099=ORIENTED_EDGE('',*,*,#9206,.F.);
#13100=ORIENTED_EDGE('',*,*,#9924,.F.);
#13101=ORIENTED_EDGE('',*,*,#9204,.F.);
#13102=ORIENTED_EDGE('',*,*,#9926,.F.);
#13103=ORIENTED_EDGE('',*,*,#9790,.F.);
#13104=ORIENTED_EDGE('',*,*,#9783,.F.);
#13105=ORIENTED_EDGE('',*,*,#9780,.F.);
#13106=ORIENTED_EDGE('',*,*,#9778,.F.);
#13107=ORIENTED_EDGE('',*,*,#9927,.T.);
#13108=ORIENTED_EDGE('',*,*,#9207,.T.);
#13109=ORIENTED_EDGE('',*,*,#9925,.T.);
#13110=ORIENTED_EDGE('',*,*,#9791,.F.);
#13111=ORIENTED_EDGE('',*,*,#9926,.T.);
#13112=ORIENTED_EDGE('',*,*,#9203,.T.);
#13113=ORIENTED_EDGE('',*,*,#9570,.T.);
#13114=ORIENTED_EDGE('',*,*,#9793,.F.);
#13115=ORIENTED_EDGE('',*,*,#9213,.F.);
#13116=ORIENTED_EDGE('',*,*,#9928,.T.);
#13117=ORIENTED_EDGE('',*,*,#9738,.F.);
#13118=ORIENTED_EDGE('',*,*,#9929,.F.);
#13119=ORIENTED_EDGE('',*,*,#9214,.F.);
#13120=ORIENTED_EDGE('',*,*,#9928,.F.);
#13121=ORIENTED_EDGE('',*,*,#9212,.F.);
#13122=ORIENTED_EDGE('',*,*,#9930,.F.);
#13123=ORIENTED_EDGE('',*,*,#9762,.F.);
#13124=ORIENTED_EDGE('',*,*,#9740,.F.);
#13125=ORIENTED_EDGE('',*,*,#9737,.F.);
#13126=ORIENTED_EDGE('',*,*,#9735,.F.);
#13127=ORIENTED_EDGE('',*,*,#9931,.T.);
#13128=ORIENTED_EDGE('',*,*,#9215,.T.);
#13129=ORIENTED_EDGE('',*,*,#9929,.T.);
#13130=ORIENTED_EDGE('',*,*,#9763,.F.);
#13131=ORIENTED_EDGE('',*,*,#9930,.T.);
#13132=ORIENTED_EDGE('',*,*,#9211,.T.);
#13133=ORIENTED_EDGE('',*,*,#9557,.T.);
#13134=ORIENTED_EDGE('',*,*,#9775,.F.);
#13135=ORIENTED_EDGE('',*,*,#9221,.F.);
#13136=ORIENTED_EDGE('',*,*,#9932,.T.);
#13137=ORIENTED_EDGE('',*,*,#9718,.F.);
#13138=ORIENTED_EDGE('',*,*,#9933,.F.);
#13139=ORIENTED_EDGE('',*,*,#9222,.F.);
#13140=ORIENTED_EDGE('',*,*,#9932,.F.);
#13141=ORIENTED_EDGE('',*,*,#9220,.F.);
#13142=ORIENTED_EDGE('',*,*,#9934,.F.);
#13143=ORIENTED_EDGE('',*,*,#9727,.F.);
#13144=ORIENTED_EDGE('',*,*,#9720,.F.);
#13145=ORIENTED_EDGE('',*,*,#9717,.F.);
#13146=ORIENTED_EDGE('',*,*,#9715,.F.);
#13147=ORIENTED_EDGE('',*,*,#9935,.T.);
#13148=ORIENTED_EDGE('',*,*,#9223,.T.);
#13149=ORIENTED_EDGE('',*,*,#9933,.T.);
#13150=ORIENTED_EDGE('',*,*,#9724,.F.);
#13151=ORIENTED_EDGE('',*,*,#9934,.T.);
#13152=ORIENTED_EDGE('',*,*,#9219,.T.);
#13153=ORIENTED_EDGE('',*,*,#9544,.T.);
#13154=ORIENTED_EDGE('',*,*,#9732,.F.);
#13155=ORIENTED_EDGE('',*,*,#9229,.F.);
#13156=ORIENTED_EDGE('',*,*,#9936,.T.);
#13157=ORIENTED_EDGE('',*,*,#9698,.F.);
#13158=ORIENTED_EDGE('',*,*,#9937,.F.);
#13159=ORIENTED_EDGE('',*,*,#9230,.F.);
#13160=ORIENTED_EDGE('',*,*,#9936,.F.);
#13161=ORIENTED_EDGE('',*,*,#9228,.F.);
#13162=ORIENTED_EDGE('',*,*,#9938,.F.);
#13163=ORIENTED_EDGE('',*,*,#9707,.F.);
#13164=ORIENTED_EDGE('',*,*,#9700,.F.);
#13165=ORIENTED_EDGE('',*,*,#9697,.F.);
#13166=ORIENTED_EDGE('',*,*,#9695,.F.);
#13167=ORIENTED_EDGE('',*,*,#9939,.T.);
#13168=ORIENTED_EDGE('',*,*,#9231,.T.);
#13169=ORIENTED_EDGE('',*,*,#9937,.T.);
#13170=ORIENTED_EDGE('',*,*,#9704,.F.);
#13171=ORIENTED_EDGE('',*,*,#9938,.T.);
#13172=ORIENTED_EDGE('',*,*,#9227,.T.);
#13173=ORIENTED_EDGE('',*,*,#9531,.T.);
#13174=ORIENTED_EDGE('',*,*,#9712,.F.);
#13175=ORIENTED_EDGE('',*,*,#9237,.F.);
#13176=ORIENTED_EDGE('',*,*,#9940,.T.);
#13177=ORIENTED_EDGE('',*,*,#9678,.F.);
#13178=ORIENTED_EDGE('',*,*,#9941,.F.);
#13179=ORIENTED_EDGE('',*,*,#9238,.F.);
#13180=ORIENTED_EDGE('',*,*,#9940,.F.);
#13181=ORIENTED_EDGE('',*,*,#9236,.F.);
#13182=ORIENTED_EDGE('',*,*,#9942,.F.);
#13183=ORIENTED_EDGE('',*,*,#9687,.F.);
#13184=ORIENTED_EDGE('',*,*,#9680,.F.);
#13185=ORIENTED_EDGE('',*,*,#9677,.F.);
#13186=ORIENTED_EDGE('',*,*,#9675,.F.);
#13187=ORIENTED_EDGE('',*,*,#9943,.T.);
#13188=ORIENTED_EDGE('',*,*,#9239,.T.);
#13189=ORIENTED_EDGE('',*,*,#9941,.T.);
#13190=ORIENTED_EDGE('',*,*,#9684,.F.);
#13191=ORIENTED_EDGE('',*,*,#9942,.T.);
#13192=ORIENTED_EDGE('',*,*,#9235,.T.);
#13193=ORIENTED_EDGE('',*,*,#9518,.T.);
#13194=ORIENTED_EDGE('',*,*,#9692,.F.);
#13195=ORIENTED_EDGE('',*,*,#9245,.F.);
#13196=ORIENTED_EDGE('',*,*,#9766,.T.);
#13197=ORIENTED_EDGE('',*,*,#9657,.F.);
#13198=ORIENTED_EDGE('',*,*,#9655,.F.);
#13199=ORIENTED_EDGE('',*,*,#9944,.T.);
#13200=ORIENTED_EDGE('',*,*,#9247,.T.);
#13201=ORIENTED_EDGE('',*,*,#9765,.T.);
#13202=ORIENTED_EDGE('',*,*,#9664,.F.);
#13203=ORIENTED_EDGE('',*,*,#9767,.T.);
#13204=ORIENTED_EDGE('',*,*,#9243,.T.);
#13205=ORIENTED_EDGE('',*,*,#9505,.T.);
#13206=ORIENTED_EDGE('',*,*,#9672,.F.);
#13207=ORIENTED_EDGE('',*,*,#9253,.F.);
#13208=ORIENTED_EDGE('',*,*,#9770,.T.);
#13209=ORIENTED_EDGE('',*,*,#9774,.F.);
#13210=ORIENTED_EDGE('',*,*,#9870,.F.);
#13211=ORIENTED_EDGE('',*,*,#9945,.T.);
#13212=ORIENTED_EDGE('',*,*,#9255,.T.);
#13213=ORIENTED_EDGE('',*,*,#9769,.T.);
#13214=ORIENTED_EDGE('',*,*,#9638,.F.);
#13215=ORIENTED_EDGE('',*,*,#9771,.T.);
#13216=ORIENTED_EDGE('',*,*,#9251,.T.);
#13217=ORIENTED_EDGE('',*,*,#9492,.T.);
#13218=ORIENTED_EDGE('',*,*,#9652,.F.);
#13219=ORIENTED_EDGE('',*,*,#9946,.T.);
#13220=ORIENTED_EDGE('',*,*,#9947,.T.);
#13221=ORIENTED_EDGE('',*,*,#9948,.F.);
#13222=ORIENTED_EDGE('',*,*,#9947,.F.);
#13223=ORIENTED_EDGE('',*,*,#9630,.F.);
#13224=ORIENTED_EDGE('',*,*,#9946,.F.);
#13225=ORIENTED_EDGE('',*,*,#9949,.F.);
#13226=ORIENTED_EDGE('',*,*,#9948,.T.);
#13227=ORIENTED_EDGE('',*,*,#9950,.F.);
#13228=ORIENTED_EDGE('',*,*,#9951,.T.);
#13229=ORIENTED_EDGE('',*,*,#9949,.T.);
#13230=ORIENTED_EDGE('',*,*,#9951,.F.);
#13231=ORIENTED_EDGE('',*,*,#9635,.T.);
#13232=ORIENTED_EDGE('',*,*,#9952,.T.);
#13233=ORIENTED_EDGE('',*,*,#9629,.F.);
#13234=ORIENTED_EDGE('',*,*,#9952,.F.);
#13235=ORIENTED_EDGE('',*,*,#9166,.F.);
#13236=ORIENTED_EDGE('',*,*,#9953,.T.);
#13237=ORIENTED_EDGE('',*,*,#9954,.F.);
#13238=ORIENTED_EDGE('',*,*,#9623,.T.);
#13239=ORIENTED_EDGE('',*,*,#9614,.F.);
#13240=ORIENTED_EDGE('',*,*,#9955,.T.);
#13241=ORIENTED_EDGE('',*,*,#9874,.F.);
#13242=ORIENTED_EDGE('',*,*,#9620,.T.);
#13243=ORIENTED_EDGE('',*,*,#9956,.T.);
#13244=ORIENTED_EDGE('',*,*,#9618,.F.);
#13245=ORIENTED_EDGE('',*,*,#9625,.T.);
#13246=ORIENTED_EDGE('',*,*,#9624,.T.);
#13247=ORIENTED_EDGE('',*,*,#9954,.T.);
#13248=ORIENTED_EDGE('',*,*,#9613,.F.);
#13249=ORIENTED_EDGE('',*,*,#9619,.F.);
#13250=ORIENTED_EDGE('',*,*,#9956,.F.);
#13251=ORIENTED_EDGE('',*,*,#9953,.F.);
#13252=ORIENTED_EDGE('',*,*,#9165,.F.);
#13253=ORIENTED_EDGE('',*,*,#9906,.F.);
#13254=ORIENTED_EDGE('',*,*,#9907,.F.);
#13255=ORIENTED_EDGE('',*,*,#9875,.F.);
#13256=ORIENTED_EDGE('',*,*,#9955,.F.);
#13257=ORIENTED_EDGE('',*,*,#9177,.F.);
#13258=ORIENTED_EDGE('',*,*,#9957,.T.);
#13259=ORIENTED_EDGE('',*,*,#9958,.F.);
#13260=ORIENTED_EDGE('',*,*,#9610,.T.);
#13261=ORIENTED_EDGE('',*,*,#9601,.F.);
#13262=ORIENTED_EDGE('',*,*,#9959,.T.);
#13263=ORIENTED_EDGE('',*,*,#9848,.F.);
#13264=ORIENTED_EDGE('',*,*,#9607,.T.);
#13265=ORIENTED_EDGE('',*,*,#9960,.T.);
#13266=ORIENTED_EDGE('',*,*,#9605,.F.);
#13267=ORIENTED_EDGE('',*,*,#9612,.T.);
#13268=ORIENTED_EDGE('',*,*,#9611,.T.);
#13269=ORIENTED_EDGE('',*,*,#9958,.T.);
#13270=ORIENTED_EDGE('',*,*,#9600,.F.);
#13271=ORIENTED_EDGE('',*,*,#9606,.F.);
#13272=ORIENTED_EDGE('',*,*,#9960,.F.);
#13273=ORIENTED_EDGE('',*,*,#9957,.F.);
#13274=ORIENTED_EDGE('',*,*,#9176,.F.);
#13275=ORIENTED_EDGE('',*,*,#9911,.F.);
#13276=ORIENTED_EDGE('',*,*,#9849,.F.);
#13277=ORIENTED_EDGE('',*,*,#9959,.F.);
#13278=ORIENTED_EDGE('',*,*,#9185,.F.);
#13279=ORIENTED_EDGE('',*,*,#9961,.T.);
#13280=ORIENTED_EDGE('',*,*,#9962,.F.);
#13281=ORIENTED_EDGE('',*,*,#9597,.T.);
#13282=ORIENTED_EDGE('',*,*,#9588,.F.);
#13283=ORIENTED_EDGE('',*,*,#9963,.T.);
#13284=ORIENTED_EDGE('',*,*,#9830,.F.);
#13285=ORIENTED_EDGE('',*,*,#9594,.T.);
#13286=ORIENTED_EDGE('',*,*,#9964,.T.);
#13287=ORIENTED_EDGE('',*,*,#9592,.F.);
#13288=ORIENTED_EDGE('',*,*,#9599,.T.);
#13289=ORIENTED_EDGE('',*,*,#9598,.T.);
#13290=ORIENTED_EDGE('',*,*,#9962,.T.);
#13291=ORIENTED_EDGE('',*,*,#9587,.F.);
#13292=ORIENTED_EDGE('',*,*,#9593,.F.);
#13293=ORIENTED_EDGE('',*,*,#9964,.F.);
#13294=ORIENTED_EDGE('',*,*,#9961,.F.);
#13295=ORIENTED_EDGE('',*,*,#9184,.F.);
#13296=ORIENTED_EDGE('',*,*,#9915,.F.);
#13297=ORIENTED_EDGE('',*,*,#9831,.F.);
#13298=ORIENTED_EDGE('',*,*,#9963,.F.);
#13299=ORIENTED_EDGE('',*,*,#9193,.F.);
#13300=ORIENTED_EDGE('',*,*,#9965,.T.);
#13301=ORIENTED_EDGE('',*,*,#9966,.F.);
#13302=ORIENTED_EDGE('',*,*,#9584,.T.);
#13303=ORIENTED_EDGE('',*,*,#9575,.F.);
#13304=ORIENTED_EDGE('',*,*,#9967,.T.);
#13305=ORIENTED_EDGE('',*,*,#9812,.F.);
#13306=ORIENTED_EDGE('',*,*,#9581,.T.);
#13307=ORIENTED_EDGE('',*,*,#9968,.T.);
#13308=ORIENTED_EDGE('',*,*,#9579,.F.);
#13309=ORIENTED_EDGE('',*,*,#9586,.T.);
#13310=ORIENTED_EDGE('',*,*,#9585,.T.);
#13311=ORIENTED_EDGE('',*,*,#9966,.T.);
#13312=ORIENTED_EDGE('',*,*,#9574,.F.);
#13313=ORIENTED_EDGE('',*,*,#9580,.F.);
#13314=ORIENTED_EDGE('',*,*,#9968,.F.);
#13315=ORIENTED_EDGE('',*,*,#9965,.F.);
#13316=ORIENTED_EDGE('',*,*,#9192,.F.);
#13317=ORIENTED_EDGE('',*,*,#9919,.F.);
#13318=ORIENTED_EDGE('',*,*,#9813,.F.);
#13319=ORIENTED_EDGE('',*,*,#9967,.F.);
#13320=ORIENTED_EDGE('',*,*,#9201,.F.);
#13321=ORIENTED_EDGE('',*,*,#9969,.T.);
#13322=ORIENTED_EDGE('',*,*,#9970,.F.);
#13323=ORIENTED_EDGE('',*,*,#9571,.T.);
#13324=ORIENTED_EDGE('',*,*,#9562,.F.);
#13325=ORIENTED_EDGE('',*,*,#9971,.T.);
#13326=ORIENTED_EDGE('',*,*,#9794,.F.);
#13327=ORIENTED_EDGE('',*,*,#9568,.T.);
#13328=ORIENTED_EDGE('',*,*,#9972,.T.);
#13329=ORIENTED_EDGE('',*,*,#9566,.F.);
#13330=ORIENTED_EDGE('',*,*,#9573,.T.);
#13331=ORIENTED_EDGE('',*,*,#9572,.T.);
#13332=ORIENTED_EDGE('',*,*,#9970,.T.);
#13333=ORIENTED_EDGE('',*,*,#9561,.F.);
#13334=ORIENTED_EDGE('',*,*,#9567,.F.);
#13335=ORIENTED_EDGE('',*,*,#9972,.F.);
#13336=ORIENTED_EDGE('',*,*,#9969,.F.);
#13337=ORIENTED_EDGE('',*,*,#9200,.F.);
#13338=ORIENTED_EDGE('',*,*,#9923,.F.);
#13339=ORIENTED_EDGE('',*,*,#9795,.F.);
#13340=ORIENTED_EDGE('',*,*,#9971,.F.);
#13341=ORIENTED_EDGE('',*,*,#9209,.F.);
#13342=ORIENTED_EDGE('',*,*,#9973,.T.);
#13343=ORIENTED_EDGE('',*,*,#9974,.F.);
#13344=ORIENTED_EDGE('',*,*,#9558,.T.);
#13345=ORIENTED_EDGE('',*,*,#9549,.F.);
#13346=ORIENTED_EDGE('',*,*,#9975,.T.);
#13347=ORIENTED_EDGE('',*,*,#9776,.F.);
#13348=ORIENTED_EDGE('',*,*,#9555,.T.);
#13349=ORIENTED_EDGE('',*,*,#9976,.T.);
#13350=ORIENTED_EDGE('',*,*,#9553,.F.);
#13351=ORIENTED_EDGE('',*,*,#9560,.T.);
#13352=ORIENTED_EDGE('',*,*,#9559,.T.);
#13353=ORIENTED_EDGE('',*,*,#9974,.T.);
#13354=ORIENTED_EDGE('',*,*,#9548,.F.);
#13355=ORIENTED_EDGE('',*,*,#9554,.F.);
#13356=ORIENTED_EDGE('',*,*,#9976,.F.);
#13357=ORIENTED_EDGE('',*,*,#9973,.F.);
#13358=ORIENTED_EDGE('',*,*,#9208,.F.);
#13359=ORIENTED_EDGE('',*,*,#9927,.F.);
#13360=ORIENTED_EDGE('',*,*,#9777,.F.);
#13361=ORIENTED_EDGE('',*,*,#9975,.F.);
#13362=ORIENTED_EDGE('',*,*,#9217,.F.);
#13363=ORIENTED_EDGE('',*,*,#9977,.T.);
#13364=ORIENTED_EDGE('',*,*,#9978,.F.);
#13365=ORIENTED_EDGE('',*,*,#9545,.T.);
#13366=ORIENTED_EDGE('',*,*,#9536,.F.);
#13367=ORIENTED_EDGE('',*,*,#9979,.T.);
#13368=ORIENTED_EDGE('',*,*,#9733,.F.);
#13369=ORIENTED_EDGE('',*,*,#9542,.T.);
#13370=ORIENTED_EDGE('',*,*,#9980,.T.);
#13371=ORIENTED_EDGE('',*,*,#9540,.F.);
#13372=ORIENTED_EDGE('',*,*,#9547,.T.);
#13373=ORIENTED_EDGE('',*,*,#9546,.T.);
#13374=ORIENTED_EDGE('',*,*,#9978,.T.);
#13375=ORIENTED_EDGE('',*,*,#9535,.F.);
#13376=ORIENTED_EDGE('',*,*,#9541,.F.);
#13377=ORIENTED_EDGE('',*,*,#9980,.F.);
#13378=ORIENTED_EDGE('',*,*,#9977,.F.);
#13379=ORIENTED_EDGE('',*,*,#9216,.F.);
#13380=ORIENTED_EDGE('',*,*,#9931,.F.);
#13381=ORIENTED_EDGE('',*,*,#9734,.F.);
#13382=ORIENTED_EDGE('',*,*,#9979,.F.);
#13383=ORIENTED_EDGE('',*,*,#9225,.F.);
#13384=ORIENTED_EDGE('',*,*,#9981,.T.);
#13385=ORIENTED_EDGE('',*,*,#9982,.F.);
#13386=ORIENTED_EDGE('',*,*,#9532,.T.);
#13387=ORIENTED_EDGE('',*,*,#9523,.F.);
#13388=ORIENTED_EDGE('',*,*,#9983,.T.);
#13389=ORIENTED_EDGE('',*,*,#9713,.F.);
#13390=ORIENTED_EDGE('',*,*,#9529,.T.);
#13391=ORIENTED_EDGE('',*,*,#9984,.T.);
#13392=ORIENTED_EDGE('',*,*,#9527,.F.);
#13393=ORIENTED_EDGE('',*,*,#9534,.T.);
#13394=ORIENTED_EDGE('',*,*,#9533,.T.);
#13395=ORIENTED_EDGE('',*,*,#9982,.T.);
#13396=ORIENTED_EDGE('',*,*,#9522,.F.);
#13397=ORIENTED_EDGE('',*,*,#9528,.F.);
#13398=ORIENTED_EDGE('',*,*,#9984,.F.);
#13399=ORIENTED_EDGE('',*,*,#9981,.F.);
#13400=ORIENTED_EDGE('',*,*,#9224,.F.);
#13401=ORIENTED_EDGE('',*,*,#9935,.F.);
#13402=ORIENTED_EDGE('',*,*,#9714,.F.);
#13403=ORIENTED_EDGE('',*,*,#9983,.F.);
#13404=ORIENTED_EDGE('',*,*,#9233,.F.);
#13405=ORIENTED_EDGE('',*,*,#9985,.T.);
#13406=ORIENTED_EDGE('',*,*,#9986,.F.);
#13407=ORIENTED_EDGE('',*,*,#9519,.T.);
#13408=ORIENTED_EDGE('',*,*,#9510,.F.);
#13409=ORIENTED_EDGE('',*,*,#9987,.T.);
#13410=ORIENTED_EDGE('',*,*,#9693,.F.);
#13411=ORIENTED_EDGE('',*,*,#9516,.T.);
#13412=ORIENTED_EDGE('',*,*,#9988,.T.);
#13413=ORIENTED_EDGE('',*,*,#9514,.F.);
#13414=ORIENTED_EDGE('',*,*,#9521,.T.);
#13415=ORIENTED_EDGE('',*,*,#9520,.T.);
#13416=ORIENTED_EDGE('',*,*,#9986,.T.);
#13417=ORIENTED_EDGE('',*,*,#9509,.F.);
#13418=ORIENTED_EDGE('',*,*,#9515,.F.);
#13419=ORIENTED_EDGE('',*,*,#9988,.F.);
#13420=ORIENTED_EDGE('',*,*,#9985,.F.);
#13421=ORIENTED_EDGE('',*,*,#9232,.F.);
#13422=ORIENTED_EDGE('',*,*,#9939,.F.);
#13423=ORIENTED_EDGE('',*,*,#9694,.F.);
#13424=ORIENTED_EDGE('',*,*,#9987,.F.);
#13425=ORIENTED_EDGE('',*,*,#9241,.F.);
#13426=ORIENTED_EDGE('',*,*,#9989,.T.);
#13427=ORIENTED_EDGE('',*,*,#9990,.F.);
#13428=ORIENTED_EDGE('',*,*,#9506,.T.);
#13429=ORIENTED_EDGE('',*,*,#9497,.F.);
#13430=ORIENTED_EDGE('',*,*,#9991,.T.);
#13431=ORIENTED_EDGE('',*,*,#9673,.F.);
#13432=ORIENTED_EDGE('',*,*,#9503,.T.);
#13433=ORIENTED_EDGE('',*,*,#9992,.T.);
#13434=ORIENTED_EDGE('',*,*,#9501,.F.);
#13435=ORIENTED_EDGE('',*,*,#9508,.T.);
#13436=ORIENTED_EDGE('',*,*,#9507,.T.);
#13437=ORIENTED_EDGE('',*,*,#9990,.T.);
#13438=ORIENTED_EDGE('',*,*,#9496,.F.);
#13439=ORIENTED_EDGE('',*,*,#9502,.F.);
#13440=ORIENTED_EDGE('',*,*,#9992,.F.);
#13441=ORIENTED_EDGE('',*,*,#9989,.F.);
#13442=ORIENTED_EDGE('',*,*,#9240,.F.);
#13443=ORIENTED_EDGE('',*,*,#9943,.F.);
#13444=ORIENTED_EDGE('',*,*,#9674,.F.);
#13445=ORIENTED_EDGE('',*,*,#9991,.F.);
#13446=ORIENTED_EDGE('',*,*,#9249,.F.);
#13447=ORIENTED_EDGE('',*,*,#9993,.T.);
#13448=ORIENTED_EDGE('',*,*,#9994,.F.);
#13449=ORIENTED_EDGE('',*,*,#9493,.T.);
#13450=ORIENTED_EDGE('',*,*,#9484,.F.);
#13451=ORIENTED_EDGE('',*,*,#9995,.T.);
#13452=ORIENTED_EDGE('',*,*,#9653,.F.);
#13453=ORIENTED_EDGE('',*,*,#9490,.T.);
#13454=ORIENTED_EDGE('',*,*,#9996,.T.);
#13455=ORIENTED_EDGE('',*,*,#9488,.F.);
#13456=ORIENTED_EDGE('',*,*,#9495,.T.);
#13457=ORIENTED_EDGE('',*,*,#9494,.T.);
#13458=ORIENTED_EDGE('',*,*,#9994,.T.);
#13459=ORIENTED_EDGE('',*,*,#9483,.F.);
#13460=ORIENTED_EDGE('',*,*,#9489,.F.);
#13461=ORIENTED_EDGE('',*,*,#9996,.F.);
#13462=ORIENTED_EDGE('',*,*,#9993,.F.);
#13463=ORIENTED_EDGE('',*,*,#9248,.F.);
#13464=ORIENTED_EDGE('',*,*,#9944,.F.);
#13465=ORIENTED_EDGE('',*,*,#9654,.F.);
#13466=ORIENTED_EDGE('',*,*,#9995,.F.);
#13467=ORIENTED_EDGE('',*,*,#9257,.F.);
#13468=ORIENTED_EDGE('',*,*,#9997,.T.);
#13469=ORIENTED_EDGE('',*,*,#9998,.F.);
#13470=ORIENTED_EDGE('',*,*,#9480,.T.);
#13471=ORIENTED_EDGE('',*,*,#9470,.F.);
#13472=ORIENTED_EDGE('',*,*,#9999,.T.);
#13473=ORIENTED_EDGE('',*,*,#9868,.F.);
#13474=ORIENTED_EDGE('',*,*,#9476,.T.);
#13475=ORIENTED_EDGE('',*,*,#10000,.T.);
#13476=ORIENTED_EDGE('',*,*,#9474,.F.);
#13477=ORIENTED_EDGE('',*,*,#9482,.T.);
#13478=ORIENTED_EDGE('',*,*,#9481,.T.);
#13479=ORIENTED_EDGE('',*,*,#9998,.T.);
#13480=ORIENTED_EDGE('',*,*,#9469,.F.);
#13481=ORIENTED_EDGE('',*,*,#9475,.F.);
#13482=ORIENTED_EDGE('',*,*,#10000,.F.);
#13483=ORIENTED_EDGE('',*,*,#9997,.F.);
#13484=ORIENTED_EDGE('',*,*,#9256,.F.);
#13485=ORIENTED_EDGE('',*,*,#9945,.F.);
#13486=ORIENTED_EDGE('',*,*,#9869,.F.);
#13487=ORIENTED_EDGE('',*,*,#9999,.F.);
#13488=ORIENTED_EDGE('',*,*,#9398,.F.);
#13489=ORIENTED_EDGE('',*,*,#10001,.T.);
#13490=ORIENTED_EDGE('',*,*,#9414,.F.);
#13491=ORIENTED_EDGE('',*,*,#10002,.T.);
#13492=ORIENTED_EDGE('',*,*,#9402,.T.);
#13493=ORIENTED_EDGE('',*,*,#9447,.F.);
#13494=ORIENTED_EDGE('',*,*,#10003,.F.);
#13495=ORIENTED_EDGE('',*,*,#9463,.F.);
#13496=ORIENTED_EDGE('',*,*,#9454,.F.);
#13497=ORIENTED_EDGE('',*,*,#9434,.F.);
#13498=ORIENTED_EDGE('',*,*,#10004,.F.);
#13499=ORIENTED_EDGE('',*,*,#9450,.F.);
#13500=ORIENTED_EDGE('',*,*,#9441,.F.);
#13501=ORIENTED_EDGE('',*,*,#9421,.F.);
#13502=ORIENTED_EDGE('',*,*,#10005,.F.);
#13503=ORIENTED_EDGE('',*,*,#9437,.F.);
#13504=ORIENTED_EDGE('',*,*,#9428,.F.);
#13505=ORIENTED_EDGE('',*,*,#9407,.F.);
#13506=ORIENTED_EDGE('',*,*,#10006,.F.);
#13507=ORIENTED_EDGE('',*,*,#9424,.F.);
#13508=ORIENTED_EDGE('',*,*,#9415,.F.);
#13509=ORIENTED_EDGE('',*,*,#9397,.F.);
#13510=ORIENTED_EDGE('',*,*,#10007,.F.);
#13511=ORIENTED_EDGE('',*,*,#9410,.F.);
#13512=ORIENTED_EDGE('',*,*,#10001,.F.);
#13513=ORIENTED_EDGE('',*,*,#9384,.F.);
#13514=ORIENTED_EDGE('',*,*,#10008,.F.);
#13515=ORIENTED_EDGE('',*,*,#9400,.F.);
#13516=ORIENTED_EDGE('',*,*,#9391,.F.);
#13517=ORIENTED_EDGE('',*,*,#9393,.F.);
#13518=ORIENTED_EDGE('',*,*,#9403,.F.);
#13519=ORIENTED_EDGE('',*,*,#10002,.F.);
#13520=ORIENTED_EDGE('',*,*,#9413,.F.);
#13521=ORIENTED_EDGE('',*,*,#9417,.F.);
#13522=ORIENTED_EDGE('',*,*,#9427,.F.);
#13523=ORIENTED_EDGE('',*,*,#9430,.F.);
#13524=ORIENTED_EDGE('',*,*,#9440,.F.);
#13525=ORIENTED_EDGE('',*,*,#9443,.F.);
#13526=ORIENTED_EDGE('',*,*,#9453,.F.);
#13527=ORIENTED_EDGE('',*,*,#9456,.F.);
#13528=ORIENTED_EDGE('',*,*,#9466,.F.);
#13529=ORIENTED_EDGE('',*,*,#9468,.F.);
#13530=ORIENTED_EDGE('',*,*,#9377,.F.);
#13531=ORIENTED_EDGE('',*,*,#9380,.F.);
#13532=ORIENTED_EDGE('',*,*,#9364,.F.);
#13533=ORIENTED_EDGE('',*,*,#9367,.F.);
#13534=ORIENTED_EDGE('',*,*,#9351,.F.);
#13535=ORIENTED_EDGE('',*,*,#9354,.F.);
#13536=ORIENTED_EDGE('',*,*,#9338,.F.);
#13537=ORIENTED_EDGE('',*,*,#9341,.F.);
#13538=ORIENTED_EDGE('',*,*,#9324,.F.);
#13539=ORIENTED_EDGE('',*,*,#9328,.F.);
#13540=ORIENTED_EDGE('',*,*,#9390,.F.);
#13541=ORIENTED_EDGE('',*,*,#9371,.F.);
#13542=ORIENTED_EDGE('',*,*,#10009,.F.);
#13543=ORIENTED_EDGE('',*,*,#9361,.F.);
#13544=ORIENTED_EDGE('',*,*,#9379,.F.);
#13545=ORIENTED_EDGE('',*,*,#9358,.F.);
#13546=ORIENTED_EDGE('',*,*,#10010,.F.);
#13547=ORIENTED_EDGE('',*,*,#9348,.F.);
#13548=ORIENTED_EDGE('',*,*,#9366,.F.);
#13549=ORIENTED_EDGE('',*,*,#9345,.F.);
#13550=ORIENTED_EDGE('',*,*,#10011,.F.);
#13551=ORIENTED_EDGE('',*,*,#9335,.F.);
#13552=ORIENTED_EDGE('',*,*,#9353,.F.);
#13553=ORIENTED_EDGE('',*,*,#9332,.F.);
#13554=ORIENTED_EDGE('',*,*,#10012,.F.);
#13555=ORIENTED_EDGE('',*,*,#9321,.F.);
#13556=ORIENTED_EDGE('',*,*,#9340,.F.);
#13557=ORIENTED_EDGE('',*,*,#9318,.F.);
#13558=ORIENTED_EDGE('',*,*,#10013,.F.);
#13559=ORIENTED_EDGE('',*,*,#9387,.F.);
#13560=ORIENTED_EDGE('',*,*,#9326,.F.);
#13561=ORIENTED_EDGE('',*,*,#9460,.F.);
#13562=ORIENTED_EDGE('',*,*,#10014,.F.);
#13563=ORIENTED_EDGE('',*,*,#9374,.F.);
#13564=ORIENTED_EDGE('',*,*,#9467,.F.);
#13565=ORIENTED_EDGE('',*,*,#9169,.F.);
#13566=ORIENTED_EDGE('',*,*,#9401,.T.);
#13567=ORIENTED_EDGE('',*,*,#10008,.T.);
#13568=ORIENTED_EDGE('',*,*,#9383,.F.);
#13569=ORIENTED_EDGE('',*,*,#9388,.T.);
#13570=ORIENTED_EDGE('',*,*,#10013,.T.);
#13571=ORIENTED_EDGE('',*,*,#9317,.F.);
#13572=ORIENTED_EDGE('',*,*,#9322,.T.);
#13573=ORIENTED_EDGE('',*,*,#10012,.T.);
#13574=ORIENTED_EDGE('',*,*,#9331,.F.);
#13575=ORIENTED_EDGE('',*,*,#9336,.T.);
#13576=ORIENTED_EDGE('',*,*,#10011,.T.);
#13577=ORIENTED_EDGE('',*,*,#9344,.F.);
#13578=ORIENTED_EDGE('',*,*,#9349,.T.);
#13579=ORIENTED_EDGE('',*,*,#10010,.T.);
#13580=ORIENTED_EDGE('',*,*,#9357,.F.);
#13581=ORIENTED_EDGE('',*,*,#9362,.T.);
#13582=ORIENTED_EDGE('',*,*,#10009,.T.);
#13583=ORIENTED_EDGE('',*,*,#9370,.F.);
#13584=ORIENTED_EDGE('',*,*,#9375,.T.);
#13585=ORIENTED_EDGE('',*,*,#10014,.T.);
#13586=ORIENTED_EDGE('',*,*,#9459,.F.);
#13587=ORIENTED_EDGE('',*,*,#9464,.T.);
#13588=ORIENTED_EDGE('',*,*,#10003,.T.);
#13589=ORIENTED_EDGE('',*,*,#9446,.F.);
#13590=ORIENTED_EDGE('',*,*,#9451,.T.);
#13591=ORIENTED_EDGE('',*,*,#10004,.T.);
#13592=ORIENTED_EDGE('',*,*,#9433,.F.);
#13593=ORIENTED_EDGE('',*,*,#9438,.T.);
#13594=ORIENTED_EDGE('',*,*,#10005,.T.);
#13595=ORIENTED_EDGE('',*,*,#9420,.F.);
#13596=ORIENTED_EDGE('',*,*,#9425,.T.);
#13597=ORIENTED_EDGE('',*,*,#10006,.T.);
#13598=ORIENTED_EDGE('',*,*,#9406,.F.);
#13599=ORIENTED_EDGE('',*,*,#9411,.T.);
#13600=ORIENTED_EDGE('',*,*,#10007,.T.);
#13601=ORIENTED_EDGE('',*,*,#9396,.F.);
#13602=ORIENTED_EDGE('',*,*,#10015,.F.);
#13603=ORIENTED_EDGE('',*,*,#10016,.T.);
#13604=ORIENTED_EDGE('',*,*,#9757,.T.);
#13605=ORIENTED_EDGE('',*,*,#10016,.F.);
#13606=ORIENTED_EDGE('',*,*,#9313,.F.);
#13607=ORIENTED_EDGE('',*,*,#10017,.T.);
#13608=ORIENTED_EDGE('',*,*,#10015,.T.);
#13609=ORIENTED_EDGE('',*,*,#10017,.F.);
#13610=ORIENTED_EDGE('',*,*,#9637,.F.);
#13611=ORIENTED_EDGE('',*,*,#10018,.T.);
#13612=ORIENTED_EDGE('',*,*,#9314,.T.);
#13613=ORIENTED_EDGE('',*,*,#10018,.F.);
#13614=ORIENTED_EDGE('',*,*,#10019,.F.);
#13615=ORIENTED_EDGE('',*,*,#10020,.T.);
#13616=ORIENTED_EDGE('',*,*,#9950,.T.);
#13617=ORIENTED_EDGE('',*,*,#10020,.F.);
#13618=ORIENTED_EDGE('',*,*,#10019,.T.);
#13619=ORIENTED_EDGE('',*,*,#10021,.F.);
#13620=ORIENTED_EDGE('',*,*,#10022,.F.);
#13621=ORIENTED_EDGE('',*,*,#10023,.T.);
#13622=ORIENTED_EDGE('',*,*,#10021,.T.);
#13623=ORIENTED_EDGE('',*,*,#10023,.F.);
#13624=ORIENTED_EDGE('',*,*,#10024,.F.);
#13625=ORIENTED_EDGE('',*,*,#10025,.T.);
#13626=ORIENTED_EDGE('',*,*,#10022,.T.);
#13627=ORIENTED_EDGE('',*,*,#10025,.F.);
#13628=ORIENTED_EDGE('',*,*,#10026,.F.);
#13629=ORIENTED_EDGE('',*,*,#10027,.T.);
#13630=ORIENTED_EDGE('',*,*,#10024,.T.);
#13631=ORIENTED_EDGE('',*,*,#10027,.F.);
#13632=ORIENTED_EDGE('',*,*,#10028,.F.);
#13633=ORIENTED_EDGE('',*,*,#10029,.T.);
#13634=ORIENTED_EDGE('',*,*,#10026,.T.);
#13635=ORIENTED_EDGE('',*,*,#10029,.F.);
#13636=ORIENTED_EDGE('',*,*,#10028,.T.);
#13637=ORIENTED_EDGE('',*,*,#10030,.F.);
#13638=ORIENTED_EDGE('',*,*,#10031,.F.);
#13639=ORIENTED_EDGE('',*,*,#10032,.T.);
#13640=ORIENTED_EDGE('',*,*,#10030,.T.);
#13641=ORIENTED_EDGE('',*,*,#10032,.F.);
#13642=ORIENTED_EDGE('',*,*,#10033,.F.);
#13643=ORIENTED_EDGE('',*,*,#10034,.T.);
#13644=ORIENTED_EDGE('',*,*,#10031,.T.);
#13645=ORIENTED_EDGE('',*,*,#10034,.F.);
#13646=ORIENTED_EDGE('',*,*,#10035,.F.);
#13647=ORIENTED_EDGE('',*,*,#10036,.T.);
#13648=ORIENTED_EDGE('',*,*,#10033,.T.);
#13649=ORIENTED_EDGE('',*,*,#10036,.F.);
#13650=ORIENTED_EDGE('',*,*,#10037,.F.);
#13651=ORIENTED_EDGE('',*,*,#10038,.T.);
#13652=ORIENTED_EDGE('',*,*,#10035,.T.);
#13653=ORIENTED_EDGE('',*,*,#10038,.F.);
#13654=ORIENTED_EDGE('',*,*,#10039,.F.);
#13655=ORIENTED_EDGE('',*,*,#10040,.T.);
#13656=ORIENTED_EDGE('',*,*,#10037,.T.);
#13657=ORIENTED_EDGE('',*,*,#10040,.F.);
#13658=ORIENTED_EDGE('',*,*,#9898,.F.);
#13659=ORIENTED_EDGE('',*,*,#9117,.F.);
#13660=ORIENTED_EDGE('',*,*,#9899,.F.);
#13661=ORIENTED_EDGE('',*,*,#10041,.T.);
#13662=ORIENTED_EDGE('',*,*,#10039,.T.);
#13663=ORIENTED_EDGE('',*,*,#10041,.F.);
#13664=ORIENTED_EDGE('',*,*,#9161,.T.);
#13665=ORIENTED_EDGE('',*,*,#9895,.T.);
#13666=ORIENTED_EDGE('',*,*,#10042,.F.);
#13667=ORIENTED_EDGE('',*,*,#9903,.T.);
#13668=ORIENTED_EDGE('',*,*,#10043,.F.);
#13669=ORIENTED_EDGE('',*,*,#10044,.T.);
#13670=ORIENTED_EDGE('',*,*,#9892,.T.);
#13671=ORIENTED_EDGE('',*,*,#10042,.T.);
#13672=ORIENTED_EDGE('',*,*,#9893,.T.);
#13673=ORIENTED_EDGE('',*,*,#10044,.F.);
#13674=ORIENTED_EDGE('',*,*,#10043,.T.);
#17215=CYLINDRICAL_SURFACE('',#18420,3.442);
#17216=CYLINDRICAL_SURFACE('',#18422,3.442);
#17217=CYLINDRICAL_SURFACE('',#18423,3.442);
#17218=CYLINDRICAL_SURFACE('',#18424,3.442);
#17219=CYLINDRICAL_SURFACE('',#18425,3.442);
#17220=CYLINDRICAL_SURFACE('',#18426,3.442);
#17221=CYLINDRICAL_SURFACE('',#18427,3.442);
#17222=CYLINDRICAL_SURFACE('',#18428,3.442);
#17223=CYLINDRICAL_SURFACE('',#18429,3.442);
#17224=CYLINDRICAL_SURFACE('',#18430,3.442);
#17225=CYLINDRICAL_SURFACE('',#18431,3.442);
#17226=CYLINDRICAL_SURFACE('',#18432,3.442);
#17227=CYLINDRICAL_SURFACE('',#18433,3.442);
#17228=CYLINDRICAL_SURFACE('',#18434,3.442);
#17229=CYLINDRICAL_SURFACE('',#18435,3.442);
#17230=CYLINDRICAL_SURFACE('',#18436,3.442);
#17231=CYLINDRICAL_SURFACE('',#18460,2.872);
#17232=CYLINDRICAL_SURFACE('',#18462,2.872);
#17233=CYLINDRICAL_SURFACE('',#18463,2.872);
#17234=CYLINDRICAL_SURFACE('',#18464,2.872);
#17235=CYLINDRICAL_SURFACE('',#18465,2.872);
#17236=CYLINDRICAL_SURFACE('',#18466,2.872);
#17237=CYLINDRICAL_SURFACE('',#18467,2.872);
#17238=CYLINDRICAL_SURFACE('',#18468,2.872);
#17239=CYLINDRICAL_SURFACE('',#18469,2.872);
#17240=CYLINDRICAL_SURFACE('',#18470,2.872);
#17241=CYLINDRICAL_SURFACE('',#18471,2.872);
#17242=CYLINDRICAL_SURFACE('',#18472,2.872);
#17243=CYLINDRICAL_SURFACE('',#18473,2.872);
#17244=CYLINDRICAL_SURFACE('',#18474,2.872);
#17245=CYLINDRICAL_SURFACE('',#18475,2.872);
#17246=CYLINDRICAL_SURFACE('',#18476,2.872);
#17247=CYLINDRICAL_SURFACE('',#18535,35.);
#17248=CYLINDRICAL_SURFACE('',#18540,35.);
#17249=CYLINDRICAL_SURFACE('',#18545,35.);
#17250=CYLINDRICAL_SURFACE('',#18550,35.);
#17251=CYLINDRICAL_SURFACE('',#18555,35.);
#17252=CYLINDRICAL_SURFACE('',#18560,35.);
#17253=CYLINDRICAL_SURFACE('',#18565,35.);
#17254=CYLINDRICAL_SURFACE('',#18570,35.);
#17255=CYLINDRICAL_SURFACE('',#18575,35.);
#17256=CYLINDRICAL_SURFACE('',#18580,35.);
#17257=CYLINDRICAL_SURFACE('',#18585,35.);
#17258=CYLINDRICAL_SURFACE('',#18590,35.);
#17259=CYLINDRICAL_SURFACE('',#18597,9.2);
#17260=CYLINDRICAL_SURFACE('',#18604,9.2);
#17261=CYLINDRICAL_SURFACE('',#18613,33.);
#17262=CYLINDRICAL_SURFACE('',#18625,33.);
#17263=CYLINDRICAL_SURFACE('',#18637,33.);
#17264=CYLINDRICAL_SURFACE('',#18649,33.);
#17265=CYLINDRICAL_SURFACE('',#18661,33.);
#17266=CYLINDRICAL_SURFACE('',#18687,8.);
#17267=CYLINDRICAL_SURFACE('',#18689,8.);
#17268=CYLINDRICAL_SURFACE('',#18692,33.);
#17269=CYLINDRICAL_SURFACE('',#18702,33.);
#17270=CYLINDRICAL_SURFACE('',#18712,33.);
#17271=CYLINDRICAL_SURFACE('',#18722,33.);
#17272=CYLINDRICAL_SURFACE('',#18732,33.);
#17273=CYLINDRICAL_SURFACE('',#18742,33.);
#17274=CYLINDRICAL_SURFACE('',#18748,33.);
#17275=CYLINDRICAL_SURFACE('',#18758,8.);
#17276=CYLINDRICAL_SURFACE('',#18767,2.872);
#17277=CYLINDRICAL_SURFACE('',#18773,8.);
#17278=CYLINDRICAL_SURFACE('',#18778,8.);
#17279=CYLINDRICAL_SURFACE('',#18783,8.);
#17280=CYLINDRICAL_SURFACE('',#18788,8.);
#17281=CYLINDRICAL_SURFACE('',#18793,8.);
#17282=CYLINDRICAL_SURFACE('',#18798,8.);
#17283=CYLINDRICAL_SURFACE('',#18803,8.);
#17284=CYLINDRICAL_SURFACE('',#18808,8.);
#17285=CYLINDRICAL_SURFACE('',#18813,8.);
#17286=CYLINDRICAL_SURFACE('',#18822,8.5);
#17287=CYLINDRICAL_SURFACE('',#18828,9.2);
#17288=CYLINDRICAL_SURFACE('',#18830,7.7);
#17289=CYLINDRICAL_SURFACE('',#18894,5.5);
#17290=CYLINDRICAL_SURFACE('',#18900,3.3);
#17291=CYLINDRICAL_SURFACE('',#18904,3.5);
#17292=CYLINDRICAL_SURFACE('',#18908,2.9);
#17293=CYLINDRICAL_SURFACE('',#18911,3.442);
#17333=ADVANCED_FACE('',(#1305),#17215,.T.);
#17334=ADVANCED_FACE('',(#1306),#17216,.T.);
#17335=ADVANCED_FACE('',(#1307),#17217,.T.);
#17336=ADVANCED_FACE('',(#1308),#17218,.T.);
#17337=ADVANCED_FACE('',(#1309),#17219,.T.);
#17338=ADVANCED_FACE('',(#1310),#17220,.T.);
#17339=ADVANCED_FACE('',(#1311),#17221,.T.);
#17340=ADVANCED_FACE('',(#1312),#17222,.T.);
#17341=ADVANCED_FACE('',(#1313),#17223,.T.);
#17342=ADVANCED_FACE('',(#1314),#17224,.T.);
#17343=ADVANCED_FACE('',(#1315),#17225,.T.);
#17344=ADVANCED_FACE('',(#1316),#17226,.T.);
#17345=ADVANCED_FACE('',(#1317),#17227,.T.);
#17346=ADVANCED_FACE('',(#1318),#17228,.T.);
#17347=ADVANCED_FACE('',(#1319),#17229,.T.);
#17348=ADVANCED_FACE('',(#1320),#17230,.T.);
#17349=ADVANCED_FACE('',(#1321),#1064,.T.);
#17350=ADVANCED_FACE('',(#1322),#17231,.T.);
#17351=ADVANCED_FACE('',(#1323),#17232,.T.);
#17352=ADVANCED_FACE('',(#1324),#17233,.T.);
#17353=ADVANCED_FACE('',(#1325),#17234,.T.);
#17354=ADVANCED_FACE('',(#1326),#17235,.T.);
#17355=ADVANCED_FACE('',(#1327),#17236,.T.);
#17356=ADVANCED_FACE('',(#1328),#17237,.T.);
#17357=ADVANCED_FACE('',(#1329),#17238,.T.);
#17358=ADVANCED_FACE('',(#1330),#17239,.T.);
#17359=ADVANCED_FACE('',(#1331),#17240,.T.);
#17360=ADVANCED_FACE('',(#1332),#17241,.T.);
#17361=ADVANCED_FACE('',(#1333),#17242,.T.);
#17362=ADVANCED_FACE('',(#1334),#17243,.T.);
#17363=ADVANCED_FACE('',(#1335),#17244,.T.);
#17364=ADVANCED_FACE('',(#1336),#17245,.T.);
#17365=ADVANCED_FACE('',(#1337),#17246,.T.);
#17366=ADVANCED_FACE('',(#1338),#827,.T.);
#17367=ADVANCED_FACE('',(#1339),#828,.T.);
#17368=ADVANCED_FACE('',(#1340,#197),#264,.T.);
#17369=ADVANCED_FACE('',(#1341),#265,.T.);
#17370=ADVANCED_FACE('',(#1342),#266,.T.);
#17371=ADVANCED_FACE('',(#1343),#267,.T.);
#17372=ADVANCED_FACE('',(#1344),#268,.T.);
#17373=ADVANCED_FACE('',(#1345),#269,.T.);
#17374=ADVANCED_FACE('',(#1346),#270,.T.);
#17375=ADVANCED_FACE('',(#1347),#271,.T.);
#17376=ADVANCED_FACE('',(#1348),#272,.T.);
#17377=ADVANCED_FACE('',(#1349),#273,.T.);
#17378=ADVANCED_FACE('',(#1350),#274,.T.);
#17379=ADVANCED_FACE('',(#1351),#275,.T.);
#17380=ADVANCED_FACE('',(#1352),#276,.T.);
#17381=ADVANCED_FACE('',(#1353),#277,.T.);
#17382=ADVANCED_FACE('',(#1354),#278,.T.);
#17383=ADVANCED_FACE('',(#1355),#279,.T.);
#17384=ADVANCED_FACE('',(#1356),#280,.T.);
#17385=ADVANCED_FACE('',(#1357),#281,.T.);
#17386=ADVANCED_FACE('',(#1358),#282,.T.);
#17387=ADVANCED_FACE('',(#1359),#283,.T.);
#17388=ADVANCED_FACE('',(#1360),#284,.T.);
#17389=ADVANCED_FACE('',(#1361),#285,.T.);
#17390=ADVANCED_FACE('',(#1362),#286,.T.);
#17391=ADVANCED_FACE('',(#1363),#287,.T.);
#17392=ADVANCED_FACE('',(#1364),#288,.T.);
#17393=ADVANCED_FACE('',(#1365),#289,.T.);
#17394=ADVANCED_FACE('',(#1366),#290,.T.);
#17395=ADVANCED_FACE('',(#1367),#291,.T.);
#17396=ADVANCED_FACE('',(#1368),#292,.T.);
#17397=ADVANCED_FACE('',(#1369),#293,.T.);
#17398=ADVANCED_FACE('',(#1370),#294,.T.);
#17399=ADVANCED_FACE('',(#1371),#295,.T.);
#17400=ADVANCED_FACE('',(#1372),#296,.T.);
#17401=ADVANCED_FACE('',(#1373),#297,.T.);
#17402=ADVANCED_FACE('',(#1374),#298,.T.);
#17403=ADVANCED_FACE('',(#1375),#299,.T.);
#17404=ADVANCED_FACE('',(#1376),#300,.T.);
#17405=ADVANCED_FACE('',(#1377),#301,.T.);
#17406=ADVANCED_FACE('',(#1378),#302,.T.);
#17407=ADVANCED_FACE('',(#1379),#303,.T.);
#17408=ADVANCED_FACE('',(#1380),#304,.T.);
#17409=ADVANCED_FACE('',(#1381),#305,.T.);
#17410=ADVANCED_FACE('',(#1382),#306,.T.);
#17411=ADVANCED_FACE('',(#1383),#307,.T.);
#17412=ADVANCED_FACE('',(#1384),#308,.T.);
#17413=ADVANCED_FACE('',(#1385),#309,.T.);
#17414=ADVANCED_FACE('',(#1386),#310,.T.);
#17415=ADVANCED_FACE('',(#1387),#311,.T.);
#17416=ADVANCED_FACE('',(#1388),#829,.T.);
#17417=ADVANCED_FACE('',(#1389),#17247,.T.);
#17418=ADVANCED_FACE('',(#1390),#97,.T.);
#17419=ADVANCED_FACE('',(#1391),#830,.T.);
#17420=ADVANCED_FACE('',(#1392),#17248,.T.);
#17421=ADVANCED_FACE('',(#1393),#98,.T.);
#17422=ADVANCED_FACE('',(#1394),#831,.T.);
#17423=ADVANCED_FACE('',(#1395),#17249,.T.);
#17424=ADVANCED_FACE('',(#1396),#99,.T.);
#17425=ADVANCED_FACE('',(#1397),#832,.T.);
#17426=ADVANCED_FACE('',(#1398),#17250,.T.);
#17427=ADVANCED_FACE('',(#1399),#100,.T.);
#17428=ADVANCED_FACE('',(#1400),#833,.T.);
#17429=ADVANCED_FACE('',(#1401),#17251,.T.);
#17430=ADVANCED_FACE('',(#1402),#101,.T.);
#17431=ADVANCED_FACE('',(#1403),#834,.T.);
#17432=ADVANCED_FACE('',(#1404),#17252,.T.);
#17433=ADVANCED_FACE('',(#1405),#102,.T.);
#17434=ADVANCED_FACE('',(#1406),#835,.T.);
#17435=ADVANCED_FACE('',(#1407),#17253,.T.);
#17436=ADVANCED_FACE('',(#1408),#103,.T.);
#17437=ADVANCED_FACE('',(#1409),#836,.T.);
#17438=ADVANCED_FACE('',(#1410),#17254,.T.);
#17439=ADVANCED_FACE('',(#1411),#104,.T.);
#17440=ADVANCED_FACE('',(#1412),#837,.T.);
#17441=ADVANCED_FACE('',(#1413),#17255,.T.);
#17442=ADVANCED_FACE('',(#1414),#105,.T.);
#17443=ADVANCED_FACE('',(#1415),#838,.T.);
#17444=ADVANCED_FACE('',(#1416),#17256,.T.);
#17445=ADVANCED_FACE('',(#1417),#106,.T.);
#17446=ADVANCED_FACE('',(#1418),#839,.T.);
#17447=ADVANCED_FACE('',(#1419),#17257,.T.);
#17448=ADVANCED_FACE('',(#1420),#107,.T.);
#17449=ADVANCED_FACE('',(#1421),#840,.T.);
#17450=ADVANCED_FACE('',(#1422),#17258,.T.);
#17451=ADVANCED_FACE('',(#1423),#108,.T.);
#17452=ADVANCED_FACE('',(#1424),#841,.T.);
#17453=ADVANCED_FACE('',(#1425,#198),#312,.F.);
#17454=ADVANCED_FACE('',(#1426),#17259,.T.);
#17455=ADVANCED_FACE('',(#1427),#842,.T.);
#17456=ADVANCED_FACE('',(#1428,#199),#313,.F.);
#17457=ADVANCED_FACE('',(#1429),#17260,.T.);
#17458=ADVANCED_FACE('',(#1430),#314,.T.);
#17459=ADVANCED_FACE('',(#1431),#843,.F.);
#17460=ADVANCED_FACE('',(#1432),#844,.T.);
#17461=ADVANCED_FACE('',(#1433),#17261,.T.);
#17462=ADVANCED_FACE('',(#1434),#315,.T.);
#17463=ADVANCED_FACE('',(#1435),#845,.F.);
#17464=ADVANCED_FACE('',(#1436),#316,.T.);
#17465=ADVANCED_FACE('',(#1437),#846,.T.);
#17466=ADVANCED_FACE('',(#1438),#17262,.T.);
#17467=ADVANCED_FACE('',(#1439),#317,.T.);
#17468=ADVANCED_FACE('',(#1440),#847,.F.);
#17469=ADVANCED_FACE('',(#1441),#318,.T.);
#17470=ADVANCED_FACE('',(#1442),#848,.T.);
#17471=ADVANCED_FACE('',(#1443),#17263,.T.);
#17472=ADVANCED_FACE('',(#1444),#319,.T.);
#17473=ADVANCED_FACE('',(#1445),#849,.F.);
#17474=ADVANCED_FACE('',(#1446),#320,.T.);
#17475=ADVANCED_FACE('',(#1447),#850,.T.);
#17476=ADVANCED_FACE('',(#1448),#17264,.T.);
#17477=ADVANCED_FACE('',(#1449),#321,.T.);
#17478=ADVANCED_FACE('',(#1450),#851,.F.);
#17479=ADVANCED_FACE('',(#1451),#322,.T.);
#17480=ADVANCED_FACE('',(#1452),#852,.T.);
#17481=ADVANCED_FACE('',(#1453),#17265,.T.);
#17482=ADVANCED_FACE('',(#1454),#323,.T.);
#17483=ADVANCED_FACE('',(#1455),#853,.F.);
#17484=ADVANCED_FACE('',(#1456,#200),#324,.T.);
#17485=ADVANCED_FACE('',(#1457),#854,.T.);
#17486=ADVANCED_FACE('',(#1458),#325,.T.);
#17487=ADVANCED_FACE('',(#1459),#17266,.F.);
#17488=ADVANCED_FACE('',(#1460),#17267,.F.);
#17489=ADVANCED_FACE('',(#1461),#326,.T.);
#17490=ADVANCED_FACE('',(#1462),#17268,.T.);
#17491=ADVANCED_FACE('',(#1463),#327,.T.);
#17492=ADVANCED_FACE('',(#1464),#855,.F.);
#17493=ADVANCED_FACE('',(#1465),#856,.T.);
#17494=ADVANCED_FACE('',(#1466),#328,.T.);
#17495=ADVANCED_FACE('',(#1467),#17269,.T.);
#17496=ADVANCED_FACE('',(#1468),#329,.T.);
#17497=ADVANCED_FACE('',(#1469),#857,.F.);
#17498=ADVANCED_FACE('',(#1470),#858,.T.);
#17499=ADVANCED_FACE('',(#1471),#330,.T.);
#17500=ADVANCED_FACE('',(#1472),#17270,.T.);
#17501=ADVANCED_FACE('',(#1473),#331,.T.);
#17502=ADVANCED_FACE('',(#1474),#859,.F.);
#17503=ADVANCED_FACE('',(#1475),#860,.T.);
#17504=ADVANCED_FACE('',(#1476),#332,.T.);
#17505=ADVANCED_FACE('',(#1477),#17271,.T.);
#17506=ADVANCED_FACE('',(#1478),#333,.T.);
#17507=ADVANCED_FACE('',(#1479),#861,.F.);
#17508=ADVANCED_FACE('',(#1480),#862,.T.);
#17509=ADVANCED_FACE('',(#1481),#334,.T.);
#17510=ADVANCED_FACE('',(#1482),#17272,.T.);
#17511=ADVANCED_FACE('',(#1483),#335,.T.);
#17512=ADVANCED_FACE('',(#1484),#863,.F.);
#17513=ADVANCED_FACE('',(#1485),#864,.T.);
#17514=ADVANCED_FACE('',(#1486),#336,.T.);
#17515=ADVANCED_FACE('',(#1487),#17273,.T.);
#17516=ADVANCED_FACE('',(#1488),#865,.T.);
#17517=ADVANCED_FACE('',(#1489),#17274,.T.);
#17518=ADVANCED_FACE('',(#1490),#337,.T.);
#17519=ADVANCED_FACE('',(#1491),#866,.F.);
#17520=ADVANCED_FACE('',(#1492),#338,.T.);
#17521=ADVANCED_FACE('',(#1493),#867,.T.);
#17522=ADVANCED_FACE('',(#1494),#17275,.F.);
#17523=ADVANCED_FACE('',(#1495),#339,.F.);
#17524=ADVANCED_FACE('',(#1496),#109,.F.);
#17525=ADVANCED_FACE('',(#1497),#340,.T.);
#17526=ADVANCED_FACE('',(#1498),#17276,.T.);
#17527=ADVANCED_FACE('',(#1499),#110,.F.);
#17528=ADVANCED_FACE('',(#1500),#341,.T.);
#17529=ADVANCED_FACE('',(#1501),#1065,.T.);
#17530=ADVANCED_FACE('',(#1502),#868,.T.);
#17531=ADVANCED_FACE('',(#1503),#342,.T.);
#17532=ADVANCED_FACE('',(#1504),#17277,.F.);
#17533=ADVANCED_FACE('',(#1505),#869,.T.);
#17534=ADVANCED_FACE('',(#1506),#870,.T.);
#17535=ADVANCED_FACE('',(#1507),#343,.T.);
#17536=ADVANCED_FACE('',(#1508),#17278,.F.);
#17537=ADVANCED_FACE('',(#1509),#871,.T.);
#17538=ADVANCED_FACE('',(#1510),#872,.T.);
#17539=ADVANCED_FACE('',(#1511),#344,.T.);
#17540=ADVANCED_FACE('',(#1512),#17279,.F.);
#17541=ADVANCED_FACE('',(#1513),#873,.T.);
#17542=ADVANCED_FACE('',(#1514),#874,.T.);
#17543=ADVANCED_FACE('',(#1515),#345,.T.);
#17544=ADVANCED_FACE('',(#1516),#17280,.F.);
#17545=ADVANCED_FACE('',(#1517),#875,.T.);
#17546=ADVANCED_FACE('',(#1518),#876,.T.);
#17547=ADVANCED_FACE('',(#1519),#346,.T.);
#17548=ADVANCED_FACE('',(#1520),#17281,.F.);
#17549=ADVANCED_FACE('',(#1521),#877,.T.);
#17550=ADVANCED_FACE('',(#1522),#878,.T.);
#17551=ADVANCED_FACE('',(#1523),#347,.T.);
#17552=ADVANCED_FACE('',(#1524),#17282,.F.);
#17553=ADVANCED_FACE('',(#1525),#879,.T.);
#17554=ADVANCED_FACE('',(#1526),#880,.T.);
#17555=ADVANCED_FACE('',(#1527),#348,.T.);
#17556=ADVANCED_FACE('',(#1528),#17283,.F.);
#17557=ADVANCED_FACE('',(#1529),#881,.T.);
#17558=ADVANCED_FACE('',(#1530),#882,.T.);
#17559=ADVANCED_FACE('',(#1531),#349,.T.);
#17560=ADVANCED_FACE('',(#1532),#17284,.F.);
#17561=ADVANCED_FACE('',(#1533),#883,.T.);
#17562=ADVANCED_FACE('',(#1534),#884,.T.);
#17563=ADVANCED_FACE('',(#1535),#350,.T.);
#17564=ADVANCED_FACE('',(#1536),#17285,.F.);
#17565=ADVANCED_FACE('',(#1537),#885,.T.);
#17566=ADVANCED_FACE('',(#1538),#886,.T.);
#17567=ADVANCED_FACE('',(#1539),#351,.T.);
#17568=ADVANCED_FACE('',(#1540),#887,.T.);
#17569=ADVANCED_FACE('',(#1541),#888,.T.);
#17570=ADVANCED_FACE('',(#1542),#352,.T.);
#17571=ADVANCED_FACE('',(#1543),#889,.T.);
#17572=ADVANCED_FACE('',(#1544),#890,.T.);
#17573=ADVANCED_FACE('',(#1545),#17286,.T.);
#17574=ADVANCED_FACE('',(#1546,#201),#353,.F.);
#17575=ADVANCED_FACE('',(#1547,#202),#354,.F.);
#17576=ADVANCED_FACE('',(#1548),#17287,.T.);
#17577=ADVANCED_FACE('',(#1549),#17288,.T.);
#17578=ADVANCED_FACE('',(#1550),#355,.T.);
#17579=ADVANCED_FACE('',(#1551),#356,.T.);
#17580=ADVANCED_FACE('',(#1552),#1066,.T.);
#17581=ADVANCED_FACE('',(#1553),#111,.F.);
#17582=ADVANCED_FACE('',(#1554),#357,.T.);
#17583=ADVANCED_FACE('',(#1555),#358,.T.);
#17584=ADVANCED_FACE('',(#1556),#1067,.T.);
#17585=ADVANCED_FACE('',(#1557),#112,.F.);
#17586=ADVANCED_FACE('',(#1558),#359,.T.);
#17587=ADVANCED_FACE('',(#1559),#360,.T.);
#17588=ADVANCED_FACE('',(#1560),#1068,.T.);
#17589=ADVANCED_FACE('',(#1561),#113,.F.);
#17590=ADVANCED_FACE('',(#1562),#361,.T.);
#17591=ADVANCED_FACE('',(#1563),#362,.T.);
#17592=ADVANCED_FACE('',(#1564),#1069,.T.);
#17593=ADVANCED_FACE('',(#1565),#114,.F.);
#17594=ADVANCED_FACE('',(#1566),#363,.T.);
#17595=ADVANCED_FACE('',(#1567),#364,.T.);
#17596=ADVANCED_FACE('',(#1568),#1070,.T.);
#17597=ADVANCED_FACE('',(#1569),#115,.F.);
#17598=ADVANCED_FACE('',(#1570),#365,.T.);
#17599=ADVANCED_FACE('',(#1571),#366,.T.);
#17600=ADVANCED_FACE('',(#1572),#1071,.T.);
#17601=ADVANCED_FACE('',(#1573),#116,.F.);
#17602=ADVANCED_FACE('',(#1574),#367,.T.);
#17603=ADVANCED_FACE('',(#1575),#368,.T.);
#17604=ADVANCED_FACE('',(#1576),#1072,.T.);
#17605=ADVANCED_FACE('',(#1577),#117,.F.);
#17606=ADVANCED_FACE('',(#1578),#369,.T.);
#17607=ADVANCED_FACE('',(#1579),#370,.T.);
#17608=ADVANCED_FACE('',(#1580),#1073,.T.);
#17609=ADVANCED_FACE('',(#1581),#118,.F.);
#17610=ADVANCED_FACE('',(#1582),#371,.T.);
#17611=ADVANCED_FACE('',(#1583),#372,.T.);
#17612=ADVANCED_FACE('',(#1584),#1074,.T.);
#17613=ADVANCED_FACE('',(#1585),#119,.F.);
#17614=ADVANCED_FACE('',(#1586),#373,.T.);
#17615=ADVANCED_FACE('',(#1587),#374,.T.);
#17616=ADVANCED_FACE('',(#1588),#1075,.T.);
#17617=ADVANCED_FACE('',(#1589),#120,.F.);
#17618=ADVANCED_FACE('',(#1590),#375,.T.);
#17619=ADVANCED_FACE('',(#1591),#376,.T.);
#17620=ADVANCED_FACE('',(#1592),#1076,.T.);
#17621=ADVANCED_FACE('',(#1593),#121,.F.);
#17622=ADVANCED_FACE('',(#1594),#377,.T.);
#17623=ADVANCED_FACE('',(#1595),#378,.T.);
#17624=ADVANCED_FACE('',(#1596),#1077,.T.);
#17625=ADVANCED_FACE('',(#1597),#122,.F.);
#17626=ADVANCED_FACE('',(#1598),#379,.T.);
#17627=ADVANCED_FACE('',(#1599),#380,.T.);
#17628=ADVANCED_FACE('',(#1600),#381,.T.);
#17629=ADVANCED_FACE('',(#1601),#382,.T.);
#17630=ADVANCED_FACE('',(#1602),#383,.T.);
#17631=ADVANCED_FACE('',(#1603),#384,.T.);
#17632=ADVANCED_FACE('',(#1604),#385,.T.);
#17633=ADVANCED_FACE('',(#1605),#386,.F.);
#17634=ADVANCED_FACE('',(#1606),#387,.T.);
#17635=ADVANCED_FACE('',(#1607),#388,.T.);
#17636=ADVANCED_FACE('',(#1608),#389,.T.);
#17637=ADVANCED_FACE('',(#1609),#390,.T.);
#17638=ADVANCED_FACE('',(#1610),#391,.T.);
#17639=ADVANCED_FACE('',(#1611),#392,.T.);
#17640=ADVANCED_FACE('',(#1612,#203),#393,.T.);
#17641=ADVANCED_FACE('',(#1613),#891,.T.);
#17642=ADVANCED_FACE('',(#1614),#892,.T.);
#17643=ADVANCED_FACE('',(#1615),#893,.T.);
#17644=ADVANCED_FACE('',(#1616),#894,.T.);
#17645=ADVANCED_FACE('',(#1617,#204),#394,.T.);
#17646=ADVANCED_FACE('',(#1618),#895,.T.);
#17647=ADVANCED_FACE('',(#1619),#896,.T.);
#17648=ADVANCED_FACE('',(#1620),#17289,.T.);
#17649=ADVANCED_FACE('',(#1621),#897,.T.);
#17650=ADVANCED_FACE('',(#1622,#205),#395,.T.);
#17651=ADVANCED_FACE('',(#1623),#17290,.T.);
#17652=ADVANCED_FACE('',(#1624),#898,.T.);
#17653=ADVANCED_FACE('',(#1625),#17291,.T.);
#17654=ADVANCED_FACE('',(#1626),#899,.T.);
#17655=ADVANCED_FACE('',(#1627),#17292,.T.);
#17656=ADVANCED_FACE('',(#1628),#900,.T.);
#17657=ADVANCED_FACE('',(#1629),#17293,.T.);
#17658=ADVANCED_FACE('',(#1630),#901,.T.);
#17659=ADVANCED_FACE('',(#1631),#396,.T.);
#18297=CLOSED_SHELL('',(#17333,#17334,#17335,#17336,#17337,#17338,#17339,
#17340,#17341,#17342,#17343,#17344,#17345,#17346,#17347,#17348,#17349,#17350,
#17351,#17352,#17353,#17354,#17355,#17356,#17357,#17358,#17359,#17360,#17361,
#17362,#17363,#17364,#17365,#17366,#17367,#17368,#17369,#17370,#17371,#17372,
#17373,#17374,#17375,#17376,#17377,#17378,#17379,#17380,#17381,#17382,#17383,
#17384,#17385,#17386,#17387,#17388,#17389,#17390,#17391,#17392,#17393,#17394,
#17395,#17396,#17397,#17398,#17399,#17400,#17401,#17402,#17403,#17404,#17405,
#17406,#17407,#17408,#17409,#17410,#17411,#17412,#17413,#17414,#17415,#17416,
#17417,#17418,#17419,#17420,#17421,#17422,#17423,#17424,#17425,#17426,#17427,
#17428,#17429,#17430,#17431,#17432,#17433,#17434,#17435,#17436,#17437,#17438,
#17439,#17440,#17441,#17442,#17443,#17444,#17445,#17446,#17447,#17448,#17449,
#17450,#17451,#17452,#17453,#17454,#17455,#17456,#17457,#17458,#17459,#17460,
#17461,#17462,#17463,#17464,#17465,#17466,#17467,#17468,#17469,#17470,#17471,
#17472,#17473,#17474,#17475,#17476,#17477,#17478,#17479,#17480,#17481,#17482,
#17483,#17484,#17485,#17486,#17487,#17488,#17489,#17490,#17491,#17492,#17493,
#17494,#17495,#17496,#17497,#17498,#17499,#17500,#17501,#17502,#17503,#17504,
#17505,#17506,#17507,#17508,#17509,#17510,#17511,#17512,#17513,#17514,#17515,
#17516,#17517,#17518,#17519,#17520,#17521,#17522,#17523,#17524,#17525,#17526,
#17527,#17528,#17529,#17530,#17531,#17532,#17533,#17534,#17535,#17536,#17537,
#17538,#17539,#17540,#17541,#17542,#17543,#17544,#17545,#17546,#17547,#17548,
#17549,#17550,#17551,#17552,#17553,#17554,#17555,#17556,#17557,#17558,#17559,
#17560,#17561,#17562,#17563,#17564,#17565,#17566,#17567,#17568,#17569,#17570,
#17571,#17572,#17573,#17574,#17575,#17576,#17577,#17578,#17579,#17580,#17581,
#17582,#17583,#17584,#17585,#17586,#17587,#17588,#17589,#17590,#17591,#17592,
#17593,#17594,#17595,#17596,#17597,#17598,#17599,#17600,#17601,#17602,#17603,
#17604,#17605,#17606,#17607,#17608,#17609,#17610,#17611,#17612,#17613,#17614,
#17615,#17616,#17617,#17618,#17619,#17620,#17621,#17622,#17623,#17624,#17625,
#17626,#17627,#17628,#17629,#17630,#17631,#17632,#17633,#17634,#17635,#17636,
#17637,#17638,#17639,#17640,#17641,#17642,#17643,#17644,#17645,#17646,#17647,
#17648,#17649,#17650,#17651,#17652,#17653,#17654,#17655,#17656,#17657,#17658,
#17659));
#18419=AXIS2_PLACEMENT_3D('',#23611,#19680,#19681);
#18420=AXIS2_PLACEMENT_3D('',#23612,#19682,#19683);
#18421=AXIS2_PLACEMENT_3D('',#23628,#19685,#19686);
#18422=AXIS2_PLACEMENT_3D('',#23636,#19687,#19688);
#18423=AXIS2_PLACEMENT_3D('',#23684,#19690,#19691);
#18424=AXIS2_PLACEMENT_3D('',#23732,#19693,#19694);
#18425=AXIS2_PLACEMENT_3D('',#23786,#19696,#19697);
#18426=AXIS2_PLACEMENT_3D('',#23834,#19699,#19700);
#18427=AXIS2_PLACEMENT_3D('',#23882,#19702,#19703);
#18428=AXIS2_PLACEMENT_3D('',#23936,#19705,#19706);
#18429=AXIS2_PLACEMENT_3D('',#23984,#19708,#19709);
#18430=AXIS2_PLACEMENT_3D('',#24032,#19711,#19712);
#18431=AXIS2_PLACEMENT_3D('',#24086,#19714,#19715);
#18432=AXIS2_PLACEMENT_3D('',#24134,#19717,#19718);
#18433=AXIS2_PLACEMENT_3D('',#24182,#19720,#19721);
#18434=AXIS2_PLACEMENT_3D('',#24236,#19723,#19724);
#18435=AXIS2_PLACEMENT_3D('',#24284,#19726,#19727);
#18436=AXIS2_PLACEMENT_3D('',#24332,#19729,#19730);
#18437=AXIS2_PLACEMENT_3D('',#24702,#19732,#19733);
#18438=AXIS2_PLACEMENT_3D('',#24772,#19734,#19735);
#18439=AXIS2_PLACEMENT_3D('',#24791,#19736,#19737);
#18440=AXIS2_PLACEMENT_3D('',#24942,#19738,#19739);
#18441=AXIS2_PLACEMENT_3D('',#24959,#19740,#19741);
#18442=AXIS2_PLACEMENT_3D('',#25110,#19742,#19743);
#18443=AXIS2_PLACEMENT_3D('',#25129,#19744,#19745);
#18444=AXIS2_PLACEMENT_3D('',#25280,#19746,#19747);
#18445=AXIS2_PLACEMENT_3D('',#25299,#19748,#19749);
#18446=AXIS2_PLACEMENT_3D('',#25450,#19750,#19751);
#18447=AXIS2_PLACEMENT_3D('',#25467,#19752,#19753);
#18448=AXIS2_PLACEMENT_3D('',#25618,#19754,#19755);
#18449=AXIS2_PLACEMENT_3D('',#25637,#19756,#19757);
#18450=AXIS2_PLACEMENT_3D('',#25788,#19758,#19759);
#18451=AXIS2_PLACEMENT_3D('',#25807,#19760,#19761);
#18452=AXIS2_PLACEMENT_3D('',#25958,#19762,#19763);
#18453=AXIS2_PLACEMENT_3D('',#25975,#19764,#19765);
#18454=AXIS2_PLACEMENT_3D('',#26126,#19766,#19767);
#18455=AXIS2_PLACEMENT_3D('',#26145,#19768,#19769);
#18456=AXIS2_PLACEMENT_3D('',#26296,#19770,#19771);
#18457=AXIS2_PLACEMENT_3D('',#26315,#19772,#19773);
#18458=AXIS2_PLACEMENT_3D('',#26466,#19774,#19775);
#18459=AXIS2_PLACEMENT_3D('',#26483,#19776,#19777);
#18460=AXIS2_PLACEMENT_3D('',#26590,#19778,#19779);
#18461=AXIS2_PLACEMENT_3D('',#26602,#19781,#19782);
#18462=AXIS2_PLACEMENT_3D('',#26608,#19783,#19784);
#18463=AXIS2_PLACEMENT_3D('',#26633,#19786,#19787);
#18464=AXIS2_PLACEMENT_3D('',#26658,#19789,#19790);
#18465=AXIS2_PLACEMENT_3D('',#26682,#19792,#19793);
#18466=AXIS2_PLACEMENT_3D('',#26707,#19795,#19796);
#18467=AXIS2_PLACEMENT_3D('',#26732,#19798,#19799);
#18468=AXIS2_PLACEMENT_3D('',#26756,#19801,#19802);
#18469=AXIS2_PLACEMENT_3D('',#26781,#19804,#19805);
#18470=AXIS2_PLACEMENT_3D('',#26806,#19807,#19808);
#18471=AXIS2_PLACEMENT_3D('',#26830,#19810,#19811);
#18472=AXIS2_PLACEMENT_3D('',#26855,#19813,#19814);
#18473=AXIS2_PLACEMENT_3D('',#26880,#19816,#19817);
#18474=AXIS2_PLACEMENT_3D('',#26904,#19819,#19820);
#18475=AXIS2_PLACEMENT_3D('',#26929,#19822,#19823);
#18476=AXIS2_PLACEMENT_3D('',#26954,#19825,#19826);
#18477=AXIS2_PLACEMENT_3D('',#26978,#19828,#19829);
#18478=AXIS2_PLACEMENT_3D('',#26980,#19830,#19831);
#18479=AXIS2_PLACEMENT_3D('',#26984,#19833,#19834);
#18480=AXIS2_PLACEMENT_3D('',#26985,#19835,#19836);
#18481=AXIS2_PLACEMENT_3D('',#26986,#19837,#19838);
#18482=AXIS2_PLACEMENT_3D('',#26989,#19840,#19841);
#18483=AXIS2_PLACEMENT_3D('',#26990,#19842,#19843);
#18484=AXIS2_PLACEMENT_3D('',#26992,#19844,#19845);
#18485=AXIS2_PLACEMENT_3D('',#26993,#19846,#19847);
#18486=AXIS2_PLACEMENT_3D('',#27004,#19853,#19854);
#18487=AXIS2_PLACEMENT_3D('',#27010,#19858,#19859);
#18488=AXIS2_PLACEMENT_3D('',#27016,#19863,#19864);
#18489=AXIS2_PLACEMENT_3D('',#27022,#19868,#19869);
#18490=AXIS2_PLACEMENT_3D('',#27033,#19875,#19876);
#18491=AXIS2_PLACEMENT_3D('',#27039,#19880,#19881);
#18492=AXIS2_PLACEMENT_3D('',#27045,#19885,#19886);
#18493=AXIS2_PLACEMENT_3D('',#27048,#19889,#19890);
#18494=AXIS2_PLACEMENT_3D('',#27059,#19896,#19897);
#18495=AXIS2_PLACEMENT_3D('',#27065,#19901,#19902);
#18496=AXIS2_PLACEMENT_3D('',#27071,#19906,#19907);
#18497=AXIS2_PLACEMENT_3D('',#27074,#19910,#19911);
#18498=AXIS2_PLACEMENT_3D('',#27085,#19917,#19918);
#18499=AXIS2_PLACEMENT_3D('',#27091,#19922,#19923);
#18500=AXIS2_PLACEMENT_3D('',#27097,#19927,#19928);
#18501=AXIS2_PLACEMENT_3D('',#27100,#19931,#19932);
#18502=AXIS2_PLACEMENT_3D('',#27111,#19938,#19939);
#18503=AXIS2_PLACEMENT_3D('',#27117,#19943,#19944);
#18504=AXIS2_PLACEMENT_3D('',#27123,#19948,#19949);
#18505=AXIS2_PLACEMENT_3D('',#27126,#19952,#19953);
#18506=AXIS2_PLACEMENT_3D('',#27137,#19959,#19960);
#18507=AXIS2_PLACEMENT_3D('',#27142,#19964,#19965);
#18508=AXIS2_PLACEMENT_3D('',#27146,#19968,#19969);
#18509=AXIS2_PLACEMENT_3D('',#27152,#19973,#19974);
#18510=AXIS2_PLACEMENT_3D('',#27163,#19980,#19981);
#18511=AXIS2_PLACEMENT_3D('',#27168,#19985,#19986);
#18512=AXIS2_PLACEMENT_3D('',#27172,#19989,#19990);
#18513=AXIS2_PLACEMENT_3D('',#27183,#19996,#19997);
#18514=AXIS2_PLACEMENT_3D('',#27189,#20001,#20002);
#18515=AXIS2_PLACEMENT_3D('',#27195,#20006,#20007);
#18516=AXIS2_PLACEMENT_3D('',#27201,#20011,#20012);
#18517=AXIS2_PLACEMENT_3D('',#27212,#20018,#20019);
#18518=AXIS2_PLACEMENT_3D('',#27217,#20023,#20024);
#18519=AXIS2_PLACEMENT_3D('',#27221,#20027,#20028);
#18520=AXIS2_PLACEMENT_3D('',#27227,#20032,#20033);
#18521=AXIS2_PLACEMENT_3D('',#27238,#20039,#20040);
#18522=AXIS2_PLACEMENT_3D('',#27243,#20044,#20045);
#18523=AXIS2_PLACEMENT_3D('',#27247,#20048,#20049);
#18524=AXIS2_PLACEMENT_3D('',#27253,#20053,#20054);
#18525=AXIS2_PLACEMENT_3D('',#27264,#20060,#20061);
#18526=AXIS2_PLACEMENT_3D('',#27269,#20065,#20066);
#18527=AXIS2_PLACEMENT_3D('',#27273,#20069,#20070);
#18528=AXIS2_PLACEMENT_3D('',#27279,#20074,#20075);
#18529=AXIS2_PLACEMENT_3D('',#27290,#20081,#20082);
#18530=AXIS2_PLACEMENT_3D('',#27295,#20086,#20087);
#18531=AXIS2_PLACEMENT_3D('',#27299,#20090,#20091);
#18532=AXIS2_PLACEMENT_3D('',#27302,#20094,#20095);
#18533=AXIS2_PLACEMENT_3D('',#27310,#20096,#20097);
#18534=AXIS2_PLACEMENT_3D('',#27316,#20098,#20099);
#18535=AXIS2_PLACEMENT_3D('',#27317,#20100,#20101);
#18536=AXIS2_PLACEMENT_3D('',#27417,#20102,#20103);
#18537=AXIS2_PLACEMENT_3D('',#27811,#20104,#20105);
#18538=AXIS2_PLACEMENT_3D('',#27819,#20106,#20107);
#18539=AXIS2_PLACEMENT_3D('',#27825,#20108,#20109);
#18540=AXIS2_PLACEMENT_3D('',#27826,#20110,#20111);
#18541=AXIS2_PLACEMENT_3D('',#27920,#20112,#20113);
#18542=AXIS2_PLACEMENT_3D('',#28247,#20114,#20115);
#18543=AXIS2_PLACEMENT_3D('',#28255,#20116,#20117);
#18544=AXIS2_PLACEMENT_3D('',#28261,#20118,#20119);
#18545=AXIS2_PLACEMENT_3D('',#28262,#20120,#20121);
#18546=AXIS2_PLACEMENT_3D('',#28362,#20122,#20123);
#18547=AXIS2_PLACEMENT_3D('',#28719,#20124,#20125);
#18548=AXIS2_PLACEMENT_3D('',#28727,#20126,#20127);
#18549=AXIS2_PLACEMENT_3D('',#28733,#20128,#20129);
#18550=AXIS2_PLACEMENT_3D('',#28734,#20130,#20131);
#18551=AXIS2_PLACEMENT_3D('',#28834,#20132,#20133);
#18552=AXIS2_PLACEMENT_3D('',#29181,#20134,#20135);
#18553=AXIS2_PLACEMENT_3D('',#29189,#20136,#20137);
#18554=AXIS2_PLACEMENT_3D('',#29195,#20138,#20139);
#18555=AXIS2_PLACEMENT_3D('',#29196,#20140,#20141);
#18556=AXIS2_PLACEMENT_3D('',#29290,#20142,#20143);
#18557=AXIS2_PLACEMENT_3D('',#29617,#20144,#20145);
#18558=AXIS2_PLACEMENT_3D('',#29625,#20146,#20147);
#18559=AXIS2_PLACEMENT_3D('',#29631,#20148,#20149);
#18560=AXIS2_PLACEMENT_3D('',#29632,#20150,#20151);
#18561=AXIS2_PLACEMENT_3D('',#29732,#20152,#20153);
#18562=AXIS2_PLACEMENT_3D('',#30089,#20154,#20155);
#18563=AXIS2_PLACEMENT_3D('',#30097,#20156,#20157);
#18564=AXIS2_PLACEMENT_3D('',#30103,#20158,#20159);
#18565=AXIS2_PLACEMENT_3D('',#30104,#20160,#20161);
#18566=AXIS2_PLACEMENT_3D('',#30204,#20162,#20163);
#18567=AXIS2_PLACEMENT_3D('',#30551,#20164,#20165);
#18568=AXIS2_PLACEMENT_3D('',#30559,#20166,#20167);
#18569=AXIS2_PLACEMENT_3D('',#30565,#20168,#20169);
#18570=AXIS2_PLACEMENT_3D('',#30566,#20170,#20171);
#18571=AXIS2_PLACEMENT_3D('',#30660,#20172,#20173);
#18572=AXIS2_PLACEMENT_3D('',#30987,#20174,#20175);
#18573=AXIS2_PLACEMENT_3D('',#30995,#20176,#20177);
#18574=AXIS2_PLACEMENT_3D('',#31001,#20178,#20179);
#18575=AXIS2_PLACEMENT_3D('',#31002,#20180,#20181);
#18576=AXIS2_PLACEMENT_3D('',#31102,#20182,#20183);
#18577=AXIS2_PLACEMENT_3D('',#31459,#20184,#20185);
#18578=AXIS2_PLACEMENT_3D('',#31467,#20186,#20187);
#18579=AXIS2_PLACEMENT_3D('',#31473,#20188,#20189);
#18580=AXIS2_PLACEMENT_3D('',#31474,#20190,#20191);
#18581=AXIS2_PLACEMENT_3D('',#31574,#20192,#20193);
#18582=AXIS2_PLACEMENT_3D('',#31921,#20194,#20195);
#18583=AXIS2_PLACEMENT_3D('',#31929,#20196,#20197);
#18584=AXIS2_PLACEMENT_3D('',#31935,#20198,#20199);
#18585=AXIS2_PLACEMENT_3D('',#31936,#20200,#20201);
#18586=AXIS2_PLACEMENT_3D('',#32030,#20202,#20203);
#18587=AXIS2_PLACEMENT_3D('',#32357,#20204,#20205);
#18588=AXIS2_PLACEMENT_3D('',#32365,#20206,#20207);
#18589=AXIS2_PLACEMENT_3D('',#32371,#20208,#20209);
#18590=AXIS2_PLACEMENT_3D('',#32372,#20210,#20211);
#18591=AXIS2_PLACEMENT_3D('',#32472,#20212,#20213);
#18592=AXIS2_PLACEMENT_3D('',#32829,#20214,#20215);
#18593=AXIS2_PLACEMENT_3D('',#32831,#20216,#20217);
#18594=AXIS2_PLACEMENT_3D('',#32834,#20219,#20220);
#18595=AXIS2_PLACEMENT_3D('',#32835,#20221,#20222);
#18596=AXIS2_PLACEMENT_3D('',#32837,#20223,#20224);
#18597=AXIS2_PLACEMENT_3D('',#32838,#20225,#20226);
#18598=AXIS2_PLACEMENT_3D('',#32840,#20227,#20228);
#18599=AXIS2_PLACEMENT_3D('',#32842,#20230,#20231);
#18600=AXIS2_PLACEMENT_3D('',#32844,#20232,#20233);
#18601=AXIS2_PLACEMENT_3D('',#32847,#20235,#20236);
#18602=AXIS2_PLACEMENT_3D('',#32848,#20237,#20238);
#18603=AXIS2_PLACEMENT_3D('',#32850,#20239,#20240);
#18604=AXIS2_PLACEMENT_3D('',#32851,#20241,#20242);
#18605=AXIS2_PLACEMENT_3D('',#32854,#20244,#20245);
#18606=AXIS2_PLACEMENT_3D('',#32855,#20246,#20247);
#18607=AXIS2_PLACEMENT_3D('',#32872,#20250,#20251);
#18608=AXIS2_PLACEMENT_3D('',#32879,#20252,#20253);
#18609=AXIS2_PLACEMENT_3D('',#32889,#20254,#20255);
#18610=AXIS2_PLACEMENT_3D('',#32890,#20256,#20257);
#18611=AXIS2_PLACEMENT_3D('',#32892,#20258,#20259);
#18612=AXIS2_PLACEMENT_3D('',#32902,#20260,#20261);
#18613=AXIS2_PLACEMENT_3D('',#32903,#20262,#20263);
#18614=AXIS2_PLACEMENT_3D('',#32904,#20264,#20265);
#18615=AXIS2_PLACEMENT_3D('',#32906,#20266,#20267);
#18616=AXIS2_PLACEMENT_3D('',#32913,#20268,#20269);
#18617=AXIS2_PLACEMENT_3D('',#32915,#20271,#20272);
#18618=AXIS2_PLACEMENT_3D('',#32925,#20274,#20275);
#18619=AXIS2_PLACEMENT_3D('',#32927,#20276,#20277);
#18620=AXIS2_PLACEMENT_3D('',#32937,#20278,#20279);
#18621=AXIS2_PLACEMENT_3D('',#32938,#20280,#20281);
#18622=AXIS2_PLACEMENT_3D('',#32950,#20284,#20285);
#18623=AXIS2_PLACEMENT_3D('',#32952,#20286,#20287);
#18624=AXIS2_PLACEMENT_3D('',#32962,#20288,#20289);
#18625=AXIS2_PLACEMENT_3D('',#32963,#20290,#20291);
#18626=AXIS2_PLACEMENT_3D('',#32964,#20292,#20293);
#18627=AXIS2_PLACEMENT_3D('',#32966,#20294,#20295);
#18628=AXIS2_PLACEMENT_3D('',#32973,#20296,#20297);
#18629=AXIS2_PLACEMENT_3D('',#32975,#20299,#20300);
#18630=AXIS2_PLACEMENT_3D('',#32985,#20302,#20303);
#18631=AXIS2_PLACEMENT_3D('',#32987,#20304,#20305);
#18632=AXIS2_PLACEMENT_3D('',#32997,#20306,#20307);
#18633=AXIS2_PLACEMENT_3D('',#32998,#20308,#20309);
#18634=AXIS2_PLACEMENT_3D('',#33010,#20312,#20313);
#18635=AXIS2_PLACEMENT_3D('',#33012,#20314,#20315);
#18636=AXIS2_PLACEMENT_3D('',#33022,#20316,#20317);
#18637=AXIS2_PLACEMENT_3D('',#33023,#20318,#20319);
#18638=AXIS2_PLACEMENT_3D('',#33024,#20320,#20321);
#18639=AXIS2_PLACEMENT_3D('',#33026,#20322,#20323);
#18640=AXIS2_PLACEMENT_3D('',#33033,#20324,#20325);
#18641=AXIS2_PLACEMENT_3D('',#33035,#20327,#20328);
#18642=AXIS2_PLACEMENT_3D('',#33045,#20330,#20331);
#18643=AXIS2_PLACEMENT_3D('',#33047,#20332,#20333);
#18644=AXIS2_PLACEMENT_3D('',#33057,#20334,#20335);
#18645=AXIS2_PLACEMENT_3D('',#33058,#20336,#20337);
#18646=AXIS2_PLACEMENT_3D('',#33070,#20340,#20341);
#18647=AXIS2_PLACEMENT_3D('',#33072,#20342,#20343);
#18648=AXIS2_PLACEMENT_3D('',#33082,#20344,#20345);
#18649=AXIS2_PLACEMENT_3D('',#33083,#20346,#20347);
#18650=AXIS2_PLACEMENT_3D('',#33084,#20348,#20349);
#18651=AXIS2_PLACEMENT_3D('',#33086,#20350,#20351);
#18652=AXIS2_PLACEMENT_3D('',#33093,#20352,#20353);
#18653=AXIS2_PLACEMENT_3D('',#33095,#20355,#20356);
#18654=AXIS2_PLACEMENT_3D('',#33105,#20358,#20359);
#18655=AXIS2_PLACEMENT_3D('',#33107,#20360,#20361);
#18656=AXIS2_PLACEMENT_3D('',#33117,#20362,#20363);
#18657=AXIS2_PLACEMENT_3D('',#33118,#20364,#20365);
#18658=AXIS2_PLACEMENT_3D('',#33130,#20368,#20369);
#18659=AXIS2_PLACEMENT_3D('',#33132,#20370,#20371);
#18660=AXIS2_PLACEMENT_3D('',#33142,#20372,#20373);
#18661=AXIS2_PLACEMENT_3D('',#33143,#20374,#20375);
#18662=AXIS2_PLACEMENT_3D('',#33144,#20376,#20377);
#18663=AXIS2_PLACEMENT_3D('',#33146,#20378,#20379);
#18664=AXIS2_PLACEMENT_3D('',#33153,#20380,#20381);
#18665=AXIS2_PLACEMENT_3D('',#33155,#20383,#20384);
#18666=AXIS2_PLACEMENT_3D('',#33165,#20386,#20387);
#18667=AXIS2_PLACEMENT_3D('',#33167,#20388,#20389);
#18668=AXIS2_PLACEMENT_3D('',#33177,#20390,#20391);
#18669=AXIS2_PLACEMENT_3D('',#33178,#20392,#20393);
#18670=AXIS2_PLACEMENT_3D('',#33180,#20394,#20395);
#18671=AXIS2_PLACEMENT_3D('',#33182,#20396,#20397);
#18672=AXIS2_PLACEMENT_3D('',#33184,#20398,#20399);
#18673=AXIS2_PLACEMENT_3D('',#33186,#20400,#20401);
#18674=AXIS2_PLACEMENT_3D('',#33188,#20402,#20403);
#18675=AXIS2_PLACEMENT_3D('',#33190,#20404,#20405);
#18676=AXIS2_PLACEMENT_3D('',#33192,#20406,#20407);
#18677=AXIS2_PLACEMENT_3D('',#33194,#20408,#20409);
#18678=AXIS2_PLACEMENT_3D('',#33196,#20410,#20411);
#18679=AXIS2_PLACEMENT_3D('',#33198,#20412,#20413);
#18680=AXIS2_PLACEMENT_3D('',#33200,#20414,#20415);
#18681=AXIS2_PLACEMENT_3D('',#33202,#20416,#20417);
#18682=AXIS2_PLACEMENT_3D('',#33203,#20418,#20419);
#18683=AXIS2_PLACEMENT_3D('',#33205,#20420,#20421);
#18684=AXIS2_PLACEMENT_3D('',#33206,#20422,#20423);
#18685=AXIS2_PLACEMENT_3D('',#33212,#20424,#20425);
#18686=AXIS2_PLACEMENT_3D('',#33221,#20426,#20427);
#18687=AXIS2_PLACEMENT_3D('',#33229,#20430,#20431);
#18688=AXIS2_PLACEMENT_3D('',#33236,#20432,#20433);
#18689=AXIS2_PLACEMENT_3D('',#33243,#20434,#20435);
#18690=AXIS2_PLACEMENT_3D('',#33252,#20437,#20438);
#18691=AXIS2_PLACEMENT_3D('',#33259,#20439,#20440);
#18692=AXIS2_PLACEMENT_3D('',#33269,#20442,#20443);
#18693=AXIS2_PLACEMENT_3D('',#33270,#20444,#20445);
#18694=AXIS2_PLACEMENT_3D('',#33272,#20446,#20447);
#18695=AXIS2_PLACEMENT_3D('',#33279,#20448,#20449);
#18696=AXIS2_PLACEMENT_3D('',#33281,#20451,#20452);
#18697=AXIS2_PLACEMENT_3D('',#33291,#20454,#20455);
#18698=AXIS2_PLACEMENT_3D('',#33293,#20456,#20457);
#18699=AXIS2_PLACEMENT_3D('',#33302,#20458,#20459);
#18700=AXIS2_PLACEMENT_3D('',#33308,#20460,#20461);
#18701=AXIS2_PLACEMENT_3D('',#33317,#20462,#20463);
#18702=AXIS2_PLACEMENT_3D('',#33325,#20466,#20467);
#18703=AXIS2_PLACEMENT_3D('',#33326,#20468,#20469);
#18704=AXIS2_PLACEMENT_3D('',#33328,#20470,#20471);
#18705=AXIS2_PLACEMENT_3D('',#33335,#20472,#20473);
#18706=AXIS2_PLACEMENT_3D('',#33337,#20475,#20476);
#18707=AXIS2_PLACEMENT_3D('',#33347,#20478,#20479);
#18708=AXIS2_PLACEMENT_3D('',#33349,#20480,#20481);
#18709=AXIS2_PLACEMENT_3D('',#33358,#20482,#20483);
#18710=AXIS2_PLACEMENT_3D('',#33364,#20484,#20485);
#18711=AXIS2_PLACEMENT_3D('',#33373,#20486,#20487);
#18712=AXIS2_PLACEMENT_3D('',#33381,#20490,#20491);
#18713=AXIS2_PLACEMENT_3D('',#33382,#20492,#20493);
#18714=AXIS2_PLACEMENT_3D('',#33384,#20494,#20495);
#18715=AXIS2_PLACEMENT_3D('',#33391,#20496,#20497);
#18716=AXIS2_PLACEMENT_3D('',#33393,#20499,#20500);
#18717=AXIS2_PLACEMENT_3D('',#33403,#20502,#20503);
#18718=AXIS2_PLACEMENT_3D('',#33405,#20504,#20505);
#18719=AXIS2_PLACEMENT_3D('',#33414,#20506,#20507);
#18720=AXIS2_PLACEMENT_3D('',#33420,#20508,#20509);
#18721=AXIS2_PLACEMENT_3D('',#33429,#20510,#20511);
#18722=AXIS2_PLACEMENT_3D('',#33437,#20514,#20515);
#18723=AXIS2_PLACEMENT_3D('',#33438,#20516,#20517);
#18724=AXIS2_PLACEMENT_3D('',#33440,#20518,#20519);
#18725=AXIS2_PLACEMENT_3D('',#33447,#20520,#20521);
#18726=AXIS2_PLACEMENT_3D('',#33449,#20523,#20524);
#18727=AXIS2_PLACEMENT_3D('',#33459,#20526,#20527);
#18728=AXIS2_PLACEMENT_3D('',#33461,#20528,#20529);
#18729=AXIS2_PLACEMENT_3D('',#33470,#20530,#20531);
#18730=AXIS2_PLACEMENT_3D('',#33476,#20532,#20533);
#18731=AXIS2_PLACEMENT_3D('',#33485,#20534,#20535);
#18732=AXIS2_PLACEMENT_3D('',#33493,#20538,#20539);
#18733=AXIS2_PLACEMENT_3D('',#33494,#20540,#20541);
#18734=AXIS2_PLACEMENT_3D('',#33496,#20542,#20543);
#18735=AXIS2_PLACEMENT_3D('',#33503,#20544,#20545);
#18736=AXIS2_PLACEMENT_3D('',#33505,#20547,#20548);
#18737=AXIS2_PLACEMENT_3D('',#33515,#20550,#20551);
#18738=AXIS2_PLACEMENT_3D('',#33517,#20552,#20553);
#18739=AXIS2_PLACEMENT_3D('',#33526,#20554,#20555);
#18740=AXIS2_PLACEMENT_3D('',#33532,#20556,#20557);
#18741=AXIS2_PLACEMENT_3D('',#33541,#20558,#20559);
#18742=AXIS2_PLACEMENT_3D('',#33549,#20562,#20563);
#18743=AXIS2_PLACEMENT_3D('',#33551,#20564,#20565);
#18744=AXIS2_PLACEMENT_3D('',#33554,#20567,#20568);
#18745=AXIS2_PLACEMENT_3D('',#33556,#20569,#20570);
#18746=AXIS2_PLACEMENT_3D('',#33562,#20571,#20572);
#18747=AXIS2_PLACEMENT_3D('',#33563,#20573,#20574);
#18748=AXIS2_PLACEMENT_3D('',#33572,#20575,#20576);
#18749=AXIS2_PLACEMENT_3D('',#33573,#20577,#20578);
#18750=AXIS2_PLACEMENT_3D('',#33575,#20579,#20580);
#18751=AXIS2_PLACEMENT_3D('',#33582,#20581,#20582);
#18752=AXIS2_PLACEMENT_3D('',#33584,#20584,#20585);
#18753=AXIS2_PLACEMENT_3D('',#33594,#20587,#20588);
#18754=AXIS2_PLACEMENT_3D('',#33596,#20589,#20590);
#18755=AXIS2_PLACEMENT_3D('',#33600,#20591,#20592);
#18756=AXIS2_PLACEMENT_3D('',#33606,#20594,#20595);
#18757=AXIS2_PLACEMENT_3D('',#33614,#20596,#20597);
#18758=AXIS2_PLACEMENT_3D('',#33615,#20598,#20599);
#18759=AXIS2_PLACEMENT_3D('',#33629,#20600,#20601);
#18760=AXIS2_PLACEMENT_3D('',#33634,#20602,#20603);
#18761=AXIS2_PLACEMENT_3D('',#33731,#20604,#20605);
#18762=AXIS2_PLACEMENT_3D('',#33733,#20606,#20607);
#18763=AXIS2_PLACEMENT_3D('',#34382,#20608,#20609);
#18764=AXIS2_PLACEMENT_3D('',#34384,#20610,#20611);
#18765=AXIS2_PLACEMENT_3D('',#34385,#20612,#20613);
#18766=AXIS2_PLACEMENT_3D('',#34484,#20614,#20615);
#18767=AXIS2_PLACEMENT_3D('',#34485,#20616,#20617);
#18768=AXIS2_PLACEMENT_3D('',#34938,#20618,#20619);
#18769=AXIS2_PLACEMENT_3D('',#35216,#20620,#20621);
#18770=AXIS2_PLACEMENT_3D('',#35281,#20622,#20623);
#18771=AXIS2_PLACEMENT_3D('',#35286,#20624,#20625);
#18772=AXIS2_PLACEMENT_3D('',#35287,#20626,#20627);
#18773=AXIS2_PLACEMENT_3D('',#35288,#20628,#20629);
#18774=AXIS2_PLACEMENT_3D('',#35301,#20630,#20631);
#18775=AXIS2_PLACEMENT_3D('',#35306,#20632,#20633);
#18776=AXIS2_PLACEMENT_3D('',#35307,#20634,#20635);
#18777=AXIS2_PLACEMENT_3D('',#35308,#20636,#20637);
#18778=AXIS2_PLACEMENT_3D('',#35309,#20638,#20639);
#18779=AXIS2_PLACEMENT_3D('',#35322,#20640,#20641);
#18780=AXIS2_PLACEMENT_3D('',#35327,#20642,#20643);
#18781=AXIS2_PLACEMENT_3D('',#35328,#20644,#20645);
#18782=AXIS2_PLACEMENT_3D('',#35329,#20646,#20647);
#18783=AXIS2_PLACEMENT_3D('',#35330,#20648,#20649);
#18784=AXIS2_PLACEMENT_3D('',#35343,#20650,#20651);
#18785=AXIS2_PLACEMENT_3D('',#35348,#20652,#20653);
#18786=AXIS2_PLACEMENT_3D('',#35349,#20654,#20655);
#18787=AXIS2_PLACEMENT_3D('',#35350,#20656,#20657);
#18788=AXIS2_PLACEMENT_3D('',#35351,#20658,#20659);
#18789=AXIS2_PLACEMENT_3D('',#35364,#20660,#20661);
#18790=AXIS2_PLACEMENT_3D('',#35369,#20662,#20663);
#18791=AXIS2_PLACEMENT_3D('',#35370,#20664,#20665);
#18792=AXIS2_PLACEMENT_3D('',#35371,#20666,#20667);
#18793=AXIS2_PLACEMENT_3D('',#35372,#20668,#20669);
#18794=AXIS2_PLACEMENT_3D('',#35385,#20670,#20671);
#18795=AXIS2_PLACEMENT_3D('',#35390,#20672,#20673);
#18796=AXIS2_PLACEMENT_3D('',#35391,#20674,#20675);
#18797=AXIS2_PLACEMENT_3D('',#35392,#20676,#20677);
#18798=AXIS2_PLACEMENT_3D('',#35393,#20678,#20679);
#18799=AXIS2_PLACEMENT_3D('',#35406,#20680,#20681);
#18800=AXIS2_PLACEMENT_3D('',#35411,#20682,#20683);
#18801=AXIS2_PLACEMENT_3D('',#35412,#20684,#20685);
#18802=AXIS2_PLACEMENT_3D('',#35413,#20686,#20687);
#18803=AXIS2_PLACEMENT_3D('',#35414,#20688,#20689);
#18804=AXIS2_PLACEMENT_3D('',#35427,#20690,#20691);
#18805=AXIS2_PLACEMENT_3D('',#35432,#20692,#20693);
#18806=AXIS2_PLACEMENT_3D('',#35433,#20694,#20695);
#18807=AXIS2_PLACEMENT_3D('',#35434,#20696,#20697);
#18808=AXIS2_PLACEMENT_3D('',#35435,#20698,#20699);
#18809=AXIS2_PLACEMENT_3D('',#35448,#20700,#20701);
#18810=AXIS2_PLACEMENT_3D('',#35453,#20702,#20703);
#18811=AXIS2_PLACEMENT_3D('',#35454,#20704,#20705);
#18812=AXIS2_PLACEMENT_3D('',#35455,#20706,#20707);
#18813=AXIS2_PLACEMENT_3D('',#35456,#20708,#20709);
#18814=AXIS2_PLACEMENT_3D('',#35469,#20710,#20711);
#18815=AXIS2_PLACEMENT_3D('',#35474,#20712,#20713);
#18816=AXIS2_PLACEMENT_3D('',#35475,#20714,#20715);
#18817=AXIS2_PLACEMENT_3D('',#35476,#20716,#20717);
#18818=AXIS2_PLACEMENT_3D('',#35481,#20718,#20719);
#18819=AXIS2_PLACEMENT_3D('',#35482,#20720,#20721);
#18820=AXIS2_PLACEMENT_3D('',#35483,#20722,#20723);
#18821=AXIS2_PLACEMENT_3D('',#35488,#20724,#20725);
#18822=AXIS2_PLACEMENT_3D('',#35489,#20726,#20727);
#18823=AXIS2_PLACEMENT_3D('',#35491,#20728,#20729);
#18824=AXIS2_PLACEMENT_3D('',#35494,#20731,#20732);
#18825=AXIS2_PLACEMENT_3D('',#35495,#20733,#20734);
#18826=AXIS2_PLACEMENT_3D('',#35496,#20735,#20736);
#18827=AXIS2_PLACEMENT_3D('',#35498,#20737,#20738);
#18828=AXIS2_PLACEMENT_3D('',#35499,#20739,#20740);
#18829=AXIS2_PLACEMENT_3D('',#35501,#20741,#20742);
#18830=AXIS2_PLACEMENT_3D('',#35503,#20744,#20745);
#18831=AXIS2_PLACEMENT_3D('',#35505,#20747,#20748);
#18832=AXIS2_PLACEMENT_3D('',#35513,#20749,#20750);
#18833=AXIS2_PLACEMENT_3D('',#35514,#20751,#20752);
#18834=AXIS2_PLACEMENT_3D('',#36014,#20753,#20754);
#18835=AXIS2_PLACEMENT_3D('',#36022,#20755,#20756);
#18836=AXIS2_PLACEMENT_3D('',#36023,#20757,#20758);
#18837=AXIS2_PLACEMENT_3D('',#36533,#20759,#20760);
#18838=AXIS2_PLACEMENT_3D('',#36541,#20761,#20762);
#18839=AXIS2_PLACEMENT_3D('',#36542,#20763,#20764);
#18840=AXIS2_PLACEMENT_3D('',#37032,#20765,#20766);
#18841=AXIS2_PLACEMENT_3D('',#37040,#20767,#20768);
#18842=AXIS2_PLACEMENT_3D('',#37041,#20769,#20770);
#18843=AXIS2_PLACEMENT_3D('',#37541,#20771,#20772);
#18844=AXIS2_PLACEMENT_3D('',#37549,#20773,#20774);
#18845=AXIS2_PLACEMENT_3D('',#37550,#20775,#20776);
#18846=AXIS2_PLACEMENT_3D('',#38060,#20777,#20778);
#18847=AXIS2_PLACEMENT_3D('',#38068,#20779,#20780);
#18848=AXIS2_PLACEMENT_3D('',#38069,#20781,#20782);
#18849=AXIS2_PLACEMENT_3D('',#38559,#20783,#20784);
#18850=AXIS2_PLACEMENT_3D('',#38567,#20785,#20786);
#18851=AXIS2_PLACEMENT_3D('',#38568,#20787,#20788);
#18852=AXIS2_PLACEMENT_3D('',#39068,#20789,#20790);
#18853=AXIS2_PLACEMENT_3D('',#39076,#20791,#20792);
#18854=AXIS2_PLACEMENT_3D('',#39077,#20793,#20794);
#18855=AXIS2_PLACEMENT_3D('',#39587,#20795,#20796);
#18856=AXIS2_PLACEMENT_3D('',#39595,#20797,#20798);
#18857=AXIS2_PLACEMENT_3D('',#39596,#20799,#20800);
#18858=AXIS2_PLACEMENT_3D('',#40096,#20801,#20802);
#18859=AXIS2_PLACEMENT_3D('',#40104,#20803,#20804);
#18860=AXIS2_PLACEMENT_3D('',#40105,#20805,#20806);
#18861=AXIS2_PLACEMENT_3D('',#40605,#20807,#20808);
#18862=AXIS2_PLACEMENT_3D('',#40613,#20809,#20810);
#18863=AXIS2_PLACEMENT_3D('',#40614,#20811,#20812);
#18864=AXIS2_PLACEMENT_3D('',#41124,#20813,#20814);
#18865=AXIS2_PLACEMENT_3D('',#41132,#20815,#20816);
#18866=AXIS2_PLACEMENT_3D('',#41133,#20817,#20818);
#18867=AXIS2_PLACEMENT_3D('',#41623,#20819,#20820);
#18868=AXIS2_PLACEMENT_3D('',#41626,#20823,#20824);
#18869=AXIS2_PLACEMENT_3D('',#41628,#20826,#20827);
#18870=AXIS2_PLACEMENT_3D('',#41630,#20829,#20830);
#18871=AXIS2_PLACEMENT_3D('',#41632,#20832,#20833);
#18872=AXIS2_PLACEMENT_3D('',#41634,#20835,#20836);
#18873=AXIS2_PLACEMENT_3D('',#41636,#20838,#20839);
#18874=AXIS2_PLACEMENT_3D('',#41638,#20841,#20842);
#18875=AXIS2_PLACEMENT_3D('',#41639,#20843,#20844);
#18876=AXIS2_PLACEMENT_3D('',#41641,#20846,#20847);
#18877=AXIS2_PLACEMENT_3D('',#41643,#20849,#20850);
#18878=AXIS2_PLACEMENT_3D('',#41645,#20852,#20853);
#18879=AXIS2_PLACEMENT_3D('',#41647,#20855,#20856);
#18880=AXIS2_PLACEMENT_3D('',#41649,#20858,#20859);
#18881=AXIS2_PLACEMENT_3D('',#41651,#20861,#20862);
#18882=AXIS2_PLACEMENT_3D('',#41652,#20863,#20864);
#18883=AXIS2_PLACEMENT_3D('',#41654,#20865,#20866);
#18884=AXIS2_PLACEMENT_3D('',#41656,#20868,#20869);
#18885=AXIS2_PLACEMENT_3D('',#41658,#20871,#20872);
#18886=AXIS2_PLACEMENT_3D('',#41660,#20874,#20875);
#18887=AXIS2_PLACEMENT_3D('',#41662,#20876,#20877);
#18888=AXIS2_PLACEMENT_3D('',#41664,#20879,#20880);
#18889=AXIS2_PLACEMENT_3D('',#41666,#20881,#20882);
#18890=AXIS2_PLACEMENT_3D('',#41667,#20883,#20884);
#18891=AXIS2_PLACEMENT_3D('',#41669,#20885,#20886);
#18892=AXIS2_PLACEMENT_3D('',#41671,#20888,#20889);
#18893=AXIS2_PLACEMENT_3D('',#41673,#20890,#20891);
#18894=AXIS2_PLACEMENT_3D('',#41675,#20893,#20894);
#18895=AXIS2_PLACEMENT_3D('',#41677,#20895,#20896);
#18896=AXIS2_PLACEMENT_3D('',#41679,#20898,#20899);
#18897=AXIS2_PLACEMENT_3D('',#41681,#20900,#20901);
#18898=AXIS2_PLACEMENT_3D('',#41683,#20903,#20904);
#18899=AXIS2_PLACEMENT_3D('',#41685,#20905,#20906);
#18900=AXIS2_PLACEMENT_3D('',#41686,#20907,#20908);
#18901=AXIS2_PLACEMENT_3D('',#41688,#20909,#20910);
#18902=AXIS2_PLACEMENT_3D('',#41690,#20912,#20913);
#18903=AXIS2_PLACEMENT_3D('',#41692,#20914,#20915);
#18904=AXIS2_PLACEMENT_3D('',#41694,#20917,#20918);
#18905=AXIS2_PLACEMENT_3D('',#41696,#20919,#20920);
#18906=AXIS2_PLACEMENT_3D('',#41698,#20922,#20923);
#18907=AXIS2_PLACEMENT_3D('',#41700,#20924,#20925);
#18908=AXIS2_PLACEMENT_3D('',#41702,#20927,#20928);
#18909=AXIS2_PLACEMENT_3D('',#41704,#20929,#20930);
#18910=AXIS2_PLACEMENT_3D('',#41706,#20932,#20933);
#18911=AXIS2_PLACEMENT_3D('',#41708,#20935,#20936);
#18912=AXIS2_PLACEMENT_3D('',#41709,#20937,#20938);
#18913=AXIS2_PLACEMENT_3D('',#41710,#20939,#20940);
#18914=AXIS2_PLACEMENT_3D('',#41712,#20941,#20942);
#18915=AXIS2_PLACEMENT_3D('',#41714,#20944,#20945);
#19680=DIRECTION('axis',(0.,0.,1.));
#19681=DIRECTION('refdir',(1.,0.,0.));
#19682=DIRECTION('center_axis',(1.,0.,0.));
#19683=DIRECTION('ref_axis',(0.,1.,0.));
#19684=DIRECTION('',(-1.,0.,0.));
#19685=DIRECTION('center_axis',(1.,0.,0.));
#19686=DIRECTION('ref_axis',(0.,1.,0.));
#19687=DIRECTION('center_axis',(1.,0.,0.));
#19688=DIRECTION('ref_axis',(0.,1.,0.));
#19689=DIRECTION('',(-1.,0.,0.));
#19690=DIRECTION('center_axis',(1.,0.,0.));
#19691=DIRECTION('ref_axis',(0.,1.,0.));
#19692=DIRECTION('',(-1.,0.,0.));
#19693=DIRECTION('center_axis',(1.,0.,0.));
#19694=DIRECTION('ref_axis',(0.,1.,0.));
#19695=DIRECTION('',(-1.,0.,0.));
#19696=DIRECTION('center_axis',(1.,0.,0.));
#19697=DIRECTION('ref_axis',(0.,1.,0.));
#19698=DIRECTION('',(-1.,0.,0.));
#19699=DIRECTION('center_axis',(1.,0.,0.));
#19700=DIRECTION('ref_axis',(0.,1.,0.));
#19701=DIRECTION('',(-1.,0.,0.));
#19702=DIRECTION('center_axis',(1.,0.,0.));
#19703=DIRECTION('ref_axis',(0.,1.,0.));
#19704=DIRECTION('',(-1.,0.,0.));
#19705=DIRECTION('center_axis',(1.,0.,0.));
#19706=DIRECTION('ref_axis',(0.,1.,0.));
#19707=DIRECTION('',(-1.,0.,0.));
#19708=DIRECTION('center_axis',(1.,0.,0.));
#19709=DIRECTION('ref_axis',(0.,1.,0.));
#19710=DIRECTION('',(-1.,0.,0.));
#19711=DIRECTION('center_axis',(1.,0.,0.));
#19712=DIRECTION('ref_axis',(0.,1.,0.));
#19713=DIRECTION('',(-1.,0.,0.));
#19714=DIRECTION('center_axis',(1.,0.,0.));
#19715=DIRECTION('ref_axis',(0.,1.,0.));
#19716=DIRECTION('',(-1.,0.,0.));
#19717=DIRECTION('center_axis',(1.,0.,0.));
#19718=DIRECTION('ref_axis',(0.,1.,0.));
#19719=DIRECTION('',(-1.,0.,0.));
#19720=DIRECTION('center_axis',(1.,0.,0.));
#19721=DIRECTION('ref_axis',(0.,1.,0.));
#19722=DIRECTION('',(-1.,0.,0.));
#19723=DIRECTION('center_axis',(1.,0.,0.));
#19724=DIRECTION('ref_axis',(0.,1.,0.));
#19725=DIRECTION('',(-1.,0.,0.));
#19726=DIRECTION('center_axis',(1.,0.,0.));
#19727=DIRECTION('ref_axis',(0.,1.,0.));
#19728=DIRECTION('',(-1.,0.,0.));
#19729=DIRECTION('center_axis',(1.,0.,0.));
#19730=DIRECTION('ref_axis',(0.,1.,0.));
#19731=DIRECTION('',(-1.,0.,0.));
#19732=DIRECTION('center_axis',(1.,0.,0.));
#19733=DIRECTION('ref_axis',(0.,0.,-1.));
#19734=DIRECTION('center_axis',(1.,0.,0.));
#19735=DIRECTION('ref_axis',(0.,0.,-1.));
#19736=DIRECTION('center_axis',(1.,0.,0.));
#19737=DIRECTION('ref_axis',(0.,0.,-1.));
#19738=DIRECTION('center_axis',(1.,0.,0.));
#19739=DIRECTION('ref_axis',(0.,0.,-1.));
#19740=DIRECTION('center_axis',(1.,0.,0.));
#19741=DIRECTION('ref_axis',(0.,0.,-1.));
#19742=DIRECTION('center_axis',(1.,0.,0.));
#19743=DIRECTION('ref_axis',(0.,0.,-1.));
#19744=DIRECTION('center_axis',(1.,0.,0.));
#19745=DIRECTION('ref_axis',(0.,0.,-1.));
#19746=DIRECTION('center_axis',(1.,0.,0.));
#19747=DIRECTION('ref_axis',(0.,0.,-1.));
#19748=DIRECTION('center_axis',(1.,0.,0.));
#19749=DIRECTION('ref_axis',(0.,0.,-1.));
#19750=DIRECTION('center_axis',(1.,0.,0.));
#19751=DIRECTION('ref_axis',(0.,0.,-1.));
#19752=DIRECTION('center_axis',(1.,0.,0.));
#19753=DIRECTION('ref_axis',(0.,0.,-1.));
#19754=DIRECTION('center_axis',(1.,0.,0.));
#19755=DIRECTION('ref_axis',(0.,0.,-1.));
#19756=DIRECTION('center_axis',(1.,0.,0.));
#19757=DIRECTION('ref_axis',(0.,0.,-1.));
#19758=DIRECTION('center_axis',(1.,0.,0.));
#19759=DIRECTION('ref_axis',(0.,0.,-1.));
#19760=DIRECTION('center_axis',(1.,0.,0.));
#19761=DIRECTION('ref_axis',(0.,0.,-1.));
#19762=DIRECTION('center_axis',(1.,0.,0.));
#19763=DIRECTION('ref_axis',(0.,0.,-1.));
#19764=DIRECTION('center_axis',(1.,0.,0.));
#19765=DIRECTION('ref_axis',(0.,0.,-1.));
#19766=DIRECTION('center_axis',(1.,0.,0.));
#19767=DIRECTION('ref_axis',(0.,0.,-1.));
#19768=DIRECTION('center_axis',(1.,0.,0.));
#19769=DIRECTION('ref_axis',(0.,0.,-1.));
#19770=DIRECTION('center_axis',(1.,0.,0.));
#19771=DIRECTION('ref_axis',(0.,0.,-1.));
#19772=DIRECTION('center_axis',(1.,0.,0.));
#19773=DIRECTION('ref_axis',(0.,0.,-1.));
#19774=DIRECTION('center_axis',(1.,0.,0.));
#19775=DIRECTION('ref_axis',(0.,0.,-1.));
#19776=DIRECTION('center_axis',(1.,0.,0.));
#19777=DIRECTION('ref_axis',(0.,0.,-1.));
#19778=DIRECTION('center_axis',(1.,0.,0.));
#19779=DIRECTION('ref_axis',(0.,-0.201120720209613,-0.9795664632389));
#19780=DIRECTION('',(1.,0.,0.));
#19781=DIRECTION('center_axis',(1.,0.,0.));
#19782=DIRECTION('ref_axis',(0.,1.,1.0886778522233E-13));
#19783=DIRECTION('center_axis',(1.,0.,0.));
#19784=DIRECTION('ref_axis',(0.,1.,1.0886778522233E-13));
#19785=DIRECTION('',(1.,0.,0.));
#19786=DIRECTION('center_axis',(1.,0.,0.));
#19787=DIRECTION('ref_axis',(0.,1.,1.0886778522233E-13));
#19788=DIRECTION('',(1.,0.,0.));
#19789=DIRECTION('center_axis',(1.,0.,0.));
#19790=DIRECTION('ref_axis',(0.,1.,1.0886778522233E-13));
#19791=DIRECTION('',(1.,0.,0.));
#19792=DIRECTION('center_axis',(1.,0.,0.));
#19793=DIRECTION('ref_axis',(0.,1.,1.0886778522233E-13));
#19794=DIRECTION('',(1.,0.,0.));
#19795=DIRECTION('center_axis',(1.,0.,0.));
#19796=DIRECTION('ref_axis',(0.,1.,1.0886778522233E-13));
#19797=DIRECTION('',(1.,0.,0.));
#19798=DIRECTION('center_axis',(1.,0.,0.));
#19799=DIRECTION('ref_axis',(0.,1.,1.0886778522233E-13));
#19800=DIRECTION('',(1.,0.,0.));
#19801=DIRECTION('center_axis',(1.,0.,0.));
#19802=DIRECTION('ref_axis',(0.,1.,1.0886778522233E-13));
#19803=DIRECTION('',(1.,0.,0.));
#19804=DIRECTION('center_axis',(1.,0.,0.));
#19805=DIRECTION('ref_axis',(0.,1.,1.0886778522233E-13));
#19806=DIRECTION('',(1.,0.,0.));
#19807=DIRECTION('center_axis',(1.,0.,0.));
#19808=DIRECTION('ref_axis',(0.,1.,1.0886778522233E-13));
#19809=DIRECTION('',(1.,0.,0.));
#19810=DIRECTION('center_axis',(1.,0.,0.));
#19811=DIRECTION('ref_axis',(0.,1.,1.0886778522233E-13));
#19812=DIRECTION('',(1.,0.,0.));
#19813=DIRECTION('center_axis',(1.,0.,0.));
#19814=DIRECTION('ref_axis',(0.,1.,1.0886778522233E-13));
#19815=DIRECTION('',(1.,0.,0.));
#19816=DIRECTION('center_axis',(1.,0.,0.));
#19817=DIRECTION('ref_axis',(0.,1.,1.0886778522233E-13));
#19818=DIRECTION('',(1.,0.,0.));
#19819=DIRECTION('center_axis',(1.,0.,0.));
#19820=DIRECTION('ref_axis',(0.,1.,1.0886778522233E-13));
#19821=DIRECTION('',(1.,0.,0.));
#19822=DIRECTION('center_axis',(1.,0.,0.));
#19823=DIRECTION('ref_axis',(0.,1.,1.0886778522233E-13));
#19824=DIRECTION('',(1.,0.,0.));
#19825=DIRECTION('center_axis',(1.,0.,0.));
#19826=DIRECTION('ref_axis',(0.,1.,1.0886778522233E-13));
#19827=DIRECTION('',(1.,0.,0.));
#19828=DIRECTION('center_axis',(-1.,0.,-1.46491071877532E-15));
#19829=DIRECTION('ref_axis',(0.,-1.,-3.17896142702966E-17));
#19830=DIRECTION('center_axis',(-1.,0.,0.));
#19831=DIRECTION('ref_axis',(0.,-1.,0.));
#19832=DIRECTION('',(-0.492698814983593,0.870199906753479,-5.87527702781227E-16));
#19833=DIRECTION('center_axis',(1.,0.,0.));
#19834=DIRECTION('ref_axis',(0.,-1.,-6.12323399573676E-17));
#19835=DIRECTION('center_axis',(1.,0.,0.));
#19836=DIRECTION('ref_axis',(0.,-1.,-6.12323399573676E-17));
#19837=DIRECTION('center_axis',(-1.,0.,0.));
#19838=DIRECTION('ref_axis',(0.,1.,0.));
#19839=DIRECTION('',(-0.857492925712545,-0.514495755427525,-6.30075580059218E-17));
#19840=DIRECTION('center_axis',(1.,0.,0.));
#19841=DIRECTION('ref_axis',(0.,0.,-1.));
#19842=DIRECTION('center_axis',(1.,0.,0.));
#19843=DIRECTION('ref_axis',(0.,0.,-1.));
#19844=DIRECTION('center_axis',(1.,0.,0.));
#19845=DIRECTION('ref_axis',(0.,0.,-1.));
#19846=DIRECTION('center_axis',(0.,0.866025403784439,0.499999999999999));
#19847=DIRECTION('ref_axis',(0.,-0.499999999999999,0.866025403784439));
#19848=DIRECTION('',(0.463876645871912,-0.442949900500785,0.767211732874941));
#19849=DIRECTION('',(1.,0.,0.));
#19850=DIRECTION('',(0.,-0.499999999999999,0.866025403784439));
#19851=DIRECTION('',(-1.,0.,0.));
#19852=DIRECTION('',(-0.463876645871911,-0.442949900500785,0.767211732874941));
#19853=DIRECTION('center_axis',(0.,0.475999928342023,0.879445318492508));
#19854=DIRECTION('ref_axis',(0.,-0.879445318492508,0.475999928342023));
#19855=DIRECTION('',(0.,0.879445318492508,-0.475999928342023));
#19856=DIRECTION('',(1.,0.,0.));
#19857=DIRECTION('',(0.,-0.879445318492508,0.475999928342023));
#19858=DIRECTION('center_axis',(-0.707106781186547,0.336582777174955,0.621861748388816));
#19859=DIRECTION('ref_axis',(0.660393123266679,0.,0.750920050832364));
#19860=DIRECTION('',(0.648510052987376,0.659223811296842,0.380603044908442));
#19861=DIRECTION('',(0.,-0.879445318492508,0.475999928342023));
#19862=DIRECTION('',(0.691947206789735,0.510494399095566,0.510494399095564));
#19863=DIRECTION('center_axis',(-0.707106781186547,0.706839460333999,-0.01944163868458));
#19864=DIRECTION('ref_axis',(-0.0274842426448097,0.,0.999622236850622));
#19865=DIRECTION('',(0.,-0.0274946291024904,-0.99962195122482));
#19866=DIRECTION('',(0.691947206789734,0.697348317654214,0.18685391855865));
#19867=DIRECTION('',(0.,0.0274946291024904,0.99962195122482));
#19868=DIRECTION('center_axis',(0.,0.500000000000001,0.866025403784438));
#19869=DIRECTION('ref_axis',(1.,0.,0.));
#19870=DIRECTION('',(0.463876645871911,-0.76721173287494,0.442949900500787));
#19871=DIRECTION('',(1.,0.,0.));
#19872=DIRECTION('',(0.,-0.866025403784438,0.500000000000001));
#19873=DIRECTION('',(-1.,0.,0.));
#19874=DIRECTION('',(-0.463876645871911,-0.76721173287494,0.442949900500787));
#19875=DIRECTION('center_axis',(0.,-0.0274946291024896,0.99962195122482));
#19876=DIRECTION('ref_axis',(0.,-0.99962195122482,-0.0274946291024896));
#19877=DIRECTION('',(0.,0.99962195122482,0.0274946291024896));
#19878=DIRECTION('',(1.,0.,0.));
#19879=DIRECTION('',(0.,-0.99962195122482,-0.0274946291024896));
#19880=DIRECTION('center_axis',(-0.707106781186548,-0.0194416386845794,
0.706839460333999));
#19881=DIRECTION('ref_axis',(0.706973082855489,0.,0.707240454242973));
#19882=DIRECTION('',(0.648510052987376,0.380603044908442,0.659223811296841));
#19883=DIRECTION('',(0.,-0.99962195122482,-0.0274946291024896));
#19884=DIRECTION('',(0.691947206789734,0.186853918558649,0.697348317654214));
#19885=DIRECTION('center_axis',(-0.707106781186547,0.621861748388816,0.336582777174955));
#19886=DIRECTION('ref_axis',(0.429793326728032,0.,0.902927292920117));
#19887=DIRECTION('',(0.,0.475999928342023,-0.879445318492508));
#19888=DIRECTION('',(0.,-0.475999928342023,0.879445318492508));
#19889=DIRECTION('center_axis',(0.,2.60630817828214E-15,1.));
#19890=DIRECTION('ref_axis',(1.,0.,0.));
#19891=DIRECTION('',(0.463876645871913,-0.885899801001572,2.30892789648892E-15));
#19892=DIRECTION('',(1.,0.,0.));
#19893=DIRECTION('',(0.,-1.,2.60630817828214E-15));
#19894=DIRECTION('',(-1.,0.,0.));
#19895=DIRECTION('',(-0.463876645871909,-0.885899801001573,2.30892789648892E-15));
#19896=DIRECTION('center_axis',(0.,-0.523622022882797,0.851950689390019));
#19897=DIRECTION('ref_axis',(0.,-0.851950689390018,-0.523622022882797));
#19898=DIRECTION('',(0.,0.851950689390018,0.523622022882797));
#19899=DIRECTION('',(1.,0.,0.));
#19900=DIRECTION('',(0.,-0.851950689390018,-0.523622022882797));
#19901=DIRECTION('center_axis',(-0.707106781186547,-0.370256683159044,0.602420109704237));
#19902=DIRECTION('ref_axis',(0.648510052987376,0.,0.761206089816884));
#19903=DIRECTION('',(0.648510052987376,3.84997679969453E-16,0.761206089816884));
#19904=DIRECTION('',(0.,-0.851950689390018,-0.523622022882797));
#19905=DIRECTION('',(0.691947206789735,-0.186853918558647,0.697348317654214));
#19906=DIRECTION('center_axis',(-0.707106781186548,0.370256683159043,0.602420109704236));
#19907=DIRECTION('ref_axis',(0.648510052987375,0.,0.761206089816885));
#19908=DIRECTION('',(0.,0.851950689390018,-0.523622022882797));
#19909=DIRECTION('',(0.,-0.851950689390018,0.523622022882797));
#19910=DIRECTION('center_axis',(0.,-0.5,0.866025403784439));
#19911=DIRECTION('ref_axis',(1.,0.,0.));
#19912=DIRECTION('',(0.463876645871911,-0.767211732874941,-0.442949900500786));
#19913=DIRECTION('',(1.,0.,0.));
#19914=DIRECTION('',(0.,-0.866025403784439,-0.5));
#19915=DIRECTION('',(-1.,0.,0.));
#19916=DIRECTION('',(-0.463876645871911,-0.767211732874941,-0.442949900500786));
#19917=DIRECTION('center_axis',(0.,-0.879445318492508,0.475999928342023));
#19918=DIRECTION('ref_axis',(0.,-0.475999928342023,-0.879445318492508));
#19919=DIRECTION('',(0.,0.475999928342023,0.879445318492508));
#19920=DIRECTION('',(1.,0.,0.));
#19921=DIRECTION('',(0.,-0.475999928342023,-0.879445318492508));
#19922=DIRECTION('center_axis',(-0.707106781186547,-0.621861748388816,0.336582777174955));
#19923=DIRECTION('ref_axis',(0.429793326728033,0.,0.902927292920117));
#19924=DIRECTION('',(0.648510052987375,-0.380603044908443,0.659223811296841));
#19925=DIRECTION('',(0.,-0.475999928342023,-0.879445318492508));
#19926=DIRECTION('',(0.691947206789734,-0.510494399095567,0.510494399095564));
#19927=DIRECTION('center_axis',(-0.707106781186547,0.01944163868458,0.706839460333999));
#19928=DIRECTION('ref_axis',(0.706973082855489,0.,0.707240454242973));
#19929=DIRECTION('',(0.,0.99962195122482,-0.0274946291024905));
#19930=DIRECTION('',(0.,-0.99962195122482,0.0274946291024905));
#19931=DIRECTION('center_axis',(0.,-0.866025403784438,0.500000000000001));
#19932=DIRECTION('ref_axis',(1.,0.,0.));
#19933=DIRECTION('',(0.463876645871912,-0.442949900500786,-0.76721173287494));
#19934=DIRECTION('',(1.,0.,0.));
#19935=DIRECTION('',(0.,-0.500000000000001,-0.866025403784438));
#19936=DIRECTION('',(-1.,0.,0.));
#19937=DIRECTION('',(-0.463876645871911,-0.442949900500787,-0.76721173287494));
#19938=DIRECTION('center_axis',(0.,-0.99962195122482,-0.0274946291024905));
#19939=DIRECTION('ref_axis',(0.,0.0274946291024905,-0.99962195122482));
#19940=DIRECTION('',(0.,-0.0274946291024905,0.99962195122482));
#19941=DIRECTION('',(1.,0.,0.));
#19942=DIRECTION('',(0.,0.0274946291024905,-0.99962195122482));
#19943=DIRECTION('center_axis',(-0.707106781186547,-0.706839460333999,-0.01944163868458));
#19944=DIRECTION('ref_axis',(-0.0274842426448098,0.,0.999622236850622));
#19945=DIRECTION('',(0.648510052987376,-0.659223811296841,0.380603044908442));
#19946=DIRECTION('',(0.,0.0274946291024905,-0.99962195122482));
#19947=DIRECTION('',(0.691947206789735,-0.697348317654213,0.18685391855865));
#19948=DIRECTION('center_axis',(-0.707106781186547,-0.336582777174955,0.621861748388816));
#19949=DIRECTION('ref_axis',(0.660393123266679,0.,0.750920050832364));
#19950=DIRECTION('',(0.,0.879445318492508,0.475999928342023));
#19951=DIRECTION('',(0.,-0.879445318492508,-0.475999928342023));
#19952=DIRECTION('center_axis',(0.,1.,-2.60630817828214E-15));
#19953=DIRECTION('ref_axis',(0.,2.60630817828214E-15,1.));
#19954=DIRECTION('',(0.463876645871912,2.30892789648892E-15,0.885899801001572));
#19955=DIRECTION('',(1.,0.,0.));
#19956=DIRECTION('',(0.,2.60630817828214E-15,1.));
#19957=DIRECTION('',(-1.,0.,0.));
#19958=DIRECTION('',(-0.46387664587191,2.30892789648892E-15,0.885899801001573));
#19959=DIRECTION('center_axis',(0.,0.851950689390018,0.523622022882797));
#19960=DIRECTION('ref_axis',(0.,-0.523622022882797,0.851950689390018));
#19961=DIRECTION('',(0.,0.523622022882797,-0.851950689390018));
#19962=DIRECTION('',(1.,0.,0.));
#19963=DIRECTION('',(0.,-0.523622022882797,0.851950689390018));
#19964=DIRECTION('center_axis',(-0.707106781186548,0.602420109704236,0.370256683159043));
#19965=DIRECTION('ref_axis',(0.463876645871911,0.,0.885899801001573));
#19966=DIRECTION('',(0.648510052987376,0.761206089816885,1.19998465421244E-15));
#19967=DIRECTION('',(0.,-0.523622022882797,0.851950689390018));
#19968=DIRECTION('center_axis',(-0.707106781186547,0.602420109704236,-0.370256683159044));
#19969=DIRECTION('ref_axis',(-0.463876645871911,0.,0.885899801001572));
#19970=DIRECTION('',(0.,-0.523622022882797,-0.851950689390018));
#19971=DIRECTION('',(-0.691947206789734,-0.697348317654214,0.186853918558648));
#19972=DIRECTION('',(0.,0.523622022882797,0.851950689390018));
#19973=DIRECTION('center_axis',(0.,0.866025403784438,-0.500000000000001));
#19974=DIRECTION('ref_axis',(-1.,0.,0.));
#19975=DIRECTION('',(0.463876645871911,0.442949900500787,0.76721173287494));
#19976=DIRECTION('',(1.,0.,0.));
#19977=DIRECTION('',(0.,0.500000000000001,0.866025403784438));
#19978=DIRECTION('',(-1.,0.,0.));
#19979=DIRECTION('',(-0.46387664587191,0.442949900500787,0.76721173287494));
#19980=DIRECTION('center_axis',(0.,0.99962195122482,0.0274946291024892));
#19981=DIRECTION('ref_axis',(0.,-0.0274946291024892,0.99962195122482));
#19982=DIRECTION('',(0.,0.0274946291024892,-0.99962195122482));
#19983=DIRECTION('',(1.,0.,0.));
#19984=DIRECTION('',(0.,-0.0274946291024892,0.99962195122482));
#19985=DIRECTION('center_axis',(-0.707106781186548,0.706839460333999,0.0194416386845791));
#19986=DIRECTION('ref_axis',(0.0274842426448084,0.,0.999622236850622));
#19987=DIRECTION('',(0.648510052987375,0.659223811296841,-0.380603044908443));
#19988=DIRECTION('',(0.,-0.0274946291024892,0.99962195122482));
#19989=DIRECTION('center_axis',(0.,0.5,-0.866025403784439));
#19990=DIRECTION('ref_axis',(-1.,0.,0.));
#19991=DIRECTION('',(0.463876645871911,0.76721173287494,0.442949900500786));
#19992=DIRECTION('',(1.,0.,0.));
#19993=DIRECTION('',(0.,0.866025403784439,0.5));
#19994=DIRECTION('',(-1.,0.,0.));
#19995=DIRECTION('',(-0.46387664587191,0.767211732874941,0.442949900500786));
#19996=DIRECTION('center_axis',(0.,0.879445318492508,-0.475999928342023));
#19997=DIRECTION('ref_axis',(0.,0.475999928342023,0.879445318492508));
#19998=DIRECTION('',(0.,-0.475999928342023,-0.879445318492508));
#19999=DIRECTION('',(1.,0.,0.));
#20000=DIRECTION('',(0.,0.475999928342023,0.879445318492508));
#20001=DIRECTION('center_axis',(-0.707106781186547,0.621861748388816,-0.336582777174955));
#20002=DIRECTION('ref_axis',(-0.429793326728032,0.,0.902927292920117));
#20003=DIRECTION('',(0.648510052987376,0.380603044908442,-0.659223811296841));
#20004=DIRECTION('',(0.,0.475999928342023,0.879445318492508));
#20005=DIRECTION('',(0.691947206789734,0.510494399095564,-0.510494399095566));
#20006=DIRECTION('center_axis',(-0.707106781186548,-0.0194416386845788,
-0.706839460333999));
#20007=DIRECTION('ref_axis',(-0.706973082855489,0.,0.707240454242973));
#20008=DIRECTION('',(0.,-0.99962195122482,0.0274946291024888));
#20009=DIRECTION('',(0.691947206789735,0.186853918558646,-0.697348317654214));
#20010=DIRECTION('',(0.,0.99962195122482,-0.0274946291024888));
#20011=DIRECTION('center_axis',(0.,-2.60630817828214E-15,-1.));
#20012=DIRECTION('ref_axis',(-1.,0.,0.));
#20013=DIRECTION('',(0.463876645871913,0.885899801001571,-2.30892789648892E-15));
#20014=DIRECTION('',(1.,0.,0.));
#20015=DIRECTION('',(0.,1.,-2.60630817828214E-15));
#20016=DIRECTION('',(-1.,0.,0.));
#20017=DIRECTION('',(-0.46387664587191,0.885899801001573,-2.30892789648892E-15));
#20018=DIRECTION('center_axis',(0.,0.523622022882797,-0.851950689390019));
#20019=DIRECTION('ref_axis',(0.,0.851950689390018,0.523622022882797));
#20020=DIRECTION('',(0.,-0.851950689390018,-0.523622022882797));
#20021=DIRECTION('',(1.,0.,0.));
#20022=DIRECTION('',(0.,0.851950689390018,0.523622022882797));
#20023=DIRECTION('center_axis',(-0.707106781186547,0.370256683159044,-0.602420109704237));
#20024=DIRECTION('ref_axis',(-0.648510052987376,0.,0.761206089816884));
#20025=DIRECTION('',(0.648510052987376,-2.3549776941208E-15,-0.761206089816885));
#20026=DIRECTION('',(0.,0.851950689390018,0.523622022882797));
#20027=DIRECTION('center_axis',(-0.707106781186548,-0.370256683159044,-0.602420109704236));
#20028=DIRECTION('ref_axis',(-0.648510052987375,0.,0.761206089816885));
#20029=DIRECTION('',(0.,-0.851950689390018,0.523622022882798));
#20030=DIRECTION('',(0.691947206789734,-0.186853918558651,-0.697348317654214));
#20031=DIRECTION('',(0.,0.851950689390018,-0.523622022882798));
#20032=DIRECTION('center_axis',(0.,-0.500000000000001,-0.866025403784438));
#20033=DIRECTION('ref_axis',(-1.,0.,0.));
#20034=DIRECTION('',(0.463876645871911,0.76721173287494,-0.442949900500787));
#20035=DIRECTION('',(1.,0.,0.));
#20036=DIRECTION('',(0.,0.866025403784438,-0.500000000000001));
#20037=DIRECTION('',(-1.,0.,0.));
#20038=DIRECTION('',(-0.46387664587191,0.767211732874941,-0.442949900500787));
#20039=DIRECTION('center_axis',(0.,0.0274946291024892,-0.99962195122482));
#20040=DIRECTION('ref_axis',(0.,0.99962195122482,0.0274946291024892));
#20041=DIRECTION('',(0.,-0.99962195122482,-0.0274946291024892));
#20042=DIRECTION('',(1.,0.,0.));
#20043=DIRECTION('',(0.,0.99962195122482,0.0274946291024892));
#20044=DIRECTION('center_axis',(-0.707106781186548,0.0194416386845791,-0.706839460333999));
#20045=DIRECTION('ref_axis',(-0.706973082855489,0.,0.707240454242973));
#20046=DIRECTION('',(0.648510052987375,-0.380603044908443,-0.659223811296841));
#20047=DIRECTION('',(0.,0.99962195122482,0.0274946291024892));
#20048=DIRECTION('center_axis',(-0.707106781186548,-0.621861748388815,-0.336582777174955));
#20049=DIRECTION('ref_axis',(-0.429793326728032,0.,0.902927292920117));
#20050=DIRECTION('',(0.,-0.475999928342023,0.879445318492508));
#20051=DIRECTION('',(0.691947206789734,-0.510494399095568,-0.510494399095563));
#20052=DIRECTION('',(0.,0.475999928342023,-0.879445318492508));
#20053=DIRECTION('center_axis',(0.,-0.866025403784438,-0.5));
#20054=DIRECTION('ref_axis',(-1.,0.,0.));
#20055=DIRECTION('',(0.463876645871911,0.442949900500787,-0.76721173287494));
#20056=DIRECTION('',(1.,0.,0.));
#20057=DIRECTION('',(0.,0.5,-0.866025403784438));
#20058=DIRECTION('',(-1.,0.,0.));
#20059=DIRECTION('',(-0.463876645871912,0.442949900500786,-0.76721173287494));
#20060=DIRECTION('center_axis',(0.,-0.475999928342023,-0.879445318492508));
#20061=DIRECTION('ref_axis',(0.,0.879445318492508,-0.475999928342023));
#20062=DIRECTION('',(0.,-0.879445318492508,0.475999928342023));
#20063=DIRECTION('',(1.,0.,0.));
#20064=DIRECTION('',(0.,0.879445318492508,-0.475999928342023));
#20065=DIRECTION('center_axis',(-0.707106781186547,-0.336582777174955,-0.621861748388816));
#20066=DIRECTION('ref_axis',(-0.660393123266679,0.,0.750920050832364));
#20067=DIRECTION('',(0.648510052987376,-0.659223811296841,-0.380603044908442));
#20068=DIRECTION('',(0.,0.879445318492508,-0.475999928342023));
#20069=DIRECTION('center_axis',(-0.707106781186547,-0.706839460333999,0.0194416386845794));
#20070=DIRECTION('ref_axis',(0.027484242644809,0.,0.999622236850622));
#20071=DIRECTION('',(0.,0.0274946291024896,0.99962195122482));
#20072=DIRECTION('',(0.691947206789735,-0.697348317654213,-0.18685391855865));
#20073=DIRECTION('',(0.,-0.0274946291024896,-0.99962195122482));
#20074=DIRECTION('center_axis',(0.,-1.,0.));
#20075=DIRECTION('ref_axis',(0.,0.,-1.));
#20076=DIRECTION('',(0.463876645871911,0.,-0.885899801001572));
#20077=DIRECTION('',(1.,0.,0.));
#20078=DIRECTION('',(0.,0.,-1.));
#20079=DIRECTION('',(-1.,0.,0.));
#20080=DIRECTION('',(-0.463876645871911,0.,-0.885899801001572));
#20081=DIRECTION('center_axis',(0.,-0.851950689390019,-0.523622022882797));
#20082=DIRECTION('ref_axis',(0.,0.523622022882797,-0.851950689390018));
#20083=DIRECTION('',(0.,-0.523622022882797,0.851950689390018));
#20084=DIRECTION('',(1.,0.,0.));
#20085=DIRECTION('',(0.,0.523622022882797,-0.851950689390018));
#20086=DIRECTION('center_axis',(-0.707106781186547,-0.602420109704237,-0.370256683159044));
#20087=DIRECTION('ref_axis',(-0.463876645871911,0.,0.885899801001572));
#20088=DIRECTION('',(0.648510052987376,-0.761206089816884,-4.29989294273536E-16));
#20089=DIRECTION('',(0.,0.523622022882797,-0.851950689390018));
#20090=DIRECTION('center_axis',(-0.707106781186547,-0.602420109704237,0.370256683159044));
#20091=DIRECTION('ref_axis',(0.463876645871911,0.,0.885899801001572));
#20092=DIRECTION('',(0.,0.523622022882797,0.851950689390018));
#20093=DIRECTION('',(0.,-0.523622022882797,-0.851950689390018));
#20094=DIRECTION('center_axis',(-1.,0.,0.));
#20095=DIRECTION('ref_axis',(0.,1.,0.));
#20096=DIRECTION('center_axis',(-1.,0.,0.));
#20097=DIRECTION('ref_axis',(0.,1.,0.));
#20098=DIRECTION('center_axis',(1.,0.,0.));
#20099=DIRECTION('ref_axis',(0.,1.,0.));
#20100=DIRECTION('center_axis',(1.,0.,0.));
#20101=DIRECTION('ref_axis',(0.,1.,0.));
#20102=DIRECTION('center_axis',(1.,0.,0.));
#20103=DIRECTION('ref_axis',(0.,0.,-1.));
#20104=DIRECTION('center_axis',(-1.,0.,0.));
#20105=DIRECTION('ref_axis',(0.,0.866025403784439,0.5));
#20106=DIRECTION('center_axis',(-1.,0.,0.));
#20107=DIRECTION('ref_axis',(0.,0.866025403784439,0.5));
#20108=DIRECTION('center_axis',(1.,0.,0.));
#20109=DIRECTION('ref_axis',(0.,0.866025403784439,0.5));
#20110=DIRECTION('center_axis',(1.,0.,0.));
#20111=DIRECTION('ref_axis',(0.,0.866025403784439,0.5));
#20112=DIRECTION('center_axis',(1.,0.,0.));
#20113=DIRECTION('ref_axis',(0.,0.5,-0.866025403784439));
#20114=DIRECTION('center_axis',(-1.,0.,0.));
#20115=DIRECTION('ref_axis',(0.,0.5,0.866025403784438));
#20116=DIRECTION('center_axis',(-1.,0.,0.));
#20117=DIRECTION('ref_axis',(0.,0.5,0.866025403784439));
#20118=DIRECTION('center_axis',(1.,0.,0.));
#20119=DIRECTION('ref_axis',(0.,0.5,0.866025403784439));
#20120=DIRECTION('center_axis',(1.,0.,0.));
#20121=DIRECTION('ref_axis',(0.,0.5,0.866025403784439));
#20122=DIRECTION('center_axis',(1.,0.,0.));
#20123=DIRECTION('ref_axis',(0.,0.866025403784439,-0.5));
#20124=DIRECTION('center_axis',(-1.,0.,0.));
#20125=DIRECTION('ref_axis',(0.,6.12323399573677E-17,1.));
#20126=DIRECTION('center_axis',(-1.,0.,0.));
#20127=DIRECTION('ref_axis',(0.,6.12323399573677E-17,1.));
#20128=DIRECTION('center_axis',(1.,0.,0.));
#20129=DIRECTION('ref_axis',(0.,6.12323399573677E-17,1.));
#20130=DIRECTION('center_axis',(1.,0.,0.));
#20131=DIRECTION('ref_axis',(0.,6.12323399573677E-17,1.));
#20132=DIRECTION('center_axis',(1.,0.,0.));
#20133=DIRECTION('ref_axis',(0.,1.,-6.12323399573677E-17));
#20134=DIRECTION('center_axis',(-1.,0.,0.));
#20135=DIRECTION('ref_axis',(0.,-0.5,0.866025403784439));
#20136=DIRECTION('center_axis',(-1.,0.,0.));
#20137=DIRECTION('ref_axis',(0.,-0.5,0.866025403784439));
#20138=DIRECTION('center_axis',(1.,0.,0.));
#20139=DIRECTION('ref_axis',(0.,-0.5,0.866025403784439));
#20140=DIRECTION('center_axis',(1.,0.,0.));
#20141=DIRECTION('ref_axis',(0.,-0.5,0.866025403784439));
#20142=DIRECTION('center_axis',(1.,0.,0.));
#20143=DIRECTION('ref_axis',(0.,0.866025403784439,0.5));
#20144=DIRECTION('center_axis',(-1.,0.,0.));
#20145=DIRECTION('ref_axis',(0.,-0.866025403784438,0.5));
#20146=DIRECTION('center_axis',(-1.,0.,0.));
#20147=DIRECTION('ref_axis',(0.,-0.866025403784439,0.5));
#20148=DIRECTION('center_axis',(1.,0.,0.));
#20149=DIRECTION('ref_axis',(0.,-0.866025403784439,0.5));
#20150=DIRECTION('center_axis',(1.,0.,0.));
#20151=DIRECTION('ref_axis',(0.,-0.866025403784438,0.5));
#20152=DIRECTION('center_axis',(1.,0.,0.));
#20153=DIRECTION('ref_axis',(0.,0.5,0.866025403784438));
#20154=DIRECTION('center_axis',(-1.,0.,0.));
#20155=DIRECTION('ref_axis',(0.,-1.,1.22464679914735E-16));
#20156=DIRECTION('center_axis',(-1.,0.,0.));
#20157=DIRECTION('ref_axis',(0.,-1.,1.22464679914735E-16));
#20158=DIRECTION('center_axis',(1.,0.,0.));
#20159=DIRECTION('ref_axis',(0.,-1.,1.22464679914735E-16));
#20160=DIRECTION('center_axis',(1.,0.,0.));
#20161=DIRECTION('ref_axis',(0.,-1.,1.22464679914735E-16));
#20162=DIRECTION('center_axis',(1.,0.,0.));
#20163=DIRECTION('ref_axis',(0.,1.22464679914735E-16,1.));
#20164=DIRECTION('center_axis',(-1.,0.,0.));
#20165=DIRECTION('ref_axis',(0.,-0.866025403784439,-0.5));
#20166=DIRECTION('center_axis',(-1.,0.,0.));
#20167=DIRECTION('ref_axis',(0.,-0.866025403784439,-0.5));
#20168=DIRECTION('center_axis',(1.,0.,0.));
#20169=DIRECTION('ref_axis',(0.,-0.866025403784439,-0.5));
#20170=DIRECTION('center_axis',(1.,0.,0.));
#20171=DIRECTION('ref_axis',(0.,-0.866025403784439,-0.5));
#20172=DIRECTION('center_axis',(1.,0.,0.));
#20173=DIRECTION('ref_axis',(0.,-0.5,0.866025403784439));
#20174=DIRECTION('center_axis',(-1.,0.,0.));
#20175=DIRECTION('ref_axis',(0.,-0.500000000000001,-0.866025403784438));
#20176=DIRECTION('center_axis',(-1.,0.,0.));
#20177=DIRECTION('ref_axis',(0.,-0.5,-0.866025403784438));
#20178=DIRECTION('center_axis',(1.,0.,0.));
#20179=DIRECTION('ref_axis',(0.,-0.5,-0.866025403784438));
#20180=DIRECTION('center_axis',(1.,0.,0.));
#20181=DIRECTION('ref_axis',(0.,-0.5,-0.866025403784438));
#20182=DIRECTION('center_axis',(1.,0.,0.));
#20183=DIRECTION('ref_axis',(0.,-0.866025403784438,0.5));
#20184=DIRECTION('center_axis',(-1.,0.,0.));
#20185=DIRECTION('ref_axis',(0.,-1.83697019872103E-16,-1.));
#20186=DIRECTION('center_axis',(-1.,0.,0.));
#20187=DIRECTION('ref_axis',(0.,-1.83697019872103E-16,-1.));
#20188=DIRECTION('center_axis',(1.,0.,0.));
#20189=DIRECTION('ref_axis',(0.,-1.83697019872103E-16,-1.));
#20190=DIRECTION('center_axis',(1.,0.,0.));
#20191=DIRECTION('ref_axis',(0.,-1.83697019872103E-16,-1.));
#20192=DIRECTION('center_axis',(1.,0.,0.));
#20193=DIRECTION('ref_axis',(0.,-1.,1.83697019872103E-16));
#20194=DIRECTION('center_axis',(-1.,0.,0.));
#20195=DIRECTION('ref_axis',(0.,0.499999999999999,-0.866025403784439));
#20196=DIRECTION('center_axis',(-1.,0.,0.));
#20197=DIRECTION('ref_axis',(0.,0.499999999999999,-0.866025403784439));
#20198=DIRECTION('center_axis',(1.,0.,0.));
#20199=DIRECTION('ref_axis',(0.,0.499999999999999,-0.866025403784439));
#20200=DIRECTION('center_axis',(1.,0.,0.));
#20201=DIRECTION('ref_axis',(0.,0.499999999999999,-0.866025403784439));
#20202=DIRECTION('center_axis',(1.,0.,0.));
#20203=DIRECTION('ref_axis',(0.,-0.866025403784439,-0.499999999999999));
#20204=DIRECTION('center_axis',(-1.,0.,0.));
#20205=DIRECTION('ref_axis',(0.,0.866025403784438,-0.500000000000001));
#20206=DIRECTION('center_axis',(-1.,0.,0.));
#20207=DIRECTION('ref_axis',(0.,0.866025403784438,-0.5));
#20208=DIRECTION('center_axis',(1.,0.,0.));
#20209=DIRECTION('ref_axis',(0.,0.866025403784438,-0.5));
#20210=DIRECTION('center_axis',(1.,0.,0.));
#20211=DIRECTION('ref_axis',(0.,0.866025403784438,-0.5));
#20212=DIRECTION('center_axis',(1.,0.,0.));
#20213=DIRECTION('ref_axis',(0.,-0.5,-0.866025403784438));
#20214=DIRECTION('center_axis',(1.,0.,0.));
#20215=DIRECTION('ref_axis',(0.,1.,0.));
#20216=DIRECTION('center_axis',(-1.,0.,0.));
#20217=DIRECTION('ref_axis',(0.,1.,0.));
#20218=DIRECTION('',(-0.707106781186546,0.707106781186549,8.65956056235495E-17));
#20219=DIRECTION('center_axis',(1.,0.,0.));
#20220=DIRECTION('ref_axis',(0.,1.,0.));
#20221=DIRECTION('center_axis',(1.,0.,0.));
#20222=DIRECTION('ref_axis',(0.,0.,-1.));
#20223=DIRECTION('center_axis',(1.,0.,0.));
#20224=DIRECTION('ref_axis',(0.,0.,-1.));
#20225=DIRECTION('center_axis',(1.,0.,0.));
#20226=DIRECTION('ref_axis',(0.,1.,0.));
#20227=DIRECTION('center_axis',(-1.,0.,0.));
#20228=DIRECTION('ref_axis',(0.,1.,0.));
#20229=DIRECTION('',(-1.,0.,0.));
#20230=DIRECTION('center_axis',(-1.,0.,0.));
#20231=DIRECTION('ref_axis',(0.,1.,0.));
#20232=DIRECTION('center_axis',(1.,0.,0.));
#20233=DIRECTION('ref_axis',(0.,1.,0.));
#20234=DIRECTION('',(0.707106781186546,0.707106781186549,-8.65956056235495E-17));
#20235=DIRECTION('center_axis',(-1.,0.,0.));
#20236=DIRECTION('ref_axis',(0.,1.,0.));
#20237=DIRECTION('center_axis',(-1.,0.,0.));
#20238=DIRECTION('ref_axis',(0.,0.,1.));
#20239=DIRECTION('center_axis',(1.,0.,0.));
#20240=DIRECTION('ref_axis',(0.,0.,-1.));
#20241=DIRECTION('center_axis',(1.,0.,0.));
#20242=DIRECTION('ref_axis',(0.,1.,0.));
#20243=DIRECTION('',(-1.,0.,0.));
#20244=DIRECTION('center_axis',(1.,0.,0.));
#20245=DIRECTION('ref_axis',(0.,0.,-1.));
#20246=DIRECTION('center_axis',(0.,0.999997730284958,0.00213059262460322));
#20247=DIRECTION('ref_axis',(0.,-0.00213059262460322,0.999997730284958));
#20248=DIRECTION('',(1.,0.,0.));
#20249=DIRECTION('',(-1.,0.,0.));
#20250=DIRECTION('center_axis',(1.,0.,0.));
#20251=DIRECTION('ref_axis',(0.,0.,-1.));
#20252=DIRECTION('center_axis',(1.,0.,0.));
#20253=DIRECTION('ref_axis',(0.,0.,-1.));
#20254=DIRECTION('center_axis',(-1.,0.,0.));
#20255=DIRECTION('ref_axis',(0.,0.,-1.));
#20256=DIRECTION('center_axis',(-1.,0.,0.));
#20257=DIRECTION('ref_axis',(0.,1.,0.));
#20258=DIRECTION('center_axis',(1.,0.,0.));
#20259=DIRECTION('ref_axis',(0.,0.,-1.));
#20260=DIRECTION('center_axis',(1.,0.,0.));
#20261=DIRECTION('ref_axis',(0.,0.,-1.));
#20262=DIRECTION('center_axis',(1.,0.,0.));
#20263=DIRECTION('ref_axis',(0.,1.,0.));
#20264=DIRECTION('center_axis',(1.,0.,0.));
#20265=DIRECTION('ref_axis',(0.,0.,-1.));
#20266=DIRECTION('center_axis',(1.,0.,0.));
#20267=DIRECTION('ref_axis',(0.,1.,0.));
#20268=DIRECTION('center_axis',(1.,0.,0.));
#20269=DIRECTION('ref_axis',(0.,0.,-1.));
#20270=DIRECTION('',(-1.,0.,0.));
#20271=DIRECTION('center_axis',(0.,0.501844012480496,0.864958141841255));
#20272=DIRECTION('ref_axis',(1.,0.,0.));
#20273=DIRECTION('',(1.,0.,0.));
#20274=DIRECTION('center_axis',(1.,0.,0.));
#20275=DIRECTION('ref_axis',(0.,0.5,-0.866025403784439));
#20276=DIRECTION('center_axis',(-1.,0.,0.));
#20277=DIRECTION('ref_axis',(0.,0.5,-0.866025403784439));
#20278=DIRECTION('center_axis',(1.,0.,0.));
#20279=DIRECTION('ref_axis',(0.,0.5,-0.866025403784439));
#20280=DIRECTION('center_axis',(0.,0.864958141841257,0.501844012480492));
#20281=DIRECTION('ref_axis',(1.,0.,0.));
#20282=DIRECTION('',(1.,0.,0.));
#20283=DIRECTION('',(-1.,0.,0.));
#20284=DIRECTION('center_axis',(-1.,0.,0.));
#20285=DIRECTION('ref_axis',(0.,1.,0.));
#20286=DIRECTION('center_axis',(1.,0.,0.));
#20287=DIRECTION('ref_axis',(0.,0.,-1.));
#20288=DIRECTION('center_axis',(1.,0.,0.));
#20289=DIRECTION('ref_axis',(0.,0.,-1.));
#20290=DIRECTION('center_axis',(1.,0.,0.));
#20291=DIRECTION('ref_axis',(0.,1.,0.));
#20292=DIRECTION('center_axis',(1.,0.,0.));
#20293=DIRECTION('ref_axis',(0.,0.,-1.));
#20294=DIRECTION('center_axis',(1.,0.,0.));
#20295=DIRECTION('ref_axis',(0.,1.,0.));
#20296=DIRECTION('center_axis',(1.,0.,0.));
#20297=DIRECTION('ref_axis',(0.,0.,-1.));
#20298=DIRECTION('',(-1.,0.,0.));
#20299=DIRECTION('center_axis',(0.,0.00213059262460321,0.999997730284958));
#20300=DIRECTION('ref_axis',(1.,0.,0.));
#20301=DIRECTION('',(1.,0.,0.));
#20302=DIRECTION('center_axis',(1.,0.,0.));
#20303=DIRECTION('ref_axis',(0.,0.866025403784439,-0.5));
#20304=DIRECTION('center_axis',(-1.,0.,0.));
#20305=DIRECTION('ref_axis',(0.,0.866025403784439,-0.5));
#20306=DIRECTION('center_axis',(1.,0.,0.));
#20307=DIRECTION('ref_axis',(0.,0.866025403784439,-0.5));
#20308=DIRECTION('center_axis',(0.,0.49815371780446,0.867088734465853));
#20309=DIRECTION('ref_axis',(1.,0.,0.));
#20310=DIRECTION('',(1.,0.,0.));
#20311=DIRECTION('',(-1.,0.,0.));
#20312=DIRECTION('center_axis',(-1.,0.,0.));
#20313=DIRECTION('ref_axis',(0.,1.,0.));
#20314=DIRECTION('center_axis',(1.,0.,0.));
#20315=DIRECTION('ref_axis',(0.,0.,-1.));
#20316=DIRECTION('center_axis',(1.,0.,0.));
#20317=DIRECTION('ref_axis',(0.,0.,-1.));
#20318=DIRECTION('center_axis',(1.,0.,0.));
#20319=DIRECTION('ref_axis',(0.,1.,0.));
#20320=DIRECTION('center_axis',(1.,0.,0.));
#20321=DIRECTION('ref_axis',(0.,0.,-1.));
#20322=DIRECTION('center_axis',(1.,0.,0.));
#20323=DIRECTION('ref_axis',(0.,1.,0.));
#20324=DIRECTION('center_axis',(1.,0.,0.));
#20325=DIRECTION('ref_axis',(0.,0.,-1.));
#20326=DIRECTION('',(-1.,0.,0.));
#20327=DIRECTION('center_axis',(0.,-0.498153717804456,0.867088734465855));
#20328=DIRECTION('ref_axis',(1.,0.,0.));
#20329=DIRECTION('',(1.,0.,0.));
#20330=DIRECTION('center_axis',(1.,0.,0.));
#20331=DIRECTION('ref_axis',(0.,1.,-6.12323399573676E-17));
#20332=DIRECTION('center_axis',(-1.,0.,0.));
#20333=DIRECTION('ref_axis',(0.,1.,-6.12323399573677E-17));
#20334=DIRECTION('center_axis',(1.,0.,0.));
#20335=DIRECTION('ref_axis',(0.,1.,-6.12323399573677E-17));
#20336=DIRECTION('center_axis',(0.,-0.00213059262459345,0.999997730284958));
#20337=DIRECTION('ref_axis',(1.,0.,0.));
#20338=DIRECTION('',(1.,0.,0.));
#20339=DIRECTION('',(-1.,0.,0.));
#20340=DIRECTION('center_axis',(-1.,0.,0.));
#20341=DIRECTION('ref_axis',(0.,1.,0.));
#20342=DIRECTION('center_axis',(1.,0.,0.));
#20343=DIRECTION('ref_axis',(0.,0.,-1.));
#20344=DIRECTION('center_axis',(1.,0.,0.));
#20345=DIRECTION('ref_axis',(0.,0.,-1.));
#20346=DIRECTION('center_axis',(1.,0.,0.));
#20347=DIRECTION('ref_axis',(0.,1.,0.));
#20348=DIRECTION('center_axis',(1.,0.,0.));
#20349=DIRECTION('ref_axis',(0.,0.,-1.));
#20350=DIRECTION('center_axis',(1.,0.,0.));
#20351=DIRECTION('ref_axis',(0.,1.,0.));
#20352=DIRECTION('center_axis',(1.,0.,0.));
#20353=DIRECTION('ref_axis',(0.,0.,-1.));
#20354=DIRECTION('',(-1.,0.,0.));
#20355=DIRECTION('center_axis',(0.,-0.864958141841252,0.5018440124805));
#20356=DIRECTION('ref_axis',(1.,0.,0.));
#20357=DIRECTION('',(1.,0.,0.));
#20358=DIRECTION('center_axis',(1.,0.,0.));
#20359=DIRECTION('ref_axis',(0.,0.866025403784439,0.5));
#20360=DIRECTION('center_axis',(-1.,0.,0.));
#20361=DIRECTION('ref_axis',(0.,0.866025403784439,0.5));
#20362=DIRECTION('center_axis',(1.,0.,0.));
#20363=DIRECTION('ref_axis',(0.,0.866025403784439,0.5));
#20364=DIRECTION('center_axis',(0.,-0.501844012480502,0.864958141841251));
#20365=DIRECTION('ref_axis',(1.,0.,0.));
#20366=DIRECTION('',(1.,0.,0.));
#20367=DIRECTION('',(-1.,0.,0.));
#20368=DIRECTION('center_axis',(-1.,0.,0.));
#20369=DIRECTION('ref_axis',(0.,1.,0.));
#20370=DIRECTION('center_axis',(1.,0.,0.));
#20371=DIRECTION('ref_axis',(0.,0.,-1.));
#20372=DIRECTION('center_axis',(1.,0.,0.));
#20373=DIRECTION('ref_axis',(0.,0.,-1.));
#20374=DIRECTION('center_axis',(1.,0.,0.));
#20375=DIRECTION('ref_axis',(0.,1.,0.));
#20376=DIRECTION('center_axis',(1.,0.,0.));
#20377=DIRECTION('ref_axis',(0.,0.,-1.));
#20378=DIRECTION('center_axis',(1.,0.,0.));
#20379=DIRECTION('ref_axis',(0.,1.,0.));
#20380=DIRECTION('center_axis',(1.,0.,0.));
#20381=DIRECTION('ref_axis',(0.,0.,-1.));
#20382=DIRECTION('',(-1.,0.,0.));
#20383=DIRECTION('center_axis',(0.,-0.999997730284958,0.00213059262460321));
#20384=DIRECTION('ref_axis',(0.,-0.00213059262460321,-0.999997730284958));
#20385=DIRECTION('',(1.,0.,0.));
#20386=DIRECTION('center_axis',(1.,0.,0.));
#20387=DIRECTION('ref_axis',(0.,0.5,0.866025403784438));
#20388=DIRECTION('center_axis',(-1.,0.,0.));
#20389=DIRECTION('ref_axis',(0.,0.5,0.866025403784438));
#20390=DIRECTION('center_axis',(1.,0.,0.));
#20391=DIRECTION('ref_axis',(0.,0.5,0.866025403784438));
#20392=DIRECTION('center_axis',(1.,0.,0.));
#20393=DIRECTION('ref_axis',(0.,0.,-1.));
#20394=DIRECTION('center_axis',(1.,0.,0.));
#20395=DIRECTION('ref_axis',(0.,0.,-1.));
#20396=DIRECTION('center_axis',(1.,0.,0.));
#20397=DIRECTION('ref_axis',(0.,1.22464679914735E-16,1.));
#20398=DIRECTION('center_axis',(1.,0.,0.));
#20399=DIRECTION('ref_axis',(0.,0.,-1.));
#20400=DIRECTION('center_axis',(1.,0.,0.));
#20401=DIRECTION('ref_axis',(0.,-0.5,0.866025403784439));
#20402=DIRECTION('center_axis',(1.,0.,0.));
#20403=DIRECTION('ref_axis',(0.,0.,-1.));
#20404=DIRECTION('center_axis',(1.,0.,0.));
#20405=DIRECTION('ref_axis',(0.,-0.866025403784438,0.500000000000001));
#20406=DIRECTION('center_axis',(1.,0.,0.));
#20407=DIRECTION('ref_axis',(0.,0.,-1.));
#20408=DIRECTION('center_axis',(1.,0.,0.));
#20409=DIRECTION('ref_axis',(0.,-1.,1.83697019872103E-16));
#20410=DIRECTION('center_axis',(1.,0.,0.));
#20411=DIRECTION('ref_axis',(0.,0.,-1.));
#20412=DIRECTION('center_axis',(1.,0.,0.));
#20413=DIRECTION('ref_axis',(0.,-0.866025403784439,-0.499999999999999));
#20414=DIRECTION('center_axis',(1.,0.,0.));
#20415=DIRECTION('ref_axis',(0.,0.,-1.));
#20416=DIRECTION('center_axis',(1.,0.,0.));
#20417=DIRECTION('ref_axis',(0.,-0.500000000000001,-0.866025403784438));
#20418=DIRECTION('center_axis',(1.,0.,0.));
#20419=DIRECTION('ref_axis',(0.,0.,-1.));
#20420=DIRECTION('center_axis',(1.,0.,0.));
#20421=DIRECTION('ref_axis',(0.,0.,-1.));
#20422=DIRECTION('center_axis',(-1.,0.,0.));
#20423=DIRECTION('ref_axis',(0.,-1.,-1.4619715404243E-10));
#20424=DIRECTION('center_axis',(1.,0.,0.));
#20425=DIRECTION('ref_axis',(0.,0.,-1.));
#20426=DIRECTION('center_axis',(0.,-0.867088734465855,0.498153717804456));
#20427=DIRECTION('ref_axis',(0.,-0.498153717804456,-0.867088734465855));
#20428=DIRECTION('',(-1.,0.,0.));
#20429=DIRECTION('',(1.,0.,0.));
#20430=DIRECTION('center_axis',(1.,0.,0.));
#20431=DIRECTION('ref_axis',(0.,0.5,-0.866025403784439));
#20432=DIRECTION('center_axis',(1.,0.,0.));
#20433=DIRECTION('ref_axis',(0.,0.5,-0.866025403784439));
#20434=DIRECTION('center_axis',(1.,0.,0.));
#20435=DIRECTION('ref_axis',(0.,0.,-1.));
#20436=DIRECTION('',(1.,0.,0.));
#20437=DIRECTION('center_axis',(1.,0.,0.));
#20438=DIRECTION('ref_axis',(0.,0.,-1.));
#20439=DIRECTION('center_axis',(0.,0.867088734465855,0.498153717804456));
#20440=DIRECTION('ref_axis',(0.,-0.498153717804456,0.867088734465855));
#20441=DIRECTION('',(-1.,0.,0.));
#20442=DIRECTION('center_axis',(1.,0.,0.));
#20443=DIRECTION('ref_axis',(0.,-1.,5.66553889764798E-16));
#20444=DIRECTION('center_axis',(1.,0.,0.));
#20445=DIRECTION('ref_axis',(0.,0.,-1.));
#20446=DIRECTION('center_axis',(1.,0.,0.));
#20447=DIRECTION('ref_axis',(0.,1.,0.));
#20448=DIRECTION('center_axis',(1.,0.,0.));
#20449=DIRECTION('ref_axis',(0.,0.,-1.));
#20450=DIRECTION('',(-1.,0.,0.));
#20451=DIRECTION('center_axis',(0.,-0.867088734465854,-0.498153717804458));
#20452=DIRECTION('ref_axis',(0.,0.498153717804458,-0.867088734465854));
#20453=DIRECTION('',(1.,0.,0.));
#20454=DIRECTION('center_axis',(1.,0.,0.));
#20455=DIRECTION('ref_axis',(0.,1.22464679914735E-16,1.));
#20456=DIRECTION('center_axis',(-1.,0.,0.));
#20457=DIRECTION('ref_axis',(0.,1.22464679914735E-16,1.));
#20458=DIRECTION('center_axis',(-1.,0.,0.));
#20459=DIRECTION('ref_axis',(0.,1.,0.));
#20460=DIRECTION('center_axis',(1.,0.,0.));
#20461=DIRECTION('ref_axis',(0.,0.,-1.));
#20462=DIRECTION('center_axis',(0.,-0.999997730284958,-0.00213059262459835));
#20463=DIRECTION('ref_axis',(0.,0.00213059262459835,-0.999997730284958));
#20464=DIRECTION('',(-1.,0.,0.));
#20465=DIRECTION('',(1.,0.,0.));
#20466=DIRECTION('center_axis',(1.,0.,0.));
#20467=DIRECTION('ref_axis',(0.,1.,0.));
#20468=DIRECTION('center_axis',(1.,0.,0.));
#20469=DIRECTION('ref_axis',(0.,0.,-1.));
#20470=DIRECTION('center_axis',(1.,0.,0.));
#20471=DIRECTION('ref_axis',(0.,1.,0.));
#20472=DIRECTION('center_axis',(1.,0.,0.));
#20473=DIRECTION('ref_axis',(0.,0.,-1.));
#20474=DIRECTION('',(-1.,0.,0.));
#20475=DIRECTION('center_axis',(0.,-0.501844012480502,-0.864958141841251));
#20476=DIRECTION('ref_axis',(-1.,0.,0.));
#20477=DIRECTION('',(1.,0.,0.));
#20478=DIRECTION('center_axis',(1.,0.,0.));
#20479=DIRECTION('ref_axis',(0.,-0.5,0.866025403784439));
#20480=DIRECTION('center_axis',(-1.,0.,0.));
#20481=DIRECTION('ref_axis',(0.,-0.5,0.866025403784439));
#20482=DIRECTION('center_axis',(-1.,0.,0.));
#20483=DIRECTION('ref_axis',(0.,1.,0.));
#20484=DIRECTION('center_axis',(1.,0.,0.));
#20485=DIRECTION('ref_axis',(0.,0.,-1.));
#20486=DIRECTION('center_axis',(0.,-0.864958141841251,-0.501844012480502));
#20487=DIRECTION('ref_axis',(-1.,0.,0.));
#20488=DIRECTION('',(-1.,0.,0.));
#20489=DIRECTION('',(1.,0.,0.));
#20490=DIRECTION('center_axis',(1.,0.,0.));
#20491=DIRECTION('ref_axis',(0.,1.,0.));
#20492=DIRECTION('center_axis',(1.,0.,0.));
#20493=DIRECTION('ref_axis',(0.,0.,-1.));
#20494=DIRECTION('center_axis',(1.,0.,0.));
#20495=DIRECTION('ref_axis',(0.,1.,0.));
#20496=DIRECTION('center_axis',(1.,0.,0.));
#20497=DIRECTION('ref_axis',(0.,0.,-1.));
#20498=DIRECTION('',(-1.,0.,0.));
#20499=DIRECTION('center_axis',(0.,-0.00213059262460321,-0.999997730284958));
#20500=DIRECTION('ref_axis',(-1.,0.,0.));
#20501=DIRECTION('',(1.,0.,0.));
#20502=DIRECTION('center_axis',(1.,0.,0.));
#20503=DIRECTION('ref_axis',(0.,-0.866025403784438,0.5));
#20504=DIRECTION('center_axis',(-1.,0.,0.));
#20505=DIRECTION('ref_axis',(0.,-0.866025403784438,0.5));
#20506=DIRECTION('center_axis',(-1.,0.,0.));
#20507=DIRECTION('ref_axis',(0.,1.,0.));
#20508=DIRECTION('center_axis',(1.,0.,0.));
#20509=DIRECTION('ref_axis',(0.,0.,-1.));
#20510=DIRECTION('center_axis',(0.,-0.498153717804456,-0.867088734465856));
#20511=DIRECTION('ref_axis',(-1.,0.,0.));
#20512=DIRECTION('',(-1.,0.,0.));
#20513=DIRECTION('',(1.,0.,0.));
#20514=DIRECTION('center_axis',(1.,0.,0.));
#20515=DIRECTION('ref_axis',(0.,1.,0.));
#20516=DIRECTION('center_axis',(1.,0.,0.));
#20517=DIRECTION('ref_axis',(0.,0.,-1.));
#20518=DIRECTION('center_axis',(1.,0.,0.));
#20519=DIRECTION('ref_axis',(0.,1.,0.));
#20520=DIRECTION('center_axis',(1.,0.,0.));
#20521=DIRECTION('ref_axis',(0.,0.,-1.));
#20522=DIRECTION('',(-1.,0.,0.));
#20523=DIRECTION('center_axis',(0.,0.498153717804458,-0.867088734465854));
#20524=DIRECTION('ref_axis',(-1.,0.,0.));
#20525=DIRECTION('',(1.,0.,0.));
#20526=DIRECTION('center_axis',(1.,0.,0.));
#20527=DIRECTION('ref_axis',(0.,-1.,1.83697019872103E-16));
#20528=DIRECTION('center_axis',(-1.,0.,0.));
#20529=DIRECTION('ref_axis',(0.,-1.,1.83697019872103E-16));
#20530=DIRECTION('center_axis',(-1.,0.,0.));
#20531=DIRECTION('ref_axis',(0.,1.,0.));
#20532=DIRECTION('center_axis',(1.,0.,0.));
#20533=DIRECTION('ref_axis',(0.,0.,-1.));
#20534=DIRECTION('center_axis',(0.,0.0021305926246276,-0.999997730284958));
#20535=DIRECTION('ref_axis',(-1.,0.,0.));
#20536=DIRECTION('',(-1.,0.,0.));
#20537=DIRECTION('',(1.,0.,0.));
#20538=DIRECTION('center_axis',(1.,0.,0.));
#20539=DIRECTION('ref_axis',(0.,1.,0.));
#20540=DIRECTION('center_axis',(1.,0.,0.));
#20541=DIRECTION('ref_axis',(0.,0.,-1.));
#20542=DIRECTION('center_axis',(1.,0.,0.));
#20543=DIRECTION('ref_axis',(0.,1.,0.));
#20544=DIRECTION('center_axis',(1.,0.,0.));
#20545=DIRECTION('ref_axis',(0.,0.,-1.));
#20546=DIRECTION('',(-1.,0.,0.));
#20547=DIRECTION('center_axis',(0.,0.864958141841252,-0.5018440124805));
#20548=DIRECTION('ref_axis',(-1.,0.,0.));
#20549=DIRECTION('',(1.,0.,0.));
#20550=DIRECTION('center_axis',(1.,0.,0.));
#20551=DIRECTION('ref_axis',(0.,-0.866025403784439,-0.499999999999999));
#20552=DIRECTION('center_axis',(-1.,0.,0.));
#20553=DIRECTION('ref_axis',(0.,-0.866025403784439,-0.499999999999999));
#20554=DIRECTION('center_axis',(-1.,0.,0.));
#20555=DIRECTION('ref_axis',(0.,1.,0.));
#20556=DIRECTION('center_axis',(1.,0.,0.));
#20557=DIRECTION('ref_axis',(0.,0.,-1.));
#20558=DIRECTION('center_axis',(0.,0.501844012480498,-0.864958141841254));
#20559=DIRECTION('ref_axis',(-1.,0.,0.));
#20560=DIRECTION('',(-1.,0.,0.));
#20561=DIRECTION('',(1.,0.,0.));
#20562=DIRECTION('center_axis',(1.,0.,0.));
#20563=DIRECTION('ref_axis',(0.,1.,0.));
#20564=DIRECTION('center_axis',(1.,0.,0.));
#20565=DIRECTION('ref_axis',(0.,0.,-1.));
#20566=DIRECTION('',(1.,0.,0.));
#20567=DIRECTION('center_axis',(1.,0.,0.));
#20568=DIRECTION('ref_axis',(0.,0.,-1.));
#20569=DIRECTION('center_axis',(1.,0.,0.));
#20570=DIRECTION('ref_axis',(0.,1.,0.));
#20571=DIRECTION('center_axis',(1.,0.,0.));
#20572=DIRECTION('ref_axis',(0.,0.,-1.));
#20573=DIRECTION('center_axis',(-1.,0.,0.));
#20574=DIRECTION('ref_axis',(0.,1.,0.));
#20575=DIRECTION('center_axis',(1.,0.,0.));
#20576=DIRECTION('ref_axis',(0.,1.,0.));
#20577=DIRECTION('center_axis',(1.,0.,0.));
#20578=DIRECTION('ref_axis',(0.,0.,-1.));
#20579=DIRECTION('center_axis',(1.,0.,0.));
#20580=DIRECTION('ref_axis',(0.,1.,0.));
#20581=DIRECTION('center_axis',(1.,0.,0.));
#20582=DIRECTION('ref_axis',(0.,0.,-1.));
#20583=DIRECTION('',(-1.,0.,0.));
#20584=DIRECTION('center_axis',(0.,0.999997730284958,-0.00213059262460321));
#20585=DIRECTION('ref_axis',(0.,0.00213059262460321,0.999997730284958));
#20586=DIRECTION('',(1.,0.,0.));
#20587=DIRECTION('center_axis',(1.,0.,0.));
#20588=DIRECTION('ref_axis',(0.,-0.5,-0.866025403784438));
#20589=DIRECTION('center_axis',(-1.,0.,0.));
#20590=DIRECTION('ref_axis',(0.,-0.5,-0.866025403784438));
#20591=DIRECTION('center_axis',(0.,0.867088734465856,-0.498153717804456));
#20592=DIRECTION('ref_axis',(0.,0.498153717804456,0.867088734465855));
#20593=DIRECTION('',(-1.,0.,0.));
#20594=DIRECTION('center_axis',(1.,0.,0.));
#20595=DIRECTION('ref_axis',(0.,1.,0.));
#20596=DIRECTION('center_axis',(1.,0.,0.));
#20597=DIRECTION('ref_axis',(0.,0.,-1.));
#20598=DIRECTION('center_axis',(1.,0.,0.));
#20599=DIRECTION('ref_axis',(0.,-0.5,-0.866025403784438));
#20600=DIRECTION('center_axis',(1.,0.,0.));
#20601=DIRECTION('ref_axis',(0.,-0.5,-0.866025403784438));
#20602=DIRECTION('center_axis',(1.,0.,0.));
#20603=DIRECTION('ref_axis',(0.,0.,-1.));
#20604=DIRECTION('center_axis',(-1.,0.,0.));
#20605=DIRECTION('ref_axis',(0.,1.,0.));
#20606=DIRECTION('center_axis',(-1.,0.,0.));
#20607=DIRECTION('ref_axis',(0.,1.,0.));
#20608=DIRECTION('center_axis',(1.,0.,0.));
#20609=DIRECTION('ref_axis',(0.,0.,-1.));
#20610=DIRECTION('center_axis',(1.,0.,0.));
#20611=DIRECTION('ref_axis',(0.,1.,0.));
#20612=DIRECTION('center_axis',(1.,0.,0.));
#20613=DIRECTION('ref_axis',(0.,1.,0.));
#20614=DIRECTION('center_axis',(-1.,0.,0.));
#20615=DIRECTION('ref_axis',(0.,1.,1.0886778522233E-13));
#20616=DIRECTION('center_axis',(1.,0.,0.));
#20617=DIRECTION('ref_axis',(0.,1.,1.0886778522233E-13));
#20618=DIRECTION('center_axis',(1.,0.,0.));
#20619=DIRECTION('ref_axis',(0.,-0.5,-0.866025403784438));
#20620=DIRECTION('center_axis',(1.,0.,0.));
#20621=DIRECTION('ref_axis',(0.,0.,-1.));
#20622=DIRECTION('center_axis',(1.,0.,0.));
#20623=DIRECTION('ref_axis',(0.,1.,0.));
#20624=DIRECTION('center_axis',(1.,0.,0.));
#20625=DIRECTION('ref_axis',(0.,-0.866025403784439,-0.499999999999999));
#20626=DIRECTION('center_axis',(1.,0.,0.));
#20627=DIRECTION('ref_axis',(0.,-0.866025403784439,-0.499999999999999));
#20628=DIRECTION('center_axis',(1.,0.,0.));
#20629=DIRECTION('ref_axis',(0.,-0.866025403784439,-0.499999999999999));
#20630=DIRECTION('center_axis',(1.,0.,0.));
#20631=DIRECTION('ref_axis',(0.,1.,0.));
#20632=DIRECTION('center_axis',(1.,0.,0.));
#20633=DIRECTION('ref_axis',(0.,1.,0.));
#20634=DIRECTION('center_axis',(1.,0.,0.));
#20635=DIRECTION('ref_axis',(0.,-1.,1.83697019872103E-16));
#20636=DIRECTION('center_axis',(1.,0.,0.));
#20637=DIRECTION('ref_axis',(0.,-1.,1.83697019872103E-16));
#20638=DIRECTION('center_axis',(1.,0.,0.));
#20639=DIRECTION('ref_axis',(0.,-1.,1.83697019872103E-16));
#20640=DIRECTION('center_axis',(1.,0.,0.));
#20641=DIRECTION('ref_axis',(0.,1.,0.));
#20642=DIRECTION('center_axis',(1.,0.,0.));
#20643=DIRECTION('ref_axis',(0.,1.,0.));
#20644=DIRECTION('center_axis',(1.,0.,0.));
#20645=DIRECTION('ref_axis',(0.,-0.866025403784438,0.5));
#20646=DIRECTION('center_axis',(1.,0.,0.));
#20647=DIRECTION('ref_axis',(0.,-0.866025403784438,0.5));
#20648=DIRECTION('center_axis',(1.,0.,0.));
#20649=DIRECTION('ref_axis',(0.,-0.866025403784438,0.5));
#20650=DIRECTION('center_axis',(1.,0.,0.));
#20651=DIRECTION('ref_axis',(0.,1.,0.));
#20652=DIRECTION('center_axis',(1.,0.,0.));
#20653=DIRECTION('ref_axis',(0.,1.,0.));
#20654=DIRECTION('center_axis',(1.,0.,0.));
#20655=DIRECTION('ref_axis',(0.,-0.5,0.866025403784439));
#20656=DIRECTION('center_axis',(1.,0.,0.));
#20657=DIRECTION('ref_axis',(0.,-0.5,0.866025403784439));
#20658=DIRECTION('center_axis',(1.,0.,0.));
#20659=DIRECTION('ref_axis',(0.,-0.5,0.866025403784439));
#20660=DIRECTION('center_axis',(1.,0.,0.));
#20661=DIRECTION('ref_axis',(0.,1.,0.));
#20662=DIRECTION('center_axis',(1.,0.,0.));
#20663=DIRECTION('ref_axis',(0.,1.,0.));
#20664=DIRECTION('center_axis',(1.,0.,0.));
#20665=DIRECTION('ref_axis',(0.,1.22464679914735E-16,1.));
#20666=DIRECTION('center_axis',(1.,0.,0.));
#20667=DIRECTION('ref_axis',(0.,1.22464679914735E-16,1.));
#20668=DIRECTION('center_axis',(1.,0.,0.));
#20669=DIRECTION('ref_axis',(0.,1.22464679914735E-16,1.));
#20670=DIRECTION('center_axis',(1.,0.,0.));
#20671=DIRECTION('ref_axis',(0.,1.,0.));
#20672=DIRECTION('center_axis',(1.,0.,0.));
#20673=DIRECTION('ref_axis',(0.,1.,0.));
#20674=DIRECTION('center_axis',(1.,0.,0.));
#20675=DIRECTION('ref_axis',(0.,0.5,0.866025403784438));
#20676=DIRECTION('center_axis',(1.,0.,0.));
#20677=DIRECTION('ref_axis',(0.,0.5,0.866025403784438));
#20678=DIRECTION('center_axis',(1.,0.,0.));
#20679=DIRECTION('ref_axis',(0.,0.5,0.866025403784438));
#20680=DIRECTION('center_axis',(1.,0.,0.));
#20681=DIRECTION('ref_axis',(0.,1.,0.));
#20682=DIRECTION('center_axis',(1.,0.,0.));
#20683=DIRECTION('ref_axis',(0.,1.,0.));
#20684=DIRECTION('center_axis',(1.,0.,0.));
#20685=DIRECTION('ref_axis',(0.,0.866025403784439,0.5));
#20686=DIRECTION('center_axis',(1.,0.,0.));
#20687=DIRECTION('ref_axis',(0.,0.866025403784439,0.5));
#20688=DIRECTION('center_axis',(1.,0.,0.));
#20689=DIRECTION('ref_axis',(0.,0.866025403784439,0.5));
#20690=DIRECTION('center_axis',(1.,0.,0.));
#20691=DIRECTION('ref_axis',(0.,1.,0.));
#20692=DIRECTION('center_axis',(1.,0.,0.));
#20693=DIRECTION('ref_axis',(0.,1.,0.));
#20694=DIRECTION('center_axis',(1.,0.,0.));
#20695=DIRECTION('ref_axis',(0.,1.,-6.12323399573677E-17));
#20696=DIRECTION('center_axis',(1.,0.,0.));
#20697=DIRECTION('ref_axis',(0.,1.,-6.12323399573677E-17));
#20698=DIRECTION('center_axis',(1.,0.,0.));
#20699=DIRECTION('ref_axis',(0.,1.,-6.12323399573677E-17));
#20700=DIRECTION('center_axis',(1.,0.,0.));
#20701=DIRECTION('ref_axis',(0.,1.,0.));
#20702=DIRECTION('center_axis',(1.,0.,0.));
#20703=DIRECTION('ref_axis',(0.,1.,0.));
#20704=DIRECTION('center_axis',(1.,0.,0.));
#20705=DIRECTION('ref_axis',(0.,0.866025403784439,-0.5));
#20706=DIRECTION('center_axis',(1.,0.,0.));
#20707=DIRECTION('ref_axis',(0.,0.866025403784439,-0.5));
#20708=DIRECTION('center_axis',(1.,0.,0.));
#20709=DIRECTION('ref_axis',(0.,0.866025403784439,-0.5));
#20710=DIRECTION('center_axis',(1.,0.,0.));
#20711=DIRECTION('ref_axis',(0.,1.,0.));
#20712=DIRECTION('center_axis',(1.,0.,0.));
#20713=DIRECTION('ref_axis',(0.,1.,0.));
#20714=DIRECTION('center_axis',(1.,0.,0.));
#20715=DIRECTION('ref_axis',(0.,0.5,-0.866025403784439));
#20716=DIRECTION('center_axis',(1.,0.,0.));
#20717=DIRECTION('ref_axis',(0.,1.,0.));
#20718=DIRECTION('center_axis',(1.,0.,0.));
#20719=DIRECTION('ref_axis',(0.,1.,0.));
#20720=DIRECTION('center_axis',(1.,0.,0.));
#20721=DIRECTION('ref_axis',(0.,0.,-1.));
#20722=DIRECTION('center_axis',(1.,0.,0.));
#20723=DIRECTION('ref_axis',(0.,1.,0.));
#20724=DIRECTION('center_axis',(1.,0.,0.));
#20725=DIRECTION('ref_axis',(0.,1.,0.));
#20726=DIRECTION('center_axis',(1.,0.,0.));
#20727=DIRECTION('ref_axis',(0.,1.,0.));
#20728=DIRECTION('center_axis',(1.,0.,0.));
#20729=DIRECTION('ref_axis',(0.,0.,-1.));
#20730=DIRECTION('',(1.,0.,0.));
#20731=DIRECTION('center_axis',(1.,0.,0.));
#20732=DIRECTION('ref_axis',(0.,0.,-1.));
#20733=DIRECTION('center_axis',(-1.,0.,0.));
#20734=DIRECTION('ref_axis',(0.,0.,1.));
#20735=DIRECTION('center_axis',(1.,0.,0.));
#20736=DIRECTION('ref_axis',(0.,0.,-1.));
#20737=DIRECTION('center_axis',(1.,0.,0.));
#20738=DIRECTION('ref_axis',(0.,1.,0.));
#20739=DIRECTION('center_axis',(1.,0.,0.));
#20740=DIRECTION('ref_axis',(0.,1.,0.));
#20741=DIRECTION('center_axis',(1.,0.,0.));
#20742=DIRECTION('ref_axis',(0.,0.,-1.));
#20743=DIRECTION('',(-1.,0.,0.));
#20744=DIRECTION('center_axis',(1.,0.,0.));
#20745=DIRECTION('ref_axis',(0.,1.,0.));
#20746=DIRECTION('',(1.,0.,0.));
#20747=DIRECTION('center_axis',(-1.,0.,0.));
#20748=DIRECTION('ref_axis',(0.,0.5,0.866025403784438));
#20749=DIRECTION('center_axis',(1.,0.,0.));
#20750=DIRECTION('ref_axis',(0.,-0.5,-0.866025403784438));
#20751=DIRECTION('center_axis',(1.,0.,0.));
#20752=DIRECTION('ref_axis',(0.,-0.5,-0.866025403784438));
#20753=DIRECTION('center_axis',(-1.,0.,0.));
#20754=DIRECTION('ref_axis',(0.,0.866025403784439,0.499999999999999));
#20755=DIRECTION('center_axis',(1.,0.,0.));
#20756=DIRECTION('ref_axis',(0.,-0.866025403784439,-0.499999999999999));
#20757=DIRECTION('center_axis',(1.,0.,0.));
#20758=DIRECTION('ref_axis',(0.,-0.866025403784439,-0.499999999999999));
#20759=DIRECTION('center_axis',(-1.,0.,0.));
#20760=DIRECTION('ref_axis',(0.,1.,-1.83697019872103E-16));
#20761=DIRECTION('center_axis',(1.,0.,0.));
#20762=DIRECTION('ref_axis',(0.,-1.,1.83697019872103E-16));
#20763=DIRECTION('center_axis',(1.,0.,0.));
#20764=DIRECTION('ref_axis',(0.,-1.,1.83697019872103E-16));
#20765=DIRECTION('center_axis',(-1.,0.,0.));
#20766=DIRECTION('ref_axis',(0.,0.866025403784438,-0.5));
#20767=DIRECTION('center_axis',(1.,0.,0.));
#20768=DIRECTION('ref_axis',(0.,-0.866025403784438,0.5));
#20769=DIRECTION('center_axis',(1.,0.,0.));
#20770=DIRECTION('ref_axis',(0.,-0.866025403784438,0.5));
#20771=DIRECTION('center_axis',(-1.,0.,0.));
#20772=DIRECTION('ref_axis',(0.,0.5,-0.866025403784439));
#20773=DIRECTION('center_axis',(1.,0.,0.));
#20774=DIRECTION('ref_axis',(0.,-0.5,0.866025403784439));
#20775=DIRECTION('center_axis',(1.,0.,0.));
#20776=DIRECTION('ref_axis',(0.,-0.5,0.866025403784439));
#20777=DIRECTION('center_axis',(-1.,0.,0.));
#20778=DIRECTION('ref_axis',(0.,-1.22464679914735E-16,-1.));
#20779=DIRECTION('center_axis',(1.,0.,0.));
#20780=DIRECTION('ref_axis',(0.,1.22464679914735E-16,1.));
#20781=DIRECTION('center_axis',(1.,0.,0.));
#20782=DIRECTION('ref_axis',(0.,1.22464679914735E-16,1.));
#20783=DIRECTION('center_axis',(-1.,0.,0.));
#20784=DIRECTION('ref_axis',(0.,-0.5,-0.866025403784438));
#20785=DIRECTION('center_axis',(1.,0.,0.));
#20786=DIRECTION('ref_axis',(0.,0.5,0.866025403784438));
#20787=DIRECTION('center_axis',(1.,0.,0.));
#20788=DIRECTION('ref_axis',(0.,0.5,0.866025403784438));
#20789=DIRECTION('center_axis',(-1.,0.,0.));
#20790=DIRECTION('ref_axis',(0.,-0.866025403784439,-0.5));
#20791=DIRECTION('center_axis',(1.,0.,0.));
#20792=DIRECTION('ref_axis',(0.,0.866025403784439,0.5));
#20793=DIRECTION('center_axis',(1.,0.,0.));
#20794=DIRECTION('ref_axis',(0.,0.866025403784439,0.5));
#20795=DIRECTION('center_axis',(-1.,0.,0.));
#20796=DIRECTION('ref_axis',(0.,-1.,6.12323399573677E-17));
#20797=DIRECTION('center_axis',(1.,0.,0.));
#20798=DIRECTION('ref_axis',(0.,1.,-6.12323399573676E-17));
#20799=DIRECTION('center_axis',(1.,0.,0.));
#20800=DIRECTION('ref_axis',(0.,1.,-6.12323399573677E-17));
#20801=DIRECTION('center_axis',(-1.,0.,0.));
#20802=DIRECTION('ref_axis',(0.,-0.866025403784439,0.5));
#20803=DIRECTION('center_axis',(1.,0.,0.));
#20804=DIRECTION('ref_axis',(0.,0.866025403784439,-0.5));
#20805=DIRECTION('center_axis',(1.,0.,0.));
#20806=DIRECTION('ref_axis',(0.,0.866025403784439,-0.5));
#20807=DIRECTION('center_axis',(-1.,0.,0.));
#20808=DIRECTION('ref_axis',(0.,-0.5,0.866025403784439));
#20809=DIRECTION('center_axis',(1.,0.,0.));
#20810=DIRECTION('ref_axis',(0.,0.5,-0.866025403784439));
#20811=DIRECTION('center_axis',(1.,0.,0.));
#20812=DIRECTION('ref_axis',(0.,0.5,-0.866025403784439));
#20813=DIRECTION('center_axis',(-1.,0.,0.));
#20814=DIRECTION('ref_axis',(0.,0.,1.));
#20815=DIRECTION('center_axis',(1.,0.,0.));
#20816=DIRECTION('ref_axis',(0.,0.,-1.));
#20817=DIRECTION('center_axis',(1.,0.,0.));
#20818=DIRECTION('ref_axis',(0.,0.,-1.));
#20819=DIRECTION('center_axis',(-0.707106781186548,0.336582777174955,-0.621861748388816));
#20820=DIRECTION('ref_axis',(-0.660393123266679,0.,0.750920050832365));
#20821=DIRECTION('',(0.,-0.879445318492508,-0.475999928342022));
#20822=DIRECTION('',(0.,0.879445318492508,0.475999928342022));
#20823=DIRECTION('center_axis',(0.,-0.99962195122482,0.0274946291024896));
#20824=DIRECTION('ref_axis',(0.,-0.0274946291024896,-0.99962195122482));
#20825=DIRECTION('',(0.,-0.0274946291024896,-0.99962195122482));
#20826=DIRECTION('center_axis',(0.,-0.879445318492508,-0.475999928342023));
#20827=DIRECTION('ref_axis',(0.,0.475999928342023,-0.879445318492508));
#20828=DIRECTION('',(0.,0.475999928342023,-0.879445318492508));
#20829=DIRECTION('center_axis',(0.,-0.523622022882798,-0.851950689390018));
#20830=DIRECTION('ref_axis',(0.,0.851950689390018,-0.523622022882798));
#20831=DIRECTION('',(0.,0.851950689390018,-0.523622022882798));
#20832=DIRECTION('center_axis',(0.,-0.0274946291024888,-0.99962195122482));
#20833=DIRECTION('ref_axis',(0.,0.99962195122482,-0.0274946291024888));
#20834=DIRECTION('',(0.,0.99962195122482,-0.0274946291024888));
#20835=DIRECTION('center_axis',(0.,0.475999928342022,-0.879445318492509));
#20836=DIRECTION('ref_axis',(0.,0.879445318492508,0.475999928342022));
#20837=DIRECTION('',(0.,0.879445318492508,0.475999928342022));
#20838=DIRECTION('center_axis',(0.,0.851950689390018,-0.523622022882797));
#20839=DIRECTION('ref_axis',(0.,0.523622022882797,0.851950689390018));
#20840=DIRECTION('',(0.,0.523622022882797,0.851950689390018));
#20841=DIRECTION('center_axis',(1.,0.,0.));
#20842=DIRECTION('ref_axis',(0.,0.,-1.));
#20843=DIRECTION('center_axis',(0.,-0.475999928342023,0.879445318492508));
#20844=DIRECTION('ref_axis',(0.,-0.879445318492508,-0.475999928342023));
#20845=DIRECTION('',(0.,-0.879445318492508,-0.475999928342023));
#20846=DIRECTION('center_axis',(0.,0.0274946291024905,0.99962195122482));
#20847=DIRECTION('ref_axis',(0.,-0.99962195122482,0.0274946291024905));
#20848=DIRECTION('',(0.,-0.99962195122482,0.0274946291024905));
#20849=DIRECTION('center_axis',(0.,0.523622022882797,0.851950689390018));
#20850=DIRECTION('ref_axis',(0.,-0.851950689390018,0.523622022882797));
#20851=DIRECTION('',(0.,-0.851950689390018,0.523622022882797));
#20852=DIRECTION('center_axis',(0.,0.879445318492508,0.475999928342023));
#20853=DIRECTION('ref_axis',(0.,-0.475999928342023,0.879445318492508));
#20854=DIRECTION('',(0.,-0.475999928342023,0.879445318492508));
#20855=DIRECTION('center_axis',(0.,0.99962195122482,-0.0274946291024904));
#20856=DIRECTION('ref_axis',(0.,0.0274946291024904,0.99962195122482));
#20857=DIRECTION('',(0.,0.0274946291024904,0.99962195122482));
#20858=DIRECTION('center_axis',(0.,-0.851950689390018,0.523622022882797));
#20859=DIRECTION('ref_axis',(0.,-0.523622022882797,-0.851950689390018));
#20860=DIRECTION('',(0.,-0.523622022882797,-0.851950689390018));
#20861=DIRECTION('center_axis',(-1.,0.,0.));
#20862=DIRECTION('ref_axis',(0.,0.,1.));
#20863=DIRECTION('center_axis',(-1.,0.,0.));
#20864=DIRECTION('ref_axis',(0.,1.,0.));
#20865=DIRECTION('center_axis',(1.,0.,0.));
#20866=DIRECTION('ref_axis',(0.,0.,-1.));
#20867=DIRECTION('',(-0.330350424728107,-0.943858356366017,-1.15589311497212E-16));
#20868=DIRECTION('center_axis',(-1.,0.,0.));
#20869=DIRECTION('ref_axis',(0.,1.,0.));
#20870=DIRECTION('',(-0.49613893835683,-0.868243142124461,-1.06329118488436E-16));
#20871=DIRECTION('center_axis',(1.,0.,0.));
#20872=DIRECTION('ref_axis',(0.,1.,0.));
#20873=DIRECTION('',(-0.70710678118654,0.707106781186555,8.65956056235503E-17));
#20874=DIRECTION('center_axis',(-1.,0.,0.));
#20875=DIRECTION('ref_axis',(0.,1.,0.));
#20876=DIRECTION('center_axis',(1.,0.,0.));
#20877=DIRECTION('ref_axis',(0.,0.,-1.));
#20878=DIRECTION('',(-0.707106781186547,-0.707106781186547,-8.65956056235493E-17));
#20879=DIRECTION('center_axis',(1.,0.,0.));
#20880=DIRECTION('ref_axis',(0.,0.,-1.));
#20881=DIRECTION('center_axis',(1.,0.,0.));
#20882=DIRECTION('ref_axis',(0.,0.,-1.));
#20883=DIRECTION('center_axis',(-1.,0.,0.));
#20884=DIRECTION('ref_axis',(0.,1.,0.));
#20885=DIRECTION('center_axis',(1.,0.,0.));
#20886=DIRECTION('ref_axis',(0.,0.,-1.));
#20887=DIRECTION('',(-0.70710678118655,-0.707106781186546,-8.65956056235491E-17));
#20888=DIRECTION('center_axis',(-1.,0.,0.));
#20889=DIRECTION('ref_axis',(0.,1.,0.));
#20890=DIRECTION('center_axis',(1.,0.,0.));
#20891=DIRECTION('ref_axis',(0.,0.,-1.));
#20892=DIRECTION('',(-0.581238193719095,-0.813733471206736,-9.96536090872394E-17));
#20893=DIRECTION('center_axis',(1.,0.,0.));
#20894=DIRECTION('ref_axis',(0.,1.,0.));
#20895=DIRECTION('center_axis',(1.,0.,0.));
#20896=DIRECTION('ref_axis',(0.,0.,-1.));
#20897=DIRECTION('',(-1.,0.,0.));
#20898=DIRECTION('center_axis',(-1.,0.,0.));
#20899=DIRECTION('ref_axis',(0.,1.,0.));
#20900=DIRECTION('center_axis',(1.,0.,0.));
#20901=DIRECTION('ref_axis',(0.,0.,-1.));
#20902=DIRECTION('',(-0.70710678118654,-0.707106781186555,-8.65956056235503E-17));
#20903=DIRECTION('center_axis',(1.,0.,0.));
#20904=DIRECTION('ref_axis',(0.,0.,-1.));
#20905=DIRECTION('center_axis',(1.,0.,0.));
#20906=DIRECTION('ref_axis',(0.,0.,-1.));
#20907=DIRECTION('center_axis',(1.,0.,0.));
#20908=DIRECTION('ref_axis',(0.,1.,0.));
#20909=DIRECTION('center_axis',(1.,0.,0.));
#20910=DIRECTION('ref_axis',(0.,0.,-1.));
#20911=DIRECTION('',(-1.,0.,0.));
#20912=DIRECTION('center_axis',(1.,0.,0.));
#20913=DIRECTION('ref_axis',(0.,1.,0.));
#20914=DIRECTION('center_axis',(1.,0.,0.));
#20915=DIRECTION('ref_axis',(0.,0.,-1.));
#20916=DIRECTION('',(-0.707106781186571,0.707106781186524,8.65956056235465E-17));
#20917=DIRECTION('center_axis',(1.,0.,0.));
#20918=DIRECTION('ref_axis',(0.,1.,0.));
#20919=DIRECTION('center_axis',(1.,0.,0.));
#20920=DIRECTION('ref_axis',(0.,0.,-1.));
#20921=DIRECTION('',(-1.,0.,0.));
#20922=DIRECTION('center_axis',(-1.,0.,0.));
#20923=DIRECTION('ref_axis',(0.,1.,0.));
#20924=DIRECTION('center_axis',(1.,0.,0.));
#20925=DIRECTION('ref_axis',(0.,0.,-1.));
#20926=DIRECTION('',(-0.316227766016807,-0.948683298050524,-1.16180196436213E-16));
#20927=DIRECTION('center_axis',(1.,0.,0.));
#20928=DIRECTION('ref_axis',(0.,1.,0.));
#20929=DIRECTION('center_axis',(1.,0.,0.));
#20930=DIRECTION('ref_axis',(0.,0.,-1.));
#20931=DIRECTION('',(-1.,0.,0.));
#20932=DIRECTION('center_axis',(1.,0.,0.));
#20933=DIRECTION('ref_axis',(0.,1.,0.));
#20934=DIRECTION('',(-0.447213595499971,0.894427190999909,1.0953573965284E-16));
#20935=DIRECTION('center_axis',(1.,0.,0.));
#20936=DIRECTION('ref_axis',(0.,0.959653292014118,-0.281185986717806));
#20937=DIRECTION('center_axis',(-1.,0.,0.));
#20938=DIRECTION('ref_axis',(0.,1.,0.));
#20939=DIRECTION('center_axis',(-1.,0.,0.));
#20940=DIRECTION('ref_axis',(0.,1.,0.));
#20941=DIRECTION('center_axis',(1.,0.,0.));
#20942=DIRECTION('ref_axis',(0.,0.,-1.));
#20943=DIRECTION('',(-0.707106781186553,-0.707106781186542,-8.65956056235487E-17));
#20944=DIRECTION('center_axis',(1.,0.,0.));
#20945=DIRECTION('ref_axis',(0.,0.,-1.));
#23611=CARTESIAN_POINT('',(0.,0.,0.));
#23612=CARTESIAN_POINT('Origin',(165.,0.,0.));
#23613=CARTESIAN_POINT('',(157.293320454657,-3.44544707048975,0.00244461032172155));
#23614=CARTESIAN_POINT('',(157.148679545343,-3.4447563047016,0.00308232498356144));
#23615=CARTESIAN_POINT('',(165.,-3.442,-4.21523428266519E-16));
#23616=CARTESIAN_POINT('',(156.971,1.51264420613078,3.09472314487926));
#23617=CARTESIAN_POINT('Ctrl Pts',(157.293320454657,-3.44544707048975,0.00244461032172155));
#23618=CARTESIAN_POINT('Ctrl Pts',(157.286646439823,-3.44655406665934,0.146366209264783));
#23619=CARTESIAN_POINT('Ctrl Pts',(157.279972424989,-3.43831085885886,0.290155103803701));
#23620=CARTESIAN_POINT('Ctrl Pts',(157.273298410156,-3.42028738572634,0.432700406627246));
#23621=CARTESIAN_POINT('Ctrl Pts',(157.22068273819,-3.27819642943416,1.5564792834418));
#23622=CARTESIAN_POINT('Ctrl Pts',(157.168067066223,-2.52824130408745,2.6029663057877));
#23623=CARTESIAN_POINT('Ctrl Pts',(157.115451394257,-1.50964233980923,3.09927108189291));
#23624=CARTESIAN_POINT('Ctrl Pts',(157.067300929505,-0.577486354841783,
3.55345715868931));
#23625=CARTESIAN_POINT('Ctrl Pts',(157.019150464752,0.579651545136316,3.5468805548435));
#23626=CARTESIAN_POINT('Ctrl Pts',(156.971,1.5145057733605,3.09672906731558));
#23627=CARTESIAN_POINT('',(156.971,-1.51078263890264,3.09271722244216));
#23628=CARTESIAN_POINT('Origin',(156.971,0.,0.));
#23629=CARTESIAN_POINT('Ctrl Pts',(156.971,-1.51078263890258,3.0927172224422));
#23630=CARTESIAN_POINT('Ctrl Pts',(157.023615671966,-2.53321644899237,2.59326152099565));
#23631=CARTESIAN_POINT('Ctrl Pts',(157.076231343932,-3.27990605922292,1.5510599284818));
#23632=CARTESIAN_POINT('Ctrl Pts',(157.128847015898,-3.42018516348441,0.428800544168781));
#23633=CARTESIAN_POINT('Ctrl Pts',(157.135457859047,-3.43781039035294,0.287795393344797));
#23634=CARTESIAN_POINT('Ctrl Pts',(157.142068702195,-3.44586257045956,0.145526417146741));
#23635=CARTESIAN_POINT('Ctrl Pts',(157.148679545343,-3.4447563047016,0.00308232498356144));
#23636=CARTESIAN_POINT('Origin',(165.,0.,0.));
#23637=CARTESIAN_POINT('',(158.293320454657,-3.43670969417942,0.000689374022927458));
#23638=CARTESIAN_POINT('',(158.148679545343,-3.43671104026434,0.000722531392082319));
#23639=CARTESIAN_POINT('',(165.,-3.442,-4.21523428266519E-16));
#23640=CARTESIAN_POINT('Ctrl Pts',(158.293320454657,-3.43670969417942,0.000689374022927458));
#23641=CARTESIAN_POINT('Ctrl Pts',(158.269007138287,-3.43766262966877,0.528446666858329));
#23642=CARTESIAN_POINT('Ctrl Pts',(158.244693821917,-3.32341965147669,1.05581244132256));
#23643=CARTESIAN_POINT('Ctrl Pts',(158.220380505546,-3.09181810624384,1.52528055684926));
#23644=CARTESIAN_POINT('Ctrl Pts',(158.16776483358,-2.59061659406446,2.54124152198624));
#23645=CARTESIAN_POINT('Ctrl Pts',(158.115149161614,-1.53980253555905,3.28605671091484));
#23646=CARTESIAN_POINT('Ctrl Pts',(158.062533489648,-0.415180135400307,
3.42248722507319));
#23647=CARTESIAN_POINT('Ctrl Pts',(158.009917817682,0.709442264758436,3.55891773923153));
#23648=CARTESIAN_POINT('Ctrl Pts',(157.957302145716,1.90787300657052,3.08696357861963));
#23649=CARTESIAN_POINT('Ctrl Pts',(157.904686473749,2.63745093069739,2.22029759264997));
#23650=CARTESIAN_POINT('Ctrl Pts',(157.852070801783,3.36702885482427,1.35363160668031));
#23651=CARTESIAN_POINT('Ctrl Pts',(157.799455129817,3.62775396126593,0.0922537953528965));
#23652=CARTESIAN_POINT('Ctrl Pts',(157.746839457851,3.30159132076051,-0.992625515603271));
#23653=CARTESIAN_POINT('Ctrl Pts',(157.694223785885,2.97542868025509,-2.07750482655944));
#23654=CARTESIAN_POINT('Ctrl Pts',(157.641608113919,2.06237829280258,-2.98588563714436));
#23655=CARTESIAN_POINT('Ctrl Pts',(157.588992441953,0.975826462102337,-3.3065682899409));
#23656=CARTESIAN_POINT('Ctrl Pts',(157.536376769987,-0.110725368597905,
-3.62725094273743));
#23657=CARTESIAN_POINT('Ctrl Pts',(157.48376109802,-1.37077864254588,-3.36023543774558));
#23658=CARTESIAN_POINT('Ctrl Pts',(157.431145426054,-2.23369188590104,-2.62619231960805));
#23659=CARTESIAN_POINT('Ctrl Pts',(157.385203768922,-2.98714922816898,-1.98525862069813));
#23660=CARTESIAN_POINT('Ctrl Pts',(157.339262111789,-3.43782688387983,-0.988262919902665));
#23661=CARTESIAN_POINT('Ctrl Pts',(157.293320454657,-3.44544707048975,0.00244461032172155));
#23662=CARTESIAN_POINT('Ctrl Pts',(157.148679545343,-3.4447563047016,0.00308232498356144));
#23663=CARTESIAN_POINT('Ctrl Pts',(157.194684374161,-3.43705780608635,-0.988185495048805));
#23664=CARTESIAN_POINT('Ctrl Pts',(157.240689202979,-2.98583756510872,-1.98793376461549));
#23665=CARTESIAN_POINT('Ctrl Pts',(157.286694031797,-2.23081923614179,-2.62925913604816));
#23666=CARTESIAN_POINT('Ctrl Pts',(157.339309703763,-1.36730560624524,-3.36274225583985));
#23667=CARTESIAN_POINT('Ctrl Pts',(157.391925375729,-0.106409748159716,
-3.62739131931104));
#23668=CARTESIAN_POINT('Ctrl Pts',(157.444541047695,0.97989223421638,-3.30519505703097));
#23669=CARTESIAN_POINT('Ctrl Pts',(157.497156719662,2.06619421659248,-2.98299879475091));
#23670=CARTESIAN_POINT('Ctrl Pts',(157.549772391628,2.97790232325914,-2.07395720671959));
#23671=CARTESIAN_POINT('Ctrl Pts',(157.602388063594,3.3027072388958,-0.988797871088526));
#23672=CARTESIAN_POINT('Ctrl Pts',(157.65500373556,3.62751215453247,0.0963614645425373));
#23673=CARTESIAN_POINT('Ctrl Pts',(157.707619407526,3.36541387913912,1.35763854777334));
#23674=CARTESIAN_POINT('Ctrl Pts',(157.760235079492,2.63483694617998,2.22348839844289));
#23675=CARTESIAN_POINT('Ctrl Pts',(157.812850751458,1.90426001322083,3.08933824911244));
#23676=CARTESIAN_POINT('Ctrl Pts',(157.865466423424,0.705204422695883,3.55976086722073));
#23677=CARTESIAN_POINT('Ctrl Pts',(157.918082095391,-0.419270853672587,
3.42196497454828));
#23678=CARTESIAN_POINT('Ctrl Pts',(157.970697767357,-1.54374613004106,3.28416908187583));
#23679=CARTESIAN_POINT('Ctrl Pts',(158.023313439323,-2.59364109225305,2.53815467842265));
#23680=CARTESIAN_POINT('Ctrl Pts',(158.075929111289,-3.0936245505079,1.52161060115695));
#23681=CARTESIAN_POINT('Ctrl Pts',(158.100179255974,-3.32406294936394,1.0530935219133));
#23682=CARTESIAN_POINT('Ctrl Pts',(158.124429400658,-3.43768833393163,0.527110129590025));
#23683=CARTESIAN_POINT('Ctrl Pts',(158.148679545343,-3.43671104026434,0.000722531392082319));
#23684=CARTESIAN_POINT('Origin',(165.,0.,0.));
#23685=CARTESIAN_POINT('',(159.293320454657,-3.44310231280533,-0.00296426346809486));
#23686=CARTESIAN_POINT('',(159.148679545343,-3.44306193045544,-0.00296971903132968));
#23687=CARTESIAN_POINT('',(165.,-3.442,-4.21523428266519E-16));
#23688=CARTESIAN_POINT('Ctrl Pts',(159.293320454657,-3.44310231280533,-0.00296426346809486));
#23689=CARTESIAN_POINT('Ctrl Pts',(159.25136783675,-3.43491299719851,0.903398659033635));
#23690=CARTESIAN_POINT('Ctrl Pts',(159.209415218844,-3.06678173055999,1.81564946014422));
#23691=CARTESIAN_POINT('Ctrl Pts',(159.167462600937,-2.42463302112472,2.45091276876142));
#23692=CARTESIAN_POINT('Ctrl Pts',(159.114846928971,-1.61927002984871,3.24764030392345));
#23693=CARTESIAN_POINT('Ctrl Pts',(159.062231257005,-0.382894089265012,
3.6086831803192));
#23694=CARTESIAN_POINT('Ctrl Pts',(159.009615585039,0.724662800527638,3.37056108274876));
#23695=CARTESIAN_POINT('Ctrl Pts',(158.956999913072,1.83221969032029,3.13243898517832));
#23696=CARTESIAN_POINT('Ctrl Pts',(158.904384241106,2.81095752932189,2.2951519136417));
#23697=CARTESIAN_POINT('Ctrl Pts',(158.85176856914,3.21770283408525,1.23782374941761));
#23698=CARTESIAN_POINT('Ctrl Pts',(158.799152897174,3.62444813884861,0.180495585193521));
#23699=CARTESIAN_POINT('Ctrl Pts',(158.746537225208,3.45920090937374,-1.09687367171803));
#23700=CARTESIAN_POINT('Ctrl Pts',(158.693921553242,2.79678554937194,-2.0158892920362));
#23701=CARTESIAN_POINT('Ctrl Pts',(158.641305881276,2.13437018937015,-2.93490491235436));
#23702=CARTESIAN_POINT('Ctrl Pts',(158.588690209309,0.974786698841445,-3.49556689607912));
#23703=CARTESIAN_POINT('Ctrl Pts',(158.536074537343,-0.156905172830018,
-3.44400872313727));
#23704=CARTESIAN_POINT('Ctrl Pts',(158.483458865377,-1.28859704450148,-3.39245055019542));
#23705=CARTESIAN_POINT('Ctrl Pts',(158.430843193411,-2.3923972973157,-2.72867222058695));
#23706=CARTESIAN_POINT('Ctrl Pts',(158.378227521445,-2.96850294079614,-1.75322968511002));
#23707=CARTESIAN_POINT('Ctrl Pts',(158.349925165849,-3.27839438897766,-1.2285319957928));
#23708=CARTESIAN_POINT('Ctrl Pts',(158.321622810253,-3.43560041239042,-0.613656046518903));
#23709=CARTESIAN_POINT('Ctrl Pts',(158.293320454657,-3.43670969417942,0.000689374022927458));
#23710=CARTESIAN_POINT('Ctrl Pts',(158.148679545343,-3.43671104026434,0.000722531392082319));
#23711=CARTESIAN_POINT('Ctrl Pts',(158.177045072625,-3.43556789449997,-0.614995930146503));
#23712=CARTESIAN_POINT('Ctrl Pts',(158.205410599906,-3.27762411237375,-1.23126743057864));
#23713=CARTESIAN_POINT('Ctrl Pts',(158.233776127187,-2.96641712416019,-1.75676955526741));
#23714=CARTESIAN_POINT('Ctrl Pts',(158.286391799154,-2.38915428525994,-2.73153188334787));
#23715=CARTESIAN_POINT('Ctrl Pts',(158.33900747112,-1.28455665316172,-3.39398278843057));
#23716=CARTESIAN_POINT('Ctrl Pts',(158.391623143086,-0.152802192417,-3.44419016734183));
#23717=CARTESIAN_POINT('Ctrl Pts',(158.444238815052,0.97895226832773,-3.49439754625309));
#23718=CARTESIAN_POINT('Ctrl Pts',(158.496854487018,2.13786355771897,-2.9323613989929));
#23719=CARTESIAN_POINT('Ctrl Pts',(158.549470158984,2.79918318783638,-2.01255919133261));
#23720=CARTESIAN_POINT('Ctrl Pts',(158.602085830951,3.46050281795378,-1.09275698367232));
#23721=CARTESIAN_POINT('Ctrl Pts',(158.654701502917,3.62423078879735,0.184811284388065));
#23722=CARTESIAN_POINT('Ctrl Pts',(158.707317174883,3.21622720968354,1.24165519098984));
#23723=CARTESIAN_POINT('Ctrl Pts',(158.759932846849,2.80822363056973,2.29849909759162));
#23724=CARTESIAN_POINT('Ctrl Pts',(158.812548518815,1.82848850149854,3.13461864273479));
#23725=CARTESIAN_POINT('Ctrl Pts',(158.865164190781,0.720648566411499,3.37142136336576));
#23726=CARTESIAN_POINT('Ctrl Pts',(158.917779862748,-0.38719136867554,3.60822408399673));
#23727=CARTESIAN_POINT('Ctrl Pts',(158.970395534714,-1.62313610977842,3.2457099801155));
#23728=CARTESIAN_POINT('Ctrl Pts',(159.02301120668,-2.42754973893992,2.44802417358987));
#23729=CARTESIAN_POINT('Ctrl Pts',(159.064900652901,-3.06797568427348,1.81295451762713));
#23730=CARTESIAN_POINT('Ctrl Pts',(159.106790099122,-3.43488035732093,0.902056040806694));
#23731=CARTESIAN_POINT('Ctrl Pts',(159.148679545343,-3.44306193045544,-0.00296971903132968));
#23732=CARTESIAN_POINT('Origin',(165.,0.,0.));
#23733=CARTESIAN_POINT('',(160.293320454657,-3.44534347095755,0.00235542500143092));
#23734=CARTESIAN_POINT('',(160.148679545343,-3.44537846153824,0.0023402370110744));
#23735=CARTESIAN_POINT('',(165.,-3.442,-4.21523428266519E-16));
#23736=CARTESIAN_POINT('Ctrl Pts',(160.293320454657,-3.44534347095755,0.00235542500143092));
#23737=CARTESIAN_POINT('Ctrl Pts',(160.28634420718,-3.44652575450077,0.152819085738542));
#23738=CARTESIAN_POINT('Ctrl Pts',(160.279367959703,-3.43751163365742,0.303140213126026));
#23739=CARTESIAN_POINT('Ctrl Pts',(160.272391712226,-3.41781664333112,0.452048662995567));
#23740=CARTESIAN_POINT('Ctrl Pts',(160.21977604026,-3.26927472967131,1.57513355602034));
#23741=CARTESIAN_POINT('Ctrl Pts',(160.167160368294,-2.51316733167226,2.61786037503484));
#23742=CARTESIAN_POINT('Ctrl Pts',(160.114544696328,-1.49186052305688,3.10808152767139));
#23743=CARTESIAN_POINT('Ctrl Pts',(160.061929024361,-0.470553714441506,
3.59830268030795));
#23744=CARTESIAN_POINT('Ctrl Pts',(160.009313352395,0.815952504790201,3.53601816656657));
#23745=CARTESIAN_POINT('Ctrl Pts',(159.956697680429,1.78512702507273,2.9494304702973));
#23746=CARTESIAN_POINT('Ctrl Pts',(159.904082008463,2.75430154535527,2.36284277402803));
#23747=CARTESIAN_POINT('Ctrl Pts',(159.851466336497,3.40614436668863,1.25195189523086));
#23748=CARTESIAN_POINT('Ctrl Pts',(159.798850664531,3.44550050263555,0.119770162913145));
#23749=CARTESIAN_POINT('Ctrl Pts',(159.746234992565,3.48485663858247,-1.01241156940458));
#23750=CARTESIAN_POINT('Ctrl Pts',(159.693619320599,2.91172608914295,-2.16588415524284));
#23751=CARTESIAN_POINT('Ctrl Pts',(159.641003648632,1.98562285942401,-2.81835421390573));
#23752=CARTESIAN_POINT('Ctrl Pts',(159.588387976666,1.05951962970507,-3.47082427256861));
#23753=CARTESIAN_POINT('Ctrl Pts',(159.5357723047,-0.219556280293278,-3.6222918040561));
#23754=CARTESIAN_POINT('Ctrl Pts',(159.483156632734,-1.27243821963341,-3.20417220625212));
#23755=CARTESIAN_POINT('Ctrl Pts',(159.430540960768,-2.32532015897354,-2.78605260844815));
#23756=CARTESIAN_POINT('Ctrl Pts',(159.377925288802,-3.15200812765545,-1.79834588135271));
#23757=CARTESIAN_POINT('Ctrl Pts',(159.325309616835,-3.37817709101225,-0.688286420840833));
#23758=CARTESIAN_POINT('Ctrl Pts',(159.314646562776,-3.42401232969197,-0.463322572724454));
#23759=CARTESIAN_POINT('Ctrl Pts',(159.303983508716,-3.44518378279179,-0.233333602080165));
#23760=CARTESIAN_POINT('Ctrl Pts',(159.293320454657,-3.44310231280533,-0.00296426346809486));
#23761=CARTESIAN_POINT('Ctrl Pts',(159.148679545343,-3.44306193045544,-0.00296971903132968));
#23762=CARTESIAN_POINT('Ctrl Pts',(159.159405771088,-3.4451569068351,-0.234710920714154));
#23763=CARTESIAN_POINT('Ctrl Pts',(159.170131996833,-3.42373152283689,-0.466067066570195));
#23764=CARTESIAN_POINT('Ctrl Pts',(159.180858222578,-3.37735531801846,-0.692308646474397));
#23765=CARTESIAN_POINT('Ctrl Pts',(159.233473894544,-3.14986475071538,-1.80209815084305));
#23766=CARTESIAN_POINT('Ctrl Pts',(159.28608956651,-2.32200109888913,-2.78881965041033));
#23767=CARTESIAN_POINT('Ctrl Pts',(159.338705238477,-1.2686219519135,-3.20568519574602));
#23768=CARTESIAN_POINT('Ctrl Pts',(159.391320910443,-0.215242804937871,
-3.62255074108171));
#23769=CARTESIAN_POINT('Ctrl Pts',(159.443936582409,1.06365183718713,-3.4695603321858));
#23770=CARTESIAN_POINT('Ctrl Pts',(159.496552254375,1.98897750290621,-2.81598796579658));
#23771=CARTESIAN_POINT('Ctrl Pts',(159.549167926341,2.91430316862528,-2.16241559940735));
#23772=CARTESIAN_POINT('Ctrl Pts',(159.601783598307,3.48605985793843,-1.00826127552482));
#23773=CARTESIAN_POINT('Ctrl Pts',(159.654399270274,3.44535560072704,0.123872851661023));
#23774=CARTESIAN_POINT('Ctrl Pts',(159.70701494224,3.40465134351564,1.25600697884687));
#23775=CARTESIAN_POINT('Ctrl Pts',(159.759630614206,2.75148613977968,2.36612090933602));
#23776=CARTESIAN_POINT('Ctrl Pts',(159.812246286172,1.78161377659822,2.95155415751702));
#23777=CARTESIAN_POINT('Ctrl Pts',(159.864861958138,0.811741413416756,3.53698740569803));
#23778=CARTESIAN_POINT('Ctrl Pts',(159.917477630104,-0.474838109210224,
3.59773997157089));
#23779=CARTESIAN_POINT('Ctrl Pts',(159.97009330207,-1.49556050213205,3.10630301852266));
#23780=CARTESIAN_POINT('Ctrl Pts',(160.022708974037,-2.51628289505388,2.61486606547443));
#23781=CARTESIAN_POINT('Ctrl Pts',(160.075324646003,-3.27114815827057,1.57123959350512));
#23782=CARTESIAN_POINT('Ctrl Pts',(160.127940317969,-3.41835265168146,0.447978568532901));
#23783=CARTESIAN_POINT('Ctrl Pts',(160.13485339376,-3.43769357771655,0.30039538069199));
#23784=CARTESIAN_POINT('Ctrl Pts',(160.141766469552,-3.44654454951433,0.151437473833138));
#23785=CARTESIAN_POINT('Ctrl Pts',(160.148679545343,-3.44537846153824,0.0023402370110744));
#23786=CARTESIAN_POINT('Origin',(165.,0.,0.));
#23787=CARTESIAN_POINT('',(161.293320454657,-3.43667385388915,0.000584777541659254));
#23788=CARTESIAN_POINT('',(161.148679545343,-3.43668114569526,0.000606329579010968));
#23789=CARTESIAN_POINT('',(165.,-3.442,-4.21523428266519E-16));
#23790=CARTESIAN_POINT('Ctrl Pts',(161.293320454657,-3.43667385388915,0.000584777541659254));
#23791=CARTESIAN_POINT('Ctrl Pts',(161.268704905644,-3.43749408857896,0.534915952136021));
#23792=CARTESIAN_POINT('Ctrl Pts',(161.24408935663,-3.32026410406894,1.06890639556271));
#23793=CARTESIAN_POINT('Ctrl Pts',(161.219473807617,-3.0830792634662,1.54286773768467));
#23794=CARTESIAN_POINT('Ctrl Pts',(161.166858135651,-2.57609728383533,2.5559588732179));
#23795=CARTESIAN_POINT('Ctrl Pts',(161.114242463684,-1.52105414681311,3.29478334035705));
#23796=CARTESIAN_POINT('Ctrl Pts',(161.061626791718,-0.395674282548231,
3.42480079172139));
#23797=CARTESIAN_POINT('Ctrl Pts',(161.009011119752,0.729705581716644,3.55481824308572));
#23798=CARTESIAN_POINT('Ctrl Pts',(160.956395447786,1.92542217322419,3.07602867867524));
#23799=CARTESIAN_POINT('Ctrl Pts',(160.90377977582,2.65005400196605,2.20522842068367));
#23800=CARTESIAN_POINT('Ctrl Pts',(160.851164103854,3.37468583070791,1.33442816269211));
#23801=CARTESIAN_POINT('Ctrl Pts',(160.798548431887,3.62823289668411,0.0716172111194516));
#23802=CARTESIAN_POINT('Ctrl Pts',(160.745932759921,3.29588887265298,-1.01140256077362));
#23803=CARTESIAN_POINT('Ctrl Pts',(160.693317087955,2.96354484862186,-2.09442233266669));
#23804=CARTESIAN_POINT('Ctrl Pts',(160.640701415989,2.04530973458342,-2.99765092488018));
#23805=CARTESIAN_POINT('Ctrl Pts',(160.588085744023,0.956961171534698,-3.31210566215452));
#23806=CARTESIAN_POINT('Ctrl Pts',(160.535470072057,-0.131387391514026,
-3.62656039942887));
#23807=CARTESIAN_POINT('Ctrl Pts',(160.482854400091,-1.38984940357303,-3.35224128176408));
#23808=CARTESIAN_POINT('Ctrl Pts',(160.430238728125,-2.24859219494225,-2.61336023941416));
#23809=CARTESIAN_POINT('Ctrl Pts',(160.384599303635,-2.99347533180661,-1.97244652913118));
#23810=CARTESIAN_POINT('Ctrl Pts',(160.338959879146,-3.43760883415252,-0.981995389001479));
#23811=CARTESIAN_POINT('Ctrl Pts',(160.293320454657,-3.44534347095755,0.00235542500143092));
#23812=CARTESIAN_POINT('Ctrl Pts',(160.148679545343,-3.44537846153824,0.0023402370110744));
#23813=CARTESIAN_POINT('Ctrl Pts',(160.194382141518,-3.43766941140137,-0.983347033151559));
#23814=CARTESIAN_POINT('Ctrl Pts',(160.240084737693,-2.992156718107,-1.97512383126673));
#23815=CARTESIAN_POINT('Ctrl Pts',(160.285787333867,-2.24547881951396,-2.61603602984151));
#23816=CARTESIAN_POINT('Ctrl Pts',(160.338403005833,-1.38585677033047,-3.35389402526855));
#23817=CARTESIAN_POINT('Ctrl Pts',(160.3910186778,-0.127068948358405,-3.6267144381475));
#23818=CARTESIAN_POINT('Ctrl Pts',(160.443634349766,0.960904451181222,-3.31096395059576));
#23819=CARTESIAN_POINT('Ctrl Pts',(160.496250021732,2.04887785072085,-2.99521346304401));
#23820=CARTESIAN_POINT('Ctrl Pts',(160.548865693698,2.96603682782804,-2.09089207506157));
#23821=CARTESIAN_POINT('Ctrl Pts',(160.601481365664,3.29709101648908,-1.00747728196484));
#23822=CARTESIAN_POINT('Ctrl Pts',(160.65409703763,3.62814520515012,0.0759375111318684));
#23823=CARTESIAN_POINT('Ctrl Pts',(160.706712709597,3.37309460536501,1.33844570934286));
#23824=CARTESIAN_POINT('Ctrl Pts',(160.759328381563,2.64742634612698,2.20838252698244));
#23825=CARTESIAN_POINT('Ctrl Pts',(160.811944053529,1.92175808688896,3.07831934462203));
#23826=CARTESIAN_POINT('Ctrl Pts',(160.864559725495,0.725472168198008,3.55568478169021));
#23827=CARTESIAN_POINT('Ctrl Pts',(160.917175397461,-0.39975212828439,3.42432736177104));
#23828=CARTESIAN_POINT('Ctrl Pts',(160.969791069427,-1.52497642476679,3.29296994185187));
#23829=CARTESIAN_POINT('Ctrl Pts',(161.022406741393,-2.57913909904063,2.55288966494535));
#23830=CARTESIAN_POINT('Ctrl Pts',(161.07502241336,-3.08491439514982,1.53919551030916));
#23831=CARTESIAN_POINT('Ctrl Pts',(161.099574790687,-3.32092745835213,1.06616912007933));
#23832=CARTESIAN_POINT('Ctrl Pts',(161.124127168015,-3.43752952918348,0.533563487206253));
#23833=CARTESIAN_POINT('Ctrl Pts',(161.148679545343,-3.43668114569526,0.000606329579010967));
#23834=CARTESIAN_POINT('Origin',(165.,0.,0.));
#23835=CARTESIAN_POINT('',(162.293320454657,-3.4432958299264,-0.0029358085113948));
#23836=CARTESIAN_POINT('',(162.148679545343,-3.44325559759246,-0.00294208160319024));
#23837=CARTESIAN_POINT('',(165.,-3.442,-4.21523428266519E-16));
#23838=CARTESIAN_POINT('Ctrl Pts',(162.293320454657,-3.4432958299264,-0.0029358085113948));
#23839=CARTESIAN_POINT('Ctrl Pts',(162.251065604107,-3.43507546920982,0.909824409735672));
#23840=CARTESIAN_POINT('Ctrl Pts',(162.208810753557,-3.06104050140918,1.82854105791307));
#23841=CARTESIAN_POINT('Ctrl Pts',(162.166555903007,-2.41063103125263,2.46468590939444));
#23842=CARTESIAN_POINT('Ctrl Pts',(162.113940231041,-1.6007422047593,3.25681245564849));
#23843=CARTESIAN_POINT('Ctrl Pts',(162.061324559075,-0.362329451333632,
3.61080605212497));
#23844=CARTESIAN_POINT('Ctrl Pts',(162.008708887109,0.743852880554024,3.36637809713911));
#23845=CARTESIAN_POINT('Ctrl Pts',(161.956093215143,1.85003521244167,3.12195014215324));
#23846=CARTESIAN_POINT('Ctrl Pts',(161.903477543177,2.82398712279132,2.27910063570504));
#23847=CARTESIAN_POINT('Ctrl Pts',(161.850861871211,3.22470235789767,1.21947255146401));
#23848=CARTESIAN_POINT('Ctrl Pts',(161.798246199244,3.62541759300402,0.159844467222955));
#23849=CARTESIAN_POINT('Ctrl Pts',(161.745630527278,3.45289615286705,-1.11656219481094));
#23850=CARTESIAN_POINT('Ctrl Pts',(161.693014855312,2.78525589237232,-2.03178941202339));
#23851=CARTESIAN_POINT('Ctrl Pts',(161.640399183346,2.11761563187759,-2.94701662923583));
#23852=CARTESIAN_POINT('Ctrl Pts',(161.58778351138,0.954856551025132,-3.50106440162682));
#23853=CARTESIAN_POINT('Ctrl Pts',(161.535167839414,-0.176523049025896,
-3.44305942643655));
#23854=CARTESIAN_POINT('Ctrl Pts',(161.482552167448,-1.30790264907693,-3.38505445124627));
#23855=CARTESIAN_POINT('Ctrl Pts',(161.429936495481,-2.40790276832652,-2.71499672847472));
#23856=CARTESIAN_POINT('Ctrl Pts',(161.377320823515,-2.97844241683156,-1.73628896512529));
#23857=CARTESIAN_POINT('Ctrl Pts',(161.349320700562,-3.28206260660803,-1.21545673616016));
#23858=CARTESIAN_POINT('Ctrl Pts',(161.32132057761,-3.43574083906375,-0.607215543224034));
#23859=CARTESIAN_POINT('Ctrl Pts',(161.293320454657,-3.43667385388915,0.000584777541659254));
#23860=CARTESIAN_POINT('Ctrl Pts',(161.148679545343,-3.43668114569526,0.000606329579010967));
#23861=CARTESIAN_POINT('Ctrl Pts',(161.176742839981,-3.4357114458785,-0.608562124634891));
#23862=CARTESIAN_POINT('Ctrl Pts',(161.20480613462,-3.28129951189907,-1.21818982563464));
#23863=CARTESIAN_POINT('Ctrl Pts',(161.232869429258,-2.97637293604331,-1.73983441449399));
#23864=CARTESIAN_POINT('Ctrl Pts',(161.285485101224,-2.40466826288309,-2.71786215229505));
#23865=CARTESIAN_POINT('Ctrl Pts',(161.33810077319,-1.30387099861813,-3.38660959553132));
#23866=CARTESIAN_POINT('Ctrl Pts',(161.390716445156,-0.172423081110959,
-3.44326733285217));
#23867=CARTESIAN_POINT('Ctrl Pts',(161.443332117123,0.959024836396215,-3.49992507017301));
#23868=CARTESIAN_POINT('Ctrl Pts',(161.495947789089,2.1211234071456,-2.94449310157842));
#23869=CARTESIAN_POINT('Ctrl Pts',(161.548563461055,2.78767340950389,-2.02847149506462));
#23870=CARTESIAN_POINT('Ctrl Pts',(161.601179133021,3.45422341186218,-1.11244988855083));
#23871=CARTESIAN_POINT('Ctrl Pts',(161.653794804987,3.62522484582938,0.164161355882143));
#23872=CARTESIAN_POINT('Ctrl Pts',(161.706410476953,3.22324811661227,1.2233115805444));
#23873=CARTESIAN_POINT('Ctrl Pts',(161.75902614892,2.82127138739515,2.28246180520667));
#23874=CARTESIAN_POINT('Ctrl Pts',(161.811641820886,1.84631649499369,3.12415101009821));
#23875=CARTESIAN_POINT('Ctrl Pts',(161.864257492852,0.739843844237031,3.36726160707729));
#23876=CARTESIAN_POINT('Ctrl Pts',(161.916873164818,-0.366628806519617,
3.61037220405638));
#23877=CARTESIAN_POINT('Ctrl Pts',(161.969488836784,-1.60461921563146,3.25490419312303));
#23878=CARTESIAN_POINT('Ctrl Pts',(162.02210450875,-2.41356427249153,2.46181379208476));
#23879=CARTESIAN_POINT('Ctrl Pts',(162.064296187615,-3.06224457595425,1.82584708747844));
#23880=CARTESIAN_POINT('Ctrl Pts',(162.106487866479,-3.43504084200054,0.908481152668783));
#23881=CARTESIAN_POINT('Ctrl Pts',(162.148679545343,-3.44325559759246,-0.00294208160319024));
#23882=CARTESIAN_POINT('Origin',(165.,0.,0.));
#23883=CARTESIAN_POINT('',(163.293320454657,-3.44517452324429,0.00242599488633463));
#23884=CARTESIAN_POINT('',(163.148679545343,-3.4452102901939,0.00241153213425219));
#23885=CARTESIAN_POINT('',(165.,-3.442,-4.21523428266519E-16));
#23886=CARTESIAN_POINT('Ctrl Pts',(163.293320454657,-3.44517452324429,0.00242599488633463));
#23887=CARTESIAN_POINT('Ctrl Pts',(163.286041974537,-3.44643442364397,0.159428330452332));
#23888=CARTESIAN_POINT('Ctrl Pts',(163.278763494417,-3.43661887138664,0.316272314327839));
#23889=CARTESIAN_POINT('Ctrl Pts',(163.271485014297,-3.41518589515111,0.471512356536619));
#23890=CARTESIAN_POINT('Ctrl Pts',(163.21886934233,-3.2602482669296,1.59373279295724));
#23891=CARTESIAN_POINT('Ctrl Pts',(163.166253670364,-2.49821280746788,2.63213520662755));
#23892=CARTESIAN_POINT('Ctrl Pts',(163.113637998398,-1.47412982119765,3.11653010109987));
#23893=CARTESIAN_POINT('Ctrl Pts',(163.061022326432,-0.450046834927408,
3.6009249955722));
#23894=CARTESIAN_POINT('Ctrl Pts',(163.008406654466,0.836083678151346,3.53131237084653));
#23895=CARTESIAN_POINT('Ctrl Pts',(162.9557909825,1.80190072739622,2.93921288262942));
#23896=CARTESIAN_POINT('Ctrl Pts',(162.903175310534,2.76771777664108,2.34711339441232));
#23897=CARTESIAN_POINT('Ctrl Pts',(162.850559638567,3.41322136205207,1.2325270427038));
#23898=CARTESIAN_POINT('Ctrl Pts',(162.797943966601,3.44612691092026,0.100139475917283));
#23899=CARTESIAN_POINT('Ctrl Pts',(162.745328294635,3.47903245978844,-1.03224809086925));
#23900=CARTESIAN_POINT('Ctrl Pts',(162.692712622669,2.8993399721138,-2.18243687273376));
#23901=CARTESIAN_POINT('Ctrl Pts',(162.640096950703,1.96953469955406,-2.82962041059543));
#23902=CARTESIAN_POINT('Ctrl Pts',(162.587481278737,1.03972942699433,-3.47680394845709));
#23903=CARTESIAN_POINT('Ctrl Pts',(162.53486560677,-0.240188630450497,-3.62098224231593));
#23904=CARTESIAN_POINT('Ctrl Pts',(162.482249934804,-1.29067148733502,-3.1968712380367));
#23905=CARTESIAN_POINT('Ctrl Pts',(162.429634262838,-2.34115434421955,-2.77276023375746));
#23906=CARTESIAN_POINT('Ctrl Pts',(162.377018590872,-3.16220200054378,-1.78035993134015));
#23907=CARTESIAN_POINT('Ctrl Pts',(162.324402918906,-3.38204337892538,-0.669030032115677));
#23908=CARTESIAN_POINT('Ctrl Pts',(162.31404209749,-3.42533347056955,-0.450192370441127));
#23909=CARTESIAN_POINT('Ctrl Pts',(162.303681276073,-3.44531144915719,-0.226743146465491));
#23910=CARTESIAN_POINT('Ctrl Pts',(162.293320454657,-3.4432958299264,-0.0029358085113948));
#23911=CARTESIAN_POINT('Ctrl Pts',(162.148679545343,-3.44325559759246,-0.00294208160319024));
#23912=CARTESIAN_POINT('Ctrl Pts',(162.159103538445,-3.44528515787374,-0.22812083159991));
#23913=CARTESIAN_POINT('Ctrl Pts',(162.169527531547,-3.42506065804876,-0.452936839079066));
#23914=CARTESIAN_POINT('Ctrl Pts',(162.179951524649,-3.38124447682805,-0.673056782348974));
#23915=CARTESIAN_POINT('Ctrl Pts',(162.232567196615,-3.1600799196962,-1.78412416460122));
#23916=CARTESIAN_POINT('Ctrl Pts',(162.285182868581,-2.3378511008242,-2.77554613796251));
#23917=CARTESIAN_POINT('Ctrl Pts',(162.337798540547,-1.28686392900068,-3.19840598933041));
#23918=CARTESIAN_POINT('Ctrl Pts',(162.390414212513,-0.235876757177136,
-3.62126584069832));
#23919=CARTESIAN_POINT('Ctrl Pts',(162.443029884479,1.04386876759795,-3.47556357007279));
#23920=CARTESIAN_POINT('Ctrl Pts',(162.495645556446,1.97290278281865,-2.827273289566));
#23921=CARTESIAN_POINT('Ctrl Pts',(162.548261228412,2.90193679803933,-2.17898300905921));
#23922=CARTESIAN_POINT('Ctrl Pts',(162.600876900378,3.48025930370564,-1.02810471867118));
#23923=CARTESIAN_POINT('Ctrl Pts',(162.653492572344,3.44600537717898,0.104242912471304));
#23924=CARTESIAN_POINT('Ctrl Pts',(162.70610824431,3.41175145065233,1.2365905436138));
#23925=CARTESIAN_POINT('Ctrl Pts',(162.758723916276,2.7649210919327,2.35040751551073));
#23926=CARTESIAN_POINT('Ctrl Pts',(162.811339588243,1.79839963781204,2.94135655558191));
#23927=CARTESIAN_POINT('Ctrl Pts',(162.863955260209,0.8318781836914,3.53230559565307));
#23928=CARTESIAN_POINT('Ctrl Pts',(162.916570932175,-0.454334365830267,
3.60038670389851));
#23929=CARTESIAN_POINT('Ctrl Pts',(162.969186604141,-1.47783987393939,3.11477269657705));
#23930=CARTESIAN_POINT('Ctrl Pts',(163.021802276107,-2.50134538204853,2.62915868925557));
#23931=CARTESIAN_POINT('Ctrl Pts',(163.074417948073,-3.26214384874513,1.58984956636719));
#23932=CARTESIAN_POINT('Ctrl Pts',(163.127033620039,-3.41574508097403,0.467445383064969));
#23933=CARTESIAN_POINT('Ctrl Pts',(163.134248928474,-3.43680877217194,0.313527509013778));
#23934=CARTESIAN_POINT('Ctrl Pts',(163.141464236908,-3.44645395580836,0.158047009967286));
#23935=CARTESIAN_POINT('Ctrl Pts',(163.148679545343,-3.4452102901939,0.00241153213425219));
#23936=CARTESIAN_POINT('Origin',(165.,0.,0.));
#23937=CARTESIAN_POINT('',(164.293320454657,-3.43664328220378,0.000481279145628788));
#23938=CARTESIAN_POINT('',(164.148679545343,-3.43664933101759,0.000502961695028516));
#23939=CARTESIAN_POINT('',(165.,-3.442,-4.21523428266519E-16));
#23940=CARTESIAN_POINT('Ctrl Pts',(164.293320454657,-3.43664328220378,0.000481279145628788));
#23941=CARTESIAN_POINT('Ctrl Pts',(164.268402673,-3.43732628447773,0.541385065300302));
#23942=CARTESIAN_POINT('Ctrl Pts',(164.243484891344,-3.31706603853791,1.08200166084634));
#23943=CARTESIAN_POINT('Ctrl Pts',(164.218567109687,-3.07423963801863,1.56040675749654));
#23944=CARTESIAN_POINT('Ctrl Pts',(164.165951437721,-2.5614943860317,2.57059321707906));
#23945=CARTESIAN_POINT('Ctrl Pts',(164.113335765755,-1.50225934571328,3.30339519821379));
#23946=CARTESIAN_POINT('Ctrl Pts',(164.060720093789,-0.37615704458299,3.42699934032914));
#23947=CARTESIAN_POINT('Ctrl Pts',(164.008104421823,0.749945256547313,3.5506034824445));
#23948=CARTESIAN_POINT('Ctrl Pts',(163.955488749856,1.94291481848948,3.06500978554047));
#23949=CARTESIAN_POINT('Ctrl Pts',(163.90287307789,2.66257400854294,2.1900954887487));
#23950=CARTESIAN_POINT('Ctrl Pts',(163.850257405924,3.38223319859638,1.31518119195694));
#23951=CARTESIAN_POINT('Ctrl Pts',(163.797641733958,3.62858201676113,0.0509462952774498));
#23952=CARTESIAN_POINT('Ctrl Pts',(163.745026061992,3.2900735085632,-1.03016256438313));
#23953=CARTESIAN_POINT('Ctrl Pts',(163.692410390026,2.95156500036526,-2.11127142404373));
#23954=CARTESIAN_POINT('Ctrl Pts',(163.63979471806,2.02819916580462,-3.00925424668543));
#23955=CARTESIAN_POINT('Ctrl Pts',(163.587179046093,0.938076840427768,-3.31750364615607));
#23956=CARTESIAN_POINT('Ctrl Pts',(163.534563374127,-0.152045484949063,
-3.62575304562671));
#23957=CARTESIAN_POINT('Ctrl Pts',(163.481947702161,-1.40892430114209,-3.34426902192632));
#23958=CARTESIAN_POINT('Ctrl Pts',(163.429332030195,-2.26344381074798,-2.60050778049066));
#23959=CARTESIAN_POINT('Ctrl Pts',(163.383994838349,-2.99975513198533,-1.95963321155401));
#23960=CARTESIAN_POINT('Ctrl Pts',(163.338657646503,-3.43732668342273,-0.975531613071623));
#23961=CARTESIAN_POINT('Ctrl Pts',(163.293320454657,-3.44517452324429,0.00242599488633463));
#23962=CARTESIAN_POINT('Ctrl Pts',(163.148679545343,-3.4452102901939,0.00241153213425219));
#23963=CARTESIAN_POINT('Ctrl Pts',(163.194079908875,-3.43738486297624,-0.976882331195102));
#23964=CARTESIAN_POINT('Ctrl Pts',(163.239480272406,-2.99844670811644,-1.96231213468243));
#23965=CARTESIAN_POINT('Ctrl Pts',(163.284880635938,-2.26034573001926,-2.60320126481429));
#23966=CARTESIAN_POINT('Ctrl Pts',(163.337496307904,-1.40494114907436,-3.34594448567534));
#23967=CARTESIAN_POINT('Ctrl Pts',(163.39011197987,-0.147727989423363,-3.62593168368139));
#23968=CARTESIAN_POINT('Ctrl Pts',(163.442727651836,0.942026560528155,-3.31638441734467));
#23969=CARTESIAN_POINT('Ctrl Pts',(163.495343323802,2.03178111047965,-3.00683715100795));
#23970=CARTESIAN_POINT('Ctrl Pts',(163.547958995769,2.95407705073166,-2.10775542032849));
#23971=CARTESIAN_POINT('Ctrl Pts',(163.600574667735,3.29129799479096,-1.02624419795294));
#23972=CARTESIAN_POINT('Ctrl Pts',(163.653190339701,3.62851893885027,0.0552670244226335));
#23973=CARTESIAN_POINT('Ctrl Pts',(163.705806011667,3.38066488671686,1.31920773849431));
#23974=CARTESIAN_POINT('Ctrl Pts',(163.758421683633,2.65996436408649,2.19326451349057));
#23975=CARTESIAN_POINT('Ctrl Pts',(163.811037355599,1.93926384145612,3.06732128848682));
#23976=CARTESIAN_POINT('Ctrl Pts',(163.863653027565,0.745716848328806,3.55149412440766));
#23977=CARTESIAN_POINT('Ctrl Pts',(163.916268699532,-0.380237521262959,
3.4265491491836));
#23978=CARTESIAN_POINT('Ctrl Pts',(163.968884371498,-1.50619189085473,3.30160417395954));
#23979=CARTESIAN_POINT('Ctrl Pts',(164.021500043464,-2.56455363691095,2.56754138759055));
#23980=CARTESIAN_POINT('Ctrl Pts',(164.07411571543,-3.07609566029694,1.55674504433108));
#23981=CARTESIAN_POINT('Ctrl Pts',(164.098970325401,-3.31773806454547,1.07926470562088));
#23982=CARTESIAN_POINT('Ctrl Pts',(164.123824935372,-3.43736136450879,0.540033154696634));
#23983=CARTESIAN_POINT('Ctrl Pts',(164.148679545343,-3.43664933101759,0.000502961695028516));
#23984=CARTESIAN_POINT('Origin',(165.,0.,0.));
#23985=CARTESIAN_POINT('',(165.293320454657,-3.44348846335203,-0.00290342158797974));
#23986=CARTESIAN_POINT('',(165.148679545343,-3.44344843612552,-0.00291051544235242));
#23987=CARTESIAN_POINT('',(165.,-3.442,-4.21523428266519E-16));
#23988=CARTESIAN_POINT('Ctrl Pts',(165.293320454657,-3.44348846335203,-0.00290342158797974));
#23989=CARTESIAN_POINT('Ctrl Pts',(165.250763371464,-3.43524791269343,0.916252704056434));
#23990=CARTESIAN_POINT('Ctrl Pts',(165.208206288271,-3.0552517495188,1.84142636681851));
#23991=CARTESIAN_POINT('Ctrl Pts',(165.165649205078,-2.396550793366,2.47837908634305));
#23992=CARTESIAN_POINT('Ctrl Pts',(165.113033533112,-1.58216242761392,3.26587890620758));
#23993=CARTESIAN_POINT('Ctrl Pts',(165.060417861146,-0.341753097329506,
3.61281161947734));
#23994=CARTESIAN_POINT('Ctrl Pts',(165.007802189179,0.7630187973166,3.36208579839172));
#23995=CARTESIAN_POINT('Ctrl Pts',(164.955186517213,1.86779069196271,3.11135997730611));
#23996=CARTESIAN_POINT('Ctrl Pts',(164.902570845247,2.8369251509705,2.26297562186511));
#23997=CARTESIAN_POINT('Ctrl Pts',(164.849955173281,3.23159726670101,1.20108189007092));
#23998=CARTESIAN_POINT('Ctrl Pts',(164.797339501315,3.62626938243153,0.139188158276714));
#23999=CARTESIAN_POINT('Ctrl Pts',(164.744723829349,3.44647915488475,-1.13621494987071));
#24000=CARTESIAN_POINT('Ctrl Pts',(164.692108157383,2.77363575207064,-2.0476238218094));
#24001=CARTESIAN_POINT('Ctrl Pts',(164.639492485417,2.10079234925652,-2.95903269374809));
#24002=CARTESIAN_POINT('Ctrl Pts',(164.58687681345,0.934895771175069,-3.50644732947806));
#24003=CARTESIAN_POINT('Ctrl Pts',(164.534261141484,-0.196135019600669,
-3.44199791616614));
#24004=CARTESIAN_POINT('Ctrl Pts',(164.481645469518,-1.32716581037639,-3.37754850285422));
#24005=CARTESIAN_POINT('Ctrl Pts',(164.429029797552,-2.42333081384639,-2.70123504050043));
#24006=CARTESIAN_POINT('Ctrl Pts',(164.376414125586,-2.98828558375369,-1.71929284030839));
#24007=CARTESIAN_POINT('Ctrl Pts',(164.348716235276,-3.28568851831746,-1.20237979263726));
#24008=CARTESIAN_POINT('Ctrl Pts',(164.321018344967,-3.43588407649575,-0.600771831723536));
#24009=CARTESIAN_POINT('Ctrl Pts',(164.293320454657,-3.43664328220378,0.000481279145628788));
#24010=CARTESIAN_POINT('Ctrl Pts',(164.148679545343,-3.43664933101759,0.000502961695028516));
#24011=CARTESIAN_POINT('Ctrl Pts',(164.176440607338,-3.43585403364963,-0.602118892102288));
#24012=CARTESIAN_POINT('Ctrl Pts',(164.204201669333,-3.28493429195908,-1.20511331706909));
#24013=CARTESIAN_POINT('Ctrl Pts',(164.231962731329,-2.98623633469664,-1.72285002181984));
#24014=CARTESIAN_POINT('Ctrl Pts',(164.284578403295,-2.42011268499457,-2.70411884456138));
#24015=CARTESIAN_POINT('Ctrl Pts',(164.337194075261,-1.32314308487464,-3.3791265898945));
#24016=CARTESIAN_POINT('Ctrl Pts',(164.389809747227,-0.192036302641559,
-3.44222917639352));
#24017=CARTESIAN_POINT('Ctrl Pts',(164.442425419193,0.939070479591511,-3.50533176289254));
#24018=CARTESIAN_POINT('Ctrl Pts',(164.495041091159,2.10431444393775,-2.95652919055749));
#24019=CARTESIAN_POINT('Ctrl Pts',(164.547656763125,2.7760721318787,-2.04431973109724));
#24020=CARTESIAN_POINT('Ctrl Pts',(164.600272435091,3.44782981981966,-1.13211027163698));
#24021=CARTESIAN_POINT('Ctrl Pts',(164.652888107058,3.62610123135531,0.14350607494847));
#24022=CARTESIAN_POINT('Ctrl Pts',(164.705503779024,3.23016491965784,1.20492914155103));
#24023=CARTESIAN_POINT('Ctrl Pts',(164.75811945099,2.83422860796038,2.26635220815355));
#24024=CARTESIAN_POINT('Ctrl Pts',(164.810735122956,1.86408457302983,3.11358199477318));
#24025=CARTESIAN_POINT('Ctrl Pts',(164.863350794922,0.759014859341979,3.36299213315243));
#24026=CARTESIAN_POINT('Ctrl Pts',(164.915966466888,-0.3460548543459,3.61240227153168));
#24027=CARTESIAN_POINT('Ctrl Pts',(164.968582138854,-1.58605024679109,3.26399276167052));
#24028=CARTESIAN_POINT('Ctrl Pts',(165.021197810821,-2.39950034922871,2.47552372608269));
#24029=CARTESIAN_POINT('Ctrl Pts',(165.063691722328,-3.05646576232802,1.83873373229116));
#24030=CARTESIAN_POINT('Ctrl Pts',(165.106185633836,-3.43521118804265,0.914908906409425));
#24031=CARTESIAN_POINT('Ctrl Pts',(165.148679545343,-3.44344843612552,-0.00291051544235242));
#24032=CARTESIAN_POINT('Origin',(165.,0.,0.));
#24033=CARTESIAN_POINT('',(166.293320454657,-3.44500202379557,0.00249305976498276));
#24034=CARTESIAN_POINT('',(166.148679545343,-3.44503851029087,0.00247933530702656));
#24035=CARTESIAN_POINT('',(165.,-3.442,-4.21523428266519E-16));
#24036=CARTESIAN_POINT('Ctrl Pts',(166.293320454657,-3.44500202379557,0.00249305976498276));
#24037=CARTESIAN_POINT('Ctrl Pts',(166.285739741894,-3.44633958802846,0.166036157384798));
#24038=CARTESIAN_POINT('Ctrl Pts',(166.27815902913,-3.43568802025806,0.329404290985655));
#24039=CARTESIAN_POINT('Ctrl Pts',(166.270578316367,-3.41244430662922,0.490960746862352));
#24040=CARTESIAN_POINT('Ctrl Pts',(166.217962644401,-3.25111599229308,1.61228030504036));
#24041=CARTESIAN_POINT('Ctrl Pts',(166.165346972435,-2.48317720304131,2.64632461267713));
#24042=CARTESIAN_POINT('Ctrl Pts',(166.112731300469,-1.45635127605751,3.12487752744511));
#24043=CARTESIAN_POINT('Ctrl Pts',(166.060115628503,-0.429525349073735,
3.60343044221307));
#24044=CARTESIAN_POINT('Ctrl Pts',(166.007499956536,0.856187715642067,3.52649196411227));
#24045=CARTESIAN_POINT('Ctrl Pts',(165.95488428457,1.81861594842145,2.92889990149082));
#24046=CARTESIAN_POINT('Ctrl Pts',(165.902268612604,2.78104418120086,2.33130783886936));
#24047=CARTESIAN_POINT('Ctrl Pts',(165.849652940638,3.42018758204383,1.21306219172721));
#24048=CARTESIAN_POINT('Ctrl Pts',(165.797037268672,3.44664147522546,0.0805055405637458));
#24049=CARTESIAN_POINT('Ctrl Pts',(165.744421596706,3.47309536840708,-1.05205111059968));
#24050=CARTESIAN_POINT('Ctrl Pts',(165.691805924739,2.88685975392742,-2.19891876578441));
#24051=CARTESIAN_POINT('Ctrl Pts',(165.639190252773,1.95338261682879,-2.84079477489608));
#24052=CARTESIAN_POINT('Ctrl Pts',(165.586574580807,1.01990547973014,-3.48267078400776));
#24053=CARTESIAN_POINT('Ctrl Pts',(165.533958908841,-0.260813179987495,
-3.61955514704634));
#24054=CARTESIAN_POINT('Ctrl Pts',(165.481343236875,-1.30886286348838,-3.18946650795815));
#24055=CARTESIAN_POINT('Ctrl Pts',(165.428727564909,-2.35691254698925,-2.75937786886997));
#24056=CARTESIAN_POINT('Ctrl Pts',(165.376111892942,-3.17229325427339,-1.76231622765505));
#24057=CARTESIAN_POINT('Ctrl Pts',(165.323496220976,-3.3857999073056,-0.649751943817944));
#24058=CARTESIAN_POINT('Ctrl Pts',(165.313437632203,-3.42661618015608,-0.437061956279473));
#24059=CARTESIAN_POINT('Ctrl Pts',(165.30337904343,-3.44543616051829,-0.220150770149137));
#24060=CARTESIAN_POINT('Ctrl Pts',(165.293320454657,-3.44348846335203,-0.00290342158797974));
#24061=CARTESIAN_POINT('Ctrl Pts',(165.148679545343,-3.44344843612552,-0.00291051544235242));
#24062=CARTESIAN_POINT('Ctrl Pts',(165.158801305802,-3.44541049254668,-0.221528853993161));
#24063=CARTESIAN_POINT('Ctrl Pts',(165.16892306626,-3.42635139806872,-0.43980646995822));
#24064=CARTESIAN_POINT('Ctrl Pts',(165.179044826719,-3.38502395824774,-0.653783179988487));
#24065=CARTESIAN_POINT('Ctrl Pts',(165.231660498685,-3.1701926523991,-1.76609248915746));
#24066=CARTESIAN_POINT('Ctrl Pts',(165.284276170651,-2.35362522827174,-2.7621825461809));
#24067=CARTESIAN_POINT('Ctrl Pts',(165.336891842617,-1.30506411029719,-3.19102292570286));
#24068=CARTESIAN_POINT('Ctrl Pts',(165.389507514584,-0.256502992322657,
-3.61986330522481));
#24069=CARTESIAN_POINT('Ctrl Pts',(165.44212318655,1.02405181949904,-3.48145400724529));
#24070=CARTESIAN_POINT('Ctrl Pts',(165.494738858516,1.95676401679889,-2.83846687965671));
#24071=CARTESIAN_POINT('Ctrl Pts',(165.547354530482,2.88947621409875,-2.19547975206813));
#24072=CARTESIAN_POINT('Ctrl Pts',(165.599970202448,3.47434579687675,-1.04791479487049));
#24073=CARTESIAN_POINT('Ctrl Pts',(165.652585874414,3.44654332040737,0.0846096028970402));
#24074=CARTESIAN_POINT('Ctrl Pts',(165.70520154638,3.41874084393799,1.21713400066456));
#24075=CARTESIAN_POINT('Ctrl Pts',(165.757817218347,2.77826630822123,2.334617839002));
#24076=CARTESIAN_POINT('Ctrl Pts',(165.810432890313,1.81512712798546,2.93106348508494));
#24077=CARTESIAN_POINT('Ctrl Pts',(165.863048562279,0.851987947749686,3.5275091311679));
#24078=CARTESIAN_POINT('Ctrl Pts',(165.915664234245,-0.433815877005108,
3.60291658499637));
#24079=CARTESIAN_POINT('Ctrl Pts',(165.968279906211,-1.46007128038759,3.12314128731545));
#24080=CARTESIAN_POINT('Ctrl Pts',(166.020895578177,-2.48632668377006,2.64336598963453));
#24081=CARTESIAN_POINT('Ctrl Pts',(166.073511250144,-3.25303366578022,1.60840794044424));
#24082=CARTESIAN_POINT('Ctrl Pts',(166.12612692211,-3.41302665260159,0.486897025025004));
#24083=CARTESIAN_POINT('Ctrl Pts',(166.133644463187,-3.43588588456886,0.326659512876953));
#24084=CARTESIAN_POINT('Ctrl Pts',(166.141162004265,-3.44635984905697,0.164655137910781));
#24085=CARTESIAN_POINT('Ctrl Pts',(166.148679545343,-3.44503851029087,0.00247933530702656));
#24086=CARTESIAN_POINT('Origin',(165.,0.,0.));
#24087=CARTESIAN_POINT('',(167.293320454657,-3.4366186727045,0.000377228489918668));
#24088=CARTESIAN_POINT('',(167.148679545343,-3.43662347336092,0.000399016594708752));
#24089=CARTESIAN_POINT('',(165.,-3.442,-4.21523428266519E-16));
#24090=CARTESIAN_POINT('Ctrl Pts',(167.293320454657,-3.4366186727045,0.000377228489918668));
#24091=CARTESIAN_POINT('Ctrl Pts',(167.268100440357,-3.43716028314427,0.547851542709962));
#24092=CARTESIAN_POINT('Ctrl Pts',(167.242880426057,-3.31382643177038,1.09509536773555));
#24093=CARTESIAN_POINT('Ctrl Pts',(167.217660411758,-3.0653002376201,1.5778951340479));
#24094=CARTESIAN_POINT('Ctrl Pts',(167.165044739791,-2.54680835450729,2.58514413191544));
#24095=CARTESIAN_POINT('Ctrl Pts',(167.112429067825,-1.48341578853514,3.31189984384937));
#24096=CARTESIAN_POINT('Ctrl Pts',(167.059813395859,-0.356627598376805,
3.42908666511678));
#24097=CARTESIAN_POINT('Ctrl Pts',(167.007197723893,0.770160591781512,3.5462734863842));
#24098=CARTESIAN_POINT('Ctrl Pts',(166.954582051927,1.960344406126,3.05389141698511));
#24099=CARTESIAN_POINT('Ctrl Pts',(166.901966379961,2.67500760083863,2.17489147689288));
#24100=CARTESIAN_POINT('Ctrl Pts',(166.849350707995,3.38967079555127,1.29589153680066));
#24101=CARTESIAN_POINT('Ctrl Pts',(166.796735036029,3.62881337063205,0.0302737260152738));
#24102=CARTESIAN_POINT('Ctrl Pts',(166.744119364062,3.28415136460691,-1.04888913387277));
#24103=CARTESIAN_POINT('Ctrl Pts',(166.691503692096,2.93948935858177,-2.12805199376081));
#24104=CARTESIAN_POINT('Ctrl Pts',(166.63888802013,2.01102277145072,-3.02075990275153));
#24105=CARTESIAN_POINT('Ctrl Pts',(166.586272348164,0.919162063864181,-3.32279396008219));
#24106=CARTESIAN_POINT('Ctrl Pts',(166.533656676198,-0.172698643722376,
-3.62482801741286));
#24107=CARTESIAN_POINT('Ctrl Pts',(166.481041004232,-1.42795347176443,-3.33618822308345));
#24108=CARTESIAN_POINT('Ctrl Pts',(166.428425332266,-2.27822196607518,-2.58757092155912));
#24109=CARTESIAN_POINT('Ctrl Pts',(166.383390373063,-3.00598625230122,-1.94681222034209));
#24110=CARTESIAN_POINT('Ctrl Pts',(166.33835541386,-3.43705591733564,-0.969072142503072));
#24111=CARTESIAN_POINT('Ctrl Pts',(166.293320454657,-3.44500202379557,0.00249305976498276));
#24112=CARTESIAN_POINT('Ctrl Pts',(166.148679545343,-3.44503851029087,0.00247933530702656));
#24113=CARTESIAN_POINT('Ctrl Pts',(166.193777676231,-3.43711172838111,-0.970421976048281));
#24114=CARTESIAN_POINT('Ctrl Pts',(166.23887580712,-3.00468799405711,-1.94949273537325));
#24115=CARTESIAN_POINT('Ctrl Pts',(166.283973938008,-2.27513928018629,-2.59028201169302));
#24116=CARTESIAN_POINT('Ctrl Pts',(166.336589609974,-1.42397992931704,-3.33788635134359));
#24117=CARTESIAN_POINT('Ctrl Pts',(166.38920528194,-0.168382235945959,-3.62503124899654));
#24118=CARTESIAN_POINT('Ctrl Pts',(166.441820953907,0.923118096027443,-3.32169725067378));
#24119=CARTESIAN_POINT('Ctrl Pts',(166.494436625873,2.01461842800086,-3.01836325235101));
#24120=CARTESIAN_POINT('Ctrl Pts',(166.547052297839,2.94202139857659,-2.12455035805251));
#24121=CARTESIAN_POINT('Ctrl Pts',(166.599667969805,3.28539815358547,-1.04497780682858));
#24122=CARTESIAN_POINT('Ctrl Pts',(166.652283641771,3.62877490859433,0.0345947443953297));
#24123=CARTESIAN_POINT('Ctrl Pts',(166.704899313737,3.38812544803635,1.29992695254466));
#24124=CARTESIAN_POINT('Ctrl Pts',(166.757514985703,2.6724160524118,2.17807531714557));
#24125=CARTESIAN_POINT('Ctrl Pts',(166.81013065767,1.95670665678724,3.0562236817465));
#24126=CARTESIAN_POINT('Ctrl Pts',(166.862746329636,0.765937326096089,3.547188202799));
#24127=CARTESIAN_POINT('Ctrl Pts',(166.915362001602,-0.360710573543627,
3.42865972742716));
#24128=CARTESIAN_POINT('Ctrl Pts',(166.967977673568,-1.48735847318333,3.31013125205532));
#24129=CARTESIAN_POINT('Ctrl Pts',(167.020593345534,-2.5498849417716,2.58210978025916));
#24130=CARTESIAN_POINT('Ctrl Pts',(167.0732090175,-3.06717709026766,1.57424405391421));
#24131=CARTESIAN_POINT('Ctrl Pts',(167.098365860115,-3.31450714762519,1.09235874281813));
#24132=CARTESIAN_POINT('Ctrl Pts',(167.123522702729,-3.43719497569704,0.54650018122335));
#24133=CARTESIAN_POINT('Ctrl Pts',(167.148679545343,-3.43662347336092,0.000399016594708752));
#24134=CARTESIAN_POINT('Origin',(165.,0.,0.));
#24135=CARTESIAN_POINT('',(168.293320454657,-3.44367996564435,-0.0028671194461008));
#24136=CARTESIAN_POINT('',(168.148679545343,-3.44364019544098,-0.00287502992418087));
#24137=CARTESIAN_POINT('',(165.,-3.442,-4.21523428266519E-16));
#24138=CARTESIAN_POINT('Ctrl Pts',(168.293320454657,-3.44367996564435,-0.0028671194461008));
#24139=CARTESIAN_POINT('Ctrl Pts',(168.250461138821,-3.43543047620403,0.9226836846828));
#24140=CARTESIAN_POINT('Ctrl Pts',(168.207601822984,-3.04941537922053,1.85430521201957));
#24141=CARTESIAN_POINT('Ctrl Pts',(168.164742507148,-2.38239277503066,2.49199182709186));
#24142=CARTESIAN_POINT('Ctrl Pts',(168.112126835182,-1.56353130112863,3.2748393621314));
#24143=CARTESIAN_POINT('Ctrl Pts',(168.059511163216,-0.321165651672412,
3.61469993243571));
#24144=CARTESIAN_POINT('Ctrl Pts',(168.00689549125,0.782159950179274,3.35768438259772));
#24145=CARTESIAN_POINT('Ctrl Pts',(167.954279819284,1.88548555203095,3.10066883275973));
#24146=CARTESIAN_POINT('Ctrl Pts',(167.901664147318,2.84977110627809,2.24677716277947));
#24147=CARTESIAN_POINT('Ctrl Pts',(167.849048475351,3.23838729348434,1.18265224736778));
#24148=CARTESIAN_POINT('Ctrl Pts',(167.796432803385,3.6270034806906,0.118527331956078));
#24149=CARTESIAN_POINT('Ctrl Pts',(167.743817131419,3.43995030085597,-1.15583082888706));
#24150=CARTESIAN_POINT('Ctrl Pts',(167.691201459453,2.76192559296549,-2.06339177562785));
#24151=CARTESIAN_POINT('Ctrl Pts',(167.638585787487,2.08390088507502,-2.97095272236863));
#24152=CARTESIAN_POINT('Ctrl Pts',(167.585970115521,0.914904649128732,-3.51171645500707));
#24153=CARTESIAN_POINT('Ctrl Pts',(167.533354443555,-0.215740624581454,
-3.44082469528903));
#24154=CARTESIAN_POINT('Ctrl Pts',(167.480738771588,-1.34638589829166,-3.36993293557099));
#24155=CARTESIAN_POINT('Ctrl Pts',(167.428123099622,-2.43868020976575,-2.68738568349645));
#24156=CARTESIAN_POINT('Ctrl Pts',(167.375507427656,-2.99803176537606,-1.7022409155586));
#24157=CARTESIAN_POINT('Ctrl Pts',(167.34811176999,-3.28927205862042,-1.18930080084075));
#24158=CARTESIAN_POINT('Ctrl Pts',(167.320716112323,-3.43603033940618,-0.594325800432333));
#24159=CARTESIAN_POINT('Ctrl Pts',(167.293320454657,-3.4366186727045,0.000377228489918668));
#24160=CARTESIAN_POINT('Ctrl Pts',(167.148679545343,-3.43662347336092,0.000399016594708752));
#24161=CARTESIAN_POINT('Ctrl Pts',(167.176138374695,-3.43599967547967,-0.595673349018475));
#24162=CARTESIAN_POINT('Ctrl Pts',(167.203597204047,-3.28852668101727,-1.19203474800941));
#24163=CARTESIAN_POINT('Ctrl Pts',(167.231056033399,-2.9960028145529,-1.70580971375418));
#24164=CARTESIAN_POINT('Ctrl Pts',(167.283671705365,-2.43547856193824,-2.69028777418379));
#24165=CARTESIAN_POINT('Ctrl Pts',(167.336287377331,-1.34237222830503,-3.3715339141493));
#24166=CARTESIAN_POINT('Ctrl Pts',(167.388903049297,-0.211643291605701,
-3.44107930182745));
#24167=CARTESIAN_POINT('Ctrl Pts',(167.441518721263,0.919085645093658,-3.51062468950561));
#24168=CARTESIAN_POINT('Ctrl Pts',(167.49413439323,2.08743718485917,-2.96846932489641));
#24169=CARTESIAN_POINT('Ctrl Pts',(167.546750065196,2.76438075637838,-2.06010161839459));
#24170=CARTESIAN_POINT('Ctrl Pts',(167.599365737162,3.44132432789757,-1.15173391189279));
#24171=CARTESIAN_POINT('Ctrl Pts',(167.651981409128,3.62685993117048,0.122846136501633));
#24172=CARTESIAN_POINT('Ctrl Pts',(167.704597081094,3.23697688716988,1.18650759638316));
#24173=CARTESIAN_POINT('Ctrl Pts',(167.75721275306,2.84709384316927,2.25016905626472));
#24174=CARTESIAN_POINT('Ctrl Pts',(167.809828425026,1.88179215189513,3.10291192763337));
#24175=CARTESIAN_POINT('Ctrl Pts',(167.862444096993,0.778161240495354,3.35861351276649));
#24176=CARTESIAN_POINT('Ctrl Pts',(167.915059768959,-0.325469670904378,
3.61431509789959));
#24177=CARTESIAN_POINT('Ctrl Pts',(167.967675440925,-1.56742980242973,3.27297539679721));
#24178=CARTESIAN_POINT('Ctrl Pts',(168.020291112891,-2.38535854978838,2.48915331655147));
#24179=CARTESIAN_POINT('Ctrl Pts',(168.063087257042,-3.05063935432642,1.85161393938135));
#24180=CARTESIAN_POINT('Ctrl Pts',(168.105883401192,-3.43539162467462,0.921339312272485));
#24181=CARTESIAN_POINT('Ctrl Pts',(168.148679545343,-3.44364019544098,-0.00287502992418087));
#24182=CARTESIAN_POINT('Origin',(165.,0.,0.));
#24183=CARTESIAN_POINT('',(169.293320454657,-3.44482624767651,0.00255655274150716));
#24184=CARTESIAN_POINT('',(169.148679545343,-3.4448633964524,0.00254358015426723));
#24185=CARTESIAN_POINT('',(165.,-3.442,-4.21523428266519E-16));
#24186=CARTESIAN_POINT('Ctrl Pts',(169.293320454657,-3.44482624767651,0.00255655274150716));
#24187=CARTESIAN_POINT('Ctrl Pts',(169.28543750925,-3.44624129304017,0.172642513390955));
#24188=CARTESIAN_POINT('Ctrl Pts',(169.277554563844,-3.43471905135417,0.342536135345187));
#24189=CARTESIAN_POINT('Ctrl Pts',(169.269671618437,-3.40959196657226,0.510393202924915));
#24190=CARTESIAN_POINT('Ctrl Pts',(169.217055946471,-3.24187820196086,1.63077549019679));
#24191=CARTESIAN_POINT('Ctrl Pts',(169.164440274505,-2.46806100668965,2.66042813182627));
#24192=CARTESIAN_POINT('Ctrl Pts',(169.111824602539,-1.43852546484462,3.13312353540276));
#24193=CARTESIAN_POINT('Ctrl Pts',(169.059208930573,-0.408989922999565,
3.60581893897926));
#24194=CARTESIAN_POINT('Ctrl Pts',(169.006593258607,0.876263965419336,3.52155710450275));
#24195=CARTESIAN_POINT('Ctrl Pts',(168.953977586641,1.83527214599084,2.9184918624124));
#24196=CARTESIAN_POINT('Ctrl Pts',(168.901361914674,2.7942803265623,2.31542662032207));
#24197=CARTESIAN_POINT('Ctrl Pts',(168.848746242708,3.4270427992864,1.19355797061799));
#24198=CARTESIAN_POINT('Ctrl Pts',(168.796130570742,3.44704417820427,0.0608689923961288));
#24199=CARTESIAN_POINT('Ctrl Pts',(168.743514898776,3.46704555712214,-1.07181998582578));
#24200=CARTESIAN_POINT('Ctrl Pts',(168.69089922681,2.87428584223369,-2.21532929256545));
#24201=CARTESIAN_POINT('Ctrl Pts',(168.638283554844,1.93716713675568,-2.85187694073908));
#24202=CARTESIAN_POINT('Ctrl Pts',(168.585667882878,1.0000484312777,-3.4884245889127));
#24203=CARTESIAN_POINT('Ctrl Pts',(168.533052210911,-0.281429264789832,
-3.61801057852031));
#24204=CARTESIAN_POINT('Ctrl Pts',(168.480436538945,-1.32701176028542,-3.181958263219));
#24205=CARTESIAN_POINT('Ctrl Pts',(168.427820866979,-2.37259425578103,-2.74590594791768));
#24206=CARTESIAN_POINT('Ctrl Pts',(168.375205195013,-3.1822815507047,-1.74421532770741));
#24207=CARTESIAN_POINT('Ctrl Pts',(168.322589523047,-3.38944654899261,-0.6304527677149));
#24208=CARTESIAN_POINT('Ctrl Pts',(168.312833166917,-3.42786049345878,-0.42393133078477));
#24209=CARTESIAN_POINT('Ctrl Pts',(168.303076810787,-3.44555785275709,-0.213556512994896));
#24210=CARTESIAN_POINT('Ctrl Pts',(168.293320454657,-3.44367996564435,-0.0028671194461008));
#24211=CARTESIAN_POINT('Ctrl Pts',(168.148679545343,-3.44364019544098,-0.00287502992418087));
#24212=CARTESIAN_POINT('Ctrl Pts',(168.158499073159,-3.44553282085585,-0.214934985809443));
#24213=CARTESIAN_POINT('Ctrl Pts',(168.168318600974,-3.4276037337122,-0.426675887125822));
#24214=CARTESIAN_POINT('Ctrl Pts',(168.178138128789,-3.3886935781589,-0.634488358987591));
#24215=CARTESIAN_POINT('Ctrl Pts',(168.230753800756,-3.18020249597882,-1.74800349489171));
#24216=CARTESIAN_POINT('Ctrl Pts',(168.283369472722,-2.36932296842675,-2.7487293073108));
#24217=CARTESIAN_POINT('Ctrl Pts',(168.335985144688,-1.32322193552417,-3.18353629690223));
#24218=CARTESIAN_POINT('Ctrl Pts',(168.388600816654,-0.2771209026216,-3.61834328649367));
#24219=CARTESIAN_POINT('Ctrl Pts',(168.44121648862,1.00420163563145,-3.48723145325744));
#24220=CARTESIAN_POINT('Ctrl Pts',(168.493832160586,1.94056174368239,-2.84956834683932));
#24221=CARTESIAN_POINT('Ctrl Pts',(168.546447832553,2.87692185173333,-2.21190524042119));
#24222=CARTESIAN_POINT('Ctrl Pts',(168.599063504519,3.46831952958212,-1.06769086082117));
#24223=CARTESIAN_POINT('Ctrl Pts',(168.651679176485,3.44696940550524,0.0649735473051323));
#24224=CARTESIAN_POINT('Ctrl Pts',(168.704294848451,3.42561928142836,1.19763795543145));
#24225=CARTESIAN_POINT('Ctrl Pts',(168.756910520417,2.79152135542575,2.31875239208407));
#24226=CARTESIAN_POINT('Ctrl Pts',(168.809526192383,1.83179570791246,2.92067528643946));
#24227=CARTESIAN_POINT('Ctrl Pts',(168.862141864349,0.872070060399187,3.52259818079485));
#24228=CARTESIAN_POINT('Ctrl Pts',(168.914757536316,-0.413283308624756,
3.60532953285307));
#24229=CARTESIAN_POINT('Ctrl Pts',(168.967373208282,-1.44225529998775,3.13140851599467));
#24230=CARTESIAN_POINT('Ctrl Pts',(169.019988880248,-2.47122729135076,2.65748749913626));
#24231=CARTESIAN_POINT('Ctrl Pts',(169.072604552214,-3.2438179050528,1.62691411336122));
#24232=CARTESIAN_POINT('Ctrl Pts',(169.12522022418,-3.41019745387857,0.50633286465407));
#24233=CARTESIAN_POINT('Ctrl Pts',(169.133039997901,-3.43492488536428,0.339791386166305));
#24234=CARTESIAN_POINT('Ctrl Pts',(169.140859771622,-3.44626227331867,0.171261806054121));
#24235=CARTESIAN_POINT('Ctrl Pts',(169.148679545343,-3.4448633964524,0.00254358015426723));
#24236=CARTESIAN_POINT('Origin',(165.,0.,0.));
#24237=CARTESIAN_POINT('',(170.293320454657,-3.43660005727478,0.000272750764409579));
#24238=CARTESIAN_POINT('',(170.148679545343,-3.43660359651311,0.000294614659134998));
#24239=CARTESIAN_POINT('',(165.,-3.442,-4.21523428266519E-16));
#24240=CARTESIAN_POINT('Ctrl Pts',(170.293320454657,-3.43660005727478,0.000272750764409579));
#24241=CARTESIAN_POINT('Ctrl Pts',(170.267798207714,-3.43699621854537,0.554315412873624));
#24242=CARTESIAN_POINT('Ctrl Pts',(170.242275960771,-3.31054519341703,1.10818746561827));
#24243=CARTESIAN_POINT('Ctrl Pts',(170.216753713828,-3.05626134594043,1.59533229623574));
#24244=CARTESIAN_POINT('Ctrl Pts',(170.164138041862,-2.53203965280226,2.59961113834073));
#24245=CARTESIAN_POINT('Ctrl Pts',(170.111522369896,-1.46452408676501,3.32029700118331));
#24246=CARTESIAN_POINT('Ctrl Pts',(170.05890669793,-0.337086580959713,3.43106270007475));
#24247=CARTESIAN_POINT('Ctrl Pts',(170.006291025963,0.790350924845598,3.54182839896619));
#24248=CARTESIAN_POINT('Ctrl Pts',(169.953675353997,1.97771037041895,3.04267393390648));
#24249=CARTESIAN_POINT('Ctrl Pts',(169.901059682031,2.68735437690533,2.15961687771555));
#24250=CARTESIAN_POINT('Ctrl Pts',(169.848444010065,3.39699838339171,1.27655982152463));
#24251=CARTESIAN_POINT('Ctrl Pts',(169.795828338099,3.62892695079112,0.00960017420250078));
#24252=CARTESIAN_POINT('Ctrl Pts',(169.743212666133,3.27812263219616,-1.06758166106696));
#24253=CARTESIAN_POINT('Ctrl Pts',(169.690596994167,2.9273183136012,-2.14476349633643));
#24254=CARTESIAN_POINT('Ctrl Pts',(169.6379813222,1.99378110901184,-3.03216751955324));
#24255=CARTESIAN_POINT('Ctrl Pts',(169.585365650234,0.900217456132267,-3.32797643239589));
#24256=CARTESIAN_POINT('Ctrl Pts',(169.532749978268,-0.19334619674729,-3.62378534523853));
#24257=CARTESIAN_POINT('Ctrl Pts',(169.480134306302,-1.44693629791706,-3.32799914770704));
#24258=CARTESIAN_POINT('Ctrl Pts',(169.427518634336,-2.29292618152615,-2.57455008248416));
#24259=CARTESIAN_POINT('Ctrl Pts',(169.382785907776,-3.01216880870502,-1.93398369319767));
#24260=CARTESIAN_POINT('Ctrl Pts',(169.338053181217,-3.43679640171692,-0.962616790092074));
#24261=CARTESIAN_POINT('Ctrl Pts',(169.293320454657,-3.44482624767651,0.00255655274150716));
#24262=CARTESIAN_POINT('Ctrl Pts',(169.148679545343,-3.4448633964524,0.00254358015426723));
#24263=CARTESIAN_POINT('Ctrl Pts',(169.193475443588,-3.43684987227702,-0.963965777940212));
#24264=CARTESIAN_POINT('Ctrl Pts',(169.238271341833,-3.01088069160431,-1.93666577160495));
#24265=CARTESIAN_POINT('Ctrl Pts',(169.283067240079,-2.28985899035532,-2.57727869052755));
#24266=CARTESIAN_POINT('Ctrl Pts',(169.335682912045,-1.44297249405678,-3.32971988536281));
#24267=CARTESIAN_POINT('Ctrl Pts',(169.388298584011,-0.189031017510179,
-3.62401316339407));
#24268=CARTESIAN_POINT('Ctrl Pts',(169.440914255977,0.904179671619464,-3.32690227780616));
#24269=CARTESIAN_POINT('Ctrl Pts',(169.493529927943,1.99739036074909,-3.02979139221826));
#24270=CARTESIAN_POINT('Ctrl Pts',(169.546145599909,2.92987026246178,-2.1412763430112));
#24271=CARTESIAN_POINT('Ctrl Pts',(169.598761271875,3.2793916841586,-1.0636775007116));
#24272=CARTESIAN_POINT('Ctrl Pts',(169.651376943842,3.62891310585543,0.0139213415880397));
#24273=CARTESIAN_POINT('Ctrl Pts',(169.703992615808,3.39547604753637,1.28060397698021));
#24274=CARTESIAN_POINT('Ctrl Pts',(169.756608287774,2.68478100720705,2.16281543087444));
#24275=CARTESIAN_POINT('Ctrl Pts',(169.80922395974,1.97408596687775,3.04502688476864));
#24276=CARTESIAN_POINT('Ctrl Pts',(169.861839631706,0.786132944538199,3.5427671571649));
#24277=CARTESIAN_POINT('Ctrl Pts',(169.914455303672,-0.341171919250267,
3.43065902822761));
#24278=CARTESIAN_POINT('Ctrl Pts',(169.967070975638,-1.46847678303873,3.31855089929033));
#24279=CARTESIAN_POINT('Ctrl Pts',(170.019686647605,-2.53513348827613,2.59659436901949));
#24280=CARTESIAN_POINT('Ctrl Pts',(170.072302319571,-3.05815897380138,1.59169197060008));
#24281=CARTESIAN_POINT('Ctrl Pts',(170.097761394828,-3.31123462027619,1.10545118279472));
#24282=CARTESIAN_POINT('Ctrl Pts',(170.123220470086,-3.43703049239502,0.552964592785464));
#24283=CARTESIAN_POINT('Ctrl Pts',(170.148679545343,-3.43660359651311,0.000294614659134998));
#24284=CARTESIAN_POINT('Origin',(165.,0.,0.));
#24285=CARTESIAN_POINT('',(171.293320454657,-3.44387122878711,-0.00282630271176032));
#24286=CARTESIAN_POINT('',(171.148679545343,-3.44383074993744,-0.0028355498312654));
#24287=CARTESIAN_POINT('',(165.,-3.442,-4.21523428266519E-16));
#24288=CARTESIAN_POINT('Ctrl Pts',(171.293320454657,-3.44387122878711,-0.00282630271176032));
#24289=CARTESIAN_POINT('Ctrl Pts',(171.250158906178,-3.43562450198846,0.929118171345689));
#24290=CARTESIAN_POINT('Ctrl Pts',(171.206997357698,-3.04353120649987,1.86717743073024));
#24291=CARTESIAN_POINT('Ctrl Pts',(171.163835809219,-2.36815699607087,2.50552345035264));
#24292=CARTESIAN_POINT('Ctrl Pts',(171.111220137253,-1.5448485383751,3.28369304696447));
#24293=CARTESIAN_POINT('Ctrl Pts',(171.058604465286,-0.300567776468357,
3.61647092641191));
#24294=CARTESIAN_POINT('Ctrl Pts',(171.00598879332,0.801275500324471,3.35317411112243));
#24295=CARTESIAN_POINT('Ctrl Pts',(170.953373121354,1.90311877711725,3.08987729583295));
#24296=CARTESIAN_POINT('Ctrl Pts',(170.900757449388,2.86252456879606,2.23050578580653));
#24297=CARTESIAN_POINT('Ctrl Pts',(170.848141777422,3.24507232555683,1.1641841628401));
#24298=CARTESIAN_POINT('Ctrl Pts',(170.795526105456,3.62762008231762,0.0978625398736385));
#24299=CARTESIAN_POINT('Ctrl Pts',(170.74291043349,3.43330980416037,-1.17540919603287));
#24300=CARTESIAN_POINT('Ctrl Pts',(170.690294761523,2.7501257418227,-2.07909273270173));
#24301=CARTESIAN_POINT('Ctrl Pts',(170.637679089557,2.06694167948504,-2.98277626937059));
#24302=CARTESIAN_POINT('Ctrl Pts',(170.585063417591,0.894883832966949,-3.5168716068018));
#24303=CARTESIAN_POINT('Ctrl Pts',(170.532447745625,-0.235339201293036,
-3.4395398162459));
#24304=CARTESIAN_POINT('Ctrl Pts',(170.479832073659,-1.365562235553,-3.36220802569001));
#24305=CARTESIAN_POINT('Ctrl Pts',(170.427216401693,-2.45395045755487,-2.67344910714704));
#24306=CARTESIAN_POINT('Ctrl Pts',(170.374600729727,-3.00768065843627,-1.68513373719186));
#24307=CARTESIAN_POINT('Ctrl Pts',(170.347507304703,-3.29281334077317,-1.17621980766165));
#24308=CARTESIAN_POINT('Ctrl Pts',(170.32041387968,-3.43617950787308,-0.587877397577702));
#24309=CARTESIAN_POINT('Ctrl Pts',(170.293320454657,-3.43660005727478,0.000272750764409579));
#24310=CARTESIAN_POINT('Ctrl Pts',(170.148679545343,-3.43660359651311,0.000294614659134998));
#24311=CARTESIAN_POINT('Ctrl Pts',(170.175836142052,-3.43614823671766,-0.589225450670685));
#24312=CARTESIAN_POINT('Ctrl Pts',(170.20299273876,-3.29207677469171,-1.178954174763));
#24313=CARTESIAN_POINT('Ctrl Pts',(170.230149335469,-3.00567206006267,-1.68871404224666));
#24314=CARTESIAN_POINT('Ctrl Pts',(170.282765007435,-2.45076539498559,-2.67636939010597));
#24315=CARTESIAN_POINT('Ctrl Pts',(170.335380679402,-1.36155779901833,-3.36383181925656));
#24316=CARTESIAN_POINT('Ctrl Pts',(170.387996351368,-0.231243408789148,
-3.43981774870589));
#24317=CARTESIAN_POINT('Ctrl Pts',(170.440612023334,0.899070981439999,-3.51580367815521));
#24318=CARTESIAN_POINT('Ctrl Pts',(170.4932276953,2.07049216593107,-2.98031310790332));
#24319=CARTESIAN_POINT('Ctrl Pts',(170.545843367266,2.7525996566615,-2.07581664023284));
#24320=CARTESIAN_POINT('Ctrl Pts',(170.598459039232,3.43470714739194,-1.17132017256236));
#24321=CARTESIAN_POINT('Ctrl Pts',(170.651074711198,3.62750094436174,0.102182192526675));
#24322=CARTESIAN_POINT('Ctrl Pts',(170.703690383164,3.2436838097568,1.16804753377652));
#24323=CARTESIAN_POINT('Ctrl Pts',(170.756306055131,2.85986667515186,2.23391287502634));
#24324=CARTESIAN_POINT('Ctrl Pts',(170.808921727097,1.89943860897218,3.09214119243696));
#24325=CARTESIAN_POINT('Ctrl Pts',(170.861537399063,0.797282342672176,3.35412590649805));
#24326=CARTESIAN_POINT('Ctrl Pts',(170.914153071029,-0.304873923627829,
3.61611062055913));
#24327=CARTESIAN_POINT('Ctrl Pts',(170.966768742995,-1.54875839004818,3.28185173127071));
#24328=CARTESIAN_POINT('Ctrl Pts',(171.019384414962,-2.37113928540063,2.50270208381497));
#24329=CARTESIAN_POINT('Ctrl Pts',(171.062482791755,-3.04476522937394,1.86448757794553));
#24330=CARTESIAN_POINT('Ctrl Pts',(171.105581168549,-3.43558242261714,0.927772636575842));
#24331=CARTESIAN_POINT('Ctrl Pts',(171.148679545343,-3.44383074993744,-0.0028355498312654));
#24332=CARTESIAN_POINT('Origin',(165.,0.,0.));
#24333=CARTESIAN_POINT('',(172.293320454657,-3.44466766225695,0.00262740410212479));
#24334=CARTESIAN_POINT('',(172.148679545343,-3.44468745739532,0.00260595186748766));
#24335=CARTESIAN_POINT('',(165.,-3.442,-4.21523428266519E-16));
#24336=CARTESIAN_POINT('Ctrl Pts',(172.293320454657,-3.44466766225695,0.00262740410212479));
#24337=CARTESIAN_POINT('Ctrl Pts',(172.285135276607,-3.44617626541761,0.179267317335753));
#24338=CARTESIAN_POINT('Ctrl Pts',(172.276950098558,-3.43376273876756,0.355695505307162));
#24339=CARTESIAN_POINT('Ctrl Pts',(172.268764920508,-3.40668944351872,0.52984202940742));
#24340=CARTESIAN_POINT('Ctrl Pts',(172.216149248542,-3.2326578447912,1.64928455472401));
#24341=CARTESIAN_POINT('Ctrl Pts',(172.163533576576,-2.4528655438326,2.67444576178309));
#24342=CARTESIAN_POINT('Ctrl Pts',(172.110917904609,-1.4206230354588,3.14125155492291));
#24343=CARTESIAN_POINT('Ctrl Pts',(172.058302232643,-0.388380527085031,
3.60805734806272));
#24344=CARTESIAN_POINT('Ctrl Pts',(172.005686560677,0.89631218870392,3.51650772728329));
#24345=CARTESIAN_POINT('Ctrl Pts',(171.953070888711,1.85185396723248,2.90799717118038));
#24346=CARTESIAN_POINT('Ctrl Pts',(171.900455216745,2.80739574576104,2.29948661507748));
#24347=CARTESIAN_POINT('Ctrl Pts',(171.847839544779,3.43378658702921,1.17401512365106));
#24348=CARTESIAN_POINT('Ctrl Pts',(171.795223872812,3.44734233714038,0.0412264759991943));
#24349=CARTESIAN_POINT('Ctrl Pts',(171.742608200846,3.46089808725154,-1.09156217165267));
#24350=CARTESIAN_POINT('Ctrl Pts',(171.68999252888,2.86161874620574,-2.23166797553003));
#24351=CARTESIAN_POINT('Ctrl Pts',(171.637376856914,1.92088515794683,-2.86286457252168));
#24352=CARTESIAN_POINT('Ctrl Pts',(171.584761184948,0.980151569687923,-3.49406116951333));
#24353=CARTESIAN_POINT('Ctrl Pts',(171.532145512982,-0.302036265784079,
-3.61634855961926));
#24354=CARTESIAN_POINT('Ctrl Pts',(171.479529841016,-1.34511579343341,-3.1743477253533));
#24355=CARTESIAN_POINT('Ctrl Pts',(171.426914169049,-2.38819532108274,-2.73234689108733));
#24356=CARTESIAN_POINT('Ctrl Pts',(171.374298497083,-3.19216654090938,-1.72605783244947));
#24357=CARTESIAN_POINT('Ctrl Pts',(171.321682825117,-3.39298407408037,-0.611132646242449));
#24358=CARTESIAN_POINT('Ctrl Pts',(171.31222870163,-3.42906750105106,-0.41079993176759));
#24359=CARTESIAN_POINT('Ctrl Pts',(171.302774578144,-3.44567759524667,-0.206959806975336));
#24360=CARTESIAN_POINT('Ctrl Pts',(171.293320454657,-3.44387122878711,-0.00282630271176032));
#24361=CARTESIAN_POINT('Ctrl Pts',(171.148679545343,-3.44383074993744,-0.0028355498312654));
#24362=CARTESIAN_POINT('Ctrl Pts',(171.158196840515,-3.44565220521313,-0.208339178010312));
#24363=CARTESIAN_POINT('Ctrl Pts',(171.167714135688,-3.4288178176788,-0.413545012325797));
#24364=CARTESIAN_POINT('Ctrl Pts',(171.17723143086,-3.3922533139467,-0.615172870133585));
#24365=CARTESIAN_POINT('Ctrl Pts',(171.229847102826,-3.19010912285572,-1.72985777100326));
#24366=CARTESIAN_POINT('Ctrl Pts',(171.282462774792,-2.38494341638922,-2.73518716711955));
#24367=CARTESIAN_POINT('Ctrl Pts',(171.335078446758,-1.34133662038965,-3.17594649833862));
#24368=CARTESIAN_POINT('Ctrl Pts',(171.387694118724,-0.297729824390071,
-3.61670582955769));
#24369=CARTESIAN_POINT('Ctrl Pts',(171.440309790691,0.984318061142581,-3.49289509587954));
#24370=CARTESIAN_POINT('Ctrl Pts',(171.492925462657,1.92429609530075,-2.86057702277709));
#24371=CARTESIAN_POINT('Ctrl Pts',(171.545541134623,2.86427412945893,-2.22825894967464));
#24372=CARTESIAN_POINT('Ctrl Pts',(171.598156806589,3.46218231224263,-1.08743353714789));
#24373=CARTESIAN_POINT('Ctrl Pts',(171.650772478555,3.44728441488538,0.0453347604952326));
#24374=CARTESIAN_POINT('Ctrl Pts',(171.703388150521,3.43238651752813,1.17810305813836));
#24375=CARTESIAN_POINT('Ctrl Pts',(171.756003822488,2.80468254002992,2.30281424089786));
#24376=CARTESIAN_POINT('Ctrl Pts',(171.808619494454,1.84840322753821,2.91019355475018));
#24377=CARTESIAN_POINT('Ctrl Pts',(171.86123516642,0.892123915046473,3.51757286860253));
#24378=CARTESIAN_POINT('Ctrl Pts',(171.913850838386,-0.392730732438793,
3.60762031354766));
#24379=CARTESIAN_POINT('Ctrl Pts',(171.966466510352,-1.42438925928684,3.13957157218144));
#24380=CARTESIAN_POINT('Ctrl Pts',(172.019082182318,-2.45604778613486,2.67152283081523));
#24381=CARTESIAN_POINT('Ctrl Pts',(172.071697854284,-3.23451019234567,1.6453779031377));
#24382=CARTESIAN_POINT('Ctrl Pts',(172.124313526251,-3.40726414772573,0.525757408362557));
#24383=CARTESIAN_POINT('Ctrl Pts',(172.132435532615,-3.4339312731772,0.352927442608599));
#24384=CARTESIAN_POINT('Ctrl Pts',(172.140557538979,-3.44616528464549,0.177870095822215));
#24385=CARTESIAN_POINT('Ctrl Pts',(172.148679545343,-3.44468745739532,0.00260595186748766));
#24386=CARTESIAN_POINT('Ctrl Pts',(37.5,32.4,0.));
#24387=CARTESIAN_POINT('Ctrl Pts',(37.5,32.4,32.4));
#24388=CARTESIAN_POINT('Ctrl Pts',(37.5,0.,32.4));
#24389=CARTESIAN_POINT('Ctrl Pts',(37.5,-32.4,32.4));
#24390=CARTESIAN_POINT('Ctrl Pts',(37.5,-32.4,0.));
#24391=CARTESIAN_POINT('Ctrl Pts',(37.5,-32.4,-32.4));
#24392=CARTESIAN_POINT('Ctrl Pts',(37.5,0.,-32.4));
#24393=CARTESIAN_POINT('Ctrl Pts',(37.5,32.4,-32.4));
#24394=CARTESIAN_POINT('Ctrl Pts',(37.5,32.4,0.));
#24395=CARTESIAN_POINT('Ctrl Pts',(37.3389083940589,32.2580145365138,0.));
#24396=CARTESIAN_POINT('Ctrl Pts',(37.3389083940589,32.2580145365137,32.2580145365137));
#24397=CARTESIAN_POINT('Ctrl Pts',(37.3389083940589,0.,32.2580145365138));
#24398=CARTESIAN_POINT('Ctrl Pts',(37.3389083940589,-32.2580145365137,32.2580145365137));
#24399=CARTESIAN_POINT('Ctrl Pts',(37.3389083940589,-32.2580145365138,0.));
#24400=CARTESIAN_POINT('Ctrl Pts',(37.3389083940589,-32.2580145365137,-32.2580145365137));
#24401=CARTESIAN_POINT('Ctrl Pts',(37.3389083940589,0.,-32.2580145365138));
#24402=CARTESIAN_POINT('Ctrl Pts',(37.3389083940589,32.2580145365137,-32.2580145365137));
#24403=CARTESIAN_POINT('Ctrl Pts',(37.3389083940589,32.2580145365138,0.));
#24404=CARTESIAN_POINT('Ctrl Pts',(37.0144855040189,31.9658168899962,0.));
#24405=CARTESIAN_POINT('Ctrl Pts',(37.0144855040189,31.9658168899962,31.9658168899962));
#24406=CARTESIAN_POINT('Ctrl Pts',(37.0144855040189,0.,31.9658168899962));
#24407=CARTESIAN_POINT('Ctrl Pts',(37.0144855040189,-31.9658168899962,31.9658168899962));
#24408=CARTESIAN_POINT('Ctrl Pts',(37.0144855040189,-31.9658168899962,0.));
#24409=CARTESIAN_POINT('Ctrl Pts',(37.0144855040189,-31.9658168899962,-31.9658168899962));
#24410=CARTESIAN_POINT('Ctrl Pts',(37.0144855040189,0.,-31.9658168899962));
#24411=CARTESIAN_POINT('Ctrl Pts',(37.0144855040189,31.9658168899962,-31.9658168899962));
#24412=CARTESIAN_POINT('Ctrl Pts',(37.0144855040189,31.9658168899962,0.));
#24413=CARTESIAN_POINT('Ctrl Pts',(36.5211322358012,31.5028400616267,0.));
#24414=CARTESIAN_POINT('Ctrl Pts',(36.5211322358012,31.5028400616266,31.5028400616266));
#24415=CARTESIAN_POINT('Ctrl Pts',(36.5211322358012,0.,31.5028400616267));
#24416=CARTESIAN_POINT('Ctrl Pts',(36.5211322358012,-31.5028400616266,31.5028400616266));
#24417=CARTESIAN_POINT('Ctrl Pts',(36.5211322358012,-31.5028400616267,0.));
#24418=CARTESIAN_POINT('Ctrl Pts',(36.5211322358012,-31.5028400616266,-31.5028400616266));
#24419=CARTESIAN_POINT('Ctrl Pts',(36.5211322358012,0.,-31.5028400616267));
#24420=CARTESIAN_POINT('Ctrl Pts',(36.5211322358012,31.5028400616266,-31.5028400616266));
#24421=CARTESIAN_POINT('Ctrl Pts',(36.5211322358012,31.5028400616267,0.));
#24422=CARTESIAN_POINT('Ctrl Pts',(35.849854090057,30.8360498427659,0.));
#24423=CARTESIAN_POINT('Ctrl Pts',(35.849854090057,30.8360498427659,30.8360498427659));
#24424=CARTESIAN_POINT('Ctrl Pts',(35.849854090057,0.,30.8360498427659));
#24425=CARTESIAN_POINT('Ctrl Pts',(35.849854090057,-30.8360498427659,30.8360498427659));
#24426=CARTESIAN_POINT('Ctrl Pts',(35.849854090057,-30.8360498427659,0.));
#24427=CARTESIAN_POINT('Ctrl Pts',(35.849854090057,-30.8360498427659,-30.8360498427659));
#24428=CARTESIAN_POINT('Ctrl Pts',(35.849854090057,0.,-30.8360498427659));
#24429=CARTESIAN_POINT('Ctrl Pts',(35.849854090057,30.8360498427659,-30.8360498427659));
#24430=CARTESIAN_POINT('Ctrl Pts',(35.849854090057,30.8360498427659,0.));
#24431=CARTESIAN_POINT('Ctrl Pts',(34.987601126175,29.9204750609072,0.));
#24432=CARTESIAN_POINT('Ctrl Pts',(34.987601126175,29.9204750609072,29.9204750609072));
#24433=CARTESIAN_POINT('Ctrl Pts',(34.987601126175,0.,29.9204750609072));
#24434=CARTESIAN_POINT('Ctrl Pts',(34.987601126175,-29.9204750609072,29.9204750609072));
#24435=CARTESIAN_POINT('Ctrl Pts',(34.987601126175,-29.9204750609072,0.));
#24436=CARTESIAN_POINT('Ctrl Pts',(34.987601126175,-29.9204750609072,-29.9204750609072));
#24437=CARTESIAN_POINT('Ctrl Pts',(34.987601126175,0.,-29.9204750609072));
#24438=CARTESIAN_POINT('Ctrl Pts',(34.987601126175,29.9204750609072,-29.9204750609072));
#24439=CARTESIAN_POINT('Ctrl Pts',(34.987601126175,29.9204750609072,0.));
#24440=CARTESIAN_POINT('Ctrl Pts',(34.1004337719427,28.9253475198501,0.));
#24441=CARTESIAN_POINT('Ctrl Pts',(34.1004337719427,28.9253475198501,28.9253475198501));
#24442=CARTESIAN_POINT('Ctrl Pts',(34.1004337719427,0.,28.9253475198501));
#24443=CARTESIAN_POINT('Ctrl Pts',(34.1004337719427,-28.9253475198501,28.9253475198501));
#24444=CARTESIAN_POINT('Ctrl Pts',(34.1004337719427,-28.9253475198501,0.));
#24445=CARTESIAN_POINT('Ctrl Pts',(34.1004337719427,-28.9253475198501,-28.9253475198501));
#24446=CARTESIAN_POINT('Ctrl Pts',(34.1004337719427,0.,-28.9253475198501));
#24447=CARTESIAN_POINT('Ctrl Pts',(34.1004337719427,28.9253475198501,-28.9253475198501));
#24448=CARTESIAN_POINT('Ctrl Pts',(34.1004337719427,28.9253475198501,0.));
#24449=CARTESIAN_POINT('Ctrl Pts',(33.1851263782876,27.8567138854442,0.));
#24450=CARTESIAN_POINT('Ctrl Pts',(33.1851263782876,27.8567138854442,27.8567138854442));
#24451=CARTESIAN_POINT('Ctrl Pts',(33.1851263782876,0.,27.8567138854442));
#24452=CARTESIAN_POINT('Ctrl Pts',(33.1851263782876,-27.8567138854442,27.8567138854442));
#24453=CARTESIAN_POINT('Ctrl Pts',(33.1851263782876,-27.8567138854442,0.));
#24454=CARTESIAN_POINT('Ctrl Pts',(33.1851263782876,-27.8567138854442,-27.8567138854442));
#24455=CARTESIAN_POINT('Ctrl Pts',(33.1851263782876,0.,-27.8567138854442));
#24456=CARTESIAN_POINT('Ctrl Pts',(33.1851263782876,27.8567138854442,-27.8567138854442));
#24457=CARTESIAN_POINT('Ctrl Pts',(33.1851263782876,27.8567138854442,0.));
#24458=CARTESIAN_POINT('Ctrl Pts',(32.2364640041498,26.7258152226803,0.));
#24459=CARTESIAN_POINT('Ctrl Pts',(32.2364640041498,26.7258152226803,26.7258152226803));
#24460=CARTESIAN_POINT('Ctrl Pts',(32.2364640041498,0.,26.7258152226803));
#24461=CARTESIAN_POINT('Ctrl Pts',(32.2364640041498,-26.7258152226803,26.7258152226803));
#24462=CARTESIAN_POINT('Ctrl Pts',(32.2364640041498,-26.7258152226803,0.));
#24463=CARTESIAN_POINT('Ctrl Pts',(32.2364640041498,-26.7258152226803,-26.7258152226803));
#24464=CARTESIAN_POINT('Ctrl Pts',(32.2364640041498,0.,-26.7258152226803));
#24465=CARTESIAN_POINT('Ctrl Pts',(32.2364640041498,26.7258152226803,-26.7258152226803));
#24466=CARTESIAN_POINT('Ctrl Pts',(32.2364640041498,26.7258152226803,0.));
#24467=CARTESIAN_POINT('Ctrl Pts',(31.2480536381088,25.5477500100038,0.));
#24468=CARTESIAN_POINT('Ctrl Pts',(31.2480536381088,25.5477500100038,25.5477500100038));
#24469=CARTESIAN_POINT('Ctrl Pts',(31.2480536381088,0.,25.5477500100038));
#24470=CARTESIAN_POINT('Ctrl Pts',(31.2480536381087,-25.5477500100038,25.5477500100038));
#24471=CARTESIAN_POINT('Ctrl Pts',(31.2480536381087,-25.5477500100038,0.));
#24472=CARTESIAN_POINT('Ctrl Pts',(31.2480536381087,-25.5477500100038,-25.5477500100038));
#24473=CARTESIAN_POINT('Ctrl Pts',(31.2480536381088,0.,-25.5477500100038));
#24474=CARTESIAN_POINT('Ctrl Pts',(31.2480536381088,25.5477500100038,-25.5477500100038));
#24475=CARTESIAN_POINT('Ctrl Pts',(31.2480536381088,25.5477500100038,0.));
#24476=CARTESIAN_POINT('Ctrl Pts',(30.2132710279087,24.339870673897,0.));
#24477=CARTESIAN_POINT('Ctrl Pts',(30.2132710279087,24.339870673897,24.339870673897));
#24478=CARTESIAN_POINT('Ctrl Pts',(30.2132710279087,0.,24.339870673897));
#24479=CARTESIAN_POINT('Ctrl Pts',(30.2132710279087,-24.339870673897,24.339870673897));
#24480=CARTESIAN_POINT('Ctrl Pts',(30.2132710279087,-24.339870673897,0.));
#24481=CARTESIAN_POINT('Ctrl Pts',(30.2132710279087,-24.339870673897,-24.339870673897));
#24482=CARTESIAN_POINT('Ctrl Pts',(30.2132710279087,0.,-24.339870673897));
#24483=CARTESIAN_POINT('Ctrl Pts',(30.2132710279087,24.339870673897,-24.339870673897));
#24484=CARTESIAN_POINT('Ctrl Pts',(30.2132710279087,24.339870673897,0.));
#24485=CARTESIAN_POINT('Ctrl Pts',(29.1261855002599,23.1203063432132,0.));
#24486=CARTESIAN_POINT('Ctrl Pts',(29.1261855002599,23.1203063432132,23.1203063432132));
#24487=CARTESIAN_POINT('Ctrl Pts',(29.1261855002599,0.,23.1203063432132));
#24488=CARTESIAN_POINT('Ctrl Pts',(29.1261855002599,-23.1203063432132,23.1203063432132));
#24489=CARTESIAN_POINT('Ctrl Pts',(29.1261855002599,-23.1203063432132,0.));
#24490=CARTESIAN_POINT('Ctrl Pts',(29.1261855002599,-23.1203063432132,-23.1203063432132));
#24491=CARTESIAN_POINT('Ctrl Pts',(29.1261855002599,0.,-23.1203063432132));
#24492=CARTESIAN_POINT('Ctrl Pts',(29.1261855002599,23.1203063432132,-23.1203063432132));
#24493=CARTESIAN_POINT('Ctrl Pts',(29.1261855002599,23.1203063432132,0.));
#24494=CARTESIAN_POINT('Ctrl Pts',(27.9824847998069,21.9065059385018,0.));
#24495=CARTESIAN_POINT('Ctrl Pts',(27.9824847998069,21.9065059385018,21.9065059385018));
#24496=CARTESIAN_POINT('Ctrl Pts',(27.9824847998069,0.,21.9065059385018));
#24497=CARTESIAN_POINT('Ctrl Pts',(27.9824847998069,-21.9065059385018,21.9065059385018));
#24498=CARTESIAN_POINT('Ctrl Pts',(27.9824847998069,-21.9065059385018,0.));
#24499=CARTESIAN_POINT('Ctrl Pts',(27.9824847998069,-21.9065059385018,-21.9065059385018));
#24500=CARTESIAN_POINT('Ctrl Pts',(27.9824847998069,0.,-21.9065059385018));
#24501=CARTESIAN_POINT('Ctrl Pts',(27.9824847998069,21.9065059385018,-21.9065059385018));
#24502=CARTESIAN_POINT('Ctrl Pts',(27.9824847998069,21.9065059385018,0.));
#24503=CARTESIAN_POINT('Ctrl Pts',(26.780529153894,20.7136594976185,0.));
#24504=CARTESIAN_POINT('Ctrl Pts',(26.780529153894,20.7136594976185,20.7136594976185));
#24505=CARTESIAN_POINT('Ctrl Pts',(26.780529153894,0.,20.7136594976185));
#24506=CARTESIAN_POINT('Ctrl Pts',(26.780529153894,-20.7136594976185,20.7136594976185));
#24507=CARTESIAN_POINT('Ctrl Pts',(26.780529153894,-20.7136594976185,0.));
#24508=CARTESIAN_POINT('Ctrl Pts',(26.780529153894,-20.7136594976185,-20.7136594976185));
#24509=CARTESIAN_POINT('Ctrl Pts',(26.780529153894,0.,-20.7136594976185));
#24510=CARTESIAN_POINT('Ctrl Pts',(26.780529153894,20.7136594976185,-20.7136594976185));
#24511=CARTESIAN_POINT('Ctrl Pts',(26.780529153894,20.7136594976185,0.));
#24512=CARTESIAN_POINT('Ctrl Pts',(25.5210824112439,19.5548484421686,0.));
#24513=CARTESIAN_POINT('Ctrl Pts',(25.5210824112439,19.5548484421686,19.5548484421686));
#24514=CARTESIAN_POINT('Ctrl Pts',(25.5210824112439,0.,19.5548484421686));
#24515=CARTESIAN_POINT('Ctrl Pts',(25.5210824112439,-19.5548484421686,19.5548484421686));
#24516=CARTESIAN_POINT('Ctrl Pts',(25.5210824112439,-19.5548484421686,0.));
#24517=CARTESIAN_POINT('Ctrl Pts',(25.5210824112439,-19.5548484421686,-19.5548484421686));
#24518=CARTESIAN_POINT('Ctrl Pts',(25.5210824112439,0.,-19.5548484421686));
#24519=CARTESIAN_POINT('Ctrl Pts',(25.5210824112439,19.5548484421686,-19.5548484421686));
#24520=CARTESIAN_POINT('Ctrl Pts',(25.5210824112439,19.5548484421686,0.));
#24521=CARTESIAN_POINT('Ctrl Pts',(24.2069345847179,18.4413554671298,0.));
#24522=CARTESIAN_POINT('Ctrl Pts',(24.2069345847179,18.4413554671298,18.4413554671298));
#24523=CARTESIAN_POINT('Ctrl Pts',(24.2069345847179,0.,18.4413554671298));
#24524=CARTESIAN_POINT('Ctrl Pts',(24.2069345847179,-18.4413554671298,18.4413554671298));
#24525=CARTESIAN_POINT('Ctrl Pts',(24.2069345847179,-18.4413554671298,0.));
#24526=CARTESIAN_POINT('Ctrl Pts',(24.2069345847179,-18.4413554671298,-18.4413554671298));
#24527=CARTESIAN_POINT('Ctrl Pts',(24.2069345847179,0.,-18.4413554671298));
#24528=CARTESIAN_POINT('Ctrl Pts',(24.2069345847179,18.4413554671298,-18.4413554671298));
#24529=CARTESIAN_POINT('Ctrl Pts',(24.2069345847179,18.4413554671298,0.));
#24530=CARTESIAN_POINT('Ctrl Pts',(22.8426190791586,17.3828861014748,0.));
#24531=CARTESIAN_POINT('Ctrl Pts',(22.8426190791586,17.3828861014748,17.3828861014748));
#24532=CARTESIAN_POINT('Ctrl Pts',(22.8426190791586,0.,17.3828861014748));
#24533=CARTESIAN_POINT('Ctrl Pts',(22.8426190791586,-17.3828861014748,17.3828861014748));
#24534=CARTESIAN_POINT('Ctrl Pts',(22.8426190791586,-17.3828861014748,0.));
#24535=CARTESIAN_POINT('Ctrl Pts',(22.8426190791586,-17.3828861014748,-17.3828861014748));
#24536=CARTESIAN_POINT('Ctrl Pts',(22.8426190791586,0.,-17.3828861014748));
#24537=CARTESIAN_POINT('Ctrl Pts',(22.8426190791586,17.3828861014748,-17.3828861014748));
#24538=CARTESIAN_POINT('Ctrl Pts',(22.8426190791586,17.3828861014748,0.));
#24539=CARTESIAN_POINT('Ctrl Pts',(21.4341168715413,16.3877853586665,0.));
#24540=CARTESIAN_POINT('Ctrl Pts',(21.4341168715413,16.3877853586665,16.3877853586665));
#24541=CARTESIAN_POINT('Ctrl Pts',(21.4341168715413,0.,16.3877853586665));
#24542=CARTESIAN_POINT('Ctrl Pts',(21.4341168715413,-16.3877853586665,16.3877853586665));
#24543=CARTESIAN_POINT('Ctrl Pts',(21.4341168715413,-16.3877853586665,0.));
#24544=CARTESIAN_POINT('Ctrl Pts',(21.4341168715413,-16.3877853586665,-16.3877853586665));
#24545=CARTESIAN_POINT('Ctrl Pts',(21.4341168715413,0.,-16.3877853586665));
#24546=CARTESIAN_POINT('Ctrl Pts',(21.4341168715413,16.3877853586665,-16.3877853586665));
#24547=CARTESIAN_POINT('Ctrl Pts',(21.4341168715413,16.3877853586665,0.));
#24548=CARTESIAN_POINT('Ctrl Pts',(19.9886520715334,15.4632288398589,0.));
#24549=CARTESIAN_POINT('Ctrl Pts',(19.9886520715334,15.4632288398589,15.4632288398589));
#24550=CARTESIAN_POINT('Ctrl Pts',(19.9886520715334,0.,15.4632288398589));
#24551=CARTESIAN_POINT('Ctrl Pts',(19.9886520715334,-15.4632288398589,15.4632288398589));
#24552=CARTESIAN_POINT('Ctrl Pts',(19.9886520715334,-15.4632288398589,0.));
#24553=CARTESIAN_POINT('Ctrl Pts',(19.9886520715334,-15.4632288398589,-15.4632288398589));
#24554=CARTESIAN_POINT('Ctrl Pts',(19.9886520715334,0.,-15.4632288398589));
#24555=CARTESIAN_POINT('Ctrl Pts',(19.9886520715334,15.4632288398589,-15.4632288398589));
#24556=CARTESIAN_POINT('Ctrl Pts',(19.9886520715334,15.4632288398589,0.));
#24557=CARTESIAN_POINT('Ctrl Pts',(18.514323186272,14.6153405598521,0.));
#24558=CARTESIAN_POINT('Ctrl Pts',(18.514323186272,14.6153405598521,14.6153405598521));
#24559=CARTESIAN_POINT('Ctrl Pts',(18.514323186272,0.,14.6153405598521));
#24560=CARTESIAN_POINT('Ctrl Pts',(18.514323186272,-14.6153405598521,14.6153405598521));
#24561=CARTESIAN_POINT('Ctrl Pts',(18.514323186272,-14.6153405598521,0.));
#24562=CARTESIAN_POINT('Ctrl Pts',(18.514323186272,-14.6153405598521,-14.6153405598521));
#24563=CARTESIAN_POINT('Ctrl Pts',(18.514323186272,0.,-14.6153405598521));
#24564=CARTESIAN_POINT('Ctrl Pts',(18.514323186272,14.6153405598521,-14.6153405598521));
#24565=CARTESIAN_POINT('Ctrl Pts',(18.514323186272,14.6153405598521,0.));
#24566=CARTESIAN_POINT('Ctrl Pts',(17.0194794456568,13.8492044429491,0.));
#24567=CARTESIAN_POINT('Ctrl Pts',(17.0194794456568,13.8492044429491,13.8492044429491));
#24568=CARTESIAN_POINT('Ctrl Pts',(17.0194794456568,0.,13.8492044429491));
#24569=CARTESIAN_POINT('Ctrl Pts',(17.0194794456568,-13.8492044429491,13.8492044429491));
#24570=CARTESIAN_POINT('Ctrl Pts',(17.0194794456568,-13.8492044429491,0.));
#24571=CARTESIAN_POINT('Ctrl Pts',(17.0194794456568,-13.8492044429491,-13.8492044429491));
#24572=CARTESIAN_POINT('Ctrl Pts',(17.0194794456568,0.,-13.8492044429491));
#24573=CARTESIAN_POINT('Ctrl Pts',(17.0194794456568,13.8492044429491,-13.8492044429491));
#24574=CARTESIAN_POINT('Ctrl Pts',(17.0194794456568,13.8492044429491,0.));
#24575=CARTESIAN_POINT('Ctrl Pts',(15.5121733229441,13.1688616684146,0.));
#24576=CARTESIAN_POINT('Ctrl Pts',(15.5121733229441,13.1688616684146,13.1688616684146));
#24577=CARTESIAN_POINT('Ctrl Pts',(15.5121733229441,0.,13.1688616684146));
#24578=CARTESIAN_POINT('Ctrl Pts',(15.5121733229441,-13.1688616684146,13.1688616684146));
#24579=CARTESIAN_POINT('Ctrl Pts',(15.5121733229441,-13.1688616684146,0.));
#24580=CARTESIAN_POINT('Ctrl Pts',(15.5121733229441,-13.1688616684146,-13.1688616684146));
#24581=CARTESIAN_POINT('Ctrl Pts',(15.5121733229441,0.,-13.1688616684146));
#24582=CARTESIAN_POINT('Ctrl Pts',(15.5121733229441,13.1688616684146,-13.1688616684146));
#24583=CARTESIAN_POINT('Ctrl Pts',(15.5121733229441,13.1688616684146,0.));
#24584=CARTESIAN_POINT('Ctrl Pts',(13.9995910956154,12.5772662595197,0.));
#24585=CARTESIAN_POINT('Ctrl Pts',(13.9995910956154,12.5772662595197,12.5772662595197));
#24586=CARTESIAN_POINT('Ctrl Pts',(13.9995910956154,0.,12.5772662595197));
#24587=CARTESIAN_POINT('Ctrl Pts',(13.9995910956154,-12.5772662595197,12.5772662595197));
#24588=CARTESIAN_POINT('Ctrl Pts',(13.9995910956154,-12.5772662595197,0.));
#24589=CARTESIAN_POINT('Ctrl Pts',(13.9995910956154,-12.5772662595197,-12.5772662595197));
#24590=CARTESIAN_POINT('Ctrl Pts',(13.9995910956154,0.,-12.5772662595197));
#24591=CARTESIAN_POINT('Ctrl Pts',(13.9995910956154,12.5772662595197,-12.5772662595197));
#24592=CARTESIAN_POINT('Ctrl Pts',(13.9995910956154,12.5772662595197,0.));
#24593=CARTESIAN_POINT('Ctrl Pts',(12.4874918670977,12.076207951456,0.));
#24594=CARTESIAN_POINT('Ctrl Pts',(12.4874918670977,12.076207951456,12.076207951456));
#24595=CARTESIAN_POINT('Ctrl Pts',(12.4874918670977,0.,12.076207951456));
#24596=CARTESIAN_POINT('Ctrl Pts',(12.4874918670977,-12.076207951456,12.076207951456));
#24597=CARTESIAN_POINT('Ctrl Pts',(12.4874918670977,-12.076207951456,0.));
#24598=CARTESIAN_POINT('Ctrl Pts',(12.4874918670977,-12.076207951456,-12.076207951456));
#24599=CARTESIAN_POINT('Ctrl Pts',(12.4874918670977,0.,-12.076207951456));
#24600=CARTESIAN_POINT('Ctrl Pts',(12.4874918670977,12.076207951456,-12.076207951456));
#24601=CARTESIAN_POINT('Ctrl Pts',(12.4874918670977,12.076207951456,0.));
#24602=CARTESIAN_POINT('Ctrl Pts',(10.979632440052,11.6661962584503,0.));
#24603=CARTESIAN_POINT('Ctrl Pts',(10.979632440052,11.6661962584503,11.6661962584503));
#24604=CARTESIAN_POINT('Ctrl Pts',(10.979632440052,0.,11.6661962584503));
#24605=CARTESIAN_POINT('Ctrl Pts',(10.979632440052,-11.6661962584503,11.6661962584503));
#24606=CARTESIAN_POINT('Ctrl Pts',(10.979632440052,-11.6661962584503,0.));
#24607=CARTESIAN_POINT('Ctrl Pts',(10.979632440052,-11.6661962584503,-11.6661962584503));
#24608=CARTESIAN_POINT('Ctrl Pts',(10.979632440052,0.,-11.6661962584503));
#24609=CARTESIAN_POINT('Ctrl Pts',(10.979632440052,11.6661962584503,-11.6661962584503));
#24610=CARTESIAN_POINT('Ctrl Pts',(10.979632440052,11.6661962584503,0.));
#24611=CARTESIAN_POINT('Ctrl Pts',(9.4782023240472,11.3469207764071,0.));
#24612=CARTESIAN_POINT('Ctrl Pts',(9.4782023240472,11.3469207764071,11.3469207764071));
#24613=CARTESIAN_POINT('Ctrl Pts',(9.4782023240472,0.,11.3469207764071));
#24614=CARTESIAN_POINT('Ctrl Pts',(9.47820232404719,-11.3469207764071,11.3469207764071));
#24615=CARTESIAN_POINT('Ctrl Pts',(9.47820232404719,-11.3469207764071,0.));
#24616=CARTESIAN_POINT('Ctrl Pts',(9.47820232404719,-11.3469207764071,-11.3469207764071));
#24617=CARTESIAN_POINT('Ctrl Pts',(9.4782023240472,0.,-11.3469207764071));
#24618=CARTESIAN_POINT('Ctrl Pts',(9.4782023240472,11.3469207764071,-11.3469207764071));
#24619=CARTESIAN_POINT('Ctrl Pts',(9.4782023240472,11.3469207764071,0.));
#24620=CARTESIAN_POINT('Ctrl Pts',(8.28303567503975,11.1635245405655,0.));
#24621=CARTESIAN_POINT('Ctrl Pts',(8.28303567503975,11.1635245405655,11.1635245405655));
#24622=CARTESIAN_POINT('Ctrl Pts',(8.28303567503976,0.,11.1635245405655));
#24623=CARTESIAN_POINT('Ctrl Pts',(8.28303567503978,-11.1635245405655,11.1635245405655));
#24624=CARTESIAN_POINT('Ctrl Pts',(8.28303567503978,-11.1635245405655,0.));
#24625=CARTESIAN_POINT('Ctrl Pts',(8.28303567503978,-11.1635245405655,-11.1635245405655));
#24626=CARTESIAN_POINT('Ctrl Pts',(8.28303567503976,0.,-11.1635245405655));
#24627=CARTESIAN_POINT('Ctrl Pts',(8.28303567503975,11.1635245405655,-11.1635245405655));
#24628=CARTESIAN_POINT('Ctrl Pts',(8.28303567503975,11.1635245405655,0.));
#24629=CARTESIAN_POINT('Ctrl Pts',(7.39016039139644,11.0661718180104,0.));
#24630=CARTESIAN_POINT('Ctrl Pts',(7.39016039139644,11.0661718180104,11.0661718180104));
#24631=CARTESIAN_POINT('Ctrl Pts',(7.39016039139642,0.,11.0661718180104));
#24632=CARTESIAN_POINT('Ctrl Pts',(7.3901603913964,-11.0661718180104,11.0661718180104));
#24633=CARTESIAN_POINT('Ctrl Pts',(7.3901603913964,-11.0661718180104,0.));
#24634=CARTESIAN_POINT('Ctrl Pts',(7.3901603913964,-11.0661718180104,-11.0661718180104));
#24635=CARTESIAN_POINT('Ctrl Pts',(7.39016039139642,0.,-11.0661718180104));
#24636=CARTESIAN_POINT('Ctrl Pts',(7.39016039139644,11.0661718180104,-11.0661718180104));
#24637=CARTESIAN_POINT('Ctrl Pts',(7.39016039139644,11.0661718180104,0.));
#24638=CARTESIAN_POINT('Ctrl Pts',(6.79646156908522,11.0190876606754,0.));
#24639=CARTESIAN_POINT('Ctrl Pts',(6.79646156908522,11.0190876606754,11.0190876606754));
#24640=CARTESIAN_POINT('Ctrl Pts',(6.79646156908522,0.,11.0190876606754));
#24641=CARTESIAN_POINT('Ctrl Pts',(6.79646156908521,-11.0190876606754,11.0190876606754));
#24642=CARTESIAN_POINT('Ctrl Pts',(6.79646156908521,-11.0190876606754,0.));
#24643=CARTESIAN_POINT('Ctrl Pts',(6.79646156908521,-11.0190876606754,-11.0190876606754));
#24644=CARTESIAN_POINT('Ctrl Pts',(6.79646156908522,0.,-11.0190876606754));
#24645=CARTESIAN_POINT('Ctrl Pts',(6.79646156908522,11.0190876606754,-11.0190876606754));
#24646=CARTESIAN_POINT('Ctrl Pts',(6.79646156908522,11.0190876606754,0.));
#24647=CARTESIAN_POINT('Ctrl Pts',(6.5,11.,0.));
#24648=CARTESIAN_POINT('Ctrl Pts',(6.5,11.,11.));
#24649=CARTESIAN_POINT('Ctrl Pts',(6.49999999999999,0.,11.));
#24650=CARTESIAN_POINT('Ctrl Pts',(6.49999999999997,-11.,11.));
#24651=CARTESIAN_POINT('Ctrl Pts',(6.49999999999997,-11.,0.));
#24652=CARTESIAN_POINT('Ctrl Pts',(6.49999999999997,-11.,-11.));
#24653=CARTESIAN_POINT('Ctrl Pts',(6.49999999999999,0.,-11.));
#24654=CARTESIAN_POINT('Ctrl Pts',(6.5,11.,-11.));
#24655=CARTESIAN_POINT('Ctrl Pts',(6.5,11.,0.));
#24656=CARTESIAN_POINT('',(12.7552064848291,12.1808231353727,0.));
#24657=CARTESIAN_POINT('',(20.644698628669,15.8947820241755,0.));
#24658=CARTESIAN_POINT('Ctrl Pts',(12.7552064848291,12.1808231353727,0.));
#24659=CARTESIAN_POINT('Ctrl Pts',(13.0039389302743,12.2584833095898,0.));
#24660=CARTESIAN_POINT('Ctrl Pts',(13.5550060380175,12.4372815016706,0.));
#24661=CARTESIAN_POINT('Ctrl Pts',(14.4089440713075,12.7375124365726,0.));
#24662=CARTESIAN_POINT('Ctrl Pts',(15.5654093565171,13.1928904640524,0.));
#24663=CARTESIAN_POINT('Ctrl Pts',(17.0194794456568,13.8492044429491,0.));
#24664=CARTESIAN_POINT('Ctrl Pts',(18.3518881687479,14.532089494745,0.));
#24665=CARTESIAN_POINT('Ctrl Pts',(19.3730718999235,15.110588732192,0.));
#24666=CARTESIAN_POINT('Ctrl Pts',(20.0905786930687,15.5451447711833,0.));
#24667=CARTESIAN_POINT('Ctrl Pts',(20.5126995086046,15.8107444141161,0.));
#24668=CARTESIAN_POINT('Ctrl Pts',(20.644698628669,15.8947820241755,0.));
#24669=CARTESIAN_POINT('',(6.9,10.3676856018661,3.76156693666918));
#24670=CARTESIAN_POINT('Ctrl Pts',(12.7552064848291,12.1808231353727,6.59194920871187E-16));
#24671=CARTESIAN_POINT('Ctrl Pts',(12.4248760810931,12.0776861414938,0.209258199173966));
#24672=CARTESIAN_POINT('Ctrl Pts',(12.0982104932216,11.9767199532399,0.41544547449944));
#24673=CARTESIAN_POINT('Ctrl Pts',(11.7781027672104,11.8786008701973,0.615504762505627));
#24674=CARTESIAN_POINT('Ctrl Pts',(10.6475684461636,11.5320706807779,1.32206031539251));
#24675=CARTESIAN_POINT('Ctrl Pts',(9.62260979259592,11.2216626837413,1.98990731305582));
#24676=CARTESIAN_POINT('Ctrl Pts',(8.83596486703766,10.9799837756658,2.49396533620343));
#24677=CARTESIAN_POINT('Ctrl Pts',(8.38139303840122,10.8403268356446,2.78524106922678));
#24678=CARTESIAN_POINT('Ctrl Pts',(7.99983674904323,10.7217571528206,3.03224089473385));
#24679=CARTESIAN_POINT('Ctrl Pts',(7.59399878797648,10.5924943041424,3.29947542405694));
#24680=CARTESIAN_POINT('Ctrl Pts',(7.36159608752553,10.5184720637837,3.45250700864596));
#24681=CARTESIAN_POINT('Ctrl Pts',(7.13011481847682,10.4436463911284,3.6065023681803));
#24682=CARTESIAN_POINT('Ctrl Pts',(6.9,10.3676856018661,3.76156693666918));
#24683=CARTESIAN_POINT('',(6.9,11.02768739857,0.168526548660245));
#24684=CARTESIAN_POINT('Ctrl Pts',(6.90000000000001,10.3676856018661,3.76156693666918));
#24685=CARTESIAN_POINT('Ctrl Pts',(6.90000000000001,10.5551707158657,3.24481773355661));
#24686=CARTESIAN_POINT('Ctrl Pts',(6.90000000000001,10.7040448708755,2.71398840242746));
#24687=CARTESIAN_POINT('Ctrl Pts',(6.90000000000001,10.9457448952802,1.51153848953113));
#24688=CARTESIAN_POINT('Ctrl Pts',(6.90000000000001,11.0174195217678,0.840414370027655));
#24689=CARTESIAN_POINT('Ctrl Pts',(6.90000000000001,11.02768739857,0.168526548660246));
#24690=CARTESIAN_POINT('',(7.15673001668648,11.0509590216245,0.));
#24691=CARTESIAN_POINT('Ctrl Pts',(6.9,11.02768739857,0.168526548660244));
#24692=CARTESIAN_POINT('Ctrl Pts',(6.98321811561625,11.0352247901797,0.113609938717567));
#24693=CARTESIAN_POINT('Ctrl Pts',(7.06875995041873,11.0429732858603,0.0574496110044951));
#24694=CARTESIAN_POINT('Ctrl Pts',(7.15673001668648,11.0509590216245,5.89805981832114E-16));
#24695=CARTESIAN_POINT('',(6.5,11.,0.));
#24696=CARTESIAN_POINT('Ctrl Pts',(6.5,11.,0.));
#24697=CARTESIAN_POINT('Ctrl Pts',(6.63119408856029,11.0084469236697,0.));
#24698=CARTESIAN_POINT('Ctrl Pts',(6.76246413041996,11.0177661811298,0.));
#24699=CARTESIAN_POINT('Ctrl Pts',(6.89381012554657,11.0279577720712,0.));
#24700=CARTESIAN_POINT('Ctrl Pts',(7.02523209337025,11.0390219194522,0.));
#24701=CARTESIAN_POINT('Ctrl Pts',(7.15673001668648,11.0509590216245,0.));
#24702=CARTESIAN_POINT('Origin',(6.49999999999999,0.,0.));
#24703=CARTESIAN_POINT('',(37.5,27.2791366260183,-17.4816676818611));
#24704=CARTESIAN_POINT('Ctrl Pts',(7.15673001668648,11.0509590216245,-9.37018525099673E-16));
#24705=CARTESIAN_POINT('Ctrl Pts',(7.1627757905312,11.0515078441327,-0.00394824478753294));
#24706=CARTESIAN_POINT('Ctrl Pts',(7.1688330327612,11.0520577886114,-0.00790257982403587));
#24707=CARTESIAN_POINT('Ctrl Pts',(7.17490177695966,11.0526088641831,-0.0118630202121361));
#24708=CARTESIAN_POINT('Ctrl Pts',(7.97363370710642,11.1251381454716,-0.533112572338659));
#24709=CARTESIAN_POINT('Ctrl Pts',(8.96287699192994,11.2096234568595,-1.17519935778271));
#24710=CARTESIAN_POINT('Ctrl Pts',(10.2403166389167,11.35643287004,-1.93497252663744));
#24711=CARTESIAN_POINT('Ctrl Pts',(10.4394308581993,11.3793160189682,-2.05339819293429));
#24712=CARTESIAN_POINT('Ctrl Pts',(10.6449414398479,11.4036124907892,-2.17569004699468));
#24713=CARTESIAN_POINT('Ctrl Pts',(10.8572312781278,11.4296465357576,-2.30181054310029));
#24714=CARTESIAN_POINT('Ctrl Pts',(11.0079313537829,11.4481275548123,-2.39134082141595));
#24715=CARTESIAN_POINT('Ctrl Pts',(11.2445785601825,11.4774507093007,-2.53195589857672));
#24716=CARTESIAN_POINT('Ctrl Pts',(11.5512317955498,11.5182357344436,-2.71303157158667));
#24717=CARTESIAN_POINT('Ctrl Pts',(12.0044708154773,11.5785167381687,-2.98066468646132));
#24718=CARTESIAN_POINT('Ctrl Pts',(12.6082499220052,11.6630669066833,-3.33560663936012));
#24719=CARTESIAN_POINT('Ctrl Pts',(13.3027146141536,11.7808809827897,-3.73133446864291));
#24720=CARTESIAN_POINT('Ctrl Pts',(14.2466220417637,11.9410123512684,-4.26920261600178));
#24721=CARTESIAN_POINT('Ctrl Pts',(15.3788107201965,12.1625996834205,-4.92664534658129));
#24722=CARTESIAN_POINT('Ctrl Pts',(16.3720853361384,12.4089023460099,-5.48881820879722));
#24723=CARTESIAN_POINT('Ctrl Pts',(17.5300464833452,12.6960423867947,-6.14420023710243));
#24724=CARTESIAN_POINT('Ctrl Pts',(18.5522571217465,13.0002012582107,-6.74248287738912));
#24725=CARTESIAN_POINT('Ctrl Pts',(19.459740928474,13.3207494833101,-7.26206394073252));
#24726=CARTESIAN_POINT('Ctrl Pts',(20.7212139011992,13.7663364121569,-7.98432197298446));
#24727=CARTESIAN_POINT('Ctrl Pts',(21.7483180915102,14.2134327156149,-8.59417302928553));
#24728=CARTESIAN_POINT('Ctrl Pts',(22.5801692622301,14.6264461342272,-9.07708247839831));
#24729=CARTESIAN_POINT('Ctrl Pts',(23.3330995247457,15.0002753871561,-9.51417645757393));
#24730=CARTESIAN_POINT('Ctrl Pts',(23.9217876539353,15.3300824095171,-9.86132841188702));
#24731=CARTESIAN_POINT('Ctrl Pts',(24.4822919858724,15.6683207380631,-10.1904384385981));
#24732=CARTESIAN_POINT('Ctrl Pts',(24.941879286597,15.9456603259318,-10.4602932464902));
#24733=CARTESIAN_POINT('Ctrl Pts',(25.362627650419,16.2195872238312,-10.7067050298478));
#24734=CARTESIAN_POINT('Ctrl Pts',(25.7525302890143,16.489196921628,-10.9324873590558));
#24735=CARTESIAN_POINT('Ctrl Pts',(26.1776080055426,16.7831294661889,-11.1786386476902));
#24736=CARTESIAN_POINT('Ctrl Pts',(26.5661459570144,17.0742513036038,-11.3970084746332));
#24737=CARTESIAN_POINT('Ctrl Pts',(26.9267016829611,17.3573257272023,-11.599025816134));
#24738=CARTESIAN_POINT('Ctrl Pts',(27.1778854595225,17.5545315892941,-11.7397626707099));
#24739=CARTESIAN_POINT('Ctrl Pts',(27.4155006347892,17.7480067679896,-11.8724116206432));
#24740=CARTESIAN_POINT('Ctrl Pts',(27.6422489803864,17.9373681845498,-11.9995864201782));
#24741=CARTESIAN_POINT('Ctrl Pts',(27.8555706599492,18.1155167629601,-12.1192306970236));
#24742=CARTESIAN_POINT('Ctrl Pts',(28.1190985482968,18.3396168643745,-12.2669566516514));
#24743=CARTESIAN_POINT('Ctrl Pts',(28.4603120647768,18.6410520014603,-12.4627251930521));
#24744=CARTESIAN_POINT('Ctrl Pts',(28.6017780250843,18.7660259813254,-12.5438901626961));
#24745=CARTESIAN_POINT('Ctrl Pts',(28.7540312887841,18.9021185408524,-12.6319528845987));
#24746=CARTESIAN_POINT('Ctrl Pts',(28.9157341130969,19.0484400367167,-12.7269375546994));
#24747=CARTESIAN_POINT('Ctrl Pts',(29.4787137469301,19.5578685053511,-13.0576332925161));
#24748=CARTESIAN_POINT('Ctrl Pts',(30.1711677436348,20.2292610528631,-13.4573416990291));
#24749=CARTESIAN_POINT('Ctrl Pts',(30.8055547543663,20.8740009526386,-13.8222365905983));
#24750=CARTESIAN_POINT('Ctrl Pts',(31.1893125644353,21.2640215044727,-14.0429713504927));
#24751=CARTESIAN_POINT('Ctrl Pts',(31.5650207098983,21.6546118380209,-14.2588547919359));
#24752=CARTESIAN_POINT('Ctrl Pts',(31.9311744366493,22.036212583627,-14.4706295271113));
#24753=CARTESIAN_POINT('Ctrl Pts',(32.1142513000247,22.22701295643,-14.5765168946991));
#24754=CARTESIAN_POINT('Ctrl Pts',(32.2949430642597,22.4155611447437,-14.6813807665083));
#24755=CARTESIAN_POINT('Ctrl Pts',(32.4730466959716,22.6006686536293,-14.7853297275554));
#24756=CARTESIAN_POINT('Ctrl Pts',(32.5932788659621,22.7256289212046,-14.8555024075554));
#24757=CARTESIAN_POINT('Ctrl Pts',(32.7123311760698,22.8490214255785,-14.9252583804635));
#24758=CARTESIAN_POINT('Ctrl Pts',(32.8301302693162,22.9704904553367,-14.9946314854392));
#24759=CARTESIAN_POINT('Ctrl Pts',(32.8868306159552,23.0289572559155,-15.0280229062995));
#24760=CARTESIAN_POINT('Ctrl Pts',(32.9387123022521,23.0823367414253,-15.0586441387564));
#24761=CARTESIAN_POINT('Ctrl Pts',(33.,23.1451817466334,-15.0949277194305));
#24762=CARTESIAN_POINT('Ctrl Pts',(33.0955022515318,23.2431106902134,-15.1514670213678));
#24763=CARTESIAN_POINT('Ctrl Pts',(33.2417478451795,23.3926999986789,-15.2378324488783));
#24764=CARTESIAN_POINT('Ctrl Pts',(33.3688392456214,23.5219737265912,-15.3124686704877));
#24765=CARTESIAN_POINT('Ctrl Pts',(34.2661932188016,24.4347364545705,-15.8394524771927));
#24766=CARTESIAN_POINT('Ctrl Pts',(35.2319960543294,25.3874835189992,-16.3895212513103));
#24767=CARTESIAN_POINT('Ctrl Pts',(36.3004607334072,26.3047571717506,-16.9191094416468));
#24768=CARTESIAN_POINT('Ctrl Pts',(36.6891719087509,26.6384645246042,-17.1117754716474));
#24769=CARTESIAN_POINT('Ctrl Pts',(37.0893059759317,26.9653128027505,-17.3004814130194));
#24770=CARTESIAN_POINT('Ctrl Pts',(37.5,27.2791366260183,-17.4816676818611));
#24771=CARTESIAN_POINT('',(37.5,25.9430157904516,-19.4092743732572));
#24772=CARTESIAN_POINT('Origin',(37.5,0.,0.));
#24773=CARTESIAN_POINT('',(36.8,24.9564959511929,-19.6435328718186));
#24774=CARTESIAN_POINT('Ctrl Pts',(37.5,25.9430157904516,-19.4092743732572));
#24775=CARTESIAN_POINT('Ctrl Pts',(37.2470086540957,25.6235740187167,-19.4640189486865));
#24776=CARTESIAN_POINT('Ctrl Pts',(37.0122659037829,25.2931530107001,-19.5406617074869));
#24777=CARTESIAN_POINT('Ctrl Pts',(36.8,24.9564959511929,-19.6435328718186));
#24778=CARTESIAN_POINT('',(36.8,19.6435328718186,-24.956495951193));
#24779=CARTESIAN_POINT('Ctrl Pts',(36.8,24.9564959511929,-19.6435328718186));
#24780=CARTESIAN_POINT('Ctrl Pts',(36.8,24.4957748831848,-20.2288646216318));
#24781=CARTESIAN_POINT('Ctrl Pts',(36.8,24.0141222843113,-20.7984186457787));
#24782=CARTESIAN_POINT('Ctrl Pts',(36.8,22.3234241559746,-22.6602579716864));
#24783=CARTESIAN_POINT('Ctrl Pts',(36.8,21.029056769996,-23.8659348286794));
#24784=CARTESIAN_POINT('Ctrl Pts',(36.8,19.6435328718186,-24.956495951193));
#24785=CARTESIAN_POINT('',(37.5,19.4092743732571,-25.9430157904517));
#24786=CARTESIAN_POINT('Ctrl Pts',(36.8,19.6435328718186,-24.9564959511929));
#24787=CARTESIAN_POINT('Ctrl Pts',(37.0122659037829,19.5406617074868,-25.2931530107001));
#24788=CARTESIAN_POINT('Ctrl Pts',(37.2470086540956,19.4640189486865,-25.6235740187166));
#24789=CARTESIAN_POINT('Ctrl Pts',(37.5,19.4092743732571,-25.9430157904517));
#24790=CARTESIAN_POINT('',(37.5,17.4816676818611,-27.2791366260183));
#24791=CARTESIAN_POINT('Origin',(37.5,0.,0.));
#24792=CARTESIAN_POINT('',(6.9,10.8594625780008,-1.92623027574191));
#24793=CARTESIAN_POINT('Ctrl Pts',(37.5,17.4816676818611,-27.2791366260183));
#24794=CARTESIAN_POINT('Ctrl Pts',(36.6490696321361,17.1062619312001,-26.6289147924198));
#24795=CARTESIAN_POINT('Ctrl Pts',(35.8406537800854,16.6974222041734,-25.920783613057));
#24796=CARTESIAN_POINT('Ctrl Pts',(35.0774452370496,16.2828706254179,-25.2027592162947));
#24797=CARTESIAN_POINT('Ctrl Pts',(34.6958409655316,16.0755948360402,-24.8437470179135));
#24798=CARTESIAN_POINT('Ctrl Pts',(34.3255255041561,15.866901215486,-24.4822790638982));
#24799=CARTESIAN_POINT('Ctrl Pts',(33.966681063517,15.6603259087598,-24.1244801370593));
#24800=CARTESIAN_POINT('Ctrl Pts',(33.7186145566451,15.5175219275854,-23.8771363861421));
#24801=CARTESIAN_POINT('Ctrl Pts',(33.4671024168887,15.3704773316442,-23.6224476749935));
#24802=CARTESIAN_POINT('Ctrl Pts',(33.2400985609687,15.2367408626649,-23.3908093158965));
#24803=CARTESIAN_POINT('Ctrl Pts',(33.1387264796141,15.1770187748682,-23.2873676254985));
#24804=CARTESIAN_POINT('Ctrl Pts',(33.0532004124033,15.1264234604399,-23.1997339702838));
#24805=CARTESIAN_POINT('Ctrl Pts',(33.,15.0949277194305,-23.1451817466334));
#24806=CARTESIAN_POINT('Ctrl Pts',(32.9185691496266,15.0467189770979,-23.0616817555444));
#24807=CARTESIAN_POINT('Ctrl Pts',(32.851682063341,15.0068117561527,-22.993092707295));
#24808=CARTESIAN_POINT('Ctrl Pts',(32.7777321456029,14.9624828491712,-22.917277339216));
#24809=CARTESIAN_POINT('Ctrl Pts',(32.1788699540295,14.6034979145429,-22.3033083332787));
#24810=CARTESIAN_POINT('Ctrl Pts',(31.5692879871724,14.2222611802151,-21.6797224976956));
#24811=CARTESIAN_POINT('Ctrl Pts',(30.9513498040902,13.8532805894451,-21.057417903561));
#24812=CARTESIAN_POINT('Ctrl Pts',(30.6423807125491,13.6687902940601,-20.7462656064936));
#24813=CARTESIAN_POINT('Ctrl Pts',(30.3347880607216,13.4893931931417,-20.438831527849));
#24814=CARTESIAN_POINT('Ctrl Pts',(30.0249306372018,13.3164737289158,-20.1317191404522));
#24815=CARTESIAN_POINT('Ctrl Pts',(29.8700019254419,13.2300139968029,-19.9781629467538));
#24816=CARTESIAN_POINT('Ctrl Pts',(29.7145097313597,13.1451740097154,-19.8246838084796));
#24817=CARTESIAN_POINT('Ctrl Pts',(29.5580100720529,13.0621556215307,-19.6708282829286));
#24818=CARTESIAN_POINT('Ctrl Pts',(29.4797602423995,13.0206464274383,-19.5939005201531));
#24819=CARTESIAN_POINT('Ctrl Pts',(29.4012586241266,12.9795931491564,-19.5168782891895));
#24820=CARTESIAN_POINT('Ctrl Pts',(29.3224502420539,12.9390249501939,-19.4397024434204));
#24821=CARTESIAN_POINT('Ctrl Pts',(29.2736528206195,12.9139054965325,-19.3919158733691));
#24822=CARTESIAN_POINT('Ctrl Pts',(29.2247377937366,12.888972078638,-19.3440703736513));
#24823=CARTESIAN_POINT('Ctrl Pts',(29.1756921969699,12.8642322645676,-19.2961515487725));
#24824=CARTESIAN_POINT('Ctrl Pts',(29.145528605723,12.8490170018663,-19.2666809348548));
#24825=CARTESIAN_POINT('Ctrl Pts',(29.1181490968401,12.8352852879351,-19.2399471036097));
#24826=CARTESIAN_POINT('Ctrl Pts',(29.0849408699094,12.8187535959654,-19.2075463476651));
#24827=CARTESIAN_POINT('Ctrl Pts',(29.0475462331541,12.8001378289312,-19.171060976083));
#24828=CARTESIAN_POINT('Ctrl Pts',(28.9599837408533,12.7566467272304,-19.085912836999));
#24829=CARTESIAN_POINT('Ctrl Pts',(28.8924081848686,12.723282629515,-19.0206341515183));
#24830=CARTESIAN_POINT('Ctrl Pts',(28.4410807636346,12.5004486185436,-18.5846471980972));
#24831=CARTESIAN_POINT('Ctrl Pts',(27.9936088568923,12.2860610268384,-18.1669902803128));
#24832=CARTESIAN_POINT('Ctrl Pts',(27.5122543097622,12.0773485866518,-17.7276863429211));
#24833=CARTESIAN_POINT('Ctrl Pts',(27.1397294107683,11.9158240281682,-17.3877048139625));
#24834=CARTESIAN_POINT('Ctrl Pts',(26.7276341641932,11.7479547990202,-17.0180715474313));
#24835=CARTESIAN_POINT('Ctrl Pts',(26.2530417505368,11.5897211649258,-16.593147989986));
#24836=CARTESIAN_POINT('Ctrl Pts',(25.8694949138879,11.461842993969,-16.2497415604139));
#24837=CARTESIAN_POINT('Ctrl Pts',(25.4447383161179,11.3368019000543,-15.8721943512539));
#24838=CARTESIAN_POINT('Ctrl Pts',(24.9635886608488,11.2164808476641,-15.4528606650932));
#24839=CARTESIAN_POINT('Ctrl Pts',(24.6119820458997,11.1285546120849,-15.1464269052216));
#24840=CARTESIAN_POINT('Ctrl Pts',(24.2873626784893,11.0505455233575,-14.8634583858277));
#24841=CARTESIAN_POINT('Ctrl Pts',(23.642661641557,10.9290047499035,-14.322314359714));
#24842=CARTESIAN_POINT('Ctrl Pts',(23.576053321007,10.9164475701654,-14.2664051976524));
#24843=CARTESIAN_POINT('Ctrl Pts',(23.5065967304414,10.903616097419,-14.2082779526344));
#24844=CARTESIAN_POINT('Ctrl Pts',(23.4342591639586,10.8905593535264,-14.1479547088373));
#24845=CARTESIAN_POINT('Ctrl Pts',(22.7443384436268,10.7660304456639,-13.5726207871031));
#24846=CARTESIAN_POINT('Ctrl Pts',(21.7987837593176,10.6409180002013,-12.7862027918382));
#24847=CARTESIAN_POINT('Ctrl Pts',(20.5610365528855,10.544989531356,-11.8220942510713));
#24848=CARTESIAN_POINT('Ctrl Pts',(19.7234582214113,10.480075139743,-11.1696860543579));
#24849=CARTESIAN_POINT('Ctrl Pts',(18.7603809281633,10.4499377288461,-10.4236916548838));
#24850=CARTESIAN_POINT('Ctrl Pts',(17.6514222906382,10.4358767824859,-9.60745933070834));
#24851=CARTESIAN_POINT('Ctrl Pts',(16.7565277906389,10.4245300440805,-8.94878569500228));
#24852=CARTESIAN_POINT('Ctrl Pts',(15.7613807992389,10.4463397170533,-8.21650708627012));
#24853=CARTESIAN_POINT('Ctrl Pts',(14.7199652846762,10.4731931404427,-7.48053645516582));
#24854=CARTESIAN_POINT('Ctrl Pts',(13.7316067501733,10.4986784628874,-6.78206130838355));
#24855=CARTESIAN_POINT('Ctrl Pts',(12.7260968661244,10.5503343111255,-6.06464296565695));
#24856=CARTESIAN_POINT('Ctrl Pts',(11.7781012037546,10.5949225697956,-5.40625658879284));
#24857=CARTESIAN_POINT('Ctrl Pts',(10.6475718363526,10.6480961631663,-4.62109990117507));
#24858=CARTESIAN_POINT('Ctrl Pts',(9.62260863652897,10.713198677066,-3.88752023758455));
#24859=CARTESIAN_POINT('Ctrl Pts',(8.83596460437641,10.7559275652365,-3.33015436441791));
#24860=CARTESIAN_POINT('Ctrl Pts',(8.38131550044803,10.7806231707767,-3.00801895826468));
#24861=CARTESIAN_POINT('Ctrl Pts',(7.9996968849037,10.8014421627467,-2.73478088895419));
#24862=CARTESIAN_POINT('Ctrl Pts',(7.59379043301474,10.8231179952784,-2.43866561789793));
#24863=CARTESIAN_POINT('Ctrl Pts',(7.36145773430791,10.8355248063683,-2.26917518547774));
#24864=CARTESIAN_POINT('Ctrl Pts',(7.13004605045641,10.8477177778402,-2.09844904428941));
#24865=CARTESIAN_POINT('Ctrl Pts',(6.9,10.8594625780007,-1.92623027574191));
#24866=CARTESIAN_POINT('',(6.9,9.63452070648529,-5.36789542693313));
#24867=CARTESIAN_POINT('Ctrl Pts',(6.90000000000001,10.8594625780008,-1.92623027574191));
#24868=CARTESIAN_POINT('Ctrl Pts',(6.90000000000001,10.7829659225815,-2.35749364924905));
#24869=CARTESIAN_POINT('Ctrl Pts',(6.90000000000001,10.6806923192591,-2.78469328079874));
#24870=CARTESIAN_POINT('Ctrl Pts',(6.90000000000001,10.3240838050858,-3.95869001001801));
#24871=CARTESIAN_POINT('Ctrl Pts',(6.90000000000001,10.0158641401962,-4.6834444613023));
#24872=CARTESIAN_POINT('Ctrl Pts',(6.90000000000001,9.63452070648529,-5.36789542693313));
#24873=CARTESIAN_POINT('',(37.5,14.8835914705078,-28.7791366260183));
#24874=CARTESIAN_POINT('Ctrl Pts',(6.9,9.63452070648529,-5.36789542693313));
#24875=CARTESIAN_POINT('Ctrl Pts',(6.98893730997611,9.61215150215923,-5.42275082836604));
#24876=CARTESIAN_POINT('Ctrl Pts',(7.080528923883,9.58928076274039,-5.47895708413964));
#24877=CARTESIAN_POINT('Ctrl Pts',(7.17490192378011,9.56590850800827,-5.5365781986047));
#24878=CARTESIAN_POINT('Ctrl Pts',(7.97363347623888,9.36809602639803,-6.02425796147394));
#24879=CARTESIAN_POINT('Ctrl Pts',(8.96286060506815,9.12022229066503,-6.62255487684896));
#24880=CARTESIAN_POINT('Ctrl Pts',(10.2403127965964,8.8674738587251,-7.35394959882413));
#24881=CARTESIAN_POINT('Ctrl Pts',(10.4394276407776,8.82807828292467,-7.4679511615181));
#24882=CARTESIAN_POINT('Ctrl Pts',(10.6449386760845,8.78797362786098,-7.58600750915109));
#24883=CARTESIAN_POINT('Ctrl Pts',(10.8572270226684,8.74745979681899,-7.70824722252714));
#24884=CARTESIAN_POINT('Ctrl Pts',(11.0079272577466,8.71869965072432,-7.79502331663734));
#24885=CARTESIAN_POINT('Ctrl Pts',(11.2445718662815,8.67378718135597,-7.93145962014351));
#24886=CARTESIAN_POINT('Ctrl Pts',(11.5512244267323,8.61857029386601,-8.10866787119591));
#24887=CARTESIAN_POINT('Ctrl Pts',(12.0044642696576,8.53695840914545,-8.37058591862391));
#24888=CARTESIAN_POINT('Ctrl Pts',(12.6082461583963,8.43270942691138,-8.72025136351868));
#24889=CARTESIAN_POINT('Ctrl Pts',(13.3027146141536,8.3368749757354,-9.12187093125612));
#24890=CARTESIAN_POINT('Ctrl Pts',(14.2466220416827,8.20661873511246,-9.6677440949479));
#24891=CARTESIAN_POINT('Ctrl Pts',(15.3788107201281,8.06979762861672,-10.347899867244));
#24892=CARTESIAN_POINT('Ctrl Pts',(16.3720853361384,8.00201556032624,-10.9579071785779));
#24893=CARTESIAN_POINT('Ctrl Pts',(17.530046483338,7.92299511593749,-11.6690546846619));
#24894=CARTESIAN_POINT('Ctrl Pts',(18.5522571217484,7.88726310522635,-12.3392620855072));
#24895=CARTESIAN_POINT('Ctrl Pts',(19.459740928474,7.90507547962869,-12.9495065982363));
#24896=CARTESIAN_POINT('Ctrl Pts',(20.7212139012673,7.92983606347967,-13.7977938667231));
#24897=CARTESIAN_POINT('Ctrl Pts',(21.7483180915983,8.0121072920729,-14.5494885257539));
#24898=CARTESIAN_POINT('Ctrl Pts',(22.5801692622301,8.12833268012626,-15.1742070856531));
#24899=CARTESIAN_POINT('Ctrl Pts',(23.3330995245126,8.23353132022012,-15.7396562017498));
#24900=CARTESIAN_POINT('Ctrl Pts',(23.9217876533125,8.34557660269292,-16.2052021240247));
#24901=CARTESIAN_POINT('Ctrl Pts',(24.4822919849709,8.47394457429969,-16.6593389318286));
#24902=CARTESIAN_POINT('Ctrl Pts',(24.9418792860364,8.57920029897796,-17.0317098449944));
#24903=CARTESIAN_POINT('Ctrl Pts',(25.3626276501528,8.69322205972909,-17.3820721583649));
#24904=CARTESIAN_POINT('Ctrl Pts',(25.7525302890143,8.8138197426061,-17.7124102403086));
#24905=CARTESIAN_POINT('Ctrl Pts',(26.1776080054479,8.94529714884838,-18.0725497816404));
#24906=CARTESIAN_POINT('Ctrl Pts',(26.5661459568577,9.08823114214577,-18.4072245178454));
#24907=CARTESIAN_POINT('Ctrl Pts',(26.9267016827717,9.2323721133757,-18.7237138793584));
#24908=CARTESIAN_POINT('Ctrl Pts',(27.1778777838254,9.33278590395925,-18.9441917642909));
#24909=CARTESIAN_POINT('Ctrl Pts',(27.4154861114682,9.43401273563673,-19.1558005175256));
#24910=CARTESIAN_POINT('Ctrl Pts',(27.6422281937235,9.5344141104218,-19.3606119908812));
#24911=CARTESIAN_POINT('Ctrl Pts',(27.855555992985,9.6288756418353,-19.5533066174801));
#24912=CARTESIAN_POINT('Ctrl Pts',(28.119083718991,9.74908875996703,-19.7932907120163));
#24913=CARTESIAN_POINT('Ctrl Pts',(28.4603051775176,9.91225869656093,-20.1135561540163));
#24914=CARTESIAN_POINT('Ctrl Pts',(28.6017730832022,9.97990775151866,-20.2463358494625));
#24915=CARTESIAN_POINT('Ctrl Pts',(28.7540286646177,10.0537371137215,-20.3906488456919));
#24916=CARTESIAN_POINT('Ctrl Pts',(28.9157341130969,10.1329641969115,-20.5460712531062));
#24917=CARTESIAN_POINT('Ctrl Pts',(29.4787137469273,10.4087943232502,-21.0871763972933));
#24918=CARTESIAN_POINT('Ctrl Pts',(30.1711677436288,10.7903831220487,-21.7690303051924));
#24919=CARTESIAN_POINT('Ctrl Pts',(30.805554754357,11.1662968083009,-22.4074085008868));
#24920=CARTESIAN_POINT('Ctrl Pts',(31.1893125644278,11.393697134241,-22.7935806863724));
#24921=CARTESIAN_POINT('Ctrl Pts',(31.5650207098923,11.6240165648458,-23.1758363976944));
#24922=CARTESIAN_POINT('Ctrl Pts',(31.9311744366447,11.8486051370568,-23.5500390710405));
#24923=CARTESIAN_POINT('Ctrl Pts',(32.1142513000209,11.9608994231623,-23.7371404077135));
#24924=CARTESIAN_POINT('Ctrl Pts',(32.2949430642566,12.0717550081754,-23.9222292787971));
#24925=CARTESIAN_POINT('Ctrl Pts',(32.4730466959692,12.1800883327784,-24.1048054742044));
#24926=CARTESIAN_POINT('Ctrl Pts',(32.5932788659337,12.2532207589465,-24.228056931497));
#24927=CARTESIAN_POINT('Ctrl Pts',(32.7123311760158,12.3252038159015,-24.3501636282619));
#24928=CARTESIAN_POINT('Ctrl Pts',(32.8301302692372,12.3957125289427,-24.4709770143638));
#24929=CARTESIAN_POINT('Ctrl Pts',(32.8868306159027,12.4296505531077,-24.5291282334138));
#24930=CARTESIAN_POINT('Ctrl Pts',(32.9387123022199,12.460567927384,-24.5823367413923));
#24931=CARTESIAN_POINT('Ctrl Pts',(33.,12.4968515080772,-24.6451817466334));
#24932=CARTESIAN_POINT('Ctrl Pts',(33.0955022515025,12.5533908099972,-24.7431106901834));
#24933=CARTESIAN_POINT('Ctrl Pts',(33.2417478451207,12.6397562374902,-24.8926999986187));
#24934=CARTESIAN_POINT('Ctrl Pts',(33.3688392455332,12.7143924590826,-25.0219737265016));
#24935=CARTESIAN_POINT('Ctrl Pts',(34.266193218727,13.2413762657968,-25.9347364544968));
#24936=CARTESIAN_POINT('Ctrl Pts',(35.2319960542628,13.7914450399216,-26.887483518938));
#24937=CARTESIAN_POINT('Ctrl Pts',(36.3004607333556,14.3210332302679,-27.8047571717062));
#24938=CARTESIAN_POINT('Ctrl Pts',(36.6891719087154,14.5136992602774,-28.1384645245753));
#24939=CARTESIAN_POINT('Ctrl Pts',(37.0893059759135,14.702405201658,-28.4653128027367));
#24940=CARTESIAN_POINT('Ctrl Pts',(37.5,14.8835914705078,-28.7791366260183));
#24941=CARTESIAN_POINT('',(37.5,12.7626735386834,-29.7804325714888));
#24942=CARTESIAN_POINT('Origin',(37.5,0.,0.));
#24943=CARTESIAN_POINT('',(36.8,11.7911930472673,-29.4900464626661));
#24944=CARTESIAN_POINT('Ctrl Pts',(37.5,12.7626735386834,-29.7804325714888));
#24945=CARTESIAN_POINT('Ctrl Pts',(37.2470086540957,12.4586565616163,-29.6681218786625));
#24946=CARTESIAN_POINT('Ctrl Pts',(37.0122659037829,12.1341821953298,-29.5692859507915));
#24947=CARTESIAN_POINT('Ctrl Pts',(36.8,11.7911930472673,-29.4900464626661));
#24948=CARTESIAN_POINT('',(36.8,4.53355051147313,-31.4347259190859));
#24949=CARTESIAN_POINT('Ctrl Pts',(36.8,11.7911930472673,-29.4900464626661));
#24950=CARTESIAN_POINT('Ctrl Pts',(36.8,9.45611053488411,-30.4236973716148));
#24951=CARTESIAN_POINT('Ctrl Pts',(36.8,7.01967470941751,-31.0761743714062));
#24952=CARTESIAN_POINT('Ctrl Pts',(36.8,4.53355051147313,-31.4347259190859));
#24953=CARTESIAN_POINT('',(37.5,3.83741678103714,-32.1719479119405));
#24954=CARTESIAN_POINT('Ctrl Pts',(36.8,4.53355051147313,-31.4347259190859));
#24955=CARTESIAN_POINT('Ctrl Pts',(37.012265903783,4.27613294009133,-31.6748439028166));
#24956=CARTESIAN_POINT('Ctrl Pts',(37.2470086540957,4.04454785994585,-31.9226755103028));
#24957=CARTESIAN_POINT('Ctrl Pts',(37.5,3.83741678103715,-32.1719479119405));
#24958=CARTESIAN_POINT('',(37.5,1.5,-32.3652591523689));
#24959=CARTESIAN_POINT('Origin',(37.5,0.,0.));
#24960=CARTESIAN_POINT('',(6.9,8.44145532612415,-7.09789564133157));
#24961=CARTESIAN_POINT('Ctrl Pts',(37.5,1.5,-32.3652591523689));
#24962=CARTESIAN_POINT('Ctrl Pts',(36.6490696321407,1.5,-31.6144476510508));
#24963=CARTESIAN_POINT('Ctrl Pts',(35.8406537800942,1.49999999999999,-30.7967681970023));
#24964=CARTESIAN_POINT('Ctrl Pts',(35.0774452370622,1.49999999999999,-29.9676650394963));
#24965=CARTESIAN_POINT('Ctrl Pts',(34.6958409655462,1.49999999999999,-29.5531134607433));
#24966=CARTESIAN_POINT('Ctrl Pts',(34.3255255041725,1.49999999999999,-29.1357262196373));
#24967=CARTESIAN_POINT('Ctrl Pts',(33.9666810635352,1.49999999999999,-28.7225756061873));
#24968=CARTESIAN_POINT('Ctrl Pts',(33.7186145566422,1.49999999999999,-28.4369676438145));
#24969=CARTESIAN_POINT('Ctrl Pts',(33.4671024168586,1.49999999999999,-28.1428784518998));
#24970=CARTESIAN_POINT('Ctrl Pts',(33.2400985609282,1.49999999999999,-27.8754055139288));
#24971=CARTESIAN_POINT('Ctrl Pts',(33.1387264795984,1.49999999999999,-27.7559613383644));
#24972=CARTESIAN_POINT('Ctrl Pts',(33.0532004124087,1.49999999999999,-27.6547707095329));
#24973=CARTESIAN_POINT('Ctrl Pts',(33.,1.49999999999999,-27.5917792275077));
#24974=CARTESIAN_POINT('Ctrl Pts',(32.9185691494976,1.49999999999999,-27.4953617426897));
#24975=CARTESIAN_POINT('Ctrl Pts',(32.8516820633063,1.49973385699142,-27.4160082741233));
#24976=CARTESIAN_POINT('Ctrl Pts',(32.7777321456263,1.49925158146344,-27.3281857859478));
#24977=CARTESIAN_POINT('Ctrl Pts',(32.17886995405,1.49534601146838,-26.6169805623525));
#24978=CARTESIAN_POINT('Ctrl Pts',(31.5692879871895,1.47697823247614,-25.8863210201293));
#24979=CARTESIAN_POINT('Ctrl Pts',(30.9513498041028,1.46858396443303,-25.1628991373263));
#24980=CARTESIAN_POINT('Ctrl Pts',(30.6423807125594,1.46438683041148,-24.8011881959248));
#24981=CARTESIAN_POINT('Ctrl Pts',(30.3347880607298,1.46274142297308,-24.4452439233677));
#24982=CARTESIAN_POINT('Ctrl Pts',(30.024930637208,1.46654496784305,-24.09281706195));
#24983=CARTESIAN_POINT('Ctrl Pts',(29.8700019254471,1.46844674027804,-23.9166036312412));
#24984=CARTESIAN_POINT('Ctrl Pts',(29.7145097313639,1.47171272534061,-23.7412668049999));
#24985=CARTESIAN_POINT('Ctrl Pts',(29.5580100720561,1.47674445496688,-23.5665148172665));
#24986=CARTESIAN_POINT('Ctrl Pts',(29.4797602424023,1.47926031978001,-23.4791388233998));
#24987=CARTESIAN_POINT('Ctrl Pts',(29.4012586241288,1.48221825336111,-23.3919089755878));
#24988=CARTESIAN_POINT('Ctrl Pts',(29.3224502420556,1.48567308535834,-23.3047886331113));
#24989=CARTESIAN_POINT('Ctrl Pts',(29.2736528205877,1.48781228538547,-23.2508445226193));
#24990=CARTESIAN_POINT('Ctrl Pts',(29.224737793671,1.49014206194626,-23.1969423954228));
#24991=CARTESIAN_POINT('Ctrl Pts',(29.1756921968704,1.4926761669178,-23.143073568686));
#24992=CARTESIAN_POINT('Ctrl Pts',(29.1455286056567,1.4942346698506,-23.1099436370539));
#24993=CARTESIAN_POINT('Ctrl Pts',(29.1181490968019,1.49570957236975,-23.0799256031206));
#24994=CARTESIAN_POINT('Ctrl Pts',(29.0849408699094,1.4975930851266,-23.0435998794277));
#24995=CARTESIAN_POINT('Ctrl Pts',(29.0475462330949,1.4997140437585,-23.0026947371893));
#24996=CARTESIAN_POINT('Ctrl Pts',(28.959983740694,1.50462371439458,-22.9072087346982));
#24997=CARTESIAN_POINT('Ctrl Pts',(28.8924081846116,1.50836890094434,-22.8339936857838));
#24998=CARTESIAN_POINT('Ctrl Pts',(28.4410807633312,1.53338246332861,-22.3450009028729));
#24999=CARTESIAN_POINT('Ctrl Pts',(27.9936088565663,1.55654582154998,-21.876105606136));
#25000=CARTESIAN_POINT('Ctrl Pts',(27.5122543093545,1.59544751497299,-21.3913010162073));
#25001=CARTESIAN_POINT('Ctrl Pts',(27.139729410468,1.62555390846788,-21.0161060961865));
#25002=CARTESIAN_POINT('Ctrl Pts',(26.7276341640204,1.66499152477457,-20.612059682844));
#25003=CARTESIAN_POINT('Ctrl Pts',(26.2530417505368,1.74041895661093,-20.1649482705455));
#25004=CARTESIAN_POINT('Ctrl Pts',(25.8694949138893,1.80137642675868,-19.803610493236));
#25005=CARTESIAN_POINT('Ctrl Pts',(25.4447383161208,1.88186126749126,-19.4141244720195));
#25006=CARTESIAN_POINT('Ctrl Pts',(24.9635886608536,1.98732702259108,-18.9908103209483));
#25007=CARTESIAN_POINT('Ctrl Pts',(24.6119820458962,2.06439754885796,-18.6814677825253));
#25008=CARTESIAN_POINT('Ctrl Pts',(24.2873626784783,2.13832395599249,-18.3974053118883));
#25009=CARTESIAN_POINT('Ctrl Pts',(23.6426616415203,2.30363857164967,-17.8679904514206));
#25010=CARTESIAN_POINT('Ctrl Pts',(23.5760533209815,2.32071831602454,-17.8132931069111));
#25011=CARTESIAN_POINT('Ctrl Pts',(23.5065967304281,2.33866955716406,-17.7565376997104));
#25012=CARTESIAN_POINT('Ctrl Pts',(23.4342591639586,2.35752370715749,-17.697767866208));
#25013=CARTESIAN_POINT('Ctrl Pts',(22.7443384436274,2.53734547031001,-17.1372496203964));
#25014=CARTESIAN_POINT('Ctrl Pts',(21.7987837593181,2.82220391184217,-16.3936354357724));
#25015=CARTESIAN_POINT('Ctrl Pts',(20.5610365528855,3.2211816912596,-15.5107287130397));
#25016=CARTESIAN_POINT('Ctrl Pts',(19.7234582214114,3.49116827740818,-14.9132694452422));
#25017=CARTESIAN_POINT('Ctrl Pts',(18.7603809281634,3.83806571370429,-14.2521506387683));
#25018=CARTESIAN_POINT('Ctrl Pts',(17.6514222906382,4.23400473904287,-13.5382422374622));
#25019=CARTESIAN_POINT('Ctrl Pts',(16.7565277906389,4.55351499318665,-12.962140766935));
#25020=CARTESIAN_POINT('Ctrl Pts',(15.7613807992389,4.93854202839548,-12.3388737256115));
#25021=CARTESIAN_POINT('Ctrl Pts',(14.7199652846762,5.32978309078144,-11.7149311743306));
#25022=CARTESIAN_POINT('Ctrl Pts',(13.7316067501733,5.70109160083332,-11.1227766145274));
#25023=CARTESIAN_POINT('Ctrl Pts',(12.7260968661244,6.1045360490248,-10.5273020287043));
#25024=CARTESIAN_POINT('Ctrl Pts',(11.7781012037546,6.47234380217571,-9.97941683016941));
#25025=CARTESIAN_POINT('Ctrl Pts',(10.6475718363527,6.91097182865409,-9.32603798942655));
#25026=CARTESIAN_POINT('Ctrl Pts',(9.62260863652904,7.33414209133672,-8.72329062200738));
#25027=CARTESIAN_POINT('Ctrl Pts',(8.83596460437641,7.64982933055117,-8.26196206072778));
#25028=CARTESIAN_POINT('Ctrl Pts',(8.38131550044628,7.83228405538812,-7.99533241830972));
#25029=CARTESIAN_POINT('Ctrl Pts',(7.99969688490065,7.98693286597114,-7.76911080499006));
#25030=CARTESIAN_POINT('Ctrl Pts',(7.59379043301065,8.15376232312029,-7.52350537407199));
#25031=CARTESIAN_POINT('Ctrl Pts',(7.36145773430516,8.24925215291372,-7.38292575944348));
#25032=CARTESIAN_POINT('Ctrl Pts',(7.13004605045505,8.34517464654957,-7.24116906982106));
#25033=CARTESIAN_POINT('Ctrl Pts',(6.9,8.44145532612415,-7.09789564133157));
#25034=CARTESIAN_POINT('',(6.9,5.6597919716369,-9.46599415782505));
#25035=CARTESIAN_POINT('Ctrl Pts',(6.90000000000001,8.44145532612415,-7.09789564133157));
#25036=CARTESIAN_POINT('Ctrl Pts',(6.90000000000001,8.09681826844945,-7.5077690000137));
#25037=CARTESIAN_POINT('Ctrl Pts',(6.89999999999998,7.72210951819363,-7.89280389060836));
#25038=CARTESIAN_POINT('Ctrl Pts',(6.89999999999998,6.80464666682922,-8.70687723936702));
#25039=CARTESIAN_POINT('Ctrl Pts',(6.90000000000001,6.24868352466685,-9.11389129061079));
#25040=CARTESIAN_POINT('Ctrl Pts',(6.90000000000001,5.6597919716369,-9.46599415782505));
#25041=CARTESIAN_POINT('',(37.5,-1.50000000000001,-32.3652591523689));
#25042=CARTESIAN_POINT('Ctrl Pts',(6.9,5.6597919716369,-9.46599415782505));
#25043=CARTESIAN_POINT('Ctrl Pts',(6.98893730997641,5.61299197171148,-9.50231572683784));
#25044=CARTESIAN_POINT('Ctrl Pts',(7.08052892388333,5.56508220248461,-9.53955640247996));
#25045=CARTESIAN_POINT('Ctrl Pts',(7.17490192378012,5.51603067891051,-9.57777162403489));
#25046=CARTESIAN_POINT('Ctrl Pts',(7.97363347626345,5.10088016320301,-9.90120844679605));
#25047=CARTESIAN_POINT('Ctrl Pts',(8.96286060510633,4.58706675343506,-10.2954119066554));
#25048=CARTESIAN_POINT('Ctrl Pts',(10.2403127965964,4.00248282963831,-10.8024441000946));
#25049=CARTESIAN_POINT('Ctrl Pts',(10.4394276407757,3.91136447885229,-10.8814745615578));
#25050=CARTESIAN_POINT('Ctrl Pts',(10.6449386760798,3.81760465494192,-10.963662030153));
#25051=CARTESIAN_POINT('Ctrl Pts',(10.8572270226597,3.72139879136867,-11.0492678117653));
#25052=CARTESIAN_POINT('Ctrl Pts',(11.0079272578272,3.65310372713856,-11.1100380406946));
#25053=CARTESIAN_POINT('Ctrl Pts',(11.2445718663453,3.54599023597307,-11.2057391108383));
#25054=CARTESIAN_POINT('Ctrl Pts',(11.5512244269296,3.40956688310414,-11.3315975143204));
#25055=CARTESIAN_POINT('Ctrl Pts',(12.0044642698092,3.20792989399308,-11.5176192547245));
#25056=CARTESIAN_POINT('Ctrl Pts',(12.6082461584696,2.94281490464851,-11.7683139216804));
#25057=CARTESIAN_POINT('Ctrl Pts',(13.3027146141536,2.65901005153358,-12.0682094443783));
#25058=CARTESIAN_POINT('Ctrl Pts',(14.2466220416228,2.27326825633123,-12.4758213510422));
#25059=CARTESIAN_POINT('Ctrl Pts',(15.3788107200775,1.81469981617802,-12.9964429751341));
#25060=CARTESIAN_POINT('Ctrl Pts',(16.3720853361384,1.45099516743195,-13.4908337691235));
#25061=CARTESIAN_POINT('Ctrl Pts',(17.5300464833328,1.02698770213283,-14.0671953530332));
#25062=CARTESIAN_POINT('Ctrl Pts',(18.55225712175,0.660939172703652,-14.6297459826175));
#25063=CARTESIAN_POINT('Ctrl Pts',(19.459740928474,0.371242885073749,-15.1671394203612));
#25064=CARTESIAN_POINT('Ctrl Pts',(20.7212139013182,-0.0314574545583951,
-15.9141580365333));
#25065=CARTESIAN_POINT('Ctrl Pts',(21.748318091664,-0.336055810111993,-16.6062803214569));
#25066=CARTESIAN_POINT('Ctrl Pts',(22.5801692622301,-0.547760951425959,
-17.2054151585246));
#25067=CARTESIAN_POINT('Ctrl Pts',(23.3330995243319,-0.739380814663484,
-17.7477077775286));
#25068=CARTESIAN_POINT('Ctrl Pts',(23.9217876528372,-0.87511971474023,-18.2069050138462));
#25069=CARTESIAN_POINT('Ctrl Pts',(24.4822919842876,-0.991018194168117,
-18.6643830118107));
#25070=CARTESIAN_POINT('Ctrl Pts',(24.9418792856086,-1.08604951934922,-19.0394935447735));
#25071=CARTESIAN_POINT('Ctrl Pts',(25.3626276499481,-1.16248493468587,-19.3999270892409));
#25072=CARTESIAN_POINT('Ctrl Pts',(25.7525302890144,-1.22321331868058,-19.7463071016619));
#25073=CARTESIAN_POINT('Ctrl Pts',(26.1776080053149,-1.28942031549629,-20.1239357963656));
#25074=CARTESIAN_POINT('Ctrl Pts',(26.5661459566312,-1.33297321433427,-20.4852396164797));
#25075=CARTESIAN_POINT('Ctrl Pts',(26.9267016824847,-1.36638815227823,-20.831397929128));
#25076=CARTESIAN_POINT('Ctrl Pts',(27.1778777834673,-1.38966620120527,-21.0725442736714));
#25077=CARTESIAN_POINT('Ctrl Pts',(27.4154861110583,-1.40780557004487,-21.3064162454173));
#25078=CARTESIAN_POINT('Ctrl Pts',(27.6422281932782,-1.42326116558415,-21.5339888716807));
#25079=CARTESIAN_POINT('Ctrl Pts',(27.8555559926927,-1.43780239301204,-21.7480980793427));
#25080=CARTESIAN_POINT('Ctrl Pts',(28.1190837187058,-1.45368682611151,-22.0160369607817));
#25081=CARTESIAN_POINT('Ctrl Pts',(28.4603051774444,-1.4725102368991,-22.3749799380264));
#25082=CARTESIAN_POINT('Ctrl Pts',(28.6017730831488,-1.48031428448795,-22.5237950548888));
#25083=CARTESIAN_POINT('Ctrl Pts',(28.754028664589,-1.48853267939111,-22.6856884568469));
#25084=CARTESIAN_POINT('Ctrl Pts',(28.9157341130969,-1.49763121638955,-22.8599017516109));
#25085=CARTESIAN_POINT('Ctrl Pts',(29.4787137469139,-1.52930789194394,-23.4664276157502));
#25086=CARTESIAN_POINT('Ctrl Pts',(30.1711677436051,-1.53976925233501,-24.2477248210474));
#25087=CARTESIAN_POINT('Ctrl Pts',(30.8055547543247,-1.53340754825804,-24.9885333988561));
#25088=CARTESIAN_POINT('Ctrl Pts',(31.1893125644012,-1.52955918190804,-25.4366684846978));
#25089=CARTESIAN_POINT('Ctrl Pts',(31.5650207098714,-1.52122455968006,-25.8828713567533));
#25090=CARTESIAN_POINT('Ctrl Pts',(31.9311744366292,-1.51382648741854,-26.319234664147));
#25091=CARTESIAN_POINT('Ctrl Pts',(32.1142513000081,-1.51012745128778,-26.5374163178438));
#25092=CARTESIAN_POINT('Ctrl Pts',(32.2949430642463,-1.50666813405683,-26.7531357746696));
#25093=CARTESIAN_POINT('Ctrl Pts',(32.4730466959614,-1.50413682057774,-26.9654180603231));
#25094=CARTESIAN_POINT('Ctrl Pts',(32.5932788659635,-1.50242801032152,-27.1087231665209));
#25095=CARTESIAN_POINT('Ctrl Pts',(32.7123311760826,-1.50114220273856,-27.2504621964129));
#25096=CARTESIAN_POINT('Ctrl Pts',(32.8301302693401,-1.50048655910789,-27.3903440144575));
#25097=CARTESIAN_POINT('Ctrl Pts',(32.8868306159707,-1.50017097755206,-27.4576734594568));
#25098=CARTESIAN_POINT('Ctrl Pts',(32.938712302257,-1.5,-27.5192120661652));
#25099=CARTESIAN_POINT('Ctrl Pts',(33.,-1.5,-27.5917792275077));
#25100=CARTESIAN_POINT('Ctrl Pts',(33.0955022515476,-1.5,-27.704857831401));
#25101=CARTESIAN_POINT('Ctrl Pts',(33.2417478452125,-1.5,-27.8775886864422));
#25102=CARTESIAN_POINT('Ctrl Pts',(33.3688392456709,-1.5,-28.0268611296802));
#25103=CARTESIAN_POINT('Ctrl Pts',(34.2661932188112,-1.5,-29.0808287430421));
#25104=CARTESIAN_POINT('Ctrl Pts',(35.2319960542962,-1.50000000000001,-30.1809662912266));
#25105=CARTESIAN_POINT('Ctrl Pts',(36.300460733321,-1.50000000000001,-31.2401426718548));
#25106=CARTESIAN_POINT('Ctrl Pts',(36.6891719086917,-1.50000000000001,-31.6254747318857));
#25107=CARTESIAN_POINT('Ctrl Pts',(37.0893059759013,-1.50000000000001,-32.0028866146587));
#25108=CARTESIAN_POINT('Ctrl Pts',(37.5,-1.50000000000001,-32.3652591523689));
#25109=CARTESIAN_POINT('',(37.5,-3.83741678103716,-32.1719479119405));
#25110=CARTESIAN_POINT('Origin',(37.5,0.,0.));
#25111=CARTESIAN_POINT('',(36.8,-4.53355051147318,-31.4347259190859));
#25112=CARTESIAN_POINT('Ctrl Pts',(37.5,-3.83741678103719,-32.1719479119405));
#25113=CARTESIAN_POINT('Ctrl Pts',(37.2470086540957,-4.04454785994588,-31.9226755103028));
#25114=CARTESIAN_POINT('Ctrl Pts',(37.012265903783,-4.27613294009135,-31.6748439028166));
#25115=CARTESIAN_POINT('Ctrl Pts',(36.8,-4.53355051147316,-31.4347259190859));
#25116=CARTESIAN_POINT('',(36.8,-11.7911930472673,-29.4900464626661));
#25117=CARTESIAN_POINT('Ctrl Pts',(36.8,-4.53355051147318,-31.4347259190859));
#25118=CARTESIAN_POINT('Ctrl Pts',(36.8,-6.18280168905534,-31.1968691126063));
#25119=CARTESIAN_POINT('Ctrl Pts',(36.8,-7.81258162569767,-30.8293258095436));
#25120=CARTESIAN_POINT('Ctrl Pts',(36.8,-10.2137688485759,-30.0846548283827));
#25121=CARTESIAN_POINT('Ctrl Pts',(36.8,-11.0089139056503,-29.8028301128151));
#25122=CARTESIAN_POINT('Ctrl Pts',(36.8,-11.7911930472673,-29.4900464626661));
#25123=CARTESIAN_POINT('',(37.5,-12.7626735386834,-29.7804325714888));
#25124=CARTESIAN_POINT('Ctrl Pts',(36.8,-11.7911930472673,-29.4900464626661));
#25125=CARTESIAN_POINT('Ctrl Pts',(37.0122659037829,-12.1341821953297,-29.5692859507915));
#25126=CARTESIAN_POINT('Ctrl Pts',(37.2470086540956,-12.4586565616162,-29.6681218786625));
#25127=CARTESIAN_POINT('Ctrl Pts',(37.5,-12.7626735386834,-29.7804325714888));
#25128=CARTESIAN_POINT('',(37.5,-14.8835914705078,-28.7791366260183));
#25129=CARTESIAN_POINT('Origin',(37.5,0.,0.));
#25130=CARTESIAN_POINT('',(6.9,3.76156693666918,-10.3676856018661));
#25131=CARTESIAN_POINT('Ctrl Pts',(37.5,-14.8835914705078,-28.7791366260183));
#25132=CARTESIAN_POINT('Ctrl Pts',(36.649069632135,-14.5081857198463,-28.128914792419));
#25133=CARTESIAN_POINT('Ctrl Pts',(35.8406537800833,-14.099345992819,-27.4207836130551));
#25134=CARTESIAN_POINT('Ctrl Pts',(35.0774452370464,-13.6847944140629,-26.7027592162917));
#25135=CARTESIAN_POINT('Ctrl Pts',(34.695840965528,-13.4775186246849,-26.34374701791));
#25136=CARTESIAN_POINT('Ctrl Pts',(34.3255255041519,-13.2688250041304,-25.9822790638941));
#25137=CARTESIAN_POINT('Ctrl Pts',(33.9666810635124,-13.0622496974039,-25.6244801370547));
#25138=CARTESIAN_POINT('Ctrl Pts',(33.7186145566387,-12.9194457162284,-25.3771363861357));
#25139=CARTESIAN_POINT('Ctrl Pts',(33.4671024168778,-12.7724011202845,-25.1224476749824));
#25140=CARTESIAN_POINT('Ctrl Pts',(33.2400985609596,-12.6386646513062,-24.8908093158872));
#25141=CARTESIAN_POINT('Ctrl Pts',(33.1387264796076,-12.578942563511,-24.7873676254918));
#25142=CARTESIAN_POINT('Ctrl Pts',(33.0532004124016,-12.5283472490856,-24.699733970282));
#25143=CARTESIAN_POINT('Ctrl Pts',(33.,-12.4968515080772,-24.6451817466334));
#25144=CARTESIAN_POINT('Ctrl Pts',(32.9185691496442,-12.448642765755,-24.5616817555624));
#25145=CARTESIAN_POINT('Ctrl Pts',(32.8516820633331,-12.4091965180072,-24.4928265642786));
#25146=CARTESIAN_POINT('Ctrl Pts',(32.7777321455747,-12.3657029367323,-24.4165289206501));
#25147=CARTESIAN_POINT('Ctrl Pts',(32.1788699540041,-12.0134826477704,-23.79865434472));
#25148=CARTESIAN_POINT('Ctrl Pts',(31.5692879871508,-11.6640598398815,-23.1567007301491));
#25149=CARTESIAN_POINT('Ctrl Pts',(30.9513498040742,-11.3096185478573,-22.5260018679775));
#25150=CARTESIAN_POINT('Ctrl Pts',(30.6423807125359,-11.1323979018452,-22.2106524368916));
#25151=CARTESIAN_POINT('Ctrl Pts',(30.3347880607108,-10.9558507302104,-21.9015729508113));
#25152=CARTESIAN_POINT('Ctrl Pts',(30.0249306371935,-10.7763433330223,-21.5982641082872));
#25153=CARTESIAN_POINT('Ctrl Pts',(29.8700019254348,-10.6865896344282,-21.4466096870251));
#25154=CARTESIAN_POINT('Ctrl Pts',(29.7145097313539,-10.5960927952763,-21.2963965338147));
#25155=CARTESIAN_POINT('Ctrl Pts',(29.5580100720483,-10.5043591957296,-21.1475727378912));
#25156=CARTESIAN_POINT('Ctrl Pts',(29.4797602423956,-10.4584923959562,-21.0731608399294));
#25157=CARTESIAN_POINT('Ctrl Pts',(29.4012586241233,-10.4123158264269,-20.9990965425476));
#25158=CARTESIAN_POINT('Ctrl Pts',(29.3224502420513,-10.365763682914,-20.9253755287763));
#25159=CARTESIAN_POINT('Ctrl Pts',(29.2736528206688,-10.3369390261512,-20.8797281587992));
#25160=CARTESIAN_POINT('Ctrl Pts',(29.224737793838,-10.3079703169171,-20.8342124356888));
#25161=CARTESIAN_POINT('Ctrl Pts',(29.1756921971237,-10.278841304319,-20.7888277158275));
#25162=CARTESIAN_POINT('Ctrl Pts',(29.1455286058255,-10.2609266353214,-20.7609156047963));
#25163=CARTESIAN_POINT('Ctrl Pts',(29.1181490968943,-10.2446403152596,-20.7356566760271));
#25164=CARTESIAN_POINT('Ctrl Pts',(29.0849408699094,-10.2248462834623,-20.7051394327917));
#25165=CARTESIAN_POINT('Ctrl Pts',(29.0475462332377,-10.2025569083726,-20.670775019915));
#25166=CARTESIAN_POINT('Ctrl Pts',(28.9599837409744,-10.1505620077132,-20.5905365514954));
#25167=CARTESIAN_POINT('Ctrl Pts',(28.8924081850374,-10.1107110566468,-20.5290030526021));
#25168=CARTESIAN_POINT('Ctrl Pts',(28.4410807638263,-9.84455228476247,-20.1180296615806));
#25169=CARTESIAN_POINT('Ctrl Pts',(27.9936088570971,-9.59004457975323,-19.7235361020228));
#25170=CARTESIAN_POINT('Ctrl Pts',(27.5122543100131,-9.3139524301101,-19.3231338580698));
#25171=CARTESIAN_POINT('Ctrl Pts',(27.1397294109546,-9.10028206841989,-19.0132587225486));
#25172=CARTESIAN_POINT('Ctrl Pts',(26.727634164301,-8.86410488405222,-18.6830630722578));
#25173=CARTESIAN_POINT('Ctrl Pts',(26.2530417505368,-8.57522710561968,-18.3335669465969));
#25174=CARTESIAN_POINT('Ctrl Pts',(25.8694949138895,-8.34176749926666,-18.0511179871739));
#25175=CARTESIAN_POINT('Ctrl Pts',(25.4447383161208,-8.07732257196432,-17.7540556187476));
#25176=CARTESIAN_POINT('Ctrl Pts',(24.9635886608529,-7.77432947328252,-17.440187687688));
#25177=CARTESIAN_POINT('Ctrl Pts',(24.6119820458988,-7.552913170443,-17.2108244540782));
#25178=CARTESIAN_POINT('Ctrl Pts',(24.287362678484,-7.34685978853744,-17.0017823418141));
#25179=CARTESIAN_POINT('Ctrl Pts',(23.6426616415357,-6.93898570153371,-16.6259529313418));
#25180=CARTESIAN_POINT('Ctrl Pts',(23.5760533209921,-6.89684553675724,-16.5871235136617));
#25181=CARTESIAN_POINT('Ctrl Pts',(23.5065967304336,-6.85292160229735,-16.5469475097905));
#25182=CARTESIAN_POINT('Ctrl Pts',(23.4342591639586,-6.80720851268155,-16.5054784159948));
#25183=CARTESIAN_POINT('Ctrl Pts',(22.7443384436271,-6.37121917473222,-16.1099662574134));
#25184=CARTESIAN_POINT('Ctrl Pts',(21.7987837593179,-5.75271743557089,-15.6084067036806));
#25185=CARTESIAN_POINT('Ctrl Pts',(20.5610365528855,-4.96573918168374,-15.0432759423309));
#25186=CARTESIAN_POINT('Ctrl Pts',(19.7234582214113,-4.43319430549925,-14.6608543317661));
#25187=CARTESIAN_POINT('Ctrl Pts',(18.7603809281633,-3.80221290992216,-14.2617573685881));
#25188=CARTESIAN_POINT('Ctrl Pts',(17.6514222906382,-3.10236545497629,-13.8414640697512));
#25189=CARTESIAN_POINT('Ctrl Pts',(16.7565277906389,-2.53761072285453,-13.5023006881889));
#25190=CARTESIAN_POINT('Ctrl Pts',(15.7613807992389,-1.89253400855811,-13.1550491146656));
#25191=CARTESIAN_POINT('Ctrl Pts',(14.7199652846762,-1.24173803388781,-12.8103195459473));
#25192=CARTESIAN_POINT('Ctrl Pts',(13.7316067501733,-0.624098151639956,
-12.4831529092169));
#25193=CARTESIAN_POINT('Ctrl Pts',(12.7260968661244,0.0230322824212332,
-12.1691790146817));
#25194=CARTESIAN_POINT('Ctrl Pts',(11.7781012037546,0.61550573962622,-11.8786003909685));
#25195=CARTESIAN_POINT('Ctrl Pts',(10.6475718363526,1.3220581737398,-11.5320717298292));
#25196=CARTESIAN_POINT('Ctrl Pts',(9.62260863652895,1.9899080550587,-11.2216623289213));
#25197=CARTESIAN_POINT('Ctrl Pts',(8.83596460437641,2.49396550450873,-10.9799836949691));
#25198=CARTESIAN_POINT('Ctrl Pts',(8.38131550044784,2.78529075246604,-10.840303013652));
#25199=CARTESIAN_POINT('Ctrl Pts',(7.99969688490338,3.03233135775506,-10.721713754924));
#25200=CARTESIAN_POINT('Ctrl Pts',(7.59379043301429,3.2996126212042,-10.5924279410164));
#25201=CARTESIAN_POINT('Ctrl Pts',(7.36145773430761,3.45259904692339,-10.5184273383902));
#25202=CARTESIAN_POINT('Ctrl Pts',(7.13004605045626,3.60654870801841,-10.4436236908384));
#25203=CARTESIAN_POINT('Ctrl Pts',(6.9,3.76156693666918,-10.3676856018661));
#25204=CARTESIAN_POINT('',(6.9,0.168526548660245,-11.02768739857));
#25205=CARTESIAN_POINT('Ctrl Pts',(6.90000000000001,3.76156693666918,-10.3676856018661));
#25206=CARTESIAN_POINT('Ctrl Pts',(6.90000000000001,3.24481773355662,-10.5551707158657));
#25207=CARTESIAN_POINT('Ctrl Pts',(6.90000000000001,2.71398840242747,-10.7040448708755));
#25208=CARTESIAN_POINT('Ctrl Pts',(6.90000000000001,1.51153848953113,-10.9457448952802));
#25209=CARTESIAN_POINT('Ctrl Pts',(6.90000000000001,0.840414370027659,-11.0174195217678));
#25210=CARTESIAN_POINT('Ctrl Pts',(6.90000000000001,0.168526548660246,-11.02768739857));
#25211=CARTESIAN_POINT('',(37.5,-17.4816676818611,-27.2791366260183));
#25212=CARTESIAN_POINT('Ctrl Pts',(6.9,0.168526548660245,-11.02768739857));
#25213=CARTESIAN_POINT('Ctrl Pts',(6.98893730997555,0.109835775321892,-11.0357428000776));
#25214=CARTESIAN_POINT('Ctrl Pts',(7.08052892388239,0.0497243602609525,
-11.0440392866244));
#25215=CARTESIAN_POINT('Ctrl Pts',(7.17490192378011,-0.01186311602662,-11.0526088775152));
#25216=CARTESIAN_POINT('Ctrl Pts',(7.97363347619349,-0.533112420358449,
-11.1251381246856));
#25217=CARTESIAN_POINT('Ctrl Pts',(8.96286060499838,-1.17518961593372,-11.2096216302935));
#25218=CARTESIAN_POINT('Ctrl Pts',(10.2403127965964,-1.93497024136951,-11.3564324284624));
#25219=CARTESIAN_POINT('Ctrl Pts',(10.4394276407766,-2.05339627863323,-11.3793156403694));
#25220=CARTESIAN_POINT('Ctrl Pts',(10.644938676084,-2.17568840229354,-11.4036121640908));
#25221=CARTESIAN_POINT('Ctrl Pts',(10.85722702267,-2.30180801495081,-11.4296460138921));
#25222=CARTESIAN_POINT('Ctrl Pts',(11.0079272575846,-2.39133838984157,-11.4481270437926));
#25223=CARTESIAN_POINT('Ctrl Pts',(11.2445718661462,-2.53195192937604,-11.4774498561298));
#25224=CARTESIAN_POINT('Ctrl Pts',(11.5512244263538,-2.71302722014986,-11.5182347543375));
#25225=CARTESIAN_POINT('Ctrl Pts',(12.0044642693653,-2.98066084534451,-11.5785158126414));
#25226=CARTESIAN_POINT('Ctrl Pts',(12.6082461582541,-3.33560449465634,-11.663066268173));
#25227=CARTESIAN_POINT('Ctrl Pts',(13.3027146141536,-3.73133446864291,-11.7808809827897));
#25228=CARTESIAN_POINT('Ctrl Pts',(14.2466220417942,-4.26920261601918,-11.9410123512736));
#25229=CARTESIAN_POINT('Ctrl Pts',(15.3788107202222,-4.92664534659587,-12.1625996834269));
#25230=CARTESIAN_POINT('Ctrl Pts',(16.3720853361384,-5.48881820879722,-12.4089023460099));
#25231=CARTESIAN_POINT('Ctrl Pts',(17.5300464833481,-6.14420023710404,-12.6960423867954));
#25232=CARTESIAN_POINT('Ctrl Pts',(18.552257121746,-6.74248287738884,-13.0002012582105));
#25233=CARTESIAN_POINT('Ctrl Pts',(19.459740928474,-7.26206394073252,-13.3207494833101));
#25234=CARTESIAN_POINT('Ctrl Pts',(20.7212139011751,-7.98432197297066,-13.7663364121484));
#25235=CARTESIAN_POINT('Ctrl Pts',(21.7483180914788,-8.5941730292673,-14.2134327155993));
#25236=CARTESIAN_POINT('Ctrl Pts',(22.5801692622301,-9.0770824783983,-14.6264461342272));
#25237=CARTESIAN_POINT('Ctrl Pts',(23.3330995248265,-9.51417645762082,-15.0002753871962));
#25238=CARTESIAN_POINT('Ctrl Pts',(23.9217876541561,-9.86132841201693,-15.330082409639));
#25239=CARTESIAN_POINT('Ctrl Pts',(24.4822919861918,-10.1904384387857,-15.6683207382559));
#25240=CARTESIAN_POINT('Ctrl Pts',(24.9418792867968,-10.4602932466073,-15.9456603260617));
#25241=CARTESIAN_POINT('Ctrl Pts',(25.3626276505146,-10.7067050299032,-16.2195872238973));
#25242=CARTESIAN_POINT('Ctrl Pts',(25.7525302890144,-10.9324873590558,-16.489196921628));
#25243=CARTESIAN_POINT('Ctrl Pts',(26.177608005596,-11.1786386477211,-16.7831294662259));
#25244=CARTESIAN_POINT('Ctrl Pts',(26.5661459571043,-11.3970084746838,-17.0742513036714));
#25245=CARTESIAN_POINT('Ctrl Pts',(26.926701683073,-11.5990258161967,-17.3573257272902));
#25246=CARTESIAN_POINT('Ctrl Pts',(27.1778777841921,-11.7397583702653,-17.5545255633491));
#25247=CARTESIAN_POINT('Ctrl Pts',(27.4154861118762,-11.872403510414,-17.7479949477845));
#25248=CARTESIAN_POINT('Ctrl Pts',(27.6422281941509,-11.9995747619455,-17.9373508256236));
#25249=CARTESIAN_POINT('Ctrl Pts',(27.8555559932678,-12.1192224379658,-18.1155042246928));
#25250=CARTESIAN_POINT('Ctrl Pts',(28.1190837192525,-12.2669482012627,-18.339603886119));
#25251=CARTESIAN_POINT('Ctrl Pts',(28.4603051775732,-12.4627212415744,-18.6410459171623));
#25252=CARTESIAN_POINT('Ctrl Pts',(28.6017730832424,-12.5438873034501,-18.7660215650076));
#25253=CARTESIAN_POINT('Ctrl Pts',(28.7540286646392,-12.631951343169,-18.9021161663187));
#25254=CARTESIAN_POINT('Ctrl Pts',(28.9157341130969,-12.7269375546994,-19.0484400367167));
#25255=CARTESIAN_POINT('Ctrl Pts',(29.4787137469345,-13.0576332925187,-19.557868505355));
#25256=CARTESIAN_POINT('Ctrl Pts',(30.1711677436418,-13.4573416990331,-20.2292610528701));
#25257=CARTESIAN_POINT('Ctrl Pts',(30.8055547543756,-13.8222365906036,-20.874000952648));
#25258=CARTESIAN_POINT('Ctrl Pts',(31.189312564443,-14.0429713504971,-21.2640215044806));
#25259=CARTESIAN_POINT('Ctrl Pts',(31.5650207099043,-14.2588547919394,-21.6546118380272));
#25260=CARTESIAN_POINT('Ctrl Pts',(31.9311744366537,-14.4706295271139,-22.0362125836316));
#25261=CARTESIAN_POINT('Ctrl Pts',(32.1142513000284,-14.5765168947012,-22.2270129564337));
#25262=CARTESIAN_POINT('Ctrl Pts',(32.2949430642625,-14.68138076651,-22.4155611447466));
#25263=CARTESIAN_POINT('Ctrl Pts',(32.4730466959737,-14.7853297275566,-22.6006686536314));
#25264=CARTESIAN_POINT('Ctrl Pts',(32.5932788659582,-14.8555024075531,-22.7256289212004));
#25265=CARTESIAN_POINT('Ctrl Pts',(32.7123311760599,-14.9252583804577,-22.8490214255682));
#25266=CARTESIAN_POINT('Ctrl Pts',(32.8301302693005,-14.99463148543,-22.9704904553205));
#25267=CARTESIAN_POINT('Ctrl Pts',(32.8868306159448,-15.0280229062934,-23.0289572559047));
#25268=CARTESIAN_POINT('Ctrl Pts',(32.9387123022458,-15.0586441387526,-23.0823367414188));
#25269=CARTESIAN_POINT('Ctrl Pts',(33.,-15.0949277194305,-23.1451817466334));
#25270=CARTESIAN_POINT('Ctrl Pts',(33.0955022515125,-15.1514670213565,-23.2431106901936));
#25271=CARTESIAN_POINT('Ctrl Pts',(33.2417478451615,-15.2378324488677,-23.3926999986605));
#25272=CARTESIAN_POINT('Ctrl Pts',(33.3688392455996,-15.3124686704749,-23.5219737265691));
#25273=CARTESIAN_POINT('Ctrl Pts',(34.2661932188049,-15.8394524771949,-24.4347364545743));
#25274=CARTESIAN_POINT('Ctrl Pts',(35.2319960543609,-16.3895212513289,-25.3874835190315));
#25275=CARTESIAN_POINT('Ctrl Pts',(36.3004607334728,-16.9191094416793,-26.3047571718069));
#25276=CARTESIAN_POINT('Ctrl Pts',(36.6891719087959,-17.1117754716687,-26.638464524641));
#25277=CARTESIAN_POINT('Ctrl Pts',(37.0893059759547,-17.3004814130296,-26.9653128027682));
#25278=CARTESIAN_POINT('Ctrl Pts',(37.5,-17.4816676818611,-27.2791366260183));
#25279=CARTESIAN_POINT('',(37.5,-19.4092743732572,-25.9430157904516));
#25280=CARTESIAN_POINT('Origin',(37.5,0.,0.));
#25281=CARTESIAN_POINT('',(36.8,-19.6435328718186,-24.9564959511929));
#25282=CARTESIAN_POINT('Ctrl Pts',(37.5,-19.4092743732572,-25.9430157904516));
#25283=CARTESIAN_POINT('Ctrl Pts',(37.2470086540957,-19.4640189486865,-25.6235740187167));
#25284=CARTESIAN_POINT('Ctrl Pts',(37.0122659037829,-19.5406617074869,-25.2931530107001));
#25285=CARTESIAN_POINT('Ctrl Pts',(36.8,-19.6435328718186,-24.9564959511929));
#25286=CARTESIAN_POINT('',(36.8,-24.9564959511929,-19.6435328718186));
#25287=CARTESIAN_POINT('Ctrl Pts',(36.8,-19.6435328718186,-24.9564959511929));
#25288=CARTESIAN_POINT('Ctrl Pts',(36.8,-20.2288646216318,-24.4957748831848));
#25289=CARTESIAN_POINT('Ctrl Pts',(36.8,-20.7984186457787,-24.0141222843114));
#25290=CARTESIAN_POINT('Ctrl Pts',(36.8,-22.6602579716864,-22.3234241559746));
#25291=CARTESIAN_POINT('Ctrl Pts',(36.8,-23.8659348286794,-21.029056769996));
#25292=CARTESIAN_POINT('Ctrl Pts',(36.8,-24.9564959511929,-19.6435328718186));
#25293=CARTESIAN_POINT('',(37.5,-25.9430157904517,-19.4092743732571));
#25294=CARTESIAN_POINT('Ctrl Pts',(36.8,-24.9564959511929,-19.6435328718186));
#25295=CARTESIAN_POINT('Ctrl Pts',(37.0122659037829,-25.2931530107001,-19.5406617074869));
#25296=CARTESIAN_POINT('Ctrl Pts',(37.2470086540956,-25.6235740187166,-19.4640189486865));
#25297=CARTESIAN_POINT('Ctrl Pts',(37.5,-25.9430157904516,-19.4092743732572));
#25298=CARTESIAN_POINT('',(37.5,-27.2791366260183,-17.4816676818611));
#25299=CARTESIAN_POINT('Origin',(37.5,0.,0.));
#25300=CARTESIAN_POINT('',(6.9,-1.92623027574191,-10.8594625780008));
#25301=CARTESIAN_POINT('Ctrl Pts',(37.5,-27.2791366260183,-17.4816676818611));
#25302=CARTESIAN_POINT('Ctrl Pts',(36.6490696321363,-26.62891479242,-17.1062619312002));
#25303=CARTESIAN_POINT('Ctrl Pts',(35.840653780086,-25.9207836130574,-16.6974222041736));
#25304=CARTESIAN_POINT('Ctrl Pts',(35.0774452370509,-25.2027592162959,-16.2828706254186));
#25305=CARTESIAN_POINT('Ctrl Pts',(34.6958409655333,-24.8437470179151,-16.0755948360411));
#25306=CARTESIAN_POINT('Ctrl Pts',(34.3255255041583,-24.4822790639003,-15.8669012154872));
#25307=CARTESIAN_POINT('Ctrl Pts',(33.9666810635198,-24.1244801370621,-15.6603259087614));
#25308=CARTESIAN_POINT('Ctrl Pts',(33.7186145566397,-23.8771363861367,-15.5175219275823));
#25309=CARTESIAN_POINT('Ctrl Pts',(33.4671024168716,-23.6224476749761,-15.3704773316342));
#25310=CARTESIAN_POINT('Ctrl Pts',(33.240098560949,-23.3908093158764,-15.2367408626533));
#25311=CARTESIAN_POINT('Ctrl Pts',(33.1387264796047,-23.2873676254888,-15.1770187748626));
#25312=CARTESIAN_POINT('Ctrl Pts',(33.0532004124041,-23.1997339702846,-15.1264234604404));
#25313=CARTESIAN_POINT('Ctrl Pts',(33.,-23.1451817466334,-15.0949277194305));
#25314=CARTESIAN_POINT('Ctrl Pts',(32.9185691495912,-23.0616817555081,-15.0467189770769));
#25315=CARTESIAN_POINT('Ctrl Pts',(32.8516820633262,-22.9930927072798,-15.0068117561438));
#25316=CARTESIAN_POINT('Ctrl Pts',(32.7777321455979,-22.9172773392108,-14.9624828491682));
#25317=CARTESIAN_POINT('Ctrl Pts',(32.178869954022,-22.303308333271,-14.6034979145383));
#25318=CARTESIAN_POINT('Ctrl Pts',(31.5692879871635,-21.6797224976866,-14.2222611802097));
#25319=CARTESIAN_POINT('Ctrl Pts',(30.9513498040836,-21.0574179035543,-13.8532805894412));
#25320=CARTESIAN_POINT('Ctrl Pts',(30.6423807125436,-20.7462656064881,-13.6687902940569));
#25321=CARTESIAN_POINT('Ctrl Pts',(30.3347880607171,-20.4388315278445,-13.4893931931391));
#25322=CARTESIAN_POINT('Ctrl Pts',(30.0249306371985,-20.1317191404489,-13.316473728914));
#25323=CARTESIAN_POINT('Ctrl Pts',(29.8700019254392,-19.9781629467512,-13.2300139968015));
#25324=CARTESIAN_POINT('Ctrl Pts',(29.7145097313576,-19.8246838084775,-13.1451740097143));
#25325=CARTESIAN_POINT('Ctrl Pts',(29.5580100720514,-19.6708282829271,-13.0621556215299));
#25326=CARTESIAN_POINT('Ctrl Pts',(29.4797602423983,-19.5939005201519,-13.0206464274377));
#25327=CARTESIAN_POINT('Ctrl Pts',(29.4012586241258,-19.5168782891887,-12.979593149156));
#25328=CARTESIAN_POINT('Ctrl Pts',(29.3224502420534,-19.4397024434199,-12.9390249501936));
#25329=CARTESIAN_POINT('Ctrl Pts',(29.2736528205548,-19.3919158733057,-12.9139054964992));
#25330=CARTESIAN_POINT('Ctrl Pts',(29.2247377936074,-19.3440703735249,-12.8889720785721));
#25331=CARTESIAN_POINT('Ctrl Pts',(29.1756921967758,-19.2961515485829,-12.8642322644697));
#25332=CARTESIAN_POINT('Ctrl Pts',(29.1455286055936,-19.2666809347284,-12.8490170018014));
#25333=CARTESIAN_POINT('Ctrl Pts',(29.1181490967682,-19.2399471035395,-12.8352852878993));
#25334=CARTESIAN_POINT('Ctrl Pts',(29.0849408699094,-19.2075463476651,-12.8187535959654));
#25335=CARTESIAN_POINT('Ctrl Pts',(29.0475462330809,-19.1710609760116,-12.8001378288948));
#25336=CARTESIAN_POINT('Ctrl Pts',(28.9599837407005,-19.0859128368506,-12.7566467271546));
#25337=CARTESIAN_POINT('Ctrl Pts',(28.8924081846425,-19.0206341513,-12.7232826294034));
#25338=CARTESIAN_POINT('Ctrl Pts',(28.4410807633615,-18.5846471978384,-12.5004486184112));
#25339=CARTESIAN_POINT('Ctrl Pts',(27.9936088565974,-18.1669902800388,-12.2860610266994));
#25340=CARTESIAN_POINT('Ctrl Pts',(27.5122543093923,-17.7276863425835,-12.0773485864914));
#25341=CARTESIAN_POINT('Ctrl Pts',(27.1397294104949,-17.3877048137166,-11.9158240280583));
#25342=CARTESIAN_POINT('Ctrl Pts',(26.7276341640354,-17.0180715472901,-11.7479547989676));
#25343=CARTESIAN_POINT('Ctrl Pts',(26.2530417505368,-16.593147989986,-11.5897211649258));
#25344=CARTESIAN_POINT('Ctrl Pts',(25.8694949138867,-16.2497415604127,-11.4618429939686));
#25345=CARTESIAN_POINT('Ctrl Pts',(25.4447383161154,-15.8721943512516,-11.3368019000536));
#25346=CARTESIAN_POINT('Ctrl Pts',(24.9635886608448,-15.4528606650898,-11.2164808476631));
#25347=CARTESIAN_POINT('Ctrl Pts',(24.6119820459015,-15.1464269052232,-11.1285546120855));
#25348=CARTESIAN_POINT('Ctrl Pts',(24.2873626784964,-14.8634583858341,-11.0505455233595));
#25349=CARTESIAN_POINT('Ctrl Pts',(23.642661641582,-14.3223143597349,-10.9290047499082));
#25350=CARTESIAN_POINT('Ctrl Pts',(23.5760533210243,-14.2664051976669,-10.9164475701686));
#25351=CARTESIAN_POINT('Ctrl Pts',(23.5065967304504,-14.2082779526419,-10.9036160974206));
#25352=CARTESIAN_POINT('Ctrl Pts',(23.4342591639586,-14.1479547088373,-10.8905593535264));
#25353=CARTESIAN_POINT('Ctrl Pts',(22.7443384436266,-13.5726207871028,-10.7660304456639));
#25354=CARTESIAN_POINT('Ctrl Pts',(21.7987837593173,-12.7862027918379,-10.6409180002012));
#25355=CARTESIAN_POINT('Ctrl Pts',(20.5610365528854,-11.8220942510713,-10.544989531356));
#25356=CARTESIAN_POINT('Ctrl Pts',(19.7234582214112,-11.1696860543578,-10.480075139743));
#25357=CARTESIAN_POINT('Ctrl Pts',(18.7603809281633,-10.4236916548837,-10.4499377288461));
#25358=CARTESIAN_POINT('Ctrl Pts',(17.6514222906382,-9.60745933070834,-10.435876782486));
#25359=CARTESIAN_POINT('Ctrl Pts',(16.7565277906389,-8.94878569500228,-10.4245300440805));
#25360=CARTESIAN_POINT('Ctrl Pts',(15.7613807992389,-8.21650708627012,-10.4463397170534));
#25361=CARTESIAN_POINT('Ctrl Pts',(14.7199652846762,-7.48053645516581,-10.4731931404428));
#25362=CARTESIAN_POINT('Ctrl Pts',(13.7316067501733,-6.78206130838354,-10.4986784628874));
#25363=CARTESIAN_POINT('Ctrl Pts',(12.7260968661244,-6.06464296565695,-10.5503343111255));
#25364=CARTESIAN_POINT('Ctrl Pts',(11.7781012037546,-5.40625658879283,-10.5949225697956));
#25365=CARTESIAN_POINT('Ctrl Pts',(10.6475718363526,-4.62109990117505,-10.6480961631663));
#25366=CARTESIAN_POINT('Ctrl Pts',(9.62260863652896,-3.88752023758453,-10.713198677066));
#25367=CARTESIAN_POINT('Ctrl Pts',(8.83596460437642,-3.33015436441791,-10.7559275652365));
#25368=CARTESIAN_POINT('Ctrl Pts',(8.38131550044705,-3.00801895826399,-10.7806231707767));
#25369=CARTESIAN_POINT('Ctrl Pts',(7.99969688490205,-2.734780888953,-10.8014421627468));
#25370=CARTESIAN_POINT('Ctrl Pts',(7.59379043301258,-2.43866561789635,-10.8231179952785));
#25371=CARTESIAN_POINT('Ctrl Pts',(7.36145773430645,-2.26917518547666,-10.8355248063684));
#25372=CARTESIAN_POINT('Ctrl Pts',(7.13004605045568,-2.09844904428886,-10.8477177778403));
#25373=CARTESIAN_POINT('Ctrl Pts',(6.9,-1.9262302757419,-10.8594625780008));
#25374=CARTESIAN_POINT('',(6.9,-5.36789542693312,-9.6345207064853));
#25375=CARTESIAN_POINT('Ctrl Pts',(6.90000000000001,-1.92623027574191,-10.8594625780008));
#25376=CARTESIAN_POINT('Ctrl Pts',(6.90000000000001,-2.35749364924904,-10.7829659225815));
#25377=CARTESIAN_POINT('Ctrl Pts',(6.90000000000001,-2.78469328079872,-10.6806923192591));
#25378=CARTESIAN_POINT('Ctrl Pts',(6.90000000000001,-3.958690010018,-10.3240838050858));
#25379=CARTESIAN_POINT('Ctrl Pts',(6.90000000000001,-4.68344446130229,-10.0158641401962));
#25380=CARTESIAN_POINT('Ctrl Pts',(6.90000000000001,-5.36789542693313,-9.6345207064853));
#25381=CARTESIAN_POINT('',(37.5,-28.7791366260183,-14.8835914705078));
#25382=CARTESIAN_POINT('Ctrl Pts',(6.9,-5.36789542693312,-9.6345207064853));
#25383=CARTESIAN_POINT('Ctrl Pts',(6.98893730997566,-5.42275082836576,-9.61215150215935));
#25384=CARTESIAN_POINT('Ctrl Pts',(7.08052892388251,-5.47895708413934,-9.58928076274051));
#25385=CARTESIAN_POINT('Ctrl Pts',(7.17490192378012,-5.5365781986047,-9.56590850800827));
#25386=CARTESIAN_POINT('Ctrl Pts',(7.97363347620185,-6.02425796145133,-9.36809602640721));
#25387=CARTESIAN_POINT('Ctrl Pts',(8.9628606050108,-6.62255487681613,-9.12022229067638));
#25388=CARTESIAN_POINT('Ctrl Pts',(10.2403127965964,-7.35394959882411,-8.86747385872511));
#25389=CARTESIAN_POINT('Ctrl Pts',(10.4394276407787,-7.46795116151874,-8.82807828292446));
#25390=CARTESIAN_POINT('Ctrl Pts',(10.6449386760882,-7.58600750915316,-8.78797362786027));
#25391=CARTESIAN_POINT('Ctrl Pts',(10.8572270226761,-7.70824722253153,-8.74745979681753));
#25392=CARTESIAN_POINT('Ctrl Pts',(11.0079272576205,-7.7950233165647,-8.71869965074842));
#25393=CARTESIAN_POINT('Ctrl Pts',(11.2445718661789,-7.93145962008442,-8.67378718137609));
#25394=CARTESIAN_POINT('Ctrl Pts',(11.5512244264302,-8.10866787102136,-8.61857029392041));
#25395=CARTESIAN_POINT('Ctrl Pts',(12.004464269425,-8.37058591848924,-8.5369584091849));
#25396=CARTESIAN_POINT('Ctrl Pts',(12.6082461582835,-8.72025136345347,-8.43270942692696));
#25397=CARTESIAN_POINT('Ctrl Pts',(13.3027146141536,-9.12187093125612,-8.33687497573541));
#25398=CARTESIAN_POINT('Ctrl Pts',(14.2466220417731,-9.66774409500015,-8.20661873509998));
#25399=CARTESIAN_POINT('Ctrl Pts',(15.3788107202044,-10.3478998672909,-8.06979762861151));
#25400=CARTESIAN_POINT('Ctrl Pts',(16.3720853361384,-10.9579071785779,-8.00201556032625));
#25401=CARTESIAN_POINT('Ctrl Pts',(17.5300464833461,-11.6690546846669,-7.92299511593695));
#25402=CARTESIAN_POINT('Ctrl Pts',(18.5522571217463,-12.3392620855058,-7.88726310522631));
#25403=CARTESIAN_POINT('Ctrl Pts',(19.459740928474,-12.9495065982363,-7.9050754796287));
#25404=CARTESIAN_POINT('Ctrl Pts',(20.7212139011916,-13.7977938666722,-7.92983606347819));
#25405=CARTESIAN_POINT('Ctrl Pts',(21.7483180915005,-14.5494885256804,-8.01210729205923));
#25406=CARTESIAN_POINT('Ctrl Pts',(22.5801692622301,-15.1742070856531,-8.12833268012627));
#25407=CARTESIAN_POINT('Ctrl Pts',(23.3330995247701,-15.7396562019433,-8.23353132025611));
#25408=CARTESIAN_POINT('Ctrl Pts',(23.9217876540031,-16.2052021245672,-8.34557660281974));
#25409=CARTESIAN_POINT('Ctrl Pts',(24.4822919859706,-16.6593389326385,-8.47394457452865));
#25410=CARTESIAN_POINT('Ctrl Pts',(24.9418792866585,-17.0317098455124,-8.57920029914614));
#25411=CARTESIAN_POINT('Ctrl Pts',(25.3626276504486,-17.3820721586154,-8.69322205982058));
#25412=CARTESIAN_POINT('Ctrl Pts',(25.7525302890143,-17.7124102403086,-8.81381974260611));
#25413=CARTESIAN_POINT('Ctrl Pts',(26.1776080055599,-18.0725497817353,-8.94529714888304));
#25414=CARTESIAN_POINT('Ctrl Pts',(26.5661459570434,-18.4072245180059,-9.08823114221459));
#25415=CARTESIAN_POINT('Ctrl Pts',(26.9267016829969,-18.7237138795562,-9.23237211346577));
#25416=CARTESIAN_POINT('Ctrl Pts',(27.1778777840957,-18.94419176453,-9.33278590407112));
#25417=CARTESIAN_POINT('Ctrl Pts',(27.4154861117651,-19.1558005177911,-9.43401273576453));
#25418=CARTESIAN_POINT('Ctrl Pts',(27.6422281940302,-19.3606119911582,-9.5344141105576));
#25419=CARTESIAN_POINT('Ctrl Pts',(27.8555559931903,-19.5533066176682,-9.62887564192972));
#25420=CARTESIAN_POINT('Ctrl Pts',(28.1190837191777,-19.7932907121909,-9.74908876005587));
#25421=CARTESIAN_POINT('Ctrl Pts',(28.4603051775583,-20.1135561540545,-9.91225869658039));
#25422=CARTESIAN_POINT('Ctrl Pts',(28.6017730832314,-20.2463358494903,-9.97990775153286));
#25423=CARTESIAN_POINT('Ctrl Pts',(28.7540286646333,-20.3906488457069,-10.0537371137291));
#25424=CARTESIAN_POINT('Ctrl Pts',(28.9157341130969,-20.5460712531062,-10.1329641969115));
#25425=CARTESIAN_POINT('Ctrl Pts',(29.4787137469313,-21.0871763972971,-10.4087943232522));
#25426=CARTESIAN_POINT('Ctrl Pts',(30.171167743637,-21.7690303052006,-10.7903831220533));
#25427=CARTESIAN_POINT('Ctrl Pts',(30.8055547543696,-22.4074085008994,-11.1662968083083));
#25428=CARTESIAN_POINT('Ctrl Pts',(31.1893125644379,-22.7935806863826,-11.3936971342472));
#25429=CARTESIAN_POINT('Ctrl Pts',(31.5650207099002,-23.1758363977024,-11.6240165648506));
#25430=CARTESIAN_POINT('Ctrl Pts',(31.9311744366506,-23.5500390710465,-11.8486051370604));
#25431=CARTESIAN_POINT('Ctrl Pts',(32.1142513000258,-23.7371404077185,-11.9608994231653));
#25432=CARTESIAN_POINT('Ctrl Pts',(32.2949430642605,-23.9222292788011,-12.0717550081777));
#25433=CARTESIAN_POINT('Ctrl Pts',(32.4730466959721,-24.1048054742075,-12.1800883327802));
#25434=CARTESIAN_POINT('Ctrl Pts',(32.593278865964,-24.2280569315281,-12.253220758965));
#25435=CARTESIAN_POINT('Ctrl Pts',(32.712331176073,-24.3501636283205,-12.3252038159361));
#25436=CARTESIAN_POINT('Ctrl Pts',(32.8301302693206,-24.4709770144493,-12.3957125289926));
#25437=CARTESIAN_POINT('Ctrl Pts',(32.8868306159582,-24.5291282334706,-12.4296505531408));
#25438=CARTESIAN_POINT('Ctrl Pts',(32.9387123022532,-24.5823367414265,-12.4605679274037));
#25439=CARTESIAN_POINT('Ctrl Pts',(33.,-24.6451817466334,-12.4968515080772));
#25440=CARTESIAN_POINT('Ctrl Pts',(33.0955022515533,-24.7431106902355,-12.5533908100273));
#25441=CARTESIAN_POINT('Ctrl Pts',(33.2417478451922,-24.8926999986918,-12.6397562375324));
#25442=CARTESIAN_POINT('Ctrl Pts',(33.3688392456331,-25.0219737266032,-12.7143924591412));
#25443=CARTESIAN_POINT('Ctrl Pts',(34.266193218824,-25.934736454593,-13.2413762658524));
#25444=CARTESIAN_POINT('Ctrl Pts',(35.231996054366,-26.8874835190347,-13.7914450399775));
#25445=CARTESIAN_POINT('Ctrl Pts',(36.3004607334594,-27.8047571717954,-14.3210332303193));
#25446=CARTESIAN_POINT('Ctrl Pts',(36.6891719087867,-28.1384645246335,-14.513699260311));
#25447=CARTESIAN_POINT('Ctrl Pts',(37.08930597595,-28.4653128027646,-14.7024052016742));
#25448=CARTESIAN_POINT('Ctrl Pts',(37.5,-28.7791366260183,-14.8835914705078));
#25449=CARTESIAN_POINT('',(37.5,-29.7804325714888,-12.7626735386834));
#25450=CARTESIAN_POINT('Origin',(37.5,0.,0.));
#25451=CARTESIAN_POINT('',(36.8,-29.4900464626661,-11.7911930472673));
#25452=CARTESIAN_POINT('Ctrl Pts',(37.5,-29.7804325714888,-12.7626735386834));
#25453=CARTESIAN_POINT('Ctrl Pts',(37.2470086540956,-29.6681218786625,-12.4586565616162));
#25454=CARTESIAN_POINT('Ctrl Pts',(37.0122659037829,-29.5692859507915,-12.1341821953297));
#25455=CARTESIAN_POINT('Ctrl Pts',(36.8,-29.4900464626661,-11.7911930472673));
#25456=CARTESIAN_POINT('',(36.8,-31.4347259190859,-4.53355051147314));
#25457=CARTESIAN_POINT('Ctrl Pts',(36.8,-29.4900464626661,-11.7911930472673));
#25458=CARTESIAN_POINT('Ctrl Pts',(36.8,-30.4236973716148,-9.45611053488413));
#25459=CARTESIAN_POINT('Ctrl Pts',(36.8,-31.0761743714062,-7.01967470941752));
#25460=CARTESIAN_POINT('Ctrl Pts',(36.8,-31.4347259190859,-4.53355051147314));
#25461=CARTESIAN_POINT('',(37.5,-32.1719479119405,-3.83741678103714));
#25462=CARTESIAN_POINT('Ctrl Pts',(36.8,-31.4347259190859,-4.53355051147314));
#25463=CARTESIAN_POINT('Ctrl Pts',(37.0122659037829,-31.6748439028166,-4.27613294009137));
#25464=CARTESIAN_POINT('Ctrl Pts',(37.2470086540956,-31.9226755103028,-4.04454785994591));
#25465=CARTESIAN_POINT('Ctrl Pts',(37.5,-32.1719479119405,-3.83741678103716));
#25466=CARTESIAN_POINT('',(37.5,-32.3652591523689,-1.5));
#25467=CARTESIAN_POINT('Origin',(37.5,0.,0.));
#25468=CARTESIAN_POINT('',(6.9,-7.09789564133157,-8.44145532612415));
#25469=CARTESIAN_POINT('Ctrl Pts',(37.5,-32.3652591523689,-1.5));
#25470=CARTESIAN_POINT('Ctrl Pts',(36.6490696321457,-31.6144476510553,-1.5));
#25471=CARTESIAN_POINT('Ctrl Pts',(35.8406537801031,-30.7967681970114,-1.49999999999999));
#25472=CARTESIAN_POINT('Ctrl Pts',(35.0774452370724,-29.9676650395074,-1.49999999999999));
#25473=CARTESIAN_POINT('Ctrl Pts',(34.6958409655571,-29.5531134607554,-1.49999999999999));
#25474=CARTESIAN_POINT('Ctrl Pts',(34.3255255041835,-29.1357262196498,-1.5));
#25475=CARTESIAN_POINT('Ctrl Pts',(33.9666810635455,-28.7225756061991,-1.5));
#25476=CARTESIAN_POINT('Ctrl Pts',(33.7186145566592,-28.4369676438341,-1.5));
#25477=CARTESIAN_POINT('Ctrl Pts',(33.4671024168883,-28.1428784519347,-1.5));
#25478=CARTESIAN_POINT('Ctrl Pts',(33.2400985609549,-27.8754055139602,-1.5));
#25479=CARTESIAN_POINT('Ctrl Pts',(33.1387264796142,-27.7559613383832,-1.5));
#25480=CARTESIAN_POINT('Ctrl Pts',(33.0532004124121,-27.6547707095369,-1.5));
#25481=CARTESIAN_POINT('Ctrl Pts',(33.,-27.5917792275077,-1.5));
#25482=CARTESIAN_POINT('Ctrl Pts',(32.9185691495509,-27.4953617427528,-1.5));
#25483=CARTESIAN_POINT('Ctrl Pts',(32.8516820632998,-27.4160082741156,-1.49973385699148));
#25484=CARTESIAN_POINT('Ctrl Pts',(32.7777321455762,-27.3281857858883,-1.49925158146312));
#25485=CARTESIAN_POINT('Ctrl Pts',(32.1788699540068,-26.6169805623009,-1.49534601146731));
#25486=CARTESIAN_POINT('Ctrl Pts',(31.5692879871545,-25.8863210200878,-1.47697823247537));
#25487=CARTESIAN_POINT('Ctrl Pts',(30.9513498040757,-25.1628991372947,-1.46858396443267));
#25488=CARTESIAN_POINT('Ctrl Pts',(30.6423807125364,-24.8011881958981,-1.46438683041132));
#25489=CARTESIAN_POINT('Ctrl Pts',(30.3347880607112,-24.4452439233464,-1.46274142297315));
#25490=CARTESIAN_POINT('Ctrl Pts',(30.024930637194,-24.0928170619341,-1.46654496784322));
#25491=CARTESIAN_POINT('Ctrl Pts',(29.8700019254354,-23.916603631228,-1.46844674027826));
#25492=CARTESIAN_POINT('Ctrl Pts',(29.7145097313546,-23.7412668049894,-1.47171272534086));
#25493=CARTESIAN_POINT('Ctrl Pts',(29.5580100720492,-23.5665148172587,-1.47674445496711));
#25494=CARTESIAN_POINT('Ctrl Pts',(29.4797602423965,-23.4791388233934,-1.47926031978023));
#25495=CARTESIAN_POINT('Ctrl Pts',(29.4012586241243,-23.3919089755827,-1.4822182533613));
#25496=CARTESIAN_POINT('Ctrl Pts',(29.3224502420522,-23.3047886331076,-1.48567308535849));
#25497=CARTESIAN_POINT('Ctrl Pts',(29.2736528206287,-23.2508445226647,-1.48781228538369));
#25498=CARTESIAN_POINT('Ctrl Pts',(29.2247377937566,-23.196942395517,-1.49014206194219));
#25499=CARTESIAN_POINT('Ctrl Pts',(29.1756921970008,-23.1430735688292,-1.49267616691107));
#25500=CARTESIAN_POINT('Ctrl Pts',(29.1455286057438,-23.1099436371495,-1.49423466984589));
#25501=CARTESIAN_POINT('Ctrl Pts',(29.1181490968576,-23.0799256031815,-1.49570957236661));
#25502=CARTESIAN_POINT('Ctrl Pts',(29.0849408699095,-23.0435998794277,-1.49759308512661));
#25503=CARTESIAN_POINT('Ctrl Pts',(29.04754623316,-23.0026947372604,-1.49971404375482));
#25504=CARTESIAN_POINT('Ctrl Pts',(28.9599837408029,-22.9072087348169,-1.50462371438851));
#25505=CARTESIAN_POINT('Ctrl Pts',(28.892408184771,-22.8339936859565,-1.50836890093551));
#25506=CARTESIAN_POINT('Ctrl Pts',(28.4410807635607,-22.3450009031177,-1.53338246331615));
#25507=CARTESIAN_POINT('Ctrl Pts',(27.9936088568423,-21.876105606424,-1.55654582153512));
#25508=CARTESIAN_POINT('Ctrl Pts',(27.5122543097379,-21.3913010165935,-1.595447514942));
#25509=CARTESIAN_POINT('Ctrl Pts',(27.1397294107505,-21.0161060964632,-1.62555390843929));
#25510=CARTESIAN_POINT('Ctrl Pts',(26.727634164183,-20.6120596829972,-1.66499152474874));
#25511=CARTESIAN_POINT('Ctrl Pts',(26.2530417505368,-20.1649482705455,-1.74041895661093));
#25512=CARTESIAN_POINT('Ctrl Pts',(25.8694949138871,-19.8036104932339,-1.80137642675904));
#25513=CARTESIAN_POINT('Ctrl Pts',(25.444738316116,-19.4141244720151,-1.88186126749218));
#25514=CARTESIAN_POINT('Ctrl Pts',(24.9635886608454,-18.9908103209411,-1.98732702259288));
#25515=CARTESIAN_POINT('Ctrl Pts',(24.61198204591,-18.6814677825376,-2.06439754885504));
#25516=CARTESIAN_POINT('Ctrl Pts',(24.2873626785129,-18.3974053119194,-2.13832395598498));
#25517=CARTESIAN_POINT('Ctrl Pts',(23.6426616416205,-17.8679904515028,-2.30363857162399));
#25518=CARTESIAN_POINT('Ctrl Pts',(23.5760533210511,-17.813293106968,-2.32071831600655));
#25519=CARTESIAN_POINT('Ctrl Pts',(23.5065967304643,-17.7565376997399,-2.33866955715462));
#25520=CARTESIAN_POINT('Ctrl Pts',(23.4342591639586,-17.697767866208,-2.35752370715749));
#25521=CARTESIAN_POINT('Ctrl Pts',(22.7443384436261,-17.1372496203954,-2.53734547031035));
#25522=CARTESIAN_POINT('Ctrl Pts',(21.7987837593168,-16.3936354357714,-2.82220391184259));
#25523=CARTESIAN_POINT('Ctrl Pts',(20.5610365528854,-15.5107287130397,-3.2211816912596));
#25524=CARTESIAN_POINT('Ctrl Pts',(19.7234582214111,-14.913269445242,-3.49116827740827));
#25525=CARTESIAN_POINT('Ctrl Pts',(18.7603809281631,-14.2521506387681,-3.83806571370439));
#25526=CARTESIAN_POINT('Ctrl Pts',(17.6514222906382,-13.5382422374622,-4.23400473904287));
#25527=CARTESIAN_POINT('Ctrl Pts',(16.7565277906389,-12.962140766935,-4.55351499318666));
#25528=CARTESIAN_POINT('Ctrl Pts',(15.7613807992389,-12.3388737256115,-4.93854202839547));
#25529=CARTESIAN_POINT('Ctrl Pts',(14.7199652846762,-11.7149311743306,-5.32978309078144));
#25530=CARTESIAN_POINT('Ctrl Pts',(13.7316067501733,-11.1227766145274,-5.70109160083331));
#25531=CARTESIAN_POINT('Ctrl Pts',(12.7260968661244,-10.5273020287043,-6.1045360490248));
#25532=CARTESIAN_POINT('Ctrl Pts',(11.7781012037546,-9.97941683016941,-6.47234380217571));
#25533=CARTESIAN_POINT('Ctrl Pts',(10.6475718363527,-9.32603798942654,-6.91097182865409));
#25534=CARTESIAN_POINT('Ctrl Pts',(9.62260863652901,-8.72329062200737,-7.33414209133674));
#25535=CARTESIAN_POINT('Ctrl Pts',(8.83596460437641,-8.26196206072778,-7.64982933055117));
#25536=CARTESIAN_POINT('Ctrl Pts',(8.381315500447,-7.99533241831015,-7.83228405538782));
#25537=CARTESIAN_POINT('Ctrl Pts',(7.99969688490193,-7.76911080499082,-7.98693286597062));
#25538=CARTESIAN_POINT('Ctrl Pts',(7.5937904330124,-7.52350537407305,-8.15376232311957));
#25539=CARTESIAN_POINT('Ctrl Pts',(7.36145773430633,-7.3829257594442,-8.24925215291324));
#25540=CARTESIAN_POINT('Ctrl Pts',(7.13004605045563,-7.24116906982142,-8.34517464654933));
#25541=CARTESIAN_POINT('Ctrl Pts',(6.9,-7.09789564133157,-8.44145532612415));
#25542=CARTESIAN_POINT('',(6.9,-9.46599415782505,-5.6597919716369));
#25543=CARTESIAN_POINT('Ctrl Pts',(6.90000000000001,-7.09789564133157,-8.44145532612415));
#25544=CARTESIAN_POINT('Ctrl Pts',(6.90000000000001,-7.5077690000137,-8.09681826844945));
#25545=CARTESIAN_POINT('Ctrl Pts',(6.89999999999998,-7.89280389060837,-7.72210951819363));
#25546=CARTESIAN_POINT('Ctrl Pts',(6.89999999999998,-8.70687723936702,-6.80464666682922));
#25547=CARTESIAN_POINT('Ctrl Pts',(6.90000000000001,-9.11389129061078,-6.24868352466685));
#25548=CARTESIAN_POINT('Ctrl Pts',(6.90000000000001,-9.46599415782505,-5.6597919716369));
#25549=CARTESIAN_POINT('',(37.5,-32.3652591523689,1.50000000000001));
#25550=CARTESIAN_POINT('Ctrl Pts',(6.9,-9.46599415782505,-5.6597919716369));
#25551=CARTESIAN_POINT('Ctrl Pts',(6.98893730997541,-9.50231572683743,-5.61299197171201));
#25552=CARTESIAN_POINT('Ctrl Pts',(7.08052892388224,-9.53955640247953,-5.56508220248518));
#25553=CARTESIAN_POINT('Ctrl Pts',(7.17490192378012,-9.57777162403489,-5.51603067891051));
#25554=CARTESIAN_POINT('Ctrl Pts',(7.97363347618197,-9.90120844676305,-5.10088016324537));
#25555=CARTESIAN_POINT('Ctrl Pts',(8.96286060498076,-10.2954119066056,-4.58706675349253));
#25556=CARTESIAN_POINT('Ctrl Pts',(10.2403127965964,-10.8024441000946,-4.00248282963831));
#25557=CARTESIAN_POINT('Ctrl Pts',(10.4394276407756,-10.8814745615577,-3.91136447885237));
#25558=CARTESIAN_POINT('Ctrl Pts',(10.6449386760823,-10.9636620301539,-3.8176046549408));
#25559=CARTESIAN_POINT('Ctrl Pts',(10.857227022668,-11.0492678117687,-3.72139879136494));
#25560=CARTESIAN_POINT('Ctrl Pts',(11.0079272575414,-11.1100380405794,-3.65310372726809));
#25561=CARTESIAN_POINT('Ctrl Pts',(11.244571866109,-11.2057391107435,-3.54599023608119));
#25562=CARTESIAN_POINT('Ctrl Pts',(11.5512244262558,-11.3315975140438,-3.40956688340392));
#25563=CARTESIAN_POINT('Ctrl Pts',(12.0044642692893,-11.5176192545079,-3.20792989421993));
#25564=CARTESIAN_POINT('Ctrl Pts',(12.608246158217,-11.7683139215713,-2.94281490475174));
#25565=CARTESIAN_POINT('Ctrl Pts',(13.3027146141536,-12.0682094443783,-2.65901005153359));
#25566=CARTESIAN_POINT('Ctrl Pts',(14.2466220418226,-12.4758213511285,-2.27326825624961));
#25567=CARTESIAN_POINT('Ctrl Pts',(15.3788107202461,-12.9964429752181,-1.81469981611628));
#25568=CARTESIAN_POINT('Ctrl Pts',(16.3720853361384,-13.4908337691235,-1.45099516743195));
#25569=CARTESIAN_POINT('Ctrl Pts',(17.5300464833505,-14.067195353042,-1.02698770212637));
#25570=CARTESIAN_POINT('Ctrl Pts',(18.5522571217452,-14.6297459826146,-0.660939172705208));
#25571=CARTESIAN_POINT('Ctrl Pts',(19.459740928474,-15.1671394203612,-0.37124288507375));
#25572=CARTESIAN_POINT('Ctrl Pts',(20.7212139011503,-15.9141580364338,0.0314574545047842));
#25573=CARTESIAN_POINT('Ctrl Pts',(21.748318091447,-16.6062803213006,0.336055810056771));
#25574=CARTESIAN_POINT('Ctrl Pts',(22.5801692622301,-17.2054151585246,0.547760951425958));
#25575=CARTESIAN_POINT('Ctrl Pts',(23.3330995249136,-17.7477077779475,0.739380814811507));
#25576=CARTESIAN_POINT('Ctrl Pts',(23.9217876543842,-18.206905015041,0.875119715101746));
#25577=CARTESIAN_POINT('Ctrl Pts',(24.4822919865211,-18.6643830136337,0.991018194629963));
#25578=CARTESIAN_POINT('Ctrl Pts',(24.9418792870016,-19.0394935459661,1.08604951960313));
#25579=CARTESIAN_POINT('Ctrl Pts',(25.3626276506119,-19.3999270898306,1.16248493478925));
#25580=CARTESIAN_POINT('Ctrl Pts',(25.7525302890144,-19.7463071016619,1.22321331868058));
#25581=CARTESIAN_POINT('Ctrl Pts',(26.1776080056337,-20.1239357966488,1.28942031554593));
#25582=CARTESIAN_POINT('Ctrl Pts',(26.5661459571672,-20.4852396169796,1.33297321439401));
#25583=CARTESIAN_POINT('Ctrl Pts',(26.9267016831501,-20.8313979297669,1.3663881523399));
#25584=CARTESIAN_POINT('Ctrl Pts',(27.1778777842841,-21.0725442744658,1.38966620127396));
#25585=CARTESIAN_POINT('Ctrl Pts',(27.4154861119772,-21.3064162463263,1.40780557011332));
#25586=CARTESIAN_POINT('Ctrl Pts',(27.6422281942556,-21.5339888726617,1.42326116565077));
#25587=CARTESIAN_POINT('Ctrl Pts',(27.8555559933378,-21.7480980800028,1.43780239305054));
#25588=CARTESIAN_POINT('Ctrl Pts',(28.1190837193167,-22.0160369614215,1.45368682614544));
#25589=CARTESIAN_POINT('Ctrl Pts',(28.4603051775879,-22.3749799381774,1.47251023690701));
#25590=CARTESIAN_POINT('Ctrl Pts',(28.601773083253,-22.5237950549995,1.4803142844936));
#25591=CARTESIAN_POINT('Ctrl Pts',(28.7540286646448,-22.6856884569071,1.48853267939426));
#25592=CARTESIAN_POINT('Ctrl Pts',(28.9157341130969,-22.8599017516109,1.49763121638955));
#25593=CARTESIAN_POINT('Ctrl Pts',(29.4787137469354,-23.4664276157734,1.52930789194515));
#25594=CARTESIAN_POINT('Ctrl Pts',(30.1711677436439,-24.2477248210915,1.53976925233531));
#25595=CARTESIAN_POINT('Ctrl Pts',(30.8055547543787,-24.9885333989192,1.53340754825749));
#25596=CARTESIAN_POINT('Ctrl Pts',(31.1893125644455,-25.4366684847504,1.52955918190716));
#25597=CARTESIAN_POINT('Ctrl Pts',(31.5650207099063,-25.8828713567949,1.52122455967932));
#25598=CARTESIAN_POINT('Ctrl Pts',(31.9311744366552,-26.319234664178,1.51382648741802));
#25599=CARTESIAN_POINT('Ctrl Pts',(32.1142513000296,-26.5374163178695,1.51012745128737));
#25600=CARTESIAN_POINT('Ctrl Pts',(32.2949430642635,-26.7531357746902,1.50666813405654));
#25601=CARTESIAN_POINT('Ctrl Pts',(32.4730466959745,-26.9654180603387,1.50413682057756));
#25602=CARTESIAN_POINT('Ctrl Pts',(32.5932788659568,-27.1087231665129,1.50242801032164));
#25603=CARTESIAN_POINT('Ctrl Pts',(32.7123311760565,-27.2504621963818,1.50114220273886));
#25604=CARTESIAN_POINT('Ctrl Pts',(32.8301302692951,-27.3903440144041,1.50048655910813));
#25605=CARTESIAN_POINT('Ctrl Pts',(32.8868306159413,-27.457673459422,1.50017097755214));
#25606=CARTESIAN_POINT('Ctrl Pts',(32.9387123022443,-27.5192120661501,1.50000000000001));
#25607=CARTESIAN_POINT('Ctrl Pts',(33.,-27.5917792275077,1.50000000000001));
#25608=CARTESIAN_POINT('Ctrl Pts',(33.0955022515216,-27.7048578313703,1.50000000000001));
#25609=CARTESIAN_POINT('Ctrl Pts',(33.24174784516,-27.8775886863802,1.5));
#25610=CARTESIAN_POINT('Ctrl Pts',(33.3688392455923,-28.0268611295878,1.5));
#25611=CARTESIAN_POINT('Ctrl Pts',(34.2661932187598,-29.0808287429838,1.5));
#25612=CARTESIAN_POINT('Ctrl Pts',(35.2319960542697,-30.180966291201,1.50000000000001));
#25613=CARTESIAN_POINT('Ctrl Pts',(36.3004607333286,-31.2401426718624,1.50000000000001));
#25614=CARTESIAN_POINT('Ctrl Pts',(36.6891719086969,-31.6254747318907,1.50000000000001));
#25615=CARTESIAN_POINT('Ctrl Pts',(37.089305975904,-32.002886614661,1.50000000000001));
#25616=CARTESIAN_POINT('Ctrl Pts',(37.5,-32.3652591523689,1.50000000000001));
#25617=CARTESIAN_POINT('',(37.5,-32.1719479119405,3.83741678103716));
#25618=CARTESIAN_POINT('Origin',(37.5,0.,0.));
#25619=CARTESIAN_POINT('',(36.8,-31.4347259190859,4.53355051147315));
#25620=CARTESIAN_POINT('Ctrl Pts',(37.5,-32.1719479119405,3.83741678103717));
#25621=CARTESIAN_POINT('Ctrl Pts',(37.2470086540956,-31.9226755103028,4.04454785994593));
#25622=CARTESIAN_POINT('Ctrl Pts',(37.0122659037829,-31.6748439028166,4.2761329400914));
#25623=CARTESIAN_POINT('Ctrl Pts',(36.8,-31.4347259190859,4.53355051147316));
#25624=CARTESIAN_POINT('',(36.8,-29.4900464626661,11.7911930472673));
#25625=CARTESIAN_POINT('Ctrl Pts',(36.8,-31.4347259190859,4.53355051147315));
#25626=CARTESIAN_POINT('Ctrl Pts',(36.8,-31.1968691126063,6.18280168905531));
#25627=CARTESIAN_POINT('Ctrl Pts',(36.8,-30.8293258095436,7.81258162569766));
#25628=CARTESIAN_POINT('Ctrl Pts',(36.8,-30.0846548283827,10.2137688485759));
#25629=CARTESIAN_POINT('Ctrl Pts',(36.8,-29.8028301128151,11.0089139056503));
#25630=CARTESIAN_POINT('Ctrl Pts',(36.8,-29.4900464626661,11.7911930472673));
#25631=CARTESIAN_POINT('',(37.5,-29.7804325714888,12.7626735386834));
#25632=CARTESIAN_POINT('Ctrl Pts',(36.8,-29.4900464626661,11.7911930472673));
#25633=CARTESIAN_POINT('Ctrl Pts',(37.0122659037829,-29.5692859507915,12.1341821953298));
#25634=CARTESIAN_POINT('Ctrl Pts',(37.2470086540957,-29.6681218786625,12.4586565616163));
#25635=CARTESIAN_POINT('Ctrl Pts',(37.5,-29.7804325714888,12.7626735386834));
#25636=CARTESIAN_POINT('',(37.5,-28.7791366260183,14.8835914705078));
#25637=CARTESIAN_POINT('Origin',(37.5,0.,0.));
#25638=CARTESIAN_POINT('',(6.9,-10.3676856018661,-3.76156693666918));
#25639=CARTESIAN_POINT('Ctrl Pts',(37.5,-28.7791366260183,14.8835914705078));
#25640=CARTESIAN_POINT('Ctrl Pts',(36.6490696321449,-28.1289147924265,14.5081857198506));
#25641=CARTESIAN_POINT('Ctrl Pts',(35.8406537801018,-27.4207836130714,14.0993459928284));
#25642=CARTESIAN_POINT('Ctrl Pts',(35.0774452370719,-26.7027592163157,13.6847944140768));
#25643=CARTESIAN_POINT('Ctrl Pts',(34.695840965557,-26.3437470179379,13.477518624701));
#25644=CARTESIAN_POINT('Ctrl Pts',(34.325525504184,-25.9822790639256,13.2688250041486));
#25645=CARTESIAN_POINT('Ctrl Pts',(33.9666810635471,-25.6244801370893,13.0622496974238));
#25646=CARTESIAN_POINT('Ctrl Pts',(33.7186145566571,-25.3771363861544,12.9194457162392));
#25647=CARTESIAN_POINT('Ctrl Pts',(33.467102416882,-25.1224476749868,12.7724011202871));
#25648=CARTESIAN_POINT('Ctrl Pts',(33.2400985609469,-24.8908093158743,12.6386646512988));
#25649=CARTESIAN_POINT('Ctrl Pts',(33.1387264796113,-24.7873676254956,12.5789425635132));
#25650=CARTESIAN_POINT('Ctrl Pts',(33.0532004124129,-24.6997339702936,12.5283472490923));
#25651=CARTESIAN_POINT('Ctrl Pts',(33.,-24.6451817466334,12.4968515080772));
#25652=CARTESIAN_POINT('Ctrl Pts',(32.9185691495402,-24.5616817554558,12.4486427656934));
#25653=CARTESIAN_POINT('Ctrl Pts',(32.8516820632897,-24.4928265642338,12.4091965179816));
#25654=CARTESIAN_POINT('Ctrl Pts',(32.7777321455643,-24.4165289206393,12.3657029367261));
#25655=CARTESIAN_POINT('Ctrl Pts',(32.1788699539947,-23.7986543447101,12.013482647765));
#25656=CARTESIAN_POINT('Ctrl Pts',(31.5692879871422,-23.1567007301401,11.6640598398765));
#25657=CARTESIAN_POINT('Ctrl Pts',(30.9513498040681,-22.5260018679712,11.3096185478538));
#25658=CARTESIAN_POINT('Ctrl Pts',(30.642380712531,-22.2106524368868,11.1323979018424));
#25659=CARTESIAN_POINT('Ctrl Pts',(30.3347880607069,-21.9015729508076,10.9558507302082));
#25660=CARTESIAN_POINT('Ctrl Pts',(30.0249306371907,-21.5982641082844,10.7763433330207));
#25661=CARTESIAN_POINT('Ctrl Pts',(29.8700019254325,-21.4466096870229,10.6865896344269));
#25662=CARTESIAN_POINT('Ctrl Pts',(29.7145097313521,-21.296396533813,10.5960927952752));
#25663=CARTESIAN_POINT('Ctrl Pts',(29.5580100720471,-21.14757273789,10.5043591957288));
#25664=CARTESIAN_POINT('Ctrl Pts',(29.4797602423946,-21.0731608399285,10.4584923959556));
#25665=CARTESIAN_POINT('Ctrl Pts',(29.4012586241226,-20.9990965425469,10.4123158264265));
#25666=CARTESIAN_POINT('Ctrl Pts',(29.3224502420508,-20.9253755287759,10.3657636829137));
#25667=CARTESIAN_POINT('Ctrl Pts',(29.2736528206127,-20.8797281587468,10.336939026118));
#25668=CARTESIAN_POINT('Ctrl Pts',(29.224737793726,-20.8342124355846,10.3079703168507));
#25669=CARTESIAN_POINT('Ctrl Pts',(29.1756921969555,-20.7888277156719,10.2788413042191));
#25670=CARTESIAN_POINT('Ctrl Pts',(29.1455286057134,-20.7609156046929,10.2609266352547));
#25671=CARTESIAN_POINT('Ctrl Pts',(29.118149096832,-20.7356566759699,10.2446403152225));
#25672=CARTESIAN_POINT('Ctrl Pts',(29.0849408699094,-20.7051394327917,10.2248462834623));
#25673=CARTESIAN_POINT('Ctrl Pts',(29.0475462331583,-20.670775019842,10.2025569083253));
#25674=CARTESIAN_POINT('Ctrl Pts',(28.9599837407919,-20.5905365513284,10.150562007605));
#25675=CARTESIAN_POINT('Ctrl Pts',(28.8924081847562,-20.529003052346,10.1107110564809));
#25676=CARTESIAN_POINT('Ctrl Pts',(28.4410807634412,-20.1180296612357,9.84455228453923));
#25677=CARTESIAN_POINT('Ctrl Pts',(27.9936088566446,-19.7235361016266,9.59004457949594));
#25678=CARTESIAN_POINT('Ctrl Pts',(27.5122543094016,-19.3231338575611,9.31395242975933));
#25679=CARTESIAN_POINT('Ctrl Pts',(27.1397294105009,-19.0132587221866,9.10028206815794));
#25680=CARTESIAN_POINT('Ctrl Pts',(26.7276341640386,-18.6830630720646,8.86410488389253));
#25681=CARTESIAN_POINT('Ctrl Pts',(26.2530417505368,-18.3335669465969,8.57522710561968));
#25682=CARTESIAN_POINT('Ctrl Pts',(25.869494913884,-18.0511179871699,8.34176749926329));
#25683=CARTESIAN_POINT('Ctrl Pts',(25.4447383161098,-17.75405561874,8.07732257195745));
#25684=CARTESIAN_POINT('Ctrl Pts',(24.9635886608355,-17.4401876876767,7.77432947327157));
#25685=CARTESIAN_POINT('Ctrl Pts',(24.6119820459486,-17.210824454111,7.5529131704743));
#25686=CARTESIAN_POINT('Ctrl Pts',(24.2873626785981,-17.0017823418902,7.3468597886102));
#25687=CARTESIAN_POINT('Ctrl Pts',(23.6426616418513,-16.6259529315257,6.93898570173334));
#25688=CARTESIAN_POINT('Ctrl Pts',(23.5760533212114,-16.5871235137886,6.8968455368959));
#25689=CARTESIAN_POINT('Ctrl Pts',(23.5065967305478,-16.546947509856,6.85292160236948));
#25690=CARTESIAN_POINT('Ctrl Pts',(23.4342591639586,-16.5054784159948,6.80720851268154));
#25691=CARTESIAN_POINT('Ctrl Pts',(22.7443384436226,-16.1099662574108,6.37121917472936));
#25692=CARTESIAN_POINT('Ctrl Pts',(21.7987837593133,-15.6084067036785,5.75271743556796));
#25693=CARTESIAN_POINT('Ctrl Pts',(20.5610365528855,-15.0432759423309,4.96573918168374));
#25694=CARTESIAN_POINT('Ctrl Pts',(19.7234582214104,-14.6608543317657,4.43319430549868));
#25695=CARTESIAN_POINT('Ctrl Pts',(18.7603809281624,-14.2617573685878,3.80221290992159));
#25696=CARTESIAN_POINT('Ctrl Pts',(17.6514222906382,-13.8414640697512,3.10236545497629));
#25697=CARTESIAN_POINT('Ctrl Pts',(16.7565277906387,-13.5023006881889,2.53761072285444));
#25698=CARTESIAN_POINT('Ctrl Pts',(15.7613807992389,-13.1550491146656,1.89253400855812));
#25699=CARTESIAN_POINT('Ctrl Pts',(14.7199652846762,-12.8103195459473,1.24173803388781));
#25700=CARTESIAN_POINT('Ctrl Pts',(13.7316067501733,-12.4831529092169,0.624098151639976));
#25701=CARTESIAN_POINT('Ctrl Pts',(12.7260968661244,-12.1691790146818,-0.023032282421214));
#25702=CARTESIAN_POINT('Ctrl Pts',(11.7781012037546,-11.8786003909685,-0.615505739626223));
#25703=CARTESIAN_POINT('Ctrl Pts',(10.6475718363527,-11.5320717298292,-1.32205817373976));
#25704=CARTESIAN_POINT('Ctrl Pts',(9.62260863652904,-11.2216623289213,-1.98990805505865));
#25705=CARTESIAN_POINT('Ctrl Pts',(8.83596460437641,-10.9799836949691,-2.49396550450873));
#25706=CARTESIAN_POINT('Ctrl Pts',(8.38131550044618,-10.8403030136515,-2.78529075246711));
#25707=CARTESIAN_POINT('Ctrl Pts',(7.99969688490049,-10.7217137549231,-3.03233135775693));
#25708=CARTESIAN_POINT('Ctrl Pts',(7.59379043301041,-10.5924279410152,-3.29961262120675));
#25709=CARTESIAN_POINT('Ctrl Pts',(7.361457734305,-10.5184273383894,-3.45259904692512));
#25710=CARTESIAN_POINT('Ctrl Pts',(7.13004605045497,-10.4436236908379,-3.60654870801928));
#25711=CARTESIAN_POINT('Ctrl Pts',(6.9,-10.3676856018661,-3.76156693666918));
#25712=CARTESIAN_POINT('',(6.9,-11.02768739857,-0.168526548660246));
#25713=CARTESIAN_POINT('Ctrl Pts',(6.90000000000001,-10.3676856018661,-3.76156693666918));
#25714=CARTESIAN_POINT('Ctrl Pts',(6.90000000000001,-10.5551707158657,-3.24481773355662));
#25715=CARTESIAN_POINT('Ctrl Pts',(6.90000000000001,-10.7040448708755,-2.71398840242747));
#25716=CARTESIAN_POINT('Ctrl Pts',(6.90000000000001,-10.9457448952802,-1.51153848953113));
#25717=CARTESIAN_POINT('Ctrl Pts',(6.90000000000001,-11.0174195217678,-0.84041437002766));
#25718=CARTESIAN_POINT('Ctrl Pts',(6.90000000000001,-11.02768739857,-0.168526548660247));
#25719=CARTESIAN_POINT('',(37.5,-27.2791366260183,17.4816676818611));
#25720=CARTESIAN_POINT('Ctrl Pts',(6.9,-11.02768739857,-0.168526548660246));
#25721=CARTESIAN_POINT('Ctrl Pts',(6.98893730997578,-11.0357428000776,-0.109835775321743));
#25722=CARTESIAN_POINT('Ctrl Pts',(7.08052892388264,-11.0440392866244,-0.049724360260793));
#25723=CARTESIAN_POINT('Ctrl Pts',(7.17490192378011,-11.0526088775152,0.0118631160266181));
#25724=CARTESIAN_POINT('Ctrl Pts',(7.97363347621222,-11.1251381246873,0.533112420370669));
#25725=CARTESIAN_POINT('Ctrl Pts',(8.96286060502742,-11.2096216302968,1.17518961595099));
#25726=CARTESIAN_POINT('Ctrl Pts',(10.2403127965964,-11.3564324284624,1.93497024136951));
#25727=CARTESIAN_POINT('Ctrl Pts',(10.439427640776,-11.3793156403693,2.05339627863287));
#25728=CARTESIAN_POINT('Ctrl Pts',(10.6449386760821,-11.4036121640905,2.17568840229239));
#25729=CARTESIAN_POINT('Ctrl Pts',(10.857227022666,-11.4296460138916,2.30180801494842));
#25730=CARTESIAN_POINT('Ctrl Pts',(11.0079272576484,-11.4481270438004,2.39133838987944));
#25731=CARTESIAN_POINT('Ctrl Pts',(11.244571866198,-11.4774498561359,2.53195192940694));
#25732=CARTESIAN_POINT('Ctrl Pts',(11.5512244265066,-11.5182347543578,2.71302722024009));
#25733=CARTESIAN_POINT('Ctrl Pts',(12.004464269483,-11.5785158126582,2.98066084541349));
#25734=CARTESIAN_POINT('Ctrl Pts',(12.6082461583111,-11.6630662681827,3.33560449468883));
#25735=CARTESIAN_POINT('Ctrl Pts',(13.3027146141536,-11.7808809827897,3.73133446864291));
#25736=CARTESIAN_POINT('Ctrl Pts',(14.2466220417484,-11.9410123512658,4.2692026159931));
#25737=CARTESIAN_POINT('Ctrl Pts',(15.3788107201835,-12.1625996834172,4.92664534657395));
#25738=CARTESIAN_POINT('Ctrl Pts',(16.3720853361384,-12.4089023460099,5.48881820879721));
#25739=CARTESIAN_POINT('Ctrl Pts',(17.5300464833438,-12.6960423867943,6.1442002371016));
#25740=CARTESIAN_POINT('Ctrl Pts',(18.5522571217469,-13.0002012582108,6.74248287738932));
#25741=CARTESIAN_POINT('Ctrl Pts',(19.459740928474,-13.3207494833101,7.26206394073252));
#25742=CARTESIAN_POINT('Ctrl Pts',(20.7212139012125,-13.7663364121616,7.98432197299206));
#25743=CARTESIAN_POINT('Ctrl Pts',(21.7483180915274,-14.2134327156235,8.59417302929552));
#25744=CARTESIAN_POINT('Ctrl Pts',(22.5801692622301,-14.6264461342272,9.0770824783983));
#25745=CARTESIAN_POINT('Ctrl Pts',(23.3330995247002,-15.0002753871335,9.51417645754747));
#25746=CARTESIAN_POINT('Ctrl Pts',(23.9217876538143,-15.3300824094504,9.8613284118158));
#25747=CARTESIAN_POINT('Ctrl Pts',(24.4822919856966,-15.668320737957,10.1904384384949));
#25748=CARTESIAN_POINT('Ctrl Pts',(24.9418792864885,-15.9456603258612,10.4602932464266));
#25749=CARTESIAN_POINT('Ctrl Pts',(25.362627650368,-16.2195872237959,10.7067050298183));
#25750=CARTESIAN_POINT('Ctrl Pts',(25.7525302890144,-16.489196921628,10.9324873590558));
#25751=CARTESIAN_POINT('Ctrl Pts',(26.1776080055415,-16.7831294661882,11.1786386476896));
#25752=CARTESIAN_POINT('Ctrl Pts',(26.5661459570144,-17.0742513036037,11.3970084746332));
#25753=CARTESIAN_POINT('Ctrl Pts',(26.9267016829645,-17.357325727205,11.5990258161359));
#25754=CARTESIAN_POINT('Ctrl Pts',(27.1778777840597,-17.554525563243,11.7397583701913));
#25755=CARTESIAN_POINT('Ctrl Pts',(27.4154861117292,-17.747994947664,11.8724035103318));
#25756=CARTESIAN_POINT('Ctrl Pts',(27.6422281939979,-17.9373508254958,11.9995747618597));
#25757=CARTESIAN_POINT('Ctrl Pts',(27.8555559931681,-18.1155042246074,12.1192224379096));
#25758=CARTESIAN_POINT('Ctrl Pts',(28.1190837191615,-18.3396038860388,12.2669482012106));
#25759=CARTESIAN_POINT('Ctrl Pts',(28.4603051775582,-18.641045917149,12.4627212415658));
#25760=CARTESIAN_POINT('Ctrl Pts',(28.6017730832315,-18.7660215649979,12.5438873034438));
#25761=CARTESIAN_POINT('Ctrl Pts',(28.7540286646334,-18.9021161663134,12.6319513431655));
#25762=CARTESIAN_POINT('Ctrl Pts',(28.9157341130969,-19.0484400367167,12.7269375546994));
#25763=CARTESIAN_POINT('Ctrl Pts',(29.4787137469378,-19.557868505358,13.0576332925206));
#25764=CARTESIAN_POINT('Ctrl Pts',(30.1711677436509,-20.2292610528789,13.4573416990383));
#25765=CARTESIAN_POINT('Ctrl Pts',(30.8055547543906,-20.8740009526632,13.8222365906122));
#25766=CARTESIAN_POINT('Ctrl Pts',(31.1893125644552,-21.2640215044932,14.0429713505041));
#25767=CARTESIAN_POINT('Ctrl Pts',(31.5650207099141,-21.6546118380374,14.258854791945));
#25768=CARTESIAN_POINT('Ctrl Pts',(31.9311744366611,-22.0362125836393,14.4706295271182));
#25769=CARTESIAN_POINT('Ctrl Pts',(32.1142513000346,-22.2270129564403,14.5765168947048));
#25770=CARTESIAN_POINT('Ctrl Pts',(32.2949430642676,-22.4155611447519,14.6813807665129));
#25771=CARTESIAN_POINT('Ctrl Pts',(32.4730466959776,-22.6006686536355,14.7853297275589));
#25772=CARTESIAN_POINT('Ctrl Pts',(32.5932788659536,-22.7256289211957,14.8555024075504));
#25773=CARTESIAN_POINT('Ctrl Pts',(32.7123311760469,-22.8490214255548,14.9252583804501));
#25774=CARTESIAN_POINT('Ctrl Pts',(32.8301302692793,-22.9704904552987,14.9946314854175));
#25775=CARTESIAN_POINT('Ctrl Pts',(32.8868306159308,-23.0289572558904,15.0280229062851));
#25776=CARTESIAN_POINT('Ctrl Pts',(32.9387123022385,-23.0823367414113,15.0586441387483));
#25777=CARTESIAN_POINT('Ctrl Pts',(33.,-23.1451817466334,15.0949277194305));
#25778=CARTESIAN_POINT('Ctrl Pts',(33.0955022515197,-23.243110690201,15.1514670213607));
#25779=CARTESIAN_POINT('Ctrl Pts',(33.2417478451538,-23.3926999986525,15.2378324488631));
#25780=CARTESIAN_POINT('Ctrl Pts',(33.3688392455845,-23.5219737265538,15.312468670466));
#25781=CARTESIAN_POINT('Ctrl Pts',(34.266193219056,-24.43473645483,15.8394524773426));
#25782=CARTESIAN_POINT('Ctrl Pts',(35.231996054922,-25.3874835195854,16.3895212516487));
#25783=CARTESIAN_POINT('Ctrl Pts',(36.3004607343901,-26.3047571725944,16.919109442134));
#25784=CARTESIAN_POINT('Ctrl Pts',(36.6891719094257,-26.6384645251555,17.1117754719657));
#25785=CARTESIAN_POINT('Ctrl Pts',(37.0893059762781,-26.9653128030153,17.3004814131722));
#25786=CARTESIAN_POINT('Ctrl Pts',(37.5,-27.2791366260183,17.4816676818611));
#25787=CARTESIAN_POINT('',(37.5,-25.9430157904516,19.4092743732572));
#25788=CARTESIAN_POINT('Origin',(37.5,0.,0.));
#25789=CARTESIAN_POINT('',(36.8,-24.9564959511929,19.6435328718186));
#25790=CARTESIAN_POINT('Ctrl Pts',(37.5,-25.9430157904516,19.4092743732572));
#25791=CARTESIAN_POINT('Ctrl Pts',(37.2470086540956,-25.6235740187166,19.4640189486865));
#25792=CARTESIAN_POINT('Ctrl Pts',(37.0122659037829,-25.2931530107001,19.5406617074869));
#25793=CARTESIAN_POINT('Ctrl Pts',(36.8,-24.9564959511929,19.6435328718186));
#25794=CARTESIAN_POINT('',(36.8,-19.6435328718186,24.9564959511929));
#25795=CARTESIAN_POINT('Ctrl Pts',(36.8,-24.9564959511929,19.6435328718186));
#25796=CARTESIAN_POINT('Ctrl Pts',(36.8,-24.4957748831848,20.2288646216318));
#25797=CARTESIAN_POINT('Ctrl Pts',(36.8,-24.0141222843114,20.7984186457787));
#25798=CARTESIAN_POINT('Ctrl Pts',(36.8,-22.3234241559746,22.6602579716864));
#25799=CARTESIAN_POINT('Ctrl Pts',(36.8,-21.029056769996,23.8659348286794));
#25800=CARTESIAN_POINT('Ctrl Pts',(36.8,-19.6435328718186,24.9564959511929));
#25801=CARTESIAN_POINT('',(37.5,-19.4092743732571,25.9430157904517));
#25802=CARTESIAN_POINT('Ctrl Pts',(36.8,-19.6435328718186,24.9564959511929));
#25803=CARTESIAN_POINT('Ctrl Pts',(37.0122659037829,-19.5406617074869,25.2931530107001));
#25804=CARTESIAN_POINT('Ctrl Pts',(37.2470086540956,-19.4640189486865,25.6235740187166));
#25805=CARTESIAN_POINT('Ctrl Pts',(37.5,-19.4092743732572,25.9430157904516));
#25806=CARTESIAN_POINT('',(37.5,-17.4816676818611,27.2791366260183));
#25807=CARTESIAN_POINT('Origin',(37.5,0.,0.));
#25808=CARTESIAN_POINT('',(6.9,-10.8594625780008,1.9262302757419));
#25809=CARTESIAN_POINT('Ctrl Pts',(37.5,-17.4816676818611,27.2791366260183));
#25810=CARTESIAN_POINT('Ctrl Pts',(36.6490696321448,-17.1062619312039,26.6289147924265));
#25811=CARTESIAN_POINT('Ctrl Pts',(35.8406537801013,-16.6974222041815,25.920783613071));
#25812=CARTESIAN_POINT('Ctrl Pts',(35.0774452370697,-16.2828706254288,25.2027592163136));
#25813=CARTESIAN_POINT('Ctrl Pts',(34.6958409655539,-16.0755948360525,24.8437470179349));
#25814=CARTESIAN_POINT('Ctrl Pts',(34.3255255041797,-15.8669012154994,24.4822790639214));
#25815=CARTESIAN_POINT('Ctrl Pts',(33.9666810635412,-15.6603259087737,24.1244801370834));
#25816=CARTESIAN_POINT('Ctrl Pts',(33.718614556661,-15.5175219275947,23.8771363861582));
#25817=CARTESIAN_POINT('Ctrl Pts',(33.4671024168984,-15.3704773316499,23.6224476750034));
#25818=CARTESIAN_POINT('Ctrl Pts',(33.2400985609675,-15.2367408626642,23.3908093158952));
#25819=CARTESIAN_POINT('Ctrl Pts',(33.1387264796193,-15.1770187748713,23.2873676255038));
#25820=CARTESIAN_POINT('Ctrl Pts',(33.0532004124107,-15.1264234604443,23.1997339702914));
#25821=CARTESIAN_POINT('Ctrl Pts',(33.,-15.0949277194305,23.1451817466334));
#25822=CARTESIAN_POINT('Ctrl Pts',(32.9185691495597,-15.0467189770583,23.0616817554757));
#25823=CARTESIAN_POINT('Ctrl Pts',(32.851682063321,-15.0068117561407,22.9930927072745));
#25824=CARTESIAN_POINT('Ctrl Pts',(32.7777321456099,-14.9624828491754,22.917277339223));
#25825=CARTESIAN_POINT('Ctrl Pts',(32.1788699540345,-14.6034979145461,22.3033083332839));
#25826=CARTESIAN_POINT('Ctrl Pts',(31.5692879871757,-14.2222611802172,21.679722497699));
#25827=CARTESIAN_POINT('Ctrl Pts',(30.9513498040926,-13.8532805894466,21.0574179035634));
#25828=CARTESIAN_POINT('Ctrl Pts',(30.6423807125511,-13.6687902940613,20.7462656064956));
#25829=CARTESIAN_POINT('Ctrl Pts',(30.3347880607231,-13.4893931931425,20.4388315278504));
#25830=CARTESIAN_POINT('Ctrl Pts',(30.0249306372029,-13.3164737289165,20.1317191404533));
#25831=CARTESIAN_POINT('Ctrl Pts',(29.8700019254428,-13.2300139968034,19.9781629467547));
#25832=CARTESIAN_POINT('Ctrl Pts',(29.7145097313604,-13.1451740097158,19.8246838084803));
#25833=CARTESIAN_POINT('Ctrl Pts',(29.5580100720534,-13.0621556215309,19.670828282929));
#25834=CARTESIAN_POINT('Ctrl Pts',(29.4797602423999,-13.0206464274385,19.5939005201534));
#25835=CARTESIAN_POINT('Ctrl Pts',(29.401258624127,-12.9795931491566,19.5168782891898));
#25836=CARTESIAN_POINT('Ctrl Pts',(29.3224502420541,-12.939024950194,19.4397024434206));
#25837=CARTESIAN_POINT('Ctrl Pts',(29.2736528205583,-12.913905496501,19.3919158733091));
#25838=CARTESIAN_POINT('Ctrl Pts',(29.2247377936137,-12.8889720785753,19.3440703735311));
#25839=CARTESIAN_POINT('Ctrl Pts',(29.1756921967849,-12.8642322644742,19.2961515485917));
#25840=CARTESIAN_POINT('Ctrl Pts',(29.1455286055995,-12.8490170018044,19.2666809347342));
#25841=CARTESIAN_POINT('Ctrl Pts',(29.1181490967649,-12.8352852878977,19.2399471035364));
#25842=CARTESIAN_POINT('Ctrl Pts',(29.0849408699094,-12.8187535959654,19.2075463476651));
#25843=CARTESIAN_POINT('Ctrl Pts',(29.0475462330785,-12.8001378288936,19.1710609760093));
#25844=CARTESIAN_POINT('Ctrl Pts',(28.9599837406718,-12.7566467271403,19.0859128368227));
#25845=CARTESIAN_POINT('Ctrl Pts',(28.8924081845882,-12.7232826293765,19.0206341512474));
#25846=CARTESIAN_POINT('Ctrl Pts',(28.441080763257,-12.5004486183602,18.5846471977387));
#25847=CARTESIAN_POINT('Ctrl Pts',(27.9936088564545,-12.286061026631,18.1669902799056));
#25848=CARTESIAN_POINT('Ctrl Pts',(27.5122543091764,-12.0773485863978,17.7276863423864));
#25849=CARTESIAN_POINT('Ctrl Pts',(27.1397294103343,-11.9158240279936,17.3877048135723));
#25850=CARTESIAN_POINT('Ctrl Pts',(26.7276341639424,-11.7479547989366,17.0180715472069));
#25851=CARTESIAN_POINT('Ctrl Pts',(26.2530417505368,-11.5897211649258,16.593147989986));
#25852=CARTESIAN_POINT('Ctrl Pts',(25.8694949138842,-11.4618429939678,16.2497415604106));
#25853=CARTESIAN_POINT('Ctrl Pts',(25.4447383161107,-11.3368019000522,15.8721943512474));
#25854=CARTESIAN_POINT('Ctrl Pts',(24.9635886608374,-11.2164808476613,15.4528606650833));
#25855=CARTESIAN_POINT('Ctrl Pts',(24.6119820459382,-11.1285546120948,15.1464269052552));
#25856=CARTESIAN_POINT('Ctrl Pts',(24.2873626785755,-11.0505455233798,14.863458385904));
#25857=CARTESIAN_POINT('Ctrl Pts',(23.6426616417925,-10.9290047499479,14.3223143599116));
#25858=CARTESIAN_POINT('Ctrl Pts',(23.5760533211706,-10.9164475701956,14.2664051977893));
#25859=CARTESIAN_POINT('Ctrl Pts',(23.5065967305265,-10.9036160974344,14.2082779527054));
#25860=CARTESIAN_POINT('Ctrl Pts',(23.4342591639586,-10.8905593535264,14.1479547088373));
#25861=CARTESIAN_POINT('Ctrl Pts',(22.7443384436235,-10.7660304456633,13.5726207871003));
#25862=CARTESIAN_POINT('Ctrl Pts',(21.7987837593143,-10.640918000201,12.7862027918356));
#25863=CARTESIAN_POINT('Ctrl Pts',(20.5610365528855,-10.544989531356,11.8220942510713));
#25864=CARTESIAN_POINT('Ctrl Pts',(19.7234582214107,-10.4800751397429,11.1696860543574));
#25865=CARTESIAN_POINT('Ctrl Pts',(18.7603809281627,-10.4499377288461,10.4236916548834));
#25866=CARTESIAN_POINT('Ctrl Pts',(17.6514222906382,-10.4358767824859,9.60745933070834));
#25867=CARTESIAN_POINT('Ctrl Pts',(16.7565277906386,-10.4245300440805,8.94878569500211));
#25868=CARTESIAN_POINT('Ctrl Pts',(15.7613807992386,-10.4463397170534,8.21650708626994));
#25869=CARTESIAN_POINT('Ctrl Pts',(14.7199652846762,-10.4731931404428,7.48053645516581));
#25870=CARTESIAN_POINT('Ctrl Pts',(13.7316067501732,-10.4986784628874,6.78206130838347));
#25871=CARTESIAN_POINT('Ctrl Pts',(12.7260968661243,-10.5503343111255,6.06464296565691));
#25872=CARTESIAN_POINT('Ctrl Pts',(11.7781012037546,-10.5949225697956,5.40625658879283));
#25873=CARTESIAN_POINT('Ctrl Pts',(10.6475718363526,-10.6480961631663,4.62109990117504));
#25874=CARTESIAN_POINT('Ctrl Pts',(9.62260863652902,-10.713198677066,3.88752023758458));
#25875=CARTESIAN_POINT('Ctrl Pts',(8.83596460437641,-10.7559275652365,3.33015436441791));
#25876=CARTESIAN_POINT('Ctrl Pts',(8.38131550044684,-10.7806231707767,3.00801895826384));
#25877=CARTESIAN_POINT('Ctrl Pts',(7.99969688490164,-10.8014421627468,2.7347808889527));
#25878=CARTESIAN_POINT('Ctrl Pts',(7.59379043301203,-10.8231179952785,2.43866561789595));
#25879=CARTESIAN_POINT('Ctrl Pts',(7.36145773430608,-10.8355248063684,2.26917518547639));
#25880=CARTESIAN_POINT('Ctrl Pts',(7.1300460504555,-10.8477177778403,2.09844904428872));
#25881=CARTESIAN_POINT('Ctrl Pts',(6.9,-10.8594625780008,1.9262302757419));
#25882=CARTESIAN_POINT('',(6.9,-9.63452070648529,5.36789542693312));
#25883=CARTESIAN_POINT('Ctrl Pts',(6.90000000000001,-10.8594625780008,1.92623027574191));
#25884=CARTESIAN_POINT('Ctrl Pts',(6.90000000000001,-10.7829659225815,2.35749364924904));
#25885=CARTESIAN_POINT('Ctrl Pts',(6.90000000000001,-10.6806923192591,2.78469328079873));
#25886=CARTESIAN_POINT('Ctrl Pts',(6.90000000000001,-10.3240838050858,3.958690010018));
#25887=CARTESIAN_POINT('Ctrl Pts',(6.90000000000001,-10.0158641401962,4.68344446130229));
#25888=CARTESIAN_POINT('Ctrl Pts',(6.90000000000001,-9.6345207064853,5.36789542693312));
#25889=CARTESIAN_POINT('',(37.5,-14.8835914705078,28.7791366260183));
#25890=CARTESIAN_POINT('Ctrl Pts',(6.9,-9.6345207064853,5.36789542693312));
#25891=CARTESIAN_POINT('Ctrl Pts',(6.98893730997577,-9.61215150215932,5.42275082836582));
#25892=CARTESIAN_POINT('Ctrl Pts',(7.08052892388263,-9.58928076274048,5.47895708413941));
#25893=CARTESIAN_POINT('Ctrl Pts',(7.17490192378011,-9.56590850800827,5.5365781986047));
#25894=CARTESIAN_POINT('Ctrl Pts',(7.97363347621106,-9.36809602640493,6.02425796145695));
#25895=CARTESIAN_POINT('Ctrl Pts',(8.96286060502533,-9.12022229067351,6.62255487682446));
#25896=CARTESIAN_POINT('Ctrl Pts',(10.2403127965964,-8.8674738587251,7.35394959882411));
#25897=CARTESIAN_POINT('Ctrl Pts',(10.4394276407753,-8.82807828292514,7.46795116151676));
#25898=CARTESIAN_POINT('Ctrl Pts',(10.6449386760807,-8.78797362786174,7.58600750914886));
#25899=CARTESIAN_POINT('Ctrl Pts',(10.8572270226639,-8.74745979681984,7.70824722252455));
#25900=CARTESIAN_POINT('Ctrl Pts',(11.0079272576426,-8.71869965074415,7.79502331657747));
#25901=CARTESIAN_POINT('Ctrl Pts',(11.2445718661922,-8.67378718137334,7.93145962009207));
#25902=CARTESIAN_POINT('Ctrl Pts',(11.5512244264957,-8.61857029390861,8.1086678710592));
#25903=CARTESIAN_POINT('Ctrl Pts',(12.0044642694743,-8.53695840917655,8.37058591851777));
#25904=CARTESIAN_POINT('Ctrl Pts',(12.6082461583068,-8.43270942692374,8.72025136346692));
#25905=CARTESIAN_POINT('Ctrl Pts',(13.3027146141536,-8.33687497573541,9.12187093125611));
#25906=CARTESIAN_POINT('Ctrl Pts',(14.2466220417512,-8.20661873510301,9.66774409498751));
#25907=CARTESIAN_POINT('Ctrl Pts',(15.3788107201857,-8.06979762861279,10.3478998672794));
#25908=CARTESIAN_POINT('Ctrl Pts',(16.3720853361384,-8.00201556032625,10.9579071785779));
#25909=CARTESIAN_POINT('Ctrl Pts',(17.5300464833433,-7.92299511593714,11.6690546846652));
#25910=CARTESIAN_POINT('Ctrl Pts',(18.5522571217459,-7.8872631052263,12.3392620855055));
#25911=CARTESIAN_POINT('Ctrl Pts',(19.459740928474,-7.9050754796287,12.9495065982363));
#25912=CARTESIAN_POINT('Ctrl Pts',(20.7212139012062,-7.92983606347848,13.797793866682));
#25913=CARTESIAN_POINT('Ctrl Pts',(21.7483180915204,-8.01210729206202,14.5494885256954));
#25914=CARTESIAN_POINT('Ctrl Pts',(22.5801692622301,-8.12833268012627,15.1742070856531));
#25915=CARTESIAN_POINT('Ctrl Pts',(23.3330995247288,-8.23353132025034,15.7396562019122));
#25916=CARTESIAN_POINT('Ctrl Pts',(23.9217876538748,-8.34557660279632,16.2052021244665));
#25917=CARTESIAN_POINT('Ctrl Pts',(24.4822919857808,-8.47394457448518,16.6593389324847));
#25918=CARTESIAN_POINT('Ctrl Pts',(24.9418792865409,-8.57920029911431,17.0317098454144));
#25919=CARTESIAN_POINT('Ctrl Pts',(25.3626276503928,-8.69322205980333,17.3820721585682));
#25920=CARTESIAN_POINT('Ctrl Pts',(25.7525302890144,-8.81381974260611,17.7124102403086));
#25921=CARTESIAN_POINT('Ctrl Pts',(26.1776080055521,-8.94529714888064,18.0725497817287));
#25922=CARTESIAN_POINT('Ctrl Pts',(26.5661459570323,-9.08823114221038,18.4072245179962));
#25923=CARTESIAN_POINT('Ctrl Pts',(26.926701682987,-9.23237211346181,18.7237138795475));
#25924=CARTESIAN_POINT('Ctrl Pts',(27.1778777840906,-9.33278590406893,18.9441917645255));
#25925=CARTESIAN_POINT('Ctrl Pts',(27.4154861117667,-9.43401273576512,19.1558005177924));
#25926=CARTESIAN_POINT('Ctrl Pts',(27.6422281940404,-9.53441411056212,19.3606119911674));
#25927=CARTESIAN_POINT('Ctrl Pts',(27.8555559931963,-9.62887564193249,19.5533066176737));
#25928=CARTESIAN_POINT('Ctrl Pts',(28.1190837191893,-9.74908876006132,19.7932907122016));
#25929=CARTESIAN_POINT('Ctrl Pts',(28.4603051775662,-9.91225869658421,20.113556154062));
#25930=CARTESIAN_POINT('Ctrl Pts',(28.6017730832374,-9.97990775153573,20.2463358494959));
#25931=CARTESIAN_POINT('Ctrl Pts',(28.7540286646365,-10.0537371137307,20.39064884571));
#25932=CARTESIAN_POINT('Ctrl Pts',(28.9157341130969,-10.1329641969115,20.5460712531062));
#25933=CARTESIAN_POINT('Ctrl Pts',(29.4787137469323,-10.4087943232527,21.0871763972981));
#25934=CARTESIAN_POINT('Ctrl Pts',(30.1711677436376,-10.7903831220537,21.7690303052012));
#25935=CARTESIAN_POINT('Ctrl Pts',(30.8055547543695,-11.1662968083083,22.4074085008994));
#25936=CARTESIAN_POINT('Ctrl Pts',(31.189312564438,-11.3936971342473,22.7935806863828));
#25937=CARTESIAN_POINT('Ctrl Pts',(31.5650207099004,-11.6240165648507,23.1758363977026));
#25938=CARTESIAN_POINT('Ctrl Pts',(31.9311744366508,-11.8486051370605,23.5500390710467));
#25939=CARTESIAN_POINT('Ctrl Pts',(32.114251300026,-11.9608994231654,23.7371404077187));
#25940=CARTESIAN_POINT('Ctrl Pts',(32.2949430642606,-12.0717550081779,23.9222292788013));
#25941=CARTESIAN_POINT('Ctrl Pts',(32.4730466959723,-12.1800883327803,24.1048054742076));
#25942=CARTESIAN_POINT('Ctrl Pts',(32.5932788659641,-12.2532207589651,24.2280569315282));
#25943=CARTESIAN_POINT('Ctrl Pts',(32.7123311760732,-12.3252038159362,24.3501636283207));
#25944=CARTESIAN_POINT('Ctrl Pts',(32.8301302693208,-12.3957125289927,24.4709770144495));
#25945=CARTESIAN_POINT('Ctrl Pts',(32.8868306159583,-12.4296505531409,24.5291282334708));
#25946=CARTESIAN_POINT('Ctrl Pts',(32.9387123022541,-12.4605679274042,24.5823367414274));
#25947=CARTESIAN_POINT('Ctrl Pts',(33.,-12.4968515080772,24.6451817466334));
#25948=CARTESIAN_POINT('Ctrl Pts',(33.0955022515283,-12.5533908100124,24.7431106902098));
#25949=CARTESIAN_POINT('Ctrl Pts',(33.2417478451817,-12.6397562375262,24.8926999986811));
#25950=CARTESIAN_POINT('Ctrl Pts',(33.3688392456272,-12.7143924591378,25.0219737265972));
#25951=CARTESIAN_POINT('Ctrl Pts',(34.2661932188391,-13.2413762658613,25.9347364546084));
#25952=CARTESIAN_POINT('Ctrl Pts',(35.2319960544065,-13.7914450400007,26.8874835190751));
#25953=CARTESIAN_POINT('Ctrl Pts',(36.3004607335293,-14.321033230354,27.8047571718553));
#25954=CARTESIAN_POINT('Ctrl Pts',(36.6891719088346,-14.5136992603336,28.1384645246727));
#25955=CARTESIAN_POINT('Ctrl Pts',(37.0893059759746,-14.702405201685,28.4653128027834));
#25956=CARTESIAN_POINT('Ctrl Pts',(37.5,-14.8835914705078,28.7791366260183));
#25957=CARTESIAN_POINT('',(37.5,-12.7626735386834,29.7804325714888));
#25958=CARTESIAN_POINT('Origin',(37.5,0.,0.));
#25959=CARTESIAN_POINT('',(36.8,-11.7911930472672,29.4900464626661));
#25960=CARTESIAN_POINT('Ctrl Pts',(37.5,-12.7626735386834,29.7804325714888));
#25961=CARTESIAN_POINT('Ctrl Pts',(37.2470086540956,-12.4586565616162,29.6681218786625));
#25962=CARTESIAN_POINT('Ctrl Pts',(37.0122659037829,-12.1341821953297,29.5692859507915));
#25963=CARTESIAN_POINT('Ctrl Pts',(36.8,-11.7911930472673,29.4900464626661));
#25964=CARTESIAN_POINT('',(36.8,-4.53355051147314,31.4347259190859));
#25965=CARTESIAN_POINT('Ctrl Pts',(36.8,-11.7911930472672,29.4900464626661));
#25966=CARTESIAN_POINT('Ctrl Pts',(36.8,-9.4561105348841,30.4236973716148));
#25967=CARTESIAN_POINT('Ctrl Pts',(36.8,-7.0196747094175,31.0761743714061));
#25968=CARTESIAN_POINT('Ctrl Pts',(36.8,-4.53355051147314,31.4347259190859));
#25969=CARTESIAN_POINT('',(37.5,-3.83741678103714,32.1719479119405));
#25970=CARTESIAN_POINT('Ctrl Pts',(36.8,-4.53355051147314,31.4347259190859));
#25971=CARTESIAN_POINT('Ctrl Pts',(37.0122659037829,-4.27613294009141,31.6748439028166));
#25972=CARTESIAN_POINT('Ctrl Pts',(37.2470086540955,-4.04454785994598,31.9226755103027));
#25973=CARTESIAN_POINT('Ctrl Pts',(37.5,-3.83741678103716,32.1719479119405));
#25974=CARTESIAN_POINT('',(37.5,-1.5,32.3652591523689));
#25975=CARTESIAN_POINT('Origin',(37.5,0.,0.));
#25976=CARTESIAN_POINT('',(6.9,-8.44145532612415,7.09789564133157));
#25977=CARTESIAN_POINT('Ctrl Pts',(37.5,-1.5,32.3652591523689));
#25978=CARTESIAN_POINT('Ctrl Pts',(36.6490696321448,-1.5,31.6144476510545));
#25979=CARTESIAN_POINT('Ctrl Pts',(35.840653780102,-1.5,30.7967681970102));
#25980=CARTESIAN_POINT('Ctrl Pts',(35.0774452370729,-1.5,29.9676650395079));
#25981=CARTESIAN_POINT('Ctrl Pts',(34.6958409655584,-1.5,29.5531134607568));
#25982=CARTESIAN_POINT('Ctrl Pts',(34.325525504186,-1.5,29.1357262196526));
#25983=CARTESIAN_POINT('Ctrl Pts',(33.9666810635498,-1.5,28.7225756062041));
#25984=CARTESIAN_POINT('Ctrl Pts',(33.7186145566569,-1.5,28.4369676438316));
#25985=CARTESIAN_POINT('Ctrl Pts',(33.4671024168784,-1.5,28.1428784519232));
#25986=CARTESIAN_POINT('Ctrl Pts',(33.2400985609418,-1.5,27.8754055139448));
#25987=CARTESIAN_POINT('Ctrl Pts',(33.13872647961,-1.5,27.7559613383782));
#25988=CARTESIAN_POINT('Ctrl Pts',(33.0532004124147,-1.5,27.65477070954));
#25989=CARTESIAN_POINT('Ctrl Pts',(33.,-1.5,27.5917792275077));
#25990=CARTESIAN_POINT('Ctrl Pts',(32.9185691495555,-1.5,27.4953617427583));
#25991=CARTESIAN_POINT('Ctrl Pts',(32.8516820632662,-1.4997338569914,27.4160082740758));
#25992=CARTESIAN_POINT('Ctrl Pts',(32.7777321455096,-1.49925158146269,27.3281857858092));
#25993=CARTESIAN_POINT('Ctrl Pts',(32.1788699539487,-1.49534601146588,26.6169805622313));
#25994=CARTESIAN_POINT('Ctrl Pts',(31.5692879871054,-1.47697823247432,25.8863210200298));
#25995=CARTESIAN_POINT('Ctrl Pts',(30.9513498040414,-1.4685839644322,25.1628991372544));
#25996=CARTESIAN_POINT('Ctrl Pts',(30.6423807125094,-1.46438683041114,24.8011881958668));
#25997=CARTESIAN_POINT('Ctrl Pts',(30.3347880606899,-1.46274142297322,24.4452439233219));
#25998=CARTESIAN_POINT('Ctrl Pts',(30.024930637178,-1.46654496784342,24.0928170619159));
#25999=CARTESIAN_POINT('Ctrl Pts',(29.870001925422,-1.46844674027852,23.9166036312129));
#26000=CARTESIAN_POINT('Ctrl Pts',(29.7145097313437,-1.47171272534115,23.7412668049772));
#26001=CARTESIAN_POINT('Ctrl Pts',(29.558010072041,-1.47674445496737,23.5665148172495));
#26002=CARTESIAN_POINT('Ctrl Pts',(29.4797602423896,-1.47926031978048,23.4791388233857));
#26003=CARTESIAN_POINT('Ctrl Pts',(29.4012586241187,-1.48221825336153,23.3919089755765));
#26004=CARTESIAN_POINT('Ctrl Pts',(29.322450242048,-1.48567308535868,23.3047886331029));
#26005=CARTESIAN_POINT('Ctrl Pts',(29.2736528205962,-1.48781228538512,23.2508445226287));
#26006=CARTESIAN_POINT('Ctrl Pts',(29.2247377936956,-1.4901420619451,23.1969423954499));
#26007=CARTESIAN_POINT('Ctrl Pts',(29.1756921969113,-1.49267616691569,23.1430735687309));
#26008=CARTESIAN_POINT('Ctrl Pts',(29.145528605684,-1.49423466984912,23.1099436370839));
#26009=CARTESIAN_POINT('Ctrl Pts',(29.1181490968213,-1.49570957236866,23.0799256031418));
#26010=CARTESIAN_POINT('Ctrl Pts',(29.0849408699094,-1.4975930851266,23.0435998794277));
#26011=CARTESIAN_POINT('Ctrl Pts',(29.0475462331498,-1.49971404375539,23.0026947372493));
#26012=CARTESIAN_POINT('Ctrl Pts',(28.9599837408025,-1.50462371438853,22.9072087348165));
#26013=CARTESIAN_POINT('Ctrl Pts',(28.8924081847867,-1.50836890093464,22.8339936859735));
#26014=CARTESIAN_POINT('Ctrl Pts',(28.4410807635146,-1.53338246331873,22.3450009030674));
#26015=CARTESIAN_POINT('Ctrl Pts',(27.9936088567427,-1.55654582153956,21.8761056063188));
#26016=CARTESIAN_POINT('Ctrl Pts',(27.5122543095517,-1.59544751495705,21.391301016406));
#26017=CARTESIAN_POINT('Ctrl Pts',(27.1397294106107,-1.62555390845339,21.0161060963261));
#26018=CARTESIAN_POINT('Ctrl Pts',(26.7276341641016,-1.66499152476168,20.6120596829205));
#26019=CARTESIAN_POINT('Ctrl Pts',(26.2530417505368,-1.74041895661093,20.1649482705455));
#26020=CARTESIAN_POINT('Ctrl Pts',(25.8694949138819,-1.80137642675986,19.8036104932291));
#26021=CARTESIAN_POINT('Ctrl Pts',(25.4447383161056,-1.88186126749416,19.4141244720056));
#26022=CARTESIAN_POINT('Ctrl Pts',(24.9635886608287,-1.98732702259654,18.9908103209264));
#26023=CARTESIAN_POINT('Ctrl Pts',(24.6119820459616,-2.06439754884394,18.6814677825833));
#26024=CARTESIAN_POINT('Ctrl Pts',(24.2873626786293,-2.13832395595953,18.3974053120239));
#26025=CARTESIAN_POINT('Ctrl Pts',(23.6426616419432,-2.30363857154125,17.8679904517678));
#26026=CARTESIAN_POINT('Ctrl Pts',(23.5760533212753,-2.3207183159486,17.8132931071512));
#26027=CARTESIAN_POINT('Ctrl Pts',(23.506596730581,-2.3386695571242,17.7565376998347));
#26028=CARTESIAN_POINT('Ctrl Pts',(23.4342591639586,-2.3575237071575,17.697767866208));
#26029=CARTESIAN_POINT('Ctrl Pts',(22.7443384436212,-2.53734547031163,17.1372496203914));
#26030=CARTESIAN_POINT('Ctrl Pts',(21.7987837593118,-2.82220391184419,16.3936354357679));
#26031=CARTESIAN_POINT('Ctrl Pts',(20.5610365528855,-3.2211816912596,15.5107287130397));
#26032=CARTESIAN_POINT('Ctrl Pts',(19.7234582214102,-3.49116827740858,14.9132694452414));
#26033=CARTESIAN_POINT('Ctrl Pts',(18.7603809281622,-3.83806571370471,14.2521506387675));
#26034=CARTESIAN_POINT('Ctrl Pts',(17.6514222906382,-4.23400473904287,13.5382422374622));
#26035=CARTESIAN_POINT('Ctrl Pts',(16.7565277906387,-4.55351499318673,12.9621407669349));
#26036=CARTESIAN_POINT('Ctrl Pts',(15.7613807992389,-4.9385420283955,12.3388737256114));
#26037=CARTESIAN_POINT('Ctrl Pts',(14.7199652846762,-5.32978309078145,11.7149311743306));
#26038=CARTESIAN_POINT('Ctrl Pts',(13.7316067501733,-5.70109160083332,11.1227766145274));
#26039=CARTESIAN_POINT('Ctrl Pts',(12.7260968661244,-6.10453604902481,10.5273020287043));
#26040=CARTESIAN_POINT('Ctrl Pts',(11.7781012037546,-6.47234380217571,9.9794168301694));
#26041=CARTESIAN_POINT('Ctrl Pts',(10.6475718363526,-6.91097182865411,9.3260379894265));
#26042=CARTESIAN_POINT('Ctrl Pts',(9.62260863652896,-7.33414209133677,8.72329062200735));
#26043=CARTESIAN_POINT('Ctrl Pts',(8.83596460437641,-7.64982933055118,8.26196206072778));
#26044=CARTESIAN_POINT('Ctrl Pts',(8.38131550044836,-7.83228405538728,7.99533241831094));
#26045=CARTESIAN_POINT('Ctrl Pts',(7.99969688490427,-7.98693286596967,7.76911080499221));
#26046=CARTESIAN_POINT('Ctrl Pts',(7.59379043301555,-8.15376232311827,7.52350537407495));
#26047=CARTESIAN_POINT('Ctrl Pts',(7.36145773430845,-8.24925215291236,7.38292575944549));
#26048=CARTESIAN_POINT('Ctrl Pts',(7.13004605045667,-8.34517464654889,7.24116906982207));
#26049=CARTESIAN_POINT('Ctrl Pts',(6.9,-8.44145532612415,7.09789564133157));
#26050=CARTESIAN_POINT('',(6.9,-5.6597919716369,9.46599415782505));
#26051=CARTESIAN_POINT('Ctrl Pts',(6.90000000000001,-8.44145532612415,7.09789564133157));
#26052=CARTESIAN_POINT('Ctrl Pts',(6.90000000000001,-8.09681826844945,7.5077690000137));
#26053=CARTESIAN_POINT('Ctrl Pts',(6.90000000000001,-7.72210951819363,7.89280389060837));
#26054=CARTESIAN_POINT('Ctrl Pts',(6.90000000000001,-6.80464666682922,8.70687723936702));
#26055=CARTESIAN_POINT('Ctrl Pts',(6.90000000000001,-6.24868352466685,9.11389129061078));
#26056=CARTESIAN_POINT('Ctrl Pts',(6.90000000000001,-5.6597919716369,9.46599415782505));
#26057=CARTESIAN_POINT('',(37.5,1.5,32.3652591523689));
#26058=CARTESIAN_POINT('Ctrl Pts',(6.9,-5.6597919716369,9.46599415782505));
#26059=CARTESIAN_POINT('Ctrl Pts',(6.98893730997566,-5.61299197171187,9.50231572683753));
#26060=CARTESIAN_POINT('Ctrl Pts',(7.08052892388252,-5.56508220248504,9.53955640247964));
#26061=CARTESIAN_POINT('Ctrl Pts',(7.17490192378012,-5.51603067891051,9.57777162403489));
#26062=CARTESIAN_POINT('Ctrl Pts',(7.97363347620239,-5.10088016323476,9.90120844677132));
#26063=CARTESIAN_POINT('Ctrl Pts',(8.96286060501197,-4.58706675347826,10.2954119066179));
#26064=CARTESIAN_POINT('Ctrl Pts',(10.2403127965964,-4.0024828296383,10.8024441000946));
#26065=CARTESIAN_POINT('Ctrl Pts',(10.4394276407768,-3.91136447885181,10.8814745615582));
#26066=CARTESIAN_POINT('Ctrl Pts',(10.6449386760841,-3.81760465493997,10.9636620301547));
#26067=CARTESIAN_POINT('Ctrl Pts',(10.8572270226697,-3.72139879136416,11.0492678117694));
#26068=CARTESIAN_POINT('Ctrl Pts',(11.0079272576165,-3.65310372723407,11.1100380406097));
#26069=CARTESIAN_POINT('Ctrl Pts',(11.2445718661728,-3.54599023605203,11.2057391107691));
#26070=CARTESIAN_POINT('Ctrl Pts',(11.5512244264283,-3.40956688332716,11.3315975141146));
#26071=CARTESIAN_POINT('Ctrl Pts',(12.0044642694228,-3.20792989416164,11.5176192545635));
#26072=CARTESIAN_POINT('Ctrl Pts',(12.6082461582821,-2.94281490472512,11.7683139215994));
#26073=CARTESIAN_POINT('Ctrl Pts',(13.3027146141536,-2.65901005153359,12.0682094443783));
#26074=CARTESIAN_POINT('Ctrl Pts',(14.2466220417723,-2.27326825627017,12.4758213511068));
#26075=CARTESIAN_POINT('Ctrl Pts',(15.3788107202037,-1.8146998161318,12.9964429751969));
#26076=CARTESIAN_POINT('Ctrl Pts',(16.3720853361384,-1.45099516743194,13.4908337691235));
#26077=CARTESIAN_POINT('Ctrl Pts',(17.5300464833461,-1.02698770212797,14.0671953530399));
#26078=CARTESIAN_POINT('Ctrl Pts',(18.5522571217465,-0.660939172704794,
14.6297459826154));
#26079=CARTESIAN_POINT('Ctrl Pts',(19.459740928474,-0.371242885073753,15.1671394203612));
#26080=CARTESIAN_POINT('Ctrl Pts',(20.7212139011928,0.0314574545183544,
15.914158036459));
#26081=CARTESIAN_POINT('Ctrl Pts',(21.7483180915019,0.336055810070734,16.6062803213401));
#26082=CARTESIAN_POINT('Ctrl Pts',(22.5801692622301,0.547760951425958,17.2054151585246));
#26083=CARTESIAN_POINT('Ctrl Pts',(23.3330995247656,0.739380814773852,17.747707777841));
#26084=CARTESIAN_POINT('Ctrl Pts',(23.9217876539922,0.875119715010134,18.2069050147382));
#26085=CARTESIAN_POINT('Ctrl Pts',(24.4822919859555,0.991018194513003,18.6643830131721));
#26086=CARTESIAN_POINT('Ctrl Pts',(24.9418792866488,1.08604951953881,19.039493545664));
#26087=CARTESIAN_POINT('Ctrl Pts',(25.3626276504437,1.16248493476306,19.3999270896812));
#26088=CARTESIAN_POINT('Ctrl Pts',(25.7525302890144,1.22321331868058,19.7463071016619));
#26089=CARTESIAN_POINT('Ctrl Pts',(26.1776080055513,1.2894203155331,20.1239357965756));
#26090=CARTESIAN_POINT('Ctrl Pts',(26.5661459570286,1.33297321437855,20.4852396168503));
#26091=CARTESIAN_POINT('Ctrl Pts',(26.9267016829778,1.36638815232393,20.8313979296014));
#26092=CARTESIAN_POINT('Ctrl Pts',(27.1778777840728,1.38966620125619,21.0725442742603));
#26093=CARTESIAN_POINT('Ctrl Pts',(27.4154861117395,1.40780557009561,21.3064162460911));
#26094=CARTESIAN_POINT('Ctrl Pts',(27.6422281940027,1.42326116563352,21.5339888724078));
#26095=CARTESIAN_POINT('Ctrl Pts',(27.8555559931731,1.43780239304073,21.7480980798342));
#26096=CARTESIAN_POINT('Ctrl Pts',(28.1190837191602,1.45368682613675,22.0160369612575));
#26097=CARTESIAN_POINT('Ctrl Pts',(28.4603051775547,1.47251023690518,22.3749799381424));
#26098=CARTESIAN_POINT('Ctrl Pts',(28.6017730832288,1.48031428449229,22.5237950549738));
#26099=CARTESIAN_POINT('Ctrl Pts',(28.7540286646318,1.48853267939352,22.685688456893));
#26100=CARTESIAN_POINT('Ctrl Pts',(28.9157341130969,1.49763121638955,22.8599017516109));
#26101=CARTESIAN_POINT('Ctrl Pts',(29.4787137469316,1.52930789194493,23.4664276157693));
#26102=CARTESIAN_POINT('Ctrl Pts',(30.1711677436387,1.53976925233529,24.2477248210855));
#26103=CARTESIAN_POINT('Ctrl Pts',(30.8055547543725,1.53340754825755,24.9885333989119));
#26104=CARTESIAN_POINT('Ctrl Pts',(31.1893125644404,1.52955918190726,25.4366684847443));
#26105=CARTESIAN_POINT('Ctrl Pts',(31.5650207099025,1.5212245596794,25.8828713567903));
#26106=CARTESIAN_POINT('Ctrl Pts',(31.9311744366524,1.51382648741807,26.3192346641747));
#26107=CARTESIAN_POINT('Ctrl Pts',(32.1142513000274,1.51012745128741,26.5374163178669));
#26108=CARTESIAN_POINT('Ctrl Pts',(32.2949430642618,1.50666813405657,26.7531357746881));
#26109=CARTESIAN_POINT('Ctrl Pts',(32.4730466959732,1.50413682057757,26.9654180603372));
#26110=CARTESIAN_POINT('Ctrl Pts',(32.5932788659586,1.50242801032161,27.108723166515));
#26111=CARTESIAN_POINT('Ctrl Pts',(32.7123311760612,1.50114220273881,27.2504621963874));
#26112=CARTESIAN_POINT('Ctrl Pts',(32.8301302693026,1.50048655910809,27.390344014413));
#26113=CARTESIAN_POINT('Ctrl Pts',(32.8868306159462,1.50017097755213,27.4576734594278));
#26114=CARTESIAN_POINT('Ctrl Pts',(32.9387123022461,1.5,27.5192120661523));
#26115=CARTESIAN_POINT('Ctrl Pts',(33.,1.5,27.5917792275077));
#26116=CARTESIAN_POINT('Ctrl Pts',(33.0955022515303,1.5,27.7048578313807));
#26117=CARTESIAN_POINT('Ctrl Pts',(33.2417478451704,1.5,27.8775886863925));
#26118=CARTESIAN_POINT('Ctrl Pts',(33.3688392456061,1.5,28.026861129604));
#26119=CARTESIAN_POINT('Ctrl Pts',(34.266193218791,1.5,29.08082874302));
#26120=CARTESIAN_POINT('Ctrl Pts',(35.2319960543154,1.5,30.1809662912516));
#26121=CARTESIAN_POINT('Ctrl Pts',(36.3004607333866,1.5,31.2401426719198));
#26122=CARTESIAN_POINT('Ctrl Pts',(36.689171908737,1.5,31.6254747319285));
#26123=CARTESIAN_POINT('Ctrl Pts',(37.0893059759246,1.5,32.0028866146793));
#26124=CARTESIAN_POINT('Ctrl Pts',(37.5,1.5,32.3652591523689));
#26125=CARTESIAN_POINT('',(37.5,3.83741678103715,32.1719479119405));
#26126=CARTESIAN_POINT('Origin',(37.5,0.,0.));
#26127=CARTESIAN_POINT('',(36.8,4.53355051147315,31.4347259190859));
#26128=CARTESIAN_POINT('Ctrl Pts',(37.5,3.83741678103717,32.1719479119405));
#26129=CARTESIAN_POINT('Ctrl Pts',(37.2470086540956,4.04454785994596,31.9226755103027));
#26130=CARTESIAN_POINT('Ctrl Pts',(37.0122659037829,4.27613294009139,31.6748439028166));
#26131=CARTESIAN_POINT('Ctrl Pts',(36.8,4.53355051147315,31.4347259190859));
#26132=CARTESIAN_POINT('',(36.8,11.7911930472673,29.4900464626661));
#26133=CARTESIAN_POINT('Ctrl Pts',(36.8,4.53355051147315,31.4347259190859));
#26134=CARTESIAN_POINT('Ctrl Pts',(36.8,6.18280168905531,31.1968691126063));
#26135=CARTESIAN_POINT('Ctrl Pts',(36.8,7.81258162569765,30.8293258095436));
#26136=CARTESIAN_POINT('Ctrl Pts',(36.8,10.2137688485759,30.0846548283827));
#26137=CARTESIAN_POINT('Ctrl Pts',(36.8,11.0089139056503,29.8028301128151));
#26138=CARTESIAN_POINT('Ctrl Pts',(36.8,11.7911930472673,29.4900464626661));
#26139=CARTESIAN_POINT('',(37.5,12.7626735386834,29.7804325714888));
#26140=CARTESIAN_POINT('Ctrl Pts',(36.8,11.7911930472673,29.4900464626661));
#26141=CARTESIAN_POINT('Ctrl Pts',(37.0122659037828,12.1341821953296,29.5692859507915));
#26142=CARTESIAN_POINT('Ctrl Pts',(37.2470086540956,12.4586565616162,29.6681218786625));
#26143=CARTESIAN_POINT('Ctrl Pts',(37.5,12.7626735386834,29.7804325714888));
#26144=CARTESIAN_POINT('',(37.5,14.8835914705078,28.7791366260183));
#26145=CARTESIAN_POINT('Origin',(37.5,0.,0.));
#26146=CARTESIAN_POINT('',(6.9,-3.76156693666918,10.3676856018661));
#26147=CARTESIAN_POINT('Ctrl Pts',(37.5,14.8835914705078,28.7791366260183));
#26148=CARTESIAN_POINT('Ctrl Pts',(36.6490696321541,14.5081857198547,28.1289147924336));
#26149=CARTESIAN_POINT('Ctrl Pts',(35.8406537801186,14.0993459928369,27.4207836130862));
#26150=CARTESIAN_POINT('Ctrl Pts',(35.0774452370931,13.6847944140883,26.7027592163357));
#26151=CARTESIAN_POINT('Ctrl Pts',(34.6958409655804,13.4775186247139,26.3437470179604));
#26152=CARTESIAN_POINT('Ctrl Pts',(34.3255255042089,13.2688250041626,25.98227906395));
#26153=CARTESIAN_POINT('Ctrl Pts',(33.9666810635723,13.0622496974384,25.6244801371145));
#26154=CARTESIAN_POINT('Ctrl Pts',(33.71861455668,12.9194457162525,25.3771363861775));
#26155=CARTESIAN_POINT('Ctrl Pts',(33.467102416908,12.7724011203023,25.1224476750133));
#26156=CARTESIAN_POINT('Ctrl Pts',(33.2400985609625,12.638664651308,24.8908093158902));
#26157=CARTESIAN_POINT('Ctrl Pts',(33.1387264796258,12.5789425635218,24.7873676255104));
#26158=CARTESIAN_POINT('Ctrl Pts',(33.0532004124213,12.5283472490973,24.6997339703023));
#26159=CARTESIAN_POINT('Ctrl Pts',(33.,12.4968515080772,24.6451817466334));
#26160=CARTESIAN_POINT('Ctrl Pts',(32.9185691495566,12.4486427657032,24.5616817554726));
#26161=CARTESIAN_POINT('Ctrl Pts',(32.8516820632524,12.4091965179596,24.4928265641956));
#26162=CARTESIAN_POINT('Ctrl Pts',(32.7777321454818,12.3657029366776,24.4165289205543));
#26163=CARTESIAN_POINT('Ctrl Pts',(32.178869953925,12.0134826477248,23.7986543446369));
#26164=CARTESIAN_POINT('Ctrl Pts',(31.5692879870854,11.664059839844,23.1567007300813));
#26165=CARTESIAN_POINT('Ctrl Pts',(30.9513498040256,11.3096185478294,22.5260018679279));
#26166=CARTESIAN_POINT('Ctrl Pts',(30.6423807124957,11.1323979018221,22.2106524368512));
#26167=CARTESIAN_POINT('Ctrl Pts',(30.3347880606787,10.9558507301919,21.9015729507795));
#26168=CARTESIAN_POINT('Ctrl Pts',(30.0249306371694,10.7763433330083,21.5982641082636));
#26169=CARTESIAN_POINT('Ctrl Pts',(29.8700019254147,10.6865896344165,21.4466096870056));
#26170=CARTESIAN_POINT('Ctrl Pts',(29.7145097313378,10.5960927952669,21.2963965337993));
#26171=CARTESIAN_POINT('Ctrl Pts',(29.5580100720363,10.5043591957225,21.1475727378798));
#26172=CARTESIAN_POINT('Ctrl Pts',(29.4797602423856,10.4584923959504,21.07316083992));
#26173=CARTESIAN_POINT('Ctrl Pts',(29.4012586241155,10.4123158264222,20.9990965425402));
#26174=CARTESIAN_POINT('Ctrl Pts',(29.3224502420455,10.3657636829105,20.9253755287709));
#26175=CARTESIAN_POINT('Ctrl Pts',(29.2736528206492,10.3369390261396,20.8797281587809));
#26176=CARTESIAN_POINT('Ctrl Pts',(29.2247377938045,10.3079703168972,20.8342124356577));
#26177=CARTESIAN_POINT('Ctrl Pts',(29.1756921970763,10.2788413042909,20.7888277157836));
#26178=CARTESIAN_POINT('Ctrl Pts',(29.145528605794,10.2609266353026,20.7609156047673));
#26179=CARTESIAN_POINT('Ctrl Pts',(29.1181490968819,10.2446403152522,20.7356566760157));
#26180=CARTESIAN_POINT('Ctrl Pts',(29.0849408699094,10.2248462834623,20.7051394327917));
#26181=CARTESIAN_POINT('Ctrl Pts',(29.0475462332256,10.2025569083654,20.6707750199039));
#26182=CARTESIAN_POINT('Ctrl Pts',(28.9599837408864,10.150562007661,20.5905365514149));
#26183=CARTESIAN_POINT('Ctrl Pts',(28.8924081848889,10.1107110565592,20.529003052467));
#26184=CARTESIAN_POINT('Ctrl Pts',(28.4410807636115,9.84455228463784,20.1180296613881));
#26185=CARTESIAN_POINT('Ctrl Pts',(27.9936088568352,9.59004457960431,19.7235361017932));
#26186=CARTESIAN_POINT('Ctrl Pts',(27.5122543096508,9.31395242990228,19.3231338577684));
#26187=CARTESIAN_POINT('Ctrl Pts',(27.1397294106844,9.10028206826387,19.0132587223329));
#26188=CARTESIAN_POINT('Ctrl Pts',(26.7276341641442,8.86410488395679,18.6830630721424));
#26189=CARTESIAN_POINT('Ctrl Pts',(26.2530417505368,8.57522710561967,18.3335669465969));
#26190=CARTESIAN_POINT('Ctrl Pts',(25.8694949138829,8.34176749926266,18.0511179871691));
#26191=CARTESIAN_POINT('Ctrl Pts',(25.4447383161075,8.07732257195607,17.7540556187384));
#26192=CARTESIAN_POINT('Ctrl Pts',(24.9635886608316,7.77432947326916,17.4401876876742));
#26193=CARTESIAN_POINT('Ctrl Pts',(24.6119820459567,7.55291317047937,17.2108244541163));
#26194=CARTESIAN_POINT('Ctrl Pts',(24.2873626786171,7.34685978862235,17.001782341903));
#26195=CARTESIAN_POINT('Ctrl Pts',(23.6426616419067,6.93898570176839,16.625952931558));
#26196=CARTESIAN_POINT('Ctrl Pts',(23.5760533212499,6.89684553692024,16.5871235138108));
#26197=CARTESIAN_POINT('Ctrl Pts',(23.5065967305678,6.85292160238213,16.5469475098675));
#26198=CARTESIAN_POINT('Ctrl Pts',(23.4342591639586,6.80720851268154,16.5054784159948));
#26199=CARTESIAN_POINT('Ctrl Pts',(22.7443384436217,6.37121917472878,16.1099662574103));
#26200=CARTESIAN_POINT('Ctrl Pts',(21.7987837593123,5.75271743556738,15.6084067036781));
#26201=CARTESIAN_POINT('Ctrl Pts',(20.5610365528855,4.96573918168373,15.0432759423309));
#26202=CARTESIAN_POINT('Ctrl Pts',(19.7234582214102,4.43319430549857,14.6608543317656));
#26203=CARTESIAN_POINT('Ctrl Pts',(18.7603809281623,3.80221290992149,14.2617573685877));
#26204=CARTESIAN_POINT('Ctrl Pts',(17.6514222906382,3.10236545497629,13.8414640697512));
#26205=CARTESIAN_POINT('Ctrl Pts',(16.7565277906387,2.53761072285442,13.5023006881889));
#26206=CARTESIAN_POINT('Ctrl Pts',(15.7613807992389,1.89253400855812,13.1550491146656));
#26207=CARTESIAN_POINT('Ctrl Pts',(14.7199652846762,1.2417380338878,12.8103195459473));
#26208=CARTESIAN_POINT('Ctrl Pts',(13.7316067501733,0.624098151639976,12.4831529092169));
#26209=CARTESIAN_POINT('Ctrl Pts',(12.7260968661244,-0.0230322824212142,
12.1691790146818));
#26210=CARTESIAN_POINT('Ctrl Pts',(11.7781012037546,-0.615505739626224,
11.8786003909685));
#26211=CARTESIAN_POINT('Ctrl Pts',(10.6475718363527,-1.32205817373976,11.5320717298292));
#26212=CARTESIAN_POINT('Ctrl Pts',(9.62260863652904,-1.98990805505865,11.2216623289213));
#26213=CARTESIAN_POINT('Ctrl Pts',(8.83596460437641,-2.49396550450873,10.9799836949691));
#26214=CARTESIAN_POINT('Ctrl Pts',(8.3813155004462,-2.7852907524671,10.8403030136515));
#26215=CARTESIAN_POINT('Ctrl Pts',(7.99969688490053,-3.03233135775691,10.7217137549231));
#26216=CARTESIAN_POINT('Ctrl Pts',(7.59379043301053,-3.29961262120668,10.5924279410152));
#26217=CARTESIAN_POINT('Ctrl Pts',(7.36145773430507,-3.45259904692508,10.5184273383894));
#26218=CARTESIAN_POINT('Ctrl Pts',(7.130046050455,-3.60654870801926,10.4436236908379));
#26219=CARTESIAN_POINT('Ctrl Pts',(6.9,-3.76156693666918,10.3676856018661));
#26220=CARTESIAN_POINT('',(6.9,-0.168526548660249,11.02768739857));
#26221=CARTESIAN_POINT('Ctrl Pts',(6.90000000000001,-3.76156693666918,10.3676856018661));
#26222=CARTESIAN_POINT('Ctrl Pts',(6.90000000000001,-3.24481773355662,10.5551707158657));
#26223=CARTESIAN_POINT('Ctrl Pts',(6.89999999999998,-2.71398840242747,10.7040448708755));
#26224=CARTESIAN_POINT('Ctrl Pts',(6.89999999999998,-1.51153848953113,10.9457448952802));
#26225=CARTESIAN_POINT('Ctrl Pts',(6.90000000000001,-0.840414370027661,
11.0174195217678));
#26226=CARTESIAN_POINT('Ctrl Pts',(6.90000000000001,-0.168526548660249,
11.02768739857));
#26227=CARTESIAN_POINT('',(37.5,17.4816676818611,27.2791366260183));
#26228=CARTESIAN_POINT('Ctrl Pts',(6.9,-0.168526548660249,11.02768739857));
#26229=CARTESIAN_POINT('Ctrl Pts',(6.98893730997575,-0.10983577532176,11.0357428000776));
#26230=CARTESIAN_POINT('Ctrl Pts',(7.08052892388262,-0.0497243602608107,
11.0440392866244));
#26231=CARTESIAN_POINT('Ctrl Pts',(7.17490192378012,0.0118631160266181,
11.0526088775152));
#26232=CARTESIAN_POINT('Ctrl Pts',(7.9736334762095,0.53311242036889,11.1251381246871));
#26233=CARTESIAN_POINT('Ctrl Pts',(8.96286060502258,1.1751896159481,11.2096216302963));
#26234=CARTESIAN_POINT('Ctrl Pts',(10.2403127965964,1.93497024136951,11.3564324284624));
#26235=CARTESIAN_POINT('Ctrl Pts',(10.4394276407766,2.05339627863326,11.3793156403694));
#26236=CARTESIAN_POINT('Ctrl Pts',(10.6449386760836,2.17568840229328,11.4036121640907));
#26237=CARTESIAN_POINT('Ctrl Pts',(10.8572270226685,2.30180801494992,11.4296460138919));
#26238=CARTESIAN_POINT('Ctrl Pts',(11.0079272576413,2.39133838987524,11.4481270437995));
#26239=CARTESIAN_POINT('Ctrl Pts',(11.2445718661931,2.53195192940405,11.4774498561353));
#26240=CARTESIAN_POINT('Ctrl Pts',(11.5512244264873,2.71302722022868,11.5182347543553));
#26241=CARTESIAN_POINT('Ctrl Pts',(12.0044642694683,2.98066084540491,11.5785158126561));
#26242=CARTESIAN_POINT('Ctrl Pts',(12.6082461583042,3.33560449468488,11.6630662681815));
#26243=CARTESIAN_POINT('Ctrl Pts',(13.3027146141536,3.73133446864291,11.7808809827897));
#26244=CARTESIAN_POINT('Ctrl Pts',(14.2466220417547,4.26920261599668,11.9410123512669));
#26245=CARTESIAN_POINT('Ctrl Pts',(15.3788107201888,4.92664534657693,12.1625996834186));
#26246=CARTESIAN_POINT('Ctrl Pts',(16.3720853361384,5.48881820879721,12.4089023460099));
#26247=CARTESIAN_POINT('Ctrl Pts',(17.5300464833439,6.14420023710166,12.6960423867944));
#26248=CARTESIAN_POINT('Ctrl Pts',(18.5522571217461,6.74248287738888,13.0002012582105));
#26249=CARTESIAN_POINT('Ctrl Pts',(19.459740928474,7.26206394073251,13.3207494833101));
#26250=CARTESIAN_POINT('Ctrl Pts',(20.7212139012038,7.98432197298711,13.7663364121585));
#26251=CARTESIAN_POINT('Ctrl Pts',(21.748318091517,8.59417302928943,14.2134327156183));
#26252=CARTESIAN_POINT('Ctrl Pts',(22.5801692622301,9.0770824783983,14.6264461342272));
#26253=CARTESIAN_POINT('Ctrl Pts',(23.3330995247344,9.51417645756738,15.0002753871505));
#26254=CARTESIAN_POINT('Ctrl Pts',(23.9217876538942,9.86132841186279,15.3300824094945));
#26255=CARTESIAN_POINT('Ctrl Pts',(24.4822919858109,10.190438438562,15.668320738026));
#26256=CARTESIAN_POINT('Ctrl Pts',(24.9418792865584,10.4602932464676,15.9456603259067));
#26257=CARTESIAN_POINT('Ctrl Pts',(25.3626276504005,10.7067050298371,16.2195872238184));
#26258=CARTESIAN_POINT('Ctrl Pts',(25.7525302890143,10.9324873590558,16.489196921628));
#26259=CARTESIAN_POINT('Ctrl Pts',(26.1776080055349,11.1786386476857,16.7831294661836));
#26260=CARTESIAN_POINT('Ctrl Pts',(26.566145957002,11.3970084746262,17.0742513035944));
#26261=CARTESIAN_POINT('Ctrl Pts',(26.9267016829466,11.5990258161259,17.357325727191));
#26262=CARTESIAN_POINT('Ctrl Pts',(27.1778854594997,11.7397626706971,17.5545315892759));
#26263=CARTESIAN_POINT('Ctrl Pts',(27.4155006347601,11.8724116206269,17.7480067679658));
#26264=CARTESIAN_POINT('Ctrl Pts',(27.6422489803528,11.9995864201593,17.9373681845217));
#26265=CARTESIAN_POINT('Ctrl Pts',(27.8555706599243,12.1192306970096,18.1155167629388));
#26266=CARTESIAN_POINT('Ctrl Pts',(28.1190985482737,12.2669566516382,18.3396168643542));
#26267=CARTESIAN_POINT('Ctrl Pts',(28.4603120647663,12.462725193046,18.6410520014511));
#26268=CARTESIAN_POINT('Ctrl Pts',(28.6017780250768,12.5438901626918,18.7660259813188));
#26269=CARTESIAN_POINT('Ctrl Pts',(28.7540312887802,12.6319528845963,18.9021185408488));
#26270=CARTESIAN_POINT('Ctrl Pts',(28.9157341130969,12.7269375546994,19.0484400367167));
#26271=CARTESIAN_POINT('Ctrl Pts',(29.4787137469306,13.0576332925164,19.5578685053516));
#26272=CARTESIAN_POINT('Ctrl Pts',(30.1711677436355,13.4573416990294,20.2292610528638));
#26273=CARTESIAN_POINT('Ctrl Pts',(30.805554754367,13.8222365905986,20.8740009526392));
#26274=CARTESIAN_POINT('Ctrl Pts',(31.1893125644359,14.042971350493,21.2640215044733));
#26275=CARTESIAN_POINT('Ctrl Pts',(31.5650207098988,14.2588547919362,21.6546118380215));
#26276=CARTESIAN_POINT('Ctrl Pts',(31.9311744366496,14.4706295271116,22.0362125836274));
#26277=CARTESIAN_POINT('Ctrl Pts',(32.1142513000251,14.5765168946992,22.2270129564303));
#26278=CARTESIAN_POINT('Ctrl Pts',(32.2949430642599,14.6813807665084,22.4155611447439));
#26279=CARTESIAN_POINT('Ctrl Pts',(32.4730466959718,14.7853297275555,22.6006686536295));
#26280=CARTESIAN_POINT('Ctrl Pts',(32.5932788659518,14.8555024075494,22.7256289211939));
#26281=CARTESIAN_POINT('Ctrl Pts',(32.7123311760492,14.9252583804514,22.8490214255572));
#26282=CARTESIAN_POINT('Ctrl Pts',(32.8301302692855,14.9946314854212,22.9704904553051));
#26283=CARTESIAN_POINT('Ctrl Pts',(32.8868306159349,15.0280229062875,23.0289572558946));
#26284=CARTESIAN_POINT('Ctrl Pts',(32.9387123022399,15.0586441387491,23.0823367414128));
#26285=CARTESIAN_POINT('Ctrl Pts',(33.,15.0949277194305,23.1451817466334));
#26286=CARTESIAN_POINT('Ctrl Pts',(33.0955022515224,15.1514670213623,23.2431106902038));
#26287=CARTESIAN_POINT('Ctrl Pts',(33.2417478451566,15.2378324488647,23.3926999986554));
#26288=CARTESIAN_POINT('Ctrl Pts',(33.3688392455861,15.3124686704669,23.5219737265553));
#26289=CARTESIAN_POINT('Ctrl Pts',(34.2661932187784,15.8394524771795,24.4347364545476));
#26290=CARTESIAN_POINT('Ctrl Pts',(35.2319960543174,16.3895212513045,25.3874835189893));
#26291=CARTESIAN_POINT('Ctrl Pts',(36.3004607334107,16.9191094416485,26.3047571717535));
#26292=CARTESIAN_POINT('Ctrl Pts',(36.6891719087532,17.1117754716485,26.6384645246061));
#26293=CARTESIAN_POINT('Ctrl Pts',(37.0893059759329,17.3004814130199,26.9653128027515));
#26294=CARTESIAN_POINT('Ctrl Pts',(37.5,17.4816676818611,27.2791366260183));
#26295=CARTESIAN_POINT('',(37.5,19.4092743732571,25.9430157904517));
#26296=CARTESIAN_POINT('Origin',(37.5,0.,0.));
#26297=CARTESIAN_POINT('',(36.8,19.6435328718186,24.9564959511929));
#26298=CARTESIAN_POINT('Ctrl Pts',(37.5,19.4092743732572,25.9430157904516));
#26299=CARTESIAN_POINT('Ctrl Pts',(37.2470086540956,19.4640189486865,25.6235740187165));
#26300=CARTESIAN_POINT('Ctrl Pts',(37.0122659037829,19.5406617074869,25.2931530107));
#26301=CARTESIAN_POINT('Ctrl Pts',(36.8,19.6435328718186,24.9564959511929));
#26302=CARTESIAN_POINT('',(36.8,24.9564959511929,19.6435328718186));
#26303=CARTESIAN_POINT('Ctrl Pts',(36.8,19.6435328718186,24.9564959511929));
#26304=CARTESIAN_POINT('Ctrl Pts',(36.8,20.2288646216318,24.4957748831848));
#26305=CARTESIAN_POINT('Ctrl Pts',(36.8,20.7984186457787,24.0141222843114));
#26306=CARTESIAN_POINT('Ctrl Pts',(36.8,22.6602579716864,22.3234241559746));
#26307=CARTESIAN_POINT('Ctrl Pts',(36.8,23.8659348286794,21.029056769996));
#26308=CARTESIAN_POINT('Ctrl Pts',(36.8,24.9564959511929,19.6435328718186));
#26309=CARTESIAN_POINT('',(37.5,25.9430157904516,19.4092743732571));
#26310=CARTESIAN_POINT('Ctrl Pts',(36.8,24.9564959511929,19.6435328718186));
#26311=CARTESIAN_POINT('Ctrl Pts',(37.0122659037829,25.2931530107001,19.5406617074869));
#26312=CARTESIAN_POINT('Ctrl Pts',(37.2470086540957,25.6235740187166,19.4640189486865));
#26313=CARTESIAN_POINT('Ctrl Pts',(37.5,25.9430157904516,19.4092743732572));
#26314=CARTESIAN_POINT('',(37.5,27.2791366260183,17.4816676818611));
#26315=CARTESIAN_POINT('Origin',(37.5,0.,0.));
#26316=CARTESIAN_POINT('',(6.9,1.9262302757419,10.8594625780008));
#26317=CARTESIAN_POINT('Ctrl Pts',(37.5,27.2791366260183,17.4816676818611));
#26318=CARTESIAN_POINT('Ctrl Pts',(36.6490696321414,26.6289147924239,17.1062619312024));
#26319=CARTESIAN_POINT('Ctrl Pts',(35.8406537800949,25.9207836130653,16.6974222041782));
#26320=CARTESIAN_POINT('Ctrl Pts',(35.0774452370608,25.2027592163052,16.282870625424));
#26321=CARTESIAN_POINT('Ctrl Pts',(34.6958409655438,24.8437470179252,16.0755948360469));
#26322=CARTESIAN_POINT('Ctrl Pts',(34.3255255041686,24.4822790639105,15.8669012154931));
#26323=CARTESIAN_POINT('Ctrl Pts',(33.9666810635291,24.1244801370714,15.6603259087668));
#26324=CARTESIAN_POINT('Ctrl Pts',(33.718614556656,23.8771363861531,15.5175219275918));
#26325=CARTESIAN_POINT('Ctrl Pts',(33.4671024169005,23.6224476750055,15.3704773316512));
#26326=CARTESIAN_POINT('Ctrl Pts',(33.2400985609757,23.3908093159037,15.2367408626691));
#26327=CARTESIAN_POINT('Ctrl Pts',(33.1387264796202,23.2873676255047,15.1770187748718));
#26328=CARTESIAN_POINT('Ctrl Pts',(33.0532004124066,23.1997339702871,15.1264234604419));
#26329=CARTESIAN_POINT('Ctrl Pts',(33.,23.1451817466334,15.0949277194305));
#26330=CARTESIAN_POINT('Ctrl Pts',(32.9185691495926,23.0616817555095,15.0467189770778));
#26331=CARTESIAN_POINT('Ctrl Pts',(32.8516820633429,22.9930927072969,15.0068117561538));
#26332=CARTESIAN_POINT('Ctrl Pts',(32.7777321456298,22.9172773392435,14.9624828491874));
#26333=CARTESIAN_POINT('Ctrl Pts',(32.1788699540528,22.3033083333026,14.6034979145574));
#26334=CARTESIAN_POINT('Ctrl Pts',(31.5692879871913,21.6797224977148,14.2222611802267));
#26335=CARTESIAN_POINT('Ctrl Pts',(30.9513498041043,21.0574179035752,13.8532805894536));
#26336=CARTESIAN_POINT('Ctrl Pts',(30.6423807125608,20.7462656065053,13.668790294067));
#26337=CARTESIAN_POINT('Ctrl Pts',(30.3347880607311,20.4388315278584,13.4893931931471));
#26338=CARTESIAN_POINT('Ctrl Pts',(30.0249306372092,20.1317191404595,13.31647372892));
#26339=CARTESIAN_POINT('Ctrl Pts',(29.8700019254482,19.9781629467601,13.2300139968064));
#26340=CARTESIAN_POINT('Ctrl Pts',(29.7145097313649,19.8246838084848,13.1451740097183));
#26341=CARTESIAN_POINT('Ctrl Pts',(29.5580100720571,19.6708282829326,13.0621556215329));
#26342=CARTESIAN_POINT('Ctrl Pts',(29.4797602424031,19.5939005201566,13.0206464274402));
#26343=CARTESIAN_POINT('Ctrl Pts',(29.4012586241297,19.5168782891925,12.979593149158));
#26344=CARTESIAN_POINT('Ctrl Pts',(29.3224502420564,19.4397024434229,12.9390249501952));
#26345=CARTESIAN_POINT('Ctrl Pts',(29.2736528205926,19.3919158733428,12.9139054965186));
#26346=CARTESIAN_POINT('Ctrl Pts',(29.2247377936802,19.3440703735961,12.8889720786092));
#26347=CARTESIAN_POINT('Ctrl Pts',(29.1756921968838,19.2961515486883,12.8642322645241));
#26348=CARTESIAN_POINT('Ctrl Pts',(29.1455286056658,19.2666809347989,12.8490170018376));
#26349=CARTESIAN_POINT('Ctrl Pts',(29.1181490968165,19.2399471035866,12.8352852879233));
#26350=CARTESIAN_POINT('Ctrl Pts',(29.0849408699094,19.2075463476651,12.8187535959654));
#26351=CARTESIAN_POINT('Ctrl Pts',(29.0475462331044,19.1710609760345,12.8001378289065));
#26352=CARTESIAN_POINT('Ctrl Pts',(28.9599837408215,19.0859128369681,12.7566467272147));
#26353=CARTESIAN_POINT('Ctrl Pts',(28.8924081848413,19.020634151492,12.7232826295015));
#26354=CARTESIAN_POINT('Ctrl Pts',(28.4410807636646,18.5846471981269,12.5004486185587));
#26355=CARTESIAN_POINT('Ctrl Pts',(27.9936088569637,18.1669902803798,12.2860610268735));
#26356=CARTESIAN_POINT('Ctrl Pts',(27.5122543099026,17.7276863430492,12.0773485867127));
#26357=CARTESIAN_POINT('Ctrl Pts',(27.1397294108722,17.3877048140558,11.91582402821));
#26358=CARTESIAN_POINT('Ctrl Pts',(26.7276341642532,17.018071547485,11.7479547990402));
#26359=CARTESIAN_POINT('Ctrl Pts',(26.2530417505368,16.593147989986,11.5897211649258));
#26360=CARTESIAN_POINT('Ctrl Pts',(25.8694949138879,16.2497415604138,11.461842993969));
#26361=CARTESIAN_POINT('Ctrl Pts',(25.4447383161176,15.8721943512536,11.3368019000542));
#26362=CARTESIAN_POINT('Ctrl Pts',(24.9635886608481,15.4528606650926,11.2164808476639));
#26363=CARTESIAN_POINT('Ctrl Pts',(24.6119820458991,15.146426905221,11.1285546120848));
#26364=CARTESIAN_POINT('Ctrl Pts',(24.2873626784886,14.8634583858271,11.0505455233574));
#26365=CARTESIAN_POINT('Ctrl Pts',(23.6426616415564,14.3223143597134,10.9290047499034));
#26366=CARTESIAN_POINT('Ctrl Pts',(23.5760533210065,14.266405197652,10.9164475701653));
#26367=CARTESIAN_POINT('Ctrl Pts',(23.5065967304411,14.2082779526342,10.9036160974189));
#26368=CARTESIAN_POINT('Ctrl Pts',(23.4342591639586,14.1479547088373,10.8905593535265));
#26369=CARTESIAN_POINT('Ctrl Pts',(22.7443384436269,13.5726207871031,10.766030445664));
#26370=CARTESIAN_POINT('Ctrl Pts',(21.7987837593177,12.7862027918382,10.6409180002013));
#26371=CARTESIAN_POINT('Ctrl Pts',(20.5610365528855,11.8220942510713,10.544989531356));
#26372=CARTESIAN_POINT('Ctrl Pts',(19.7234582214113,11.1696860543579,10.480075139743));
#26373=CARTESIAN_POINT('Ctrl Pts',(18.7603809281633,10.4236916548838,10.4499377288461));
#26374=CARTESIAN_POINT('Ctrl Pts',(17.6514222906382,9.60745933070834,10.4358767824859));
#26375=CARTESIAN_POINT('Ctrl Pts',(16.7565277906389,8.94878569500229,10.4245300440805));
#26376=CARTESIAN_POINT('Ctrl Pts',(15.7613807992389,8.21650708627013,10.4463397170534));
#26377=CARTESIAN_POINT('Ctrl Pts',(14.7199652846762,7.48053645516581,10.4731931404428));
#26378=CARTESIAN_POINT('Ctrl Pts',(13.7316067501733,6.78206130838355,10.4986784628874));
#26379=CARTESIAN_POINT('Ctrl Pts',(12.7260968661244,6.06464296565697,10.5503343111255));
#26380=CARTESIAN_POINT('Ctrl Pts',(11.7781012037546,5.40625658879283,10.5949225697956));
#26381=CARTESIAN_POINT('Ctrl Pts',(10.6475718363527,4.62109990117509,10.6480961631663));
#26382=CARTESIAN_POINT('Ctrl Pts',(9.62260863652905,3.8875202375846,10.713198677066));
#26383=CARTESIAN_POINT('Ctrl Pts',(8.83596460437641,3.33015436441791,10.7559275652365));
#26384=CARTESIAN_POINT('Ctrl Pts',(8.38131550044648,3.00801895826358,10.7806231707768));
#26385=CARTESIAN_POINT('Ctrl Pts',(7.999696884901,2.73478088895225,10.8014421627469));
#26386=CARTESIAN_POINT('Ctrl Pts',(7.59379043301109,2.43866561789527,10.8231179952786));
#26387=CARTESIAN_POINT('Ctrl Pts',(7.36145773430546,2.26917518547593,10.8355248063685));
#26388=CARTESIAN_POINT('Ctrl Pts',(7.13004605045519,2.0984490442885,10.8477177778403));
#26389=CARTESIAN_POINT('Ctrl Pts',(6.9,1.9262302757419,10.8594625780008));
#26390=CARTESIAN_POINT('',(6.9,5.36789542693312,9.63452070648529));
#26391=CARTESIAN_POINT('Ctrl Pts',(6.90000000000001,1.9262302757419,10.8594625780008));
#26392=CARTESIAN_POINT('Ctrl Pts',(6.90000000000001,2.35749364924904,10.7829659225815));
#26393=CARTESIAN_POINT('Ctrl Pts',(6.90000000000001,2.78469328079872,10.6806923192591));
#26394=CARTESIAN_POINT('Ctrl Pts',(6.90000000000001,3.958690010018,10.3240838050858));
#26395=CARTESIAN_POINT('Ctrl Pts',(6.90000000000001,4.68344446130229,10.0158641401962));
#26396=CARTESIAN_POINT('Ctrl Pts',(6.90000000000001,5.36789542693312,9.6345207064853));
#26397=CARTESIAN_POINT('',(37.5,28.7791366260183,14.8835914705078));
#26398=CARTESIAN_POINT('Ctrl Pts',(6.9,5.36789542693312,9.6345207064853));
#26399=CARTESIAN_POINT('Ctrl Pts',(6.98893730997578,5.42275082836583,9.61215150215932));
#26400=CARTESIAN_POINT('Ctrl Pts',(7.08052892388264,5.47895708413941,9.58928076274048));
#26401=CARTESIAN_POINT('Ctrl Pts',(7.17490192378012,5.5365781986047,9.56590850800827));
#26402=CARTESIAN_POINT('Ctrl Pts',(7.97363347621182,6.02425796145741,9.36809602640473));
#26403=CARTESIAN_POINT('Ctrl Pts',(8.96286060502644,6.62255487682508,9.12022229067329));
#26404=CARTESIAN_POINT('Ctrl Pts',(10.2403127965964,7.35394959882411,8.86747385872511));
#26405=CARTESIAN_POINT('Ctrl Pts',(10.4394276407767,7.46795116151759,8.82807828292486));
#26406=CARTESIAN_POINT('Ctrl Pts',(10.6449386760836,7.58600750915056,8.78797362786116));
#26407=CARTESIAN_POINT('Ctrl Pts',(10.8572270226685,7.70824722252718,8.74745979681897));
#26408=CARTESIAN_POINT('Ctrl Pts',(11.0079272576493,7.79502331658132,8.71869965074289));
#26409=CARTESIAN_POINT('Ctrl Pts',(11.2445718661999,7.93145962009647,8.67378718137191));
#26410=CARTESIAN_POINT('Ctrl Pts',(11.551224426506,8.10866787106516,8.61857029390676));
#26411=CARTESIAN_POINT('Ctrl Pts',(12.0044642694828,8.37058591852268,8.53695840917511));
#26412=CARTESIAN_POINT('Ctrl Pts',(12.6082461583112,8.72025136346947,8.43270942692314));
#26413=CARTESIAN_POINT('Ctrl Pts',(13.3027146141536,9.12187093125612,8.33687497573541));
#26414=CARTESIAN_POINT('Ctrl Pts',(14.2466220417493,9.66774409498637,8.20661873510328));
#26415=CARTESIAN_POINT('Ctrl Pts',(15.3788107201844,10.3478998672786,8.06979762861289));
#26416=CARTESIAN_POINT('Ctrl Pts',(16.3720853361384,10.9579071785779,8.00201556032625));
#26417=CARTESIAN_POINT('Ctrl Pts',(17.5300464833445,11.669054684666,7.92299511593705));
#26418=CARTESIAN_POINT('Ctrl Pts',(18.5522571217475,12.3392620855066,7.88726310522634));
#26419=CARTESIAN_POINT('Ctrl Pts',(19.459740928474,12.9495065982363,7.9050754796287));
#26420=CARTESIAN_POINT('Ctrl Pts',(20.7212139012143,13.7977938666874,7.92983606347863));
#26421=CARTESIAN_POINT('Ctrl Pts',(21.7483180915291,14.5494885257019,8.01210729206323));
#26422=CARTESIAN_POINT('Ctrl Pts',(22.5801692622301,15.1742070856531,8.12833268012627));
#26423=CARTESIAN_POINT('Ctrl Pts',(23.3330995246905,15.7396562018834,8.23353132024499));
#26424=CARTESIAN_POINT('Ctrl Pts',(23.9217876537976,16.2052021244058,8.34557660278196));
#26425=CARTESIAN_POINT('Ctrl Pts',(24.4822919856751,16.6593389323991,8.47394457446099));
#26426=CARTESIAN_POINT('Ctrl Pts',(24.9418792864744,17.0317098453591,8.57920029909639));
#26427=CARTESIAN_POINT('Ctrl Pts',(25.3626276503609,17.3820721585412,8.69322205979346));
#26428=CARTESIAN_POINT('Ctrl Pts',(25.7525302890143,17.7124102403086,8.81381974260611));
#26429=CARTESIAN_POINT('Ctrl Pts',(26.177608005523,18.0725497817041,8.94529714887164));
#26430=CARTESIAN_POINT('Ctrl Pts',(26.5661459569821,18.4072245179529,9.08823114219187));
#26431=CARTESIAN_POINT('Ctrl Pts',(26.926701682922,18.7237138794904,9.23237211343583));
#26432=CARTESIAN_POINT('Ctrl Pts',(27.1778777840053,18.9441917644501,9.33278590403371));
#26433=CARTESIAN_POINT('Ctrl Pts',(27.4154861116651,19.1558005177017,9.43401273572152));
#26434=CARTESIAN_POINT('Ctrl Pts',(27.6422281939261,19.3606119910642,9.5344141105115));
#26435=CARTESIAN_POINT('Ctrl Pts',(27.8555559931215,19.5533066176051,9.62887564189806));
#26436=CARTESIAN_POINT('Ctrl Pts',(28.119083719114,19.7932907121314,9.74908876002559));
#26437=CARTESIAN_POINT('Ctrl Pts',(28.460305177545,20.113556154042,9.91225869657406));
#26438=CARTESIAN_POINT('Ctrl Pts',(28.6017730832218,20.2463358494812,9.97990775152821));
#26439=CARTESIAN_POINT('Ctrl Pts',(28.7540286646281,20.390648845702,10.0537371137266));
#26440=CARTESIAN_POINT('Ctrl Pts',(28.9157341130969,20.5460712531062,10.1329641969115));
#26441=CARTESIAN_POINT('Ctrl Pts',(29.4787137469279,21.0871763972938,10.4087943232505));
#26442=CARTESIAN_POINT('Ctrl Pts',(30.1711677436301,21.7690303051937,10.7903831220494));
#26443=CARTESIAN_POINT('Ctrl Pts',(30.8055547543591,22.4074085008889,11.1662968083021));
#26444=CARTESIAN_POINT('Ctrl Pts',(31.1893125644294,22.793580686374,11.393697134242));
#26445=CARTESIAN_POINT('Ctrl Pts',(31.5650207098935,23.1758363976956,11.6240165648465));
#26446=CARTESIAN_POINT('Ctrl Pts',(31.9311744366457,23.5500390710414,11.8486051370574));
#26447=CARTESIAN_POINT('Ctrl Pts',(32.1142513000217,23.7371404077143,11.9608994231628));
#26448=CARTESIAN_POINT('Ctrl Pts',(32.2949430642572,23.9222292787978,12.0717550081758));
#26449=CARTESIAN_POINT('Ctrl Pts',(32.4730466959697,24.1048054742049,12.1800883327787));
#26450=CARTESIAN_POINT('Ctrl Pts',(32.5932788659409,24.2280569315044,12.2532207589509));
#26451=CARTESIAN_POINT('Ctrl Pts',(32.7123311760297,24.3501636282761,12.3252038159099));
#26452=CARTESIAN_POINT('Ctrl Pts',(32.8301302692575,24.4709770143846,12.3957125289548));
#26453=CARTESIAN_POINT('Ctrl Pts',(32.8868306159163,24.5291282334276,12.4296505531158));
#26454=CARTESIAN_POINT('Ctrl Pts',(32.9387123022288,24.5823367414014,12.4605679273892));
#26455=CARTESIAN_POINT('Ctrl Pts',(33.,24.6451817466334,12.4968515080772));
#26456=CARTESIAN_POINT('Ctrl Pts',(33.0955022515085,24.7431106901895,12.5533908100007));
#26457=CARTESIAN_POINT('Ctrl Pts',(33.2417478451339,24.8926999986323,12.6397562374981));
#26458=CARTESIAN_POINT('Ctrl Pts',(33.3688392455532,25.0219737265219,12.7143924590943));
#26459=CARTESIAN_POINT('Ctrl Pts',(34.2661932187446,25.9347364545141,13.2413762658068));
#26460=CARTESIAN_POINT('Ctrl Pts',(35.2319960542717,26.8874835189453,13.7914450399258));
#26461=CARTESIAN_POINT('Ctrl Pts',(36.3004607333495,27.804757171701,14.3210332302649));
#26462=CARTESIAN_POINT('Ctrl Pts',(36.6891719087116,28.1384645245721,14.5136992602756));
#26463=CARTESIAN_POINT('Ctrl Pts',(37.0893059759116,28.4653128027352,14.7024052016572));
#26464=CARTESIAN_POINT('Ctrl Pts',(37.5,28.7791366260183,14.8835914705078));
#26465=CARTESIAN_POINT('',(37.5,29.7804325714888,12.7626735386834));
#26466=CARTESIAN_POINT('Origin',(37.5,0.,0.));
#26467=CARTESIAN_POINT('',(36.8,29.4900464626661,11.7911930472673));
#26468=CARTESIAN_POINT('Ctrl Pts',(37.5,29.7804325714888,12.7626735386834));
#26469=CARTESIAN_POINT('Ctrl Pts',(37.2470086540956,29.6681218786625,12.4586565616162));
#26470=CARTESIAN_POINT('Ctrl Pts',(37.0122659037829,29.5692859507915,12.1341821953297));
#26471=CARTESIAN_POINT('Ctrl Pts',(36.8,29.4900464626661,11.7911930472673));
#26472=CARTESIAN_POINT('',(36.8,31.4347259190859,4.53355051147315));
#26473=CARTESIAN_POINT('Ctrl Pts',(36.8,29.4900464626661,11.7911930472673));
#26474=CARTESIAN_POINT('Ctrl Pts',(36.8,30.4236973716148,9.45611053488411));
#26475=CARTESIAN_POINT('Ctrl Pts',(36.8,31.0761743714062,7.01967470941751));
#26476=CARTESIAN_POINT('Ctrl Pts',(36.8,31.4347259190859,4.53355051147315));
#26477=CARTESIAN_POINT('',(37.5,32.1719479119405,3.83741678103715));
#26478=CARTESIAN_POINT('Ctrl Pts',(36.8,31.4347259190859,4.53355051147314));
#26479=CARTESIAN_POINT('Ctrl Pts',(37.0122659037829,31.6748439028166,4.27613294009139));
#26480=CARTESIAN_POINT('Ctrl Pts',(37.2470086540956,31.9226755103027,4.04454785994593));
#26481=CARTESIAN_POINT('Ctrl Pts',(37.5,32.1719479119405,3.83741678103717));
#26482=CARTESIAN_POINT('',(37.5,32.3652591523689,1.5));
#26483=CARTESIAN_POINT('Origin',(37.5,0.,0.));
#26484=CARTESIAN_POINT('',(6.9,7.09789564133157,8.44145532612415));
#26485=CARTESIAN_POINT('Ctrl Pts',(37.5,32.3652591523689,1.5));
#26486=CARTESIAN_POINT('Ctrl Pts',(36.64906963214,31.6144476510502,1.5));
#26487=CARTESIAN_POINT('Ctrl Pts',(35.8406537800928,30.7967681970009,1.5));
#26488=CARTESIAN_POINT('Ctrl Pts',(35.0774452370603,29.9676650394942,1.5));
#26489=CARTESIAN_POINT('Ctrl Pts',(34.6958409655441,29.5531134607409,1.5));
#26490=CARTESIAN_POINT('Ctrl Pts',(34.3255255041702,29.1357262196348,1.5));
#26491=CARTESIAN_POINT('Ctrl Pts',(33.9666810635328,28.7225756061845,1.5));
#26492=CARTESIAN_POINT('Ctrl Pts',(33.7186145566461,28.436967643819,1.5));
#26493=CARTESIAN_POINT('Ctrl Pts',(33.4671024168721,28.1428784519157,1.5));
#26494=CARTESIAN_POINT('Ctrl Pts',(33.2400985609432,27.8754055139464,1.5));
#26495=CARTESIAN_POINT('Ctrl Pts',(33.1387264796055,27.7559613383729,1.5));
#26496=CARTESIAN_POINT('Ctrl Pts',(33.0532004124081,27.6547707095322,1.5));
#26497=CARTESIAN_POINT('Ctrl Pts',(33.,27.5917792275077,1.5));
#26498=CARTESIAN_POINT('Ctrl Pts',(32.9185691495653,27.4953617427699,1.5));
#26499=CARTESIAN_POINT('Ctrl Pts',(32.8516820633046,27.4160082741213,1.49973385699152));
#26500=CARTESIAN_POINT('Ctrl Pts',(32.7777321455755,27.3281857858874,1.49925158146312));
#26501=CARTESIAN_POINT('Ctrl Pts',(32.1788699540067,26.6169805623007,1.4953460114673));
#26502=CARTESIAN_POINT('Ctrl Pts',(31.569287987155,25.8863210200885,1.47697823247539));
#26503=CARTESIAN_POINT('Ctrl Pts',(30.9513498040767,25.1628991372958,1.46858396443269));
#26504=CARTESIAN_POINT('Ctrl Pts',(30.6423807125376,24.8011881958995,1.46438683041133));
#26505=CARTESIAN_POINT('Ctrl Pts',(30.3347880607121,24.4452439233475,1.46274142297315));
#26506=CARTESIAN_POINT('Ctrl Pts',(30.0249306371945,24.0928170619347,1.46654496784322));
#26507=CARTESIAN_POINT('Ctrl Pts',(29.8700019254357,23.9166036312283,1.46844674027826));
#26508=CARTESIAN_POINT('Ctrl Pts',(29.7145097313546,23.7412668049894,1.47171272534086));
#26509=CARTESIAN_POINT('Ctrl Pts',(29.558010072049,23.5665148172585,1.47674445496712));
#26510=CARTESIAN_POINT('Ctrl Pts',(29.4797602423961,23.479138823393,1.47926031978024));
#26511=CARTESIAN_POINT('Ctrl Pts',(29.4012586241238,23.3919089755822,1.48221825336132));
#26512=CARTESIAN_POINT('Ctrl Pts',(29.3224502420517,23.3047886331069,1.48567308535852));
#26513=CARTESIAN_POINT('Ctrl Pts',(29.2736528206717,23.2508445227123,1.4878122853818));
#26514=CARTESIAN_POINT('Ctrl Pts',(29.2247377938435,23.1969423956128,1.49014206193805));
#26515=CARTESIAN_POINT('Ctrl Pts',(29.1756921971318,23.1430735689731,1.4926761669043));
#26516=CARTESIAN_POINT('Ctrl Pts',(29.145528605831,23.109943637245,1.49423466984117));
#26517=CARTESIAN_POINT('Ctrl Pts',(29.118149096899,23.0799256032268,1.49570957236425));
#26518=CARTESIAN_POINT('Ctrl Pts',(29.0849408699094,23.0435998794277,1.49759308512661));
#26519=CARTESIAN_POINT('Ctrl Pts',(29.0475462332514,23.0026947373604,1.49971404374963));
#26520=CARTESIAN_POINT('Ctrl Pts',(28.9599837410406,22.9072087350758,1.50462371437525));
#26521=CARTESIAN_POINT('Ctrl Pts',(28.8924081851533,22.8339936863707,1.50836890091433));
#26522=CARTESIAN_POINT('Ctrl Pts',(28.441080763973,22.3450009035549,1.53338246329392));
#26523=CARTESIAN_POINT('Ctrl Pts',(27.9936088572591,21.8761056068567,1.55654582151093));
#26524=CARTESIAN_POINT('Ctrl Pts',(27.5122543102273,21.3913010170864,1.59544751490245));
#26525=CARTESIAN_POINT('Ctrl Pts',(27.1397294111092,21.0161060968145,1.62555390840296));
#26526=CARTESIAN_POINT('Ctrl Pts',(26.7276341643888,20.612059683191,1.66499152471603));
#26527=CARTESIAN_POINT('Ctrl Pts',(26.2530417505368,20.1649482705455,1.74041895661093));
#26528=CARTESIAN_POINT('Ctrl Pts',(25.869494913883,19.8036104932301,1.80137642675969));
#26529=CARTESIAN_POINT('Ctrl Pts',(25.4447383161079,19.4141244720077,1.88186126749374));
#26530=CARTESIAN_POINT('Ctrl Pts',(24.9635886608324,18.9908103209297,1.98732702259573));
#26531=CARTESIAN_POINT('Ctrl Pts',(24.6119820459508,18.6814677825737,2.06439754884626));
#26532=CARTESIAN_POINT('Ctrl Pts',(24.2873626786048,18.3974053120019,2.1383239559649));
#26533=CARTESIAN_POINT('Ctrl Pts',(23.642661641875,17.8679904517118,2.30363857155873));
#26534=CARTESIAN_POINT('Ctrl Pts',(23.5760533212279,17.8132931071125,2.32071831596085));
#26535=CARTESIAN_POINT('Ctrl Pts',(23.5065967305564,17.7565376998146,2.33866955713063));
#26536=CARTESIAN_POINT('Ctrl Pts',(23.4342591639586,17.697767866208,2.3575237071575));
#26537=CARTESIAN_POINT('Ctrl Pts',(22.7443384436221,17.1372496203922,2.53734547031137));
#26538=CARTESIAN_POINT('Ctrl Pts',(21.7987837593128,16.3936354357686,2.82220391184387));
#26539=CARTESIAN_POINT('Ctrl Pts',(20.5610365528854,15.5107287130397,3.22118169125961));
#26540=CARTESIAN_POINT('Ctrl Pts',(19.7234582214103,14.9132694452415,3.49116827740851));
#26541=CARTESIAN_POINT('Ctrl Pts',(18.7603809281624,14.2521506387677,3.83806571370465));
#26542=CARTESIAN_POINT('Ctrl Pts',(17.6514222906382,13.5382422374622,4.23400473904287));
#26543=CARTESIAN_POINT('Ctrl Pts',(16.7565277906387,12.9621407669349,4.55351499318671));
#26544=CARTESIAN_POINT('Ctrl Pts',(15.7613807992389,12.3388737256115,4.93854202839549));
#26545=CARTESIAN_POINT('Ctrl Pts',(14.7199652846762,11.7149311743306,5.32978309078145));
#26546=CARTESIAN_POINT('Ctrl Pts',(13.7316067501733,11.1227766145274,5.7010916008333));
#26547=CARTESIAN_POINT('Ctrl Pts',(12.7260968661244,10.5273020287043,6.10453604902479));
#26548=CARTESIAN_POINT('Ctrl Pts',(11.7781012037546,9.97941683016941,6.47234380217571));
#26549=CARTESIAN_POINT('Ctrl Pts',(10.6475718363527,9.32603798942654,6.91097182865408));
#26550=CARTESIAN_POINT('Ctrl Pts',(9.62260863652904,8.72329062200739,7.33414209133673));
#26551=CARTESIAN_POINT('Ctrl Pts',(8.83596460437641,8.26196206072778,7.64982933055117));
#26552=CARTESIAN_POINT('Ctrl Pts',(8.38131550044699,7.99533241831014,7.83228405538783));
#26553=CARTESIAN_POINT('Ctrl Pts',(7.99969688490189,7.7691108049908,7.98693286597064));
#26554=CARTESIAN_POINT('Ctrl Pts',(7.59379043301236,7.52350537407302,8.15376232311959));
#26555=CARTESIAN_POINT('Ctrl Pts',(7.36145773430631,7.38292575944418,8.24925215291325));
#26556=CARTESIAN_POINT('Ctrl Pts',(7.13004605045561,7.24116906982141,8.34517464654934));
#26557=CARTESIAN_POINT('Ctrl Pts',(6.9,7.09789564133157,8.44145532612415));
#26558=CARTESIAN_POINT('',(6.9,9.46599415782505,5.6597919716369));
#26559=CARTESIAN_POINT('Ctrl Pts',(6.90000000000001,7.09789564133157,8.44145532612415));
#26560=CARTESIAN_POINT('Ctrl Pts',(6.90000000000001,7.5077690000137,8.09681826844945));
#26561=CARTESIAN_POINT('Ctrl Pts',(6.90000000000001,7.89280389060836,7.72210951819363));
#26562=CARTESIAN_POINT('Ctrl Pts',(6.90000000000001,8.70687723936702,6.80464666682922));
#26563=CARTESIAN_POINT('Ctrl Pts',(6.90000000000001,9.11389129061078,6.24868352466685));
#26564=CARTESIAN_POINT('Ctrl Pts',(6.90000000000001,9.46599415782505,5.6597919716369));
#26565=CARTESIAN_POINT('Ctrl Pts',(6.9,9.46599415782505,5.6597919716369));
#26566=CARTESIAN_POINT('Ctrl Pts',(6.98893730997541,9.50231572683742,5.61299197171201));
#26567=CARTESIAN_POINT('Ctrl Pts',(7.08052892388223,9.53955640247952,5.56508220248518));
#26568=CARTESIAN_POINT('Ctrl Pts',(7.17490192378012,9.57777162403489,5.51603067891051));
#26569=CARTESIAN_POINT('Ctrl Pts',(7.97363347618104,9.90120844676267,5.10088016324584));
#26570=CARTESIAN_POINT('Ctrl Pts',(8.96286060497891,10.2954119066048,4.58706675349338));
#26571=CARTESIAN_POINT('Ctrl Pts',(10.2403127965964,10.8024441000946,4.00248282963831));
#26572=CARTESIAN_POINT('Ctrl Pts',(10.439427640778,10.8814745615587,3.91136447885127));
#26573=CARTESIAN_POINT('Ctrl Pts',(10.6449386760872,10.9636620301559,3.81760465493853));
#26574=CARTESIAN_POINT('Ctrl Pts',(10.8572270226758,11.0492678117718,3.7213987913614));
#26575=CARTESIAN_POINT('Ctrl Pts',(11.0079272575452,11.1100380405809,3.6531037272664));
#26576=CARTESIAN_POINT('Ctrl Pts',(11.2445718661156,11.2057391107462,3.54599023607825));
#26577=CARTESIAN_POINT('Ctrl Pts',(11.5512244262555,11.3315975140437,3.40956688340402));
#26578=CARTESIAN_POINT('Ctrl Pts',(12.00446426929,11.5176192545082,3.20792989421962));
#26579=CARTESIAN_POINT('Ctrl Pts',(12.6082461582178,11.7683139215717,2.9428149047514));
#26580=CARTESIAN_POINT('Ctrl Pts',(13.3027146141536,12.0682094443783,2.65901005153358));
#26581=CARTESIAN_POINT('Ctrl Pts',(14.2466220418243,12.4758213511293,2.2732682562489));
#26582=CARTESIAN_POINT('Ctrl Pts',(15.3788272822924,12.9964524563587,1.81469502494887));
#26583=CARTESIAN_POINT('Ctrl Pts',(16.3720352459916,13.4908088373714,1.45101350883608));
#26584=CARTESIAN_POINT('Ctrl Pts',(17.5299186899716,14.0671303026852,1.02703301151891));
#26585=CARTESIAN_POINT('Ctrl Pts',(18.5521204793993,14.6296677023245,0.660984941495812));
#26586=CARTESIAN_POINT('Ctrl Pts',(19.4596586821662,15.1670907158914,0.371269140680975));
#26587=CARTESIAN_POINT('Ctrl Pts',(19.880385055414,15.4162350876749,0.236959557042726));
#26588=CARTESIAN_POINT('Ctrl Pts',(20.27477945539,15.6592719448482,0.112950602571839));
#26589=CARTESIAN_POINT('Ctrl Pts',(20.644698628669,15.8947820241755,3.27862736959617E-15));
#26590=CARTESIAN_POINT('Origin',(155.122410108095,0.,0.));
#26591=CARTESIAN_POINT('',(172.622410108095,-2.87422589366703,0.00219230231809422));
#26592=CARTESIAN_POINT('',(172.819589891905,-2.86687004470951,-0.000292364604808637));
#26593=CARTESIAN_POINT('',(155.122410108095,-2.872,-3.13019997719247E-13));
#26594=CARTESIAN_POINT('',(173.058,2.64453949578291,-1.13133757670319));
#26595=CARTESIAN_POINT('Ctrl Pts',(172.622410108095,-2.87422589366703,0.00219230231809418));
#26596=CARTESIAN_POINT('Ctrl Pts',(172.666840602011,-2.86739304828907,-0.797854553035495));
#26597=CARTESIAN_POINT('Ctrl Pts',(172.763886767894,-2.10484582911375,-2.55670607422354));
#26598=CARTESIAN_POINT('Ctrl Pts',(172.909083398529,0.776574793634194,-3.25358644951632));
#26599=CARTESIAN_POINT('Ctrl Pts',(173.009849535248,2.29916206741707,-1.92522559845067));
#26600=CARTESIAN_POINT('Ctrl Pts',(173.058,2.64453949578291,-1.13133757670319));
#26601=CARTESIAN_POINT('',(173.058,-0.208958374082678,-2.86438831129802));
#26602=CARTESIAN_POINT('Origin',(173.058,0.,0.));
#26603=CARTESIAN_POINT('Ctrl Pts',(172.819589891905,-2.86687004470951,-0.000292364604808186));
#26604=CARTESIAN_POINT('Ctrl Pts',(172.846444255971,-2.86629933481412,-0.486922577646889));
#26605=CARTESIAN_POINT('Ctrl Pts',(172.925914292002,-2.51836703171159,-1.92675278851268));
#26606=CARTESIAN_POINT('Ctrl Pts',(173.005384328034,-1.15590801223433,-2.79530792301902));
#26607=CARTESIAN_POINT('Ctrl Pts',(173.058,-0.208958374082637,-2.86438831129802));
#26608=CARTESIAN_POINT('Origin',(155.122410108095,0.,0.));
#26609=CARTESIAN_POINT('',(171.622410108095,-2.87356135069046,-0.00235826304143971));
#26610=CARTESIAN_POINT('',(171.819589891905,-2.87424241070289,0.00217440260399965));
#26611=CARTESIAN_POINT('',(155.122410108095,-2.872,-3.13019997719247E-13));
#26612=CARTESIAN_POINT('Ctrl Pts',(171.622410108095,-2.87356135069046,-0.00235826304143932));
#26613=CARTESIAN_POINT('Ctrl Pts',(171.631864231582,-2.87506858034527,-0.172686974326985));
#26614=CARTESIAN_POINT('Ctrl Pts',(171.693934027035,-2.78407626657566,-1.28935039450392));
#26615=CARTESIAN_POINT('Ctrl Pts',(171.808619494454,-1.32187438082726,-3.1195126227806));
#26616=CARTESIAN_POINT('Ctrl Pts',(171.966466510352,1.88769284474709,-2.81340333947064));
#26617=CARTESIAN_POINT('Ctrl Pts',(172.124313526251,3.38780638409936,0.0405047390324093));
#26618=CARTESIAN_POINT('Ctrl Pts',(172.282160542149,1.81982745081448,2.85778026783241));
#26619=CARTESIAN_POINT('Ctrl Pts',(172.440007558048,-1.39600998068982,3.08694689555915));
#26620=CARTESIAN_POINT('Ctrl Pts',(172.553424080029,-2.79854500868001,1.24309116568133));
#26621=CARTESIAN_POINT('Ctrl Pts',(172.614224930045,-2.87548467004053,0.149580399589383));
#26622=CARTESIAN_POINT('Ctrl Pts',(172.622410108095,-2.87422589366703,0.00219230231809418));
#26623=CARTESIAN_POINT('Ctrl Pts',(171.819589891905,-2.87424241070289,0.00217440260399975));
#26624=CARTESIAN_POINT('Ctrl Pts',(171.864083557507,-2.86748730574921,-0.798952851534598));
#26625=CARTESIAN_POINT('Ctrl Pts',(171.961192895075,-2.10336452521562,-2.55874939692443));
#26626=CARTESIAN_POINT('Ctrl Pts',(172.110917904609,0.869829193827587,-3.27436767007504));
#26627=CARTESIAN_POINT('Ctrl Pts',(172.268764920508,3.21691519730582,-1.0637880016197));
#26628=CARTESIAN_POINT('Ctrl Pts',(172.426611936406,2.65009699317679,2.11067616912988));
#26629=CARTESIAN_POINT('Ctrl Pts',(172.584458952305,-0.315318796737369,
3.37266439996185));
#26630=CARTESIAN_POINT('Ctrl Pts',(172.715451604138,-2.54150147573075,1.88704582168949));
#26631=CARTESIAN_POINT('Ctrl Pts',(172.793828584004,-2.8674175249366,0.466530484796677));
#26632=CARTESIAN_POINT('Ctrl Pts',(172.819589891905,-2.86687004470951,-0.000292364604808186));
#26633=CARTESIAN_POINT('Origin',(155.122410108095,0.,0.));
#26634=CARTESIAN_POINT('',(170.622410108095,-2.8674942953205,0.000227582857409601));
#26635=CARTESIAN_POINT('',(170.819589891905,-2.87352757519475,-0.00236597882501771));
#26636=CARTESIAN_POINT('',(155.122410108095,-2.872,-3.13019997719247E-13));
#26637=CARTESIAN_POINT('Ctrl Pts',(170.622410108095,-2.8674942953205,0.000227582857409842));
#26638=CARTESIAN_POINT('Ctrl Pts',(170.649503533118,-2.86714338948619,-0.490524080721482));
#26639=CARTESIAN_POINT('Ctrl Pts',(170.729212630108,-2.51520696034054,-1.93479179819195));
#26640=CARTESIAN_POINT('Ctrl Pts',(170.861537399063,-0.231273610377281,
-3.38012116904044));
#26641=CARTESIAN_POINT('Ctrl Pts',(171.019384414961,2.70261668758891,-2.04317595483142));
#26642=CARTESIAN_POINT('Ctrl Pts',(171.17723143086,3.18901336295286,1.14407252761205));
#26643=CARTESIAN_POINT('Ctrl Pts',(171.335078446758,0.787432799006144,3.2952476962313));
#26644=CARTESIAN_POINT('Ctrl Pts',(171.48347133917,-2.14069437351883,2.51213187458012));
#26645=CARTESIAN_POINT('Ctrl Pts',(171.579248559616,-2.86668029335008,0.775254906480099));
#26646=CARTESIAN_POINT('Ctrl Pts',(171.622410108095,-2.87356135069046,-0.00235826304143932));
#26647=CARTESIAN_POINT('Ctrl Pts',(170.819589891905,-2.87352757519475,-0.0023659788250179));
#26648=CARTESIAN_POINT('Ctrl Pts',(170.829107187077,-2.87504739493669,-0.173837919594956));
#26649=CARTESIAN_POINT('Ctrl Pts',(170.891240154216,-2.78334526035724,-1.29165779848931));
#26650=CARTESIAN_POINT('Ctrl Pts',(171.00598879332,-1.31816431809934,-3.12108180407131));
#26651=CARTESIAN_POINT('Ctrl Pts',(171.163835809219,1.89105258537231,-2.81115929350443));
#26652=CARTESIAN_POINT('Ctrl Pts',(171.321682825117,3.38773384709925,0.04455010635921));
#26653=CARTESIAN_POINT('Ctrl Pts',(171.479529841016,1.81646787669691,2.85992243368512));
#26654=CARTESIAN_POINT('Ctrl Pts',(171.637376856914,-1.39977490155201,3.08532882114793));
#26655=CARTESIAN_POINT('Ctrl Pts',(171.75073020721,-2.79913811640008,1.2407317623324));
#26656=CARTESIAN_POINT('Ctrl Pts',(171.811467885541,-2.87547550769956,0.148414559907332));
#26657=CARTESIAN_POINT('Ctrl Pts',(171.819589891905,-2.87424241070289,0.00217440260399975));
#26658=CARTESIAN_POINT('Origin',(155.122410108095,0.,0.));
#26659=CARTESIAN_POINT('',(169.622410108095,-2.87435821711997,0.00213318404225128));
#26660=CARTESIAN_POINT('',(169.819589891905,-2.86749724845603,0.000245826060064624));
#26661=CARTESIAN_POINT('',(155.122410108095,-2.872,-3.13019997719247E-13));
#26662=CARTESIAN_POINT('Ctrl Pts',(169.622410108095,-2.87435821711997,0.00213318404225135));
#26663=CARTESIAN_POINT('Ctrl Pts',(169.667142834655,-2.8676581248492,-0.803206107247127));
#26664=CARTESIAN_POINT('Ctrl Pts',(169.76449123318,-2.09660336467381,-2.56705067797754));
#26665=CARTESIAN_POINT('Ctrl Pts',(169.914455303673,0.884666035299711,-3.27048502929561));
#26666=CARTESIAN_POINT('Ctrl Pts',(170.072302319571,3.22149246026824,-1.04913899093533));
#26667=CARTESIAN_POINT('Ctrl Pts',(170.230149335469,2.64092984065361,2.12230909777109));
#26668=CARTESIAN_POINT('Ctrl Pts',(170.387996351368,-0.331263356051794,
3.37179046643881));
#26669=CARTESIAN_POINT('Ctrl Pts',(170.518749942243,-2.54479782657719,1.87742068807177));
#26670=CARTESIAN_POINT('Ctrl Pts',(170.596887861152,-2.86782485173223,0.46252000748776));
#26671=CARTESIAN_POINT('Ctrl Pts',(170.622410108095,-2.8674942953205,0.000227582857409842));
#26672=CARTESIAN_POINT('Ctrl Pts',(169.819589891905,-2.86749724845603,0.00024582606006452));
#26673=CARTESIAN_POINT('Ctrl Pts',(169.846746488614,-2.86711729687761,-0.491648894342766));
#26674=CARTESIAN_POINT('Ctrl Pts',(169.926518757289,-2.51399256659462,-1.93709682488167));
#26675=CARTESIAN_POINT('Ctrl Pts',(170.05890669793,-0.227248629623084,-3.38039427118688));
#26676=CARTESIAN_POINT('Ctrl Pts',(170.216753713828,2.7050479786207,-2.03995651601825));
#26677=CARTESIAN_POINT('Ctrl Pts',(170.374600729726,3.18764860462061,1.14786927643015));
#26678=CARTESIAN_POINT('Ctrl Pts',(170.532447745625,0.783509087420058,3.2961828100762));
#26679=CARTESIAN_POINT('Ctrl Pts',(170.680777466351,-2.1424393721461,2.50991663454912));
#26680=CARTESIAN_POINT('Ctrl Pts',(170.776491515111,-2.86664518238132,0.77413219414454));
#26681=CARTESIAN_POINT('Ctrl Pts',(170.819589891905,-2.87352757519475,-0.0023659788250179));
#26682=CARTESIAN_POINT('Origin',(155.122410108095,0.,0.));
#26683=CARTESIAN_POINT('',(168.622410108095,-2.87340176099087,-0.00239232046765291));
#26684=CARTESIAN_POINT('',(168.819589891905,-2.87438921400676,0.00212235973350849));
#26685=CARTESIAN_POINT('',(155.122410108095,-2.872,-3.13019997719247E-13));
#26686=CARTESIAN_POINT('Ctrl Pts',(168.622410108095,-2.87340176099087,-0.00239232046765273));
#26687=CARTESIAN_POINT('Ctrl Pts',(168.632166464225,-2.87496866737895,-0.178191256630362));
#26688=CARTESIAN_POINT('Ctrl Pts',(168.694538492321,-2.78056600145512,-1.300389394094));
#26689=CARTESIAN_POINT('Ctrl Pts',(168.809526192383,-1.30408738860609,-3.12698935027992));
#26690=CARTESIAN_POINT('Ctrl Pts',(168.967373208282,1.9037022189819,-2.80261024323187));
#26691=CARTESIAN_POINT('Ctrl Pts',(169.12522022418,3.38749585741264,0.0598174693970574));
#26692=CARTESIAN_POINT('Ctrl Pts',(169.283067240079,1.80356748292359,2.86807437987086));
#26693=CARTESIAN_POINT('Ctrl Pts',(169.440914255977,-1.41367467356012,3.07899825141338));
#26694=CARTESIAN_POINT('Ctrl Pts',(169.554028545316,-2.80175403108198,1.23199926250765));
#26695=CARTESIAN_POINT('Ctrl Pts',(169.614527162688,-2.87553892899808,0.144052672416806));
#26696=CARTESIAN_POINT('Ctrl Pts',(169.622410108095,-2.87435821711997,0.00213318404225135));
#26697=CARTESIAN_POINT('Ctrl Pts',(168.819589891905,-2.87438921400676,0.00212235973350855));
#26698=CARTESIAN_POINT('Ctrl Pts',(168.86438579015,-2.86770274060997,-0.804331700826428));
#26699=CARTESIAN_POINT('Ctrl Pts',(168.961797360362,-2.09480143196574,-2.56925069528134));
#26700=CARTESIAN_POINT('Ctrl Pts',(169.111824602539,0.888559801961863,-3.26942943049782));
#26701=CARTESIAN_POINT('Ctrl Pts',(169.269671618437,3.2227395907929,-1.04530227652681));
#26702=CARTESIAN_POINT('Ctrl Pts',(169.427518634336,2.63840092301917,2.12545239707543));
#26703=CARTESIAN_POINT('Ctrl Pts',(169.585365650234,-0.335278112564125,
3.37139376458444));
#26704=CARTESIAN_POINT('Ctrl Pts',(169.716056069424,-2.54596312587379,1.87511246443019));
#26705=CARTESIAN_POINT('Ctrl Pts',(169.794130816648,-2.86785344978467,0.461392885089547));
#26706=CARTESIAN_POINT('Ctrl Pts',(169.819589891905,-2.86749724845603,0.00024582606006452));
#26707=CARTESIAN_POINT('Origin',(155.122410108095,0.,0.));
#26708=CARTESIAN_POINT('',(167.622410108095,-2.8675098280091,0.000314758925835955));
#26709=CARTESIAN_POINT('',(167.819589891905,-2.87336857678864,-0.00239892095949074));
#26710=CARTESIAN_POINT('',(155.122410108095,-2.872,-3.13019997719247E-13));
#26711=CARTESIAN_POINT('Ctrl Pts',(167.622410108095,-2.8675098280091,0.000314758925835865));
#26712=CARTESIAN_POINT('Ctrl Pts',(167.649805765761,-2.86701892352542,-0.49590461907087));
#26713=CARTESIAN_POINT('Ctrl Pts',(167.729817095394,-2.50937904224953,-1.94581795526478));
#26714=CARTESIAN_POINT('Ctrl Pts',(167.862444096993,-0.212013665700137,
-3.38138381723357));
#26715=CARTESIAN_POINT('Ctrl Pts',(168.020291112891,2.7142128214914,-2.02774630403978));
#26716=CARTESIAN_POINT('Ctrl Pts',(168.17813812879,3.18244355869507,1.16222171275988));
#26717=CARTESIAN_POINT('Ctrl Pts',(168.335985144688,0.76864799350228,3.29967976870115));
#26718=CARTESIAN_POINT('Ctrl Pts',(168.484075804457,-2.14901785032668,2.50152539436281));
#26719=CARTESIAN_POINT('Ctrl Pts',(168.579550792259,-2.86651839850613,0.769885979781707));
#26720=CARTESIAN_POINT('Ctrl Pts',(168.622410108095,-2.87340176099087,-0.00239232046765273));
#26721=CARTESIAN_POINT('Ctrl Pts',(167.819589891905,-2.87336857678864,-0.00239892095949067));
#26722=CARTESIAN_POINT('Ctrl Pts',(167.82940941972,-2.87494778079546,-0.17934145242446));
#26723=CARTESIAN_POINT('Ctrl Pts',(167.891844619502,-2.7798280420658,-1.30269698359132));
#26724=CARTESIAN_POINT('Ctrl Pts',(168.00689549125,-1.30036303375706,-3.12854012314479));
#26725=CARTESIAN_POINT('Ctrl Pts',(168.164742507148,1.90703818343888,-2.80034153070911));
#26726=CARTESIAN_POINT('Ctrl Pts',(168.322589523047,3.38742237645021,0.0638511173542441));
#26727=CARTESIAN_POINT('Ctrl Pts',(168.480436538945,1.80015110090155,2.87022008487266));
#26728=CARTESIAN_POINT('Ctrl Pts',(168.638283554844,-1.41734007501666,3.07731285922868));
#26729=CARTESIAN_POINT('Ctrl Pts',(168.751334672497,-2.80244519982093,1.22969466039503));
#26730=CARTESIAN_POINT('Ctrl Pts',(168.811770118184,-2.8755564349132,0.142900612140373));
#26731=CARTESIAN_POINT('Ctrl Pts',(168.819589891905,-2.87438921400676,0.00212235973350855));
#26732=CARTESIAN_POINT('Origin',(155.122410108095,0.,0.));
#26733=CARTESIAN_POINT('',(166.622410108095,-2.87450488446859,0.00208020559110183));
#26734=CARTESIAN_POINT('',(166.819589891905,-2.86751383367012,0.000332938889392731));
#26735=CARTESIAN_POINT('',(155.122410108095,-2.872,-3.13019997719247E-13));
#26736=CARTESIAN_POINT('Ctrl Pts',(166.622410108095,-2.87450488446859,0.00208020559110164));
#26737=CARTESIAN_POINT('Ctrl Pts',(166.667445067298,-2.86787466431953,-0.808592444296684));
#26738=CARTESIAN_POINT('Ctrl Pts',(166.765095698467,-2.08796138916789,-2.57756977721455));
#26739=CARTESIAN_POINT('Ctrl Pts',(166.915362001602,0.903283370530585,-3.26539208463793));
#26740=CARTESIAN_POINT('Ctrl Pts',(167.0732090175,3.22741704709102,-1.03076938159775));
#26741=CARTESIAN_POINT('Ctrl Pts',(167.231056033399,2.62879635362904,2.13731982750353));
#26742=CARTESIAN_POINT('Ctrl Pts',(167.388903049297,-0.350466791168255,
3.36984856368669));
#26743=CARTESIAN_POINT('Ctrl Pts',(167.519354407529,-2.55035531167827,1.86637599950059));
#26744=CARTESIAN_POINT('Ctrl Pts',(167.597190093795,-2.86796174700476,0.457126563237285));
#26745=CARTESIAN_POINT('Ctrl Pts',(167.622410108095,-2.8675098280091,0.000314758925835865));
#26746=CARTESIAN_POINT('Ctrl Pts',(166.819589891905,-2.86751383367012,0.000332938889392939));
#26747=CARTESIAN_POINT('Ctrl Pts',(166.847048721257,-2.86699333758779,-0.497029011732394));
#26748=CARTESIAN_POINT('Ctrl Pts',(166.927123222575,-2.50815544873722,-1.94812225213107));
#26749=CARTESIAN_POINT('Ctrl Pts',(167.059813395859,-0.207987114903346,
-3.38163402539736));
#26750=CARTESIAN_POINT('Ctrl Pts',(167.217660411758,2.71662557150557,-2.02451298487645));
#26751=CARTESIAN_POINT('Ctrl Pts',(167.375507427656,3.18105751740887,1.16601045991334));
#26752=CARTESIAN_POINT('Ctrl Pts',(167.533354443555,0.764718362261322,3.3005928479761));
#26753=CARTESIAN_POINT('Ctrl Pts',(167.681381931638,-2.15075093712925,2.4993067245601));
#26754=CARTESIAN_POINT('Ctrl Pts',(167.776793747754,-2.86648598084416,0.768764237317345));
#26755=CARTESIAN_POINT('Ctrl Pts',(167.819589891905,-2.87336857678864,-0.00239892095949067));
#26756=CARTESIAN_POINT('Origin',(155.122410108095,0.,0.));
#26757=CARTESIAN_POINT('',(165.622410108095,-2.87324197174522,-0.00242261092417198));
#26758=CARTESIAN_POINT('',(165.819589891905,-2.87453532874939,0.00206875392256244));
#26759=CARTESIAN_POINT('',(155.122410108095,-2.872,-3.13019997719247E-13));
#26760=CARTESIAN_POINT('Ctrl Pts',(165.622410108095,-2.87324197174522,-0.00242261092417158));
#26761=CARTESIAN_POINT('Ctrl Pts',(165.632468696868,-2.8748671275446,-0.183693495603892));
#26762=CARTESIAN_POINT('Ctrl Pts',(165.695142957607,-2.7770207161025,-1.31143012210531));
#26763=CARTESIAN_POINT('Ctrl Pts',(165.810432890313,-1.28625201732507,-3.13436788871701));
#26764=CARTESIAN_POINT('Ctrl Pts',(165.968279906211,1.91963757364734,-2.79171952383016));
#26765=CARTESIAN_POINT('Ctrl Pts',(166.12612692211,3.38710011122917,0.0791147925766244));
#26766=CARTESIAN_POINT('Ctrl Pts',(166.283973938008,1.78719902416841,2.87830261819438));
#26767=CARTESIAN_POINT('Ctrl Pts',(166.441820953907,-1.43119254050081,3.07089469469534));
#26768=CARTESIAN_POINT('Ctrl Pts',(166.554633010602,-2.80504650106343,1.22097398834813));
#26769=CARTESIAN_POINT('Ctrl Pts',(166.614829395332,-2.87562094619924,0.138540338178042));
#26770=CARTESIAN_POINT('Ctrl Pts',(166.622410108095,-2.87450488446859,0.00208020559110164));
#26771=CARTESIAN_POINT('Ctrl Pts',(165.819589891905,-2.87453532874939,0.00206875392256263));
#26772=CARTESIAN_POINT('Ctrl Pts',(165.864688022793,-2.86792123297805,-0.809718743524386));
#26773=CARTESIAN_POINT('Ctrl Pts',(165.962401825648,-2.08614859619317,-2.57976665801494));
#26774=CARTESIAN_POINT('Ctrl Pts',(166.112731300469,0.90717106151226,-3.26431432108579));
#26775=CARTESIAN_POINT('Ctrl Pts',(166.270578316367,3.22864229756116,-1.02692562344606));
#26776=CARTESIAN_POINT('Ctrl Pts',(166.428425332265,2.62624957467685,2.14044866633159));
#26777=CARTESIAN_POINT('Ctrl Pts',(166.586272348164,-0.354479232189763,
3.36942900142401));
#26778=CARTESIAN_POINT('Ctrl Pts',(166.71666053471,-2.55151157895156,1.86406723401458));
#26779=CARTESIAN_POINT('Ctrl Pts',(166.794433049291,-2.86799069442252,0.455998989096919));
#26780=CARTESIAN_POINT('Ctrl Pts',(166.819589891905,-2.86751383367012,0.000332938889392939));
#26781=CARTESIAN_POINT('Origin',(155.122410108095,0.,0.));
#26782=CARTESIAN_POINT('',(164.622410108095,-2.86753036214098,0.00040157864720313));
#26783=CARTESIAN_POINT('',(164.819589891905,-2.87320857308323,-0.00242853002640792));
#26784=CARTESIAN_POINT('',(155.122410108095,-2.872,-3.13019997719247E-13));
#26785=CARTESIAN_POINT('Ctrl Pts',(164.622410108095,-2.86753036214098,0.000401578647203325));
#26786=CARTESIAN_POINT('Ctrl Pts',(164.650107998405,-2.86689688195682,-0.501283178591449));
#26787=CARTESIAN_POINT('Ctrl Pts',(164.73042156068,-2.50350697808224,-1.95684059811892));
#26788=CARTESIAN_POINT('Ctrl Pts',(164.863350794922,-0.192746751143198,
-3.38253677050477));
#26789=CARTESIAN_POINT('Ctrl Pts',(165.021197810821,2.72572068544879,-2.01225074451711));
#26790=CARTESIAN_POINT('Ctrl Pts',(165.179044826719,3.1757708308709,1.18033298000295));
#26791=CARTESIAN_POINT('Ctrl Pts',(165.336891842617,0.749837507567218,3.30400514923002));
#26792=CARTESIAN_POINT('Ctrl Pts',(165.484680269743,-2.15728879001875,2.49090483660323));
#26793=CARTESIAN_POINT('Ctrl Pts',(165.579853024902,-2.86636606776747,0.764519978515341));
#26794=CARTESIAN_POINT('Ctrl Pts',(165.622410108095,-2.87324197174522,-0.00242261092417158));
#26795=CARTESIAN_POINT('Ctrl Pts',(164.819589891905,-2.87320857308323,-0.00242853002640802));
#26796=CARTESIAN_POINT('Ctrl Pts',(164.829711652364,-2.87484571022488,-0.184843366841589));
#26797=CARTESIAN_POINT('Ctrl Pts',(164.892449084789,-2.77627531036844,-1.31373812678202));
#26798=CARTESIAN_POINT('Ctrl Pts',(165.007802189179,-1.28251888829241,-3.13589741905954));
#26799=CARTESIAN_POINT('Ctrl Pts',(165.165649205078,1.92296055931244,-2.78943184340823));
#26800=CARTESIAN_POINT('Ctrl Pts',(165.323496220976,3.38700365205358,0.0831479564798997));
#26801=CARTESIAN_POINT('Ctrl Pts',(165.481343236875,1.78377047374568,2.88042882548487));
#26802=CARTESIAN_POINT('Ctrl Pts',(165.639190252773,-1.43484828107338,3.06918844843256));
#26803=CARTESIAN_POINT('Ctrl Pts',(165.751939137783,-2.80573043323553,1.21866986550307));
#26804=CARTESIAN_POINT('Ctrl Pts',(165.812072350827,-2.87563785197317,0.13738801745482));
#26805=CARTESIAN_POINT('Ctrl Pts',(165.819589891905,-2.87453532874939,0.00206875392256263));
#26806=CARTESIAN_POINT('Origin',(155.122410108095,0.,0.));
#26807=CARTESIAN_POINT('',(163.622410108095,-2.87464881776804,0.00202424674990214));
#26808=CARTESIAN_POINT('',(163.819589891905,-2.86753540926279,0.000419670536143391));
#26809=CARTESIAN_POINT('',(155.122410108095,-2.872,-3.13019997719247E-13));
#26810=CARTESIAN_POINT('Ctrl Pts',(163.622410108095,-2.87464881776804,0.00202424674990246));
#26811=CARTESIAN_POINT('Ctrl Pts',(163.667747299941,-2.86810059116501,-0.813982217531092));
#26812=CARTESIAN_POINT('Ctrl Pts',(163.765700163753,-2.07926741161996,-2.58807376981798));
#26813=CARTESIAN_POINT('Ctrl Pts',(163.916268699531,0.921871390857911,-3.26019316185573));
#26814=CARTESIAN_POINT('Ctrl Pts',(164.07411571543,3.23323688492365,-1.01236631703268));
#26815=CARTESIAN_POINT('Ctrl Pts',(164.231962731328,2.61657755392199,2.15226118726438));
#26816=CARTESIAN_POINT('Ctrl Pts',(164.389809747227,-0.369658862607259,
3.36779729781782));
#26817=CARTESIAN_POINT('Ctrl Pts',(164.519958872816,-2.55586969631235,1.85532880014071));
#26818=CARTESIAN_POINT('Ctrl Pts',(164.597492326438,-2.868100258286,0.451730943503979));
#26819=CARTESIAN_POINT('Ctrl Pts',(164.622410108095,-2.86753036214098,0.000401578647203325));
#26820=CARTESIAN_POINT('Ctrl Pts',(163.819589891905,-2.86753540926279,0.000419670536143772));
#26821=CARTESIAN_POINT('Ctrl Pts',(163.8473509539,-2.86687181424791,-0.502407163892982));
#26822=CARTESIAN_POINT('Ctrl Pts',(163.927727687861,-2.50227413339466,-1.95914414506922));
#26823=CARTESIAN_POINT('Ctrl Pts',(164.060720093789,-0.188718840271762,
-3.38276403566928));
#26824=CARTESIAN_POINT('Ctrl Pts',(164.218567109687,2.72811497634857,-2.00900373257834));
#26825=CARTESIAN_POINT('Ctrl Pts',(164.376414125585,3.17436322788575,1.18411376950773));
#26826=CARTESIAN_POINT('Ctrl Pts',(164.534261141484,0.74590273835584,3.30489582689142));
#26827=CARTESIAN_POINT('Ctrl Pts',(164.681986396924,-2.15901119308368,2.48868340770977));
#26828=CARTESIAN_POINT('Ctrl Pts',(164.777095980397,-2.86633542477008,0.763398715632628));
#26829=CARTESIAN_POINT('Ctrl Pts',(164.819589891905,-2.87320857308323,-0.00242853002640802));
#26830=CARTESIAN_POINT('Origin',(155.122410108095,0.,0.));
#26831=CARTESIAN_POINT('',(162.622410108095,-2.8730812386835,-0.00244963452792444));
#26832=CARTESIAN_POINT('',(162.819589891905,-2.87467866166092,0.0020121790497752));
#26833=CARTESIAN_POINT('',(155.122410108095,-2.872,-3.13019997719247E-13));
#26834=CARTESIAN_POINT('Ctrl Pts',(162.622410108095,-2.8730812386835,-0.00244963452792442));
#26835=CARTESIAN_POINT('Ctrl Pts',(162.632770929511,-2.87476306855881,-0.189194165208951));
#26836=CARTESIAN_POINT('Ctrl Pts',(162.695747422894,-2.7734397513437,-1.32247281514995));
#26837=CARTESIAN_POINT('Ctrl Pts',(162.811339588242,-1.26837490053319,-3.14164470072457));
#26838=CARTESIAN_POINT('Ctrl Pts',(162.969186604141,1.9355106261794,-2.78073819872344));
#26839=CARTESIAN_POINT('Ctrl Pts',(163.127033620039,3.38659443611677,0.0984095480937175));
#26840=CARTESIAN_POINT('Ctrl Pts',(163.284880635938,1.77077256165387,2.88843744069124));
#26841=CARTESIAN_POINT('Ctrl Pts',(163.442727651836,-1.44866395801099,3.0626914716721));
#26842=CARTESIAN_POINT('Ctrl Pts',(163.555237475889,-2.80830440148675,1.20995102409985));
#26843=CARTESIAN_POINT('Ctrl Pts',(163.615131627975,-2.87570007690456,0.133026776600459));
#26844=CARTESIAN_POINT('Ctrl Pts',(163.622410108095,-2.87464881776804,0.00202424674990246));
#26845=CARTESIAN_POINT('Ctrl Pts',(162.819589891905,-2.87467866166092,0.00201217904977503));
#26846=CARTESIAN_POINT('Ctrl Pts',(162.864990255437,-2.86814913610333,-0.815109254849669));
#26847=CARTESIAN_POINT('Ctrl Pts',(162.963006290934,-2.07744373508779,-2.59026746179106));
#26848=CARTESIAN_POINT('Ctrl Pts',(163.113637998398,0.925752878818704,-3.25909326792743));
#26849=CARTESIAN_POINT('Ctrl Pts',(163.271485014297,3.23444021792712,-1.00851564110162));
#26850=CARTESIAN_POINT('Ctrl Pts',(163.429332030195,2.61401299155246,2.15537546652226));
#26851=CARTESIAN_POINT('Ctrl Pts',(163.587179046093,-0.37366884830378,3.36735488380693));
#26852=CARTESIAN_POINT('Ctrl Pts',(163.717264999997,-2.55701697759514,1.85301952789162));
#26853=CARTESIAN_POINT('Ctrl Pts',(163.794735281934,-2.868129529015,0.450602911181542));
#26854=CARTESIAN_POINT('Ctrl Pts',(163.819589891905,-2.86753540926279,0.000419670536143772));
#26855=CARTESIAN_POINT('Origin',(155.122410108095,0.,0.));
#26856=CARTESIAN_POINT('',(161.622410108095,-2.86755587111262,0.000487937565173562));
#26857=CARTESIAN_POINT('',(161.819589891905,-2.87304766888017,-0.00245486878760248));
#26858=CARTESIAN_POINT('',(155.122410108095,-2.872,-3.13019997719247E-13));
#26859=CARTESIAN_POINT('Ctrl Pts',(161.622410108095,-2.86755587111262,0.000487937565173541));
#26860=CARTESIAN_POINT('Ctrl Pts',(161.650410231048,-2.86677736484341,-0.506659802481027));
#26861=CARTESIAN_POINT('Ctrl Pts',(161.731026025967,-2.49759059547312,-1.96785959265111));
#26862=CARTESIAN_POINT('Ctrl Pts',(161.864257492852,-0.173473580959878,
-3.38357994299221));
#26863=CARTESIAN_POINT('Ctrl Pts',(162.02210450875,2.73714008569463,-1.99668987706511));
#26864=CARTESIAN_POINT('Ctrl Pts',(162.179951524649,3.16899503288228,1.1984059393451));
#26865=CARTESIAN_POINT('Ctrl Pts',(162.337798540547,0.731002685534005,3.30822329772906));
#26866=CARTESIAN_POINT('Ctrl Pts',(162.485284735029,-2.16550866044979,2.48027117452657));
#26867=CARTESIAN_POINT('Ctrl Pts',(162.580155257545,-2.86622218116522,0.759156218698579));
#26868=CARTESIAN_POINT('Ctrl Pts',(162.622410108095,-2.8730812386835,-0.00244963452792442));
#26869=CARTESIAN_POINT('Ctrl Pts',(161.819589891905,-2.87304766888017,-0.00245486878760231));
#26870=CARTESIAN_POINT('Ctrl Pts',(161.830013885007,-2.87474113114852,-0.190343703764303));
#26871=CARTESIAN_POINT('Ctrl Pts',(161.893053550075,-2.77268687039962,-1.32478122490515));
#26872=CARTESIAN_POINT('Ctrl Pts',(162.008708887109,-1.26463311846787,-3.14315293890823));
#26873=CARTESIAN_POINT('Ctrl Pts',(162.166555903007,1.93882052518752,-2.77843162464046));
#26874=CARTESIAN_POINT('Ctrl Pts',(162.324402918906,3.38647500189316,0.102442097028211));
#26875=CARTESIAN_POINT('Ctrl Pts',(162.482249934804,1.76733195403479,2.89054408130007));
#26876=CARTESIAN_POINT('Ctrl Pts',(162.640096950703,-1.4523099189108,3.0609644266349));
#26877=CARTESIAN_POINT('Ctrl Pts',(162.75254360307,-2.80898112495851,1.20764738811918));
#26878=CARTESIAN_POINT('Ctrl Pts',(162.81237458347,-2.87571637451529,0.131874204714068));
#26879=CARTESIAN_POINT('Ctrl Pts',(162.819589891905,-2.87467866166092,0.00201217904977503));
#26880=CARTESIAN_POINT('Origin',(155.122410108095,0.,0.));
#26881=CARTESIAN_POINT('',(160.622410108095,-2.87478978750438,0.00196536333635101));
#26882=CARTESIAN_POINT('',(160.819589891905,-2.86756195538547,0.000505920555084749));
#26883=CARTESIAN_POINT('',(155.122410108095,-2.872,-3.13019997719247E-13));
#26884=CARTESIAN_POINT('Ctrl Pts',(160.622410108095,-2.87478978750438,0.00196536333635124));
#26885=CARTESIAN_POINT('Ctrl Pts',(160.668049532584,-2.86833601734048,-0.819375583152982));
#26886=CARTESIAN_POINT('Ctrl Pts',(160.76630462904,-2.07052132275083,-2.59856240354522));
#26887=CARTESIAN_POINT('Ctrl Pts',(160.917175397461,0.940429491634335,-3.25488842913799));
#26888=CARTESIAN_POINT('Ctrl Pts',(161.075022413359,3.23895178755388,-0.993930395869087));
#26889=CARTESIAN_POINT('Ctrl Pts',(161.232869429258,2.60427383274531,2.16713269499377));
#26890=CARTESIAN_POINT('Ctrl Pts',(161.390716445156,-0.388838936699488,
3.36563672955522));
#26891=CARTESIAN_POINT('Ctrl Pts',(161.520563338102,-2.56134114788908,1.84427923030537));
#26892=CARTESIAN_POINT('Ctrl Pts',(161.597794559082,-2.86824027379397,0.446333124501563));
#26893=CARTESIAN_POINT('Ctrl Pts',(161.622410108095,-2.86755587111262,0.000487937565173541));
#26894=CARTESIAN_POINT('Ctrl Pts',(160.819589891905,-2.86756195538547,0.000505920555084784));
#26895=CARTESIAN_POINT('Ctrl Pts',(160.847653186543,-2.86675283921063,-0.507783388132381));
#26896=CARTESIAN_POINT('Ctrl Pts',(160.928332153148,-2.49634846830188,-1.97016235883692));
#26897=CARTESIAN_POINT('Ctrl Pts',(161.061626791718,-0.169444440750171,
-3.38378425779796));
#26898=CARTESIAN_POINT('Ctrl Pts',(161.219473807617,2.73951583977761,-1.99342927772498));
#26899=CARTESIAN_POINT('Ctrl Pts',(161.377320823515,3.16756591388022,1.2021786484908));
#26900=CARTESIAN_POINT('Ctrl Pts',(161.535167839414,0.727062906055984,3.30909154487233));
#26901=CARTESIAN_POINT('Ctrl Pts',(161.68259086221,-2.16722040452248,2.47804703603232));
#26902=CARTESIAN_POINT('Ctrl Pts',(161.777398213041,-2.86619328827026,0.758035406874766));
#26903=CARTESIAN_POINT('Ctrl Pts',(161.819589891905,-2.87304766888017,-0.00245486878760231));
#26904=CARTESIAN_POINT('Origin',(155.122410108095,0.,0.));
#26905=CARTESIAN_POINT('',(159.622410108095,-2.87291976826755,-0.00247337730410335));
#26906=CARTESIAN_POINT('',(159.819589891905,-2.87481898359611,0.00195269049801133));
#26907=CARTESIAN_POINT('',(155.122410108095,-2.872,-3.13019997719247E-13));
#26908=CARTESIAN_POINT('Ctrl Pts',(159.622410108095,-2.87291976826755,-0.00247337730410344));
#26909=CARTESIAN_POINT('Ctrl Pts',(159.633073162154,-2.87465654392156,-0.194693232183184));
#26910=CARTESIAN_POINT('Ctrl Pts',(159.69635188818,-2.76982297949715,-1.33351745257318));
#26911=CARTESIAN_POINT('Ctrl Pts',(159.812246286172,-1.25045660967965,-3.14881952692657));
#26912=CARTESIAN_POINT('Ctrl Pts',(159.97009330207,1.9513208570681,-2.76966663578875));
#26913=CARTESIAN_POINT('Ctrl Pts',(160.127940317969,3.38597885066797,0.117701115397386));
#26914=CARTESIAN_POINT('Ctrl Pts',(160.285787333867,1.75428862736512,2.89847851566358));
#26915=CARTESIAN_POINT('Ctrl Pts',(160.443634349766,-1.46608835837003,3.05438884988658));
#26916=CARTESIAN_POINT('Ctrl Pts',(160.555841941175,-2.81152786482851,1.19893040514894));
#26917=CARTESIAN_POINT('Ctrl Pts',(160.615433860618,-2.87577628324411,0.127512032028115));
#26918=CARTESIAN_POINT('Ctrl Pts',(160.622410108095,-2.87478978750438,0.00196536333635124));
#26919=CARTESIAN_POINT('Ctrl Pts',(159.819589891905,-2.87481898359611,0.00195269049801145));
#26920=CARTESIAN_POINT('Ctrl Pts',(159.86529248808,-2.86838656291233,-0.820503393147137));
#26921=CARTESIAN_POINT('Ctrl Pts',(159.963610756221,-2.0686867388201,-2.60075285164511));
#26922=CARTESIAN_POINT('Ctrl Pts',(160.114544696328,0.944304649918255,-3.25376644164669));
#26923=CARTESIAN_POINT('Ctrl Pts',(160.272391712226,3.24013316437363,-0.99007292658079));
#26924=CARTESIAN_POINT('Ctrl Pts',(160.430238728125,2.6016915700248,2.17023231333377));
#26925=CARTESIAN_POINT('Ctrl Pts',(160.588085744023,-0.392846336843677,
3.36517147828997));
#26926=CARTESIAN_POINT('Ctrl Pts',(160.717869465283,-2.56247947481748,1.84196947851954));
#26927=CARTESIAN_POINT('Ctrl Pts',(160.795037514577,-2.86826984538495,0.445204629650228));
#26928=CARTESIAN_POINT('Ctrl Pts',(160.819589891905,-2.86756195538547,0.000505920555084784));
#26929=CARTESIAN_POINT('Origin',(155.122410108095,0.,0.));
#26930=CARTESIAN_POINT('',(158.622410108095,-2.86758577620084,0.000575212723279395));
#26931=CARTESIAN_POINT('',(158.819589891905,-2.87288607329111,-0.00247792941845876));
#26932=CARTESIAN_POINT('',(155.122410108095,-2.872,-3.13019997719247E-13));
#26933=CARTESIAN_POINT('Ctrl Pts',(158.622410108095,-2.86758577620084,0.000575212723279185));
#26934=CARTESIAN_POINT('Ctrl Pts',(158.650712463691,-2.86666019302301,-0.51203374944874));
#26935=CARTESIAN_POINT('Ctrl Pts',(158.731630491253,-2.49163067088092,-1.97887724836087));
#26936=CARTESIAN_POINT('Ctrl Pts',(158.865164190781,-0.154194185277631,
-3.38451172074282));
#26937=CARTESIAN_POINT('Ctrl Pts',(159.02301120668,2.74847035696387,-1.98106498867635));
#26938=CARTESIAN_POINT('Ctrl Pts',(159.180858222578,3.16211653045467,1.21644039120453));
#26939=CARTESIAN_POINT('Ctrl Pts',(159.338705238477,0.71214406652733,3.31233388578888));
#26940=CARTESIAN_POINT('Ctrl Pts',(159.485889200316,-2.17367755200914,2.4696247196516));
#26941=CARTESIAN_POINT('Ctrl Pts',(159.580457490188,-2.86608661474556,0.753794581273767));
#26942=CARTESIAN_POINT('Ctrl Pts',(159.622410108095,-2.87291976826755,-0.00247337730410344));
#26943=CARTESIAN_POINT('Ctrl Pts',(158.819589891905,-2.87288607329111,-0.00247792941845921));
#26944=CARTESIAN_POINT('Ctrl Pts',(158.83031611765,-2.87463411866077,-0.195842464930666));
#26945=CARTESIAN_POINT('Ctrl Pts',(158.893658015361,-2.76906270875085,-1.33582644427906));
#26946=CARTESIAN_POINT('Ctrl Pts',(159.009615585039,-1.24670620219767,-3.15030627040552));
#26947=CARTESIAN_POINT('Ctrl Pts',(159.167462600937,1.95461751556788,-2.76734131891007));
#26948=CARTESIAN_POINT('Ctrl Pts',(159.325309616835,3.38583646824711,0.121732956096346));
#26949=CARTESIAN_POINT('Ctrl Pts',(159.483156632734,1.75083606284643,2.90056550260836));
#26950=CARTESIAN_POINT('Ctrl Pts',(159.641003648632,-1.46972441564107,3.05264107133596));
#26951=CARTESIAN_POINT('Ctrl Pts',(159.753148068356,-2.81219740750062,1.1966272626752));
#26952=CARTESIAN_POINT('Ctrl Pts',(159.812676816114,-2.87579196577723,0.126359216980713));
#26953=CARTESIAN_POINT('Ctrl Pts',(159.819589891905,-2.87481898359611,0.00195269049801145));
#26954=CARTESIAN_POINT('Origin',(155.122410108095,0.,0.));
#26955=CARTESIAN_POINT('',(157.622410108095,-2.87487623080957,0.00203977944324937));
#26956=CARTESIAN_POINT('',(157.819589891905,-2.86758689937222,0.000602879185873928));
#26957=CARTESIAN_POINT('',(155.122410108095,-2.872,-3.13019997719247E-13));
#26958=CARTESIAN_POINT('Ctrl Pts',(157.622410108095,-2.87487623080957,0.00203977944324927));
#26959=CARTESIAN_POINT('Ctrl Pts',(157.668351765227,-2.86851795772887,-0.824605202196607));
#26960=CARTESIAN_POINT('Ctrl Pts',(157.766909094326,-2.06179973823486,-2.60923904502658));
#26961=CARTESIAN_POINT('Ctrl Pts',(157.918082095391,0.958997601442651,-3.24937049328252));
#26962=CARTESIAN_POINT('Ctrl Pts',(158.075929111289,3.24454151146318,-0.97551544854114));
#26963=CARTESIAN_POINT('Ctrl Pts',(158.233776127188,2.5918955157916,2.18196021165553));
#26964=CARTESIAN_POINT('Ctrl Pts',(158.391623143086,-0.408011303340585,
3.36335389202508));
#26965=CARTESIAN_POINT('Ctrl Pts',(158.521167803389,-2.56676870336052,1.83323037708674));
#26966=CARTESIAN_POINT('Ctrl Pts',(158.598096791725,-2.86838090424426,0.44093516188752));
#26967=CARTESIAN_POINT('Ctrl Pts',(158.622410108095,-2.86758577620084,0.000575212723279185));
#26968=CARTESIAN_POINT('Ctrl Pts',(157.819589891905,-2.86758689937222,0.000602879185874344));
#26969=CARTESIAN_POINT('Ctrl Pts',(157.847955419186,-2.86663306014058,-0.513151746479082));
#26970=CARTESIAN_POINT('Ctrl Pts',(157.928936618434,-2.49038917880739,-1.98119549062785));
#26971=CARTESIAN_POINT('Ctrl Pts',(158.062533489648,-0.150157556215628,
-3.38468261701631));
#26972=CARTESIAN_POINT('Ctrl Pts',(158.220380505546,2.7508243349508,-1.97779608453694));
#26973=CARTESIAN_POINT('Ctrl Pts',(158.378227521445,3.1606675065917,1.2202074592191));
#26974=CARTESIAN_POINT('Ctrl Pts',(158.536074537343,0.708198630334437,3.31317840661986));
#26975=CARTESIAN_POINT('Ctrl Pts',(158.683195327497,-2.17537835758644,2.46739841906479));
#26976=CARTESIAN_POINT('Ctrl Pts',(158.777700445684,-2.86605938007723,0.752674302497539));
#26977=CARTESIAN_POINT('Ctrl Pts',(158.819589891905,-2.87288607329111,-0.00247792941845921));
#26978=CARTESIAN_POINT('Origin',(43.7856267685719,0.,-3.14037644537578E-16));
#26979=CARTESIAN_POINT('',(44.,9.5,-1.16341445918999E-15));
#26980=CARTESIAN_POINT('Origin',(44.,0.,0.));
#26981=CARTESIAN_POINT('',(43.5712535371437,10.2572478777138,1.25615057815031E-15));
#26982=CARTESIAN_POINT('',(43.7856267685719,9.87862393885688,1.20978251867015E-15));
#26983=CARTESIAN_POINT('',(43.5712535371437,-10.2572478777138,-1.25615057815031E-15));
#26984=CARTESIAN_POINT('Origin',(43.5712535371437,0.,-6.28075289075157E-16));
#26985=CARTESIAN_POINT('Origin',(43.5712535371437,0.,-6.28075289075157E-16));
#26986=CARTESIAN_POINT('Origin',(43.5,0.,0.));
#26987=CARTESIAN_POINT('',(43.,-10.6,-1.29812560709619E-15));
#26988=CARTESIAN_POINT('',(43.5,-10.3,-1.26138620312177E-15));
#26989=CARTESIAN_POINT('Origin',(43.,0.,0.));
#26990=CARTESIAN_POINT('Origin',(44.,8.8,0.));
#26991=CARTESIAN_POINT('',(44.,-8.8,-1.07768918324967E-15));
#26992=CARTESIAN_POINT('Origin',(44.,0.,0.));
#26993=CARTESIAN_POINT('Origin',(0.,8.73662794227019,5.0440944942793));
#26994=CARTESIAN_POINT('',(0.376949928312602,8.73662794227019,5.0440944942793));
#26995=CARTESIAN_POINT('',(0.6,8.52364026992269,5.41299996417101));
#26996=CARTESIAN_POINT('',(0.770188275695485,8.36112965323919,5.69447660903617));
#26997=CARTESIAN_POINT('',(6.5,8.52364026992269,5.41299996417101));
#26998=CARTESIAN_POINT('',(0.,8.52364026992269,5.41299996417101));
#26999=CARTESIAN_POINT('',(6.5,8.9496156146177,4.67518902438759));
#27000=CARTESIAN_POINT('',(6.5,10.1116279422702,2.66252463387209));
#27001=CARTESIAN_POINT('',(0.6,8.9496156146177,4.67518902438759));
#27002=CARTESIAN_POINT('',(0.,8.9496156146177,4.67518902438759));
#27003=CARTESIAN_POINT('',(1.01481910015687,9.34572108958711,3.98911421658436));
#27004=CARTESIAN_POINT('Origin',(0.,8.96336292916894,5.175));
#27005=CARTESIAN_POINT('',(0.6,6.50538238691624,6.50538238691624));
#27006=CARTESIAN_POINT('',(0.6,6.58029128183,6.46483793479242));
#27007=CARTESIAN_POINT('',(6.5,6.50538238691624,6.50538238691624));
#27008=CARTESIAN_POINT('',(0.,6.50538238691624,6.50538238691624));
#27009=CARTESIAN_POINT('',(6.5,10.8341236570311,4.16245043758503));
#27010=CARTESIAN_POINT('Origin',(0.3,6.43749130332739,6.20100433924467));
#27011=CARTESIAN_POINT('',(0.,8.3534505847788,4.82286694378428));
#27012=CARTESIAN_POINT('',(0.,8.3534505847788,4.82286694378428));
#27013=CARTESIAN_POINT('',(0.,6.06272341459609,6.06272341459609));
#27014=CARTESIAN_POINT('',(0.,6.29469132482479,5.93717074369692));
#27015=CARTESIAN_POINT('',(0.,6.06272341459609,6.06272341459609));
#27016=CARTESIAN_POINT('Origin',(0.3,8.55055027477236,1.07759644317218));
#27017=CARTESIAN_POINT('',(0.6,8.88651760185943,2.38113521494319));
#27018=CARTESIAN_POINT('',(0.6,8.85043686013981,1.06934805444143));
#27019=CARTESIAN_POINT('',(0.,8.28183420045699,2.2191107858609));
#27020=CARTESIAN_POINT('',(0.,8.28183420045699,2.2191107858609));
#27021=CARTESIAN_POINT('',(0.,8.25066368940492,1.08584483190292));
#27022=CARTESIAN_POINT('Origin',(0.,5.0440944942793,8.73662794227019));
#27023=CARTESIAN_POINT('',(0.376949928312603,5.0440944942793,8.73662794227019));
#27024=CARTESIAN_POINT('',(0.6,4.67518902438759,8.9496156146177));
#27025=CARTESIAN_POINT('',(0.770188275695485,4.39371237952243,9.11212623130119));
#27026=CARTESIAN_POINT('',(6.5,4.67518902438759,8.9496156146177));
#27027=CARTESIAN_POINT('',(0.,4.67518902438759,8.9496156146177));
#27028=CARTESIAN_POINT('',(6.5,5.41299996417101,8.52364026992268));
#27029=CARTESIAN_POINT('',(6.5,9.1690944942793,6.35505808186298));
#27030=CARTESIAN_POINT('',(0.6,5.41299996417101,8.52364026992269));
#27031=CARTESIAN_POINT('',(0.,5.41299996417101,8.52364026992268));
#27032=CARTESIAN_POINT('',(1.01481910015687,6.09907477197424,8.12753479495327));
#27033=CARTESIAN_POINT('Origin',(0.,5.175,8.96336292916894));
#27034=CARTESIAN_POINT('',(0.6,2.38113521494319,8.88651760185943));
#27035=CARTESIAN_POINT('',(0.6,2.46628044696984,8.88885952379457));
#27036=CARTESIAN_POINT('',(6.5,2.38113521494319,8.88651760185943));
#27037=CARTESIAN_POINT('',(0.,2.38113521494319,8.88651760185943));
#27038=CARTESIAN_POINT('',(6.5,7.96212269650768,9.04002281514855));
#27039=CARTESIAN_POINT('Origin',(0.3,2.47452883570058,8.58897293842712));
#27040=CARTESIAN_POINT('',(0.,4.82286694378428,8.3534505847788));
#27041=CARTESIAN_POINT('',(0.,4.82286694378428,8.3534505847788));
#27042=CARTESIAN_POINT('',(0.,2.2191107858609,8.28183420045699));
#27043=CARTESIAN_POINT('',(0.,2.48277722443133,8.28908635305967));
#27044=CARTESIAN_POINT('',(0.,2.2191107858609,8.28183420045699));
#27045=CARTESIAN_POINT('Origin',(0.3,6.86619553270279,5.20850103220104));
#27046=CARTESIAN_POINT('',(0.6,7.13002912825054,5.35130101070365));
#27047=CARTESIAN_POINT('',(0.,6.60236193715504,5.06570105369843));
#27048=CARTESIAN_POINT('Origin',(0.,2.98372437868011E-15,10.0881889885586));
#27049=CARTESIAN_POINT('',(0.376949928312603,5.01337711727344E-16,10.0881889885586));
#27050=CARTESIAN_POINT('',(0.6,-0.425975344695007,10.0881889885586));
#27051=CARTESIAN_POINT('',(0.770188275695485,-0.750996578061993,10.0881889885586));
#27052=CARTESIAN_POINT('',(6.5,-0.425975344695008,10.0881889885586));
#27053=CARTESIAN_POINT('',(0.,-0.425975344695007,10.0881889885586));
#27054=CARTESIAN_POINT('',(6.5,0.425975344695013,10.0881889885586));
#27055=CARTESIAN_POINT('',(6.5,5.50000000000002,10.0881889885586));
#27056=CARTESIAN_POINT('',(0.6,0.425975344695013,10.0881889885586));
#27057=CARTESIAN_POINT('',(0.,0.425975344695013,10.0881889885586));
#27058=CARTESIAN_POINT('',(1.01481910015687,1.21818629463384,10.0881889885586));
#27059=CARTESIAN_POINT('Origin',(0.,6.33754718558755E-16,10.35));
#27060=CARTESIAN_POINT('',(0.6,-2.38113521494319,8.88651760185943));
#27061=CARTESIAN_POINT('',(0.6,-2.30856824196456,8.93111838176226));
#27062=CARTESIAN_POINT('',(6.5,-2.38113521494319,8.88651760185943));
#27063=CARTESIAN_POINT('',(0.,-2.38113521494319,8.88651760185943));
#27064=CARTESIAN_POINT('',(6.5,1.68344163237214,11.3846691703236));
#27065=CARTESIAN_POINT('Origin',(0.3,-2.15148163509972,8.67553317494525));
#27066=CARTESIAN_POINT('',(0.,5.55111512312578E-16,9.64573388756855));
#27067=CARTESIAN_POINT('',(0.,2.77555756156289E-16,9.64573388756855));
#27068=CARTESIAN_POINT('',(0.,-2.21911078586091,8.28183420045699));
#27069=CARTESIAN_POINT('',(0.,-1.99439502823489,8.41994796812825));
#27070=CARTESIAN_POINT('',(0.,-2.21911078586091,8.28183420045699));
#27071=CARTESIAN_POINT('Origin',(0.3,3.34204924257132,7.94379197587497));
#27072=CARTESIAN_POINT('',(0.6,3.49913584943616,8.19937718269197));
#27073=CARTESIAN_POINT('',(0.,3.18496263570648,7.68820676905796));
#27074=CARTESIAN_POINT('Origin',(0.,-5.0440944942793,8.73662794227019));
#27075=CARTESIAN_POINT('',(0.376949928312603,-5.0440944942793,8.73662794227019));
#27076=CARTESIAN_POINT('',(0.6,-5.41299996417101,8.52364026992269));
#27077=CARTESIAN_POINT('',(0.770188275695485,-5.69447660903617,8.36112965323919));
#27078=CARTESIAN_POINT('',(6.5,-5.41299996417101,8.52364026992269));
#27079=CARTESIAN_POINT('',(0.,-5.41299996417101,8.52364026992269));
#27080=CARTESIAN_POINT('',(6.5,-4.67518902438759,8.9496156146177));
#27081=CARTESIAN_POINT('',(6.5,-0.919094494279296,11.1181978026774));
#27082=CARTESIAN_POINT('',(0.6,-4.67518902438759,8.9496156146177));
#27083=CARTESIAN_POINT('',(0.,-4.67518902438759,8.9496156146177));
#27084=CARTESIAN_POINT('',(1.01481910015687,-3.98911421658436,9.34572108958711));
#27085=CARTESIAN_POINT('Origin',(0.,-5.175,8.96336292916894));
#27086=CARTESIAN_POINT('',(0.6,-6.50538238691624,6.50538238691624));
#27087=CARTESIAN_POINT('',(0.6,-6.46483793479242,6.58029128183));
#27088=CARTESIAN_POINT('',(6.5,-6.50538238691624,6.50538238691624));
#27089=CARTESIAN_POINT('',(0.,-6.50538238691624,6.50538238691624));
#27090=CARTESIAN_POINT('',(6.5,-5.21867030999356,8.88267877903739));
#27091=CARTESIAN_POINT('Origin',(0.3,-6.20100433924467,6.4374913033274));
#27092=CARTESIAN_POINT('',(0.,-4.82286694378427,8.3534505847788));
#27093=CARTESIAN_POINT('',(0.,-4.82286694378427,8.3534505847788));
#27094=CARTESIAN_POINT('',(0.,-6.06272341459609,6.06272341459609));
#27095=CARTESIAN_POINT('',(0.,-5.93717074369692,6.29469132482479));
#27096=CARTESIAN_POINT('',(0.,-6.06272341459609,6.06272341459609));
#27097=CARTESIAN_POINT('Origin',(0.3,-1.07759644317218,8.55055027477236));
#27098=CARTESIAN_POINT('',(0.6,-1.06934805444143,8.85043686013981));
#27099=CARTESIAN_POINT('',(0.,-1.08584483190292,8.25066368940492));
#27100=CARTESIAN_POINT('Origin',(0.,-8.73662794227019,5.0440944942793));
#27101=CARTESIAN_POINT('',(0.376949928312603,-8.73662794227019,5.0440944942793));
#27102=CARTESIAN_POINT('',(0.6,-8.9496156146177,4.67518902438759));
#27103=CARTESIAN_POINT('',(0.770188275695485,-9.11212623130119,4.39371237952243));
#27104=CARTESIAN_POINT('',(6.5,-8.9496156146177,4.67518902438759));
#27105=CARTESIAN_POINT('',(0.,-8.9496156146177,4.67518902438759));
#27106=CARTESIAN_POINT('',(6.5,-8.52364026992269,5.41299996417101));
#27107=CARTESIAN_POINT('',(6.5,-7.36162794227019,7.42566435468651));
#27108=CARTESIAN_POINT('',(0.6,-8.52364026992269,5.41299996417101));
#27109=CARTESIAN_POINT('',(0.,-8.52364026992269,5.41299996417101));
#27110=CARTESIAN_POINT('',(1.01481910015687,-8.12753479495327,6.09907477197424));
#27111=CARTESIAN_POINT('Origin',(0.,-8.96336292916894,5.175));
#27112=CARTESIAN_POINT('',(0.6,-8.88651760185943,2.38113521494319));
#27113=CARTESIAN_POINT('',(0.6,-8.88885952379457,2.46628044696983));
#27114=CARTESIAN_POINT('',(6.5,-8.88651760185943,2.38113521494319));
#27115=CARTESIAN_POINT('',(0.,-8.88651760185943,2.38113521494319));
#27116=CARTESIAN_POINT('',(6.5,-8.88470177333241,2.31511715561584));
#27117=CARTESIAN_POINT('Origin',(0.3,-8.58897293842712,2.47452883570058));
#27118=CARTESIAN_POINT('',(0.,-8.3534505847788,4.82286694378428));
#27119=CARTESIAN_POINT('',(0.,-8.3534505847788,4.82286694378428));
#27120=CARTESIAN_POINT('',(0.,-8.281834200457,2.21911078586091));
#27121=CARTESIAN_POINT('',(0.,-8.28908635305967,2.48277722443133));
#27122=CARTESIAN_POINT('',(0.,-8.281834200457,2.21911078586091));
#27123=CARTESIAN_POINT('Origin',(0.3,-5.20850103220104,6.86619553270279));
#27124=CARTESIAN_POINT('',(0.6,-5.35130101070365,7.13002912825054));
#27125=CARTESIAN_POINT('',(0.,-5.06570105369844,6.60236193715504));
#27126=CARTESIAN_POINT('Origin',(0.,10.0881889885586,-3.46944695195361E-16));
#27127=CARTESIAN_POINT('',(0.376949928312603,10.0881889885586,-4.12725542052732E-16));
#27128=CARTESIAN_POINT('',(0.6,10.0881889885586,0.425975344695008));
#27129=CARTESIAN_POINT('',(0.770188275695485,10.0881889885586,0.750996578061995));
#27130=CARTESIAN_POINT('',(6.5,10.0881889885586,0.425975344695008));
#27131=CARTESIAN_POINT('',(0.,10.0881889885586,0.425975344695009));
#27132=CARTESIAN_POINT('',(6.5,10.0881889885586,-0.42597534469501));
#27133=CARTESIAN_POINT('',(6.5,10.0881889885586,1.01475790048603E-15));
#27134=CARTESIAN_POINT('',(0.6,10.0881889885586,-0.42597534469501));
#27135=CARTESIAN_POINT('',(0.,10.0881889885586,-0.42597534469501));
#27136=CARTESIAN_POINT('',(1.01481910015687,10.0881889885586,-1.21818629463384));
#27137=CARTESIAN_POINT('Origin',(0.,10.35,0.));
#27138=CARTESIAN_POINT('',(0.6,8.93111838176226,2.30856824196456));
#27139=CARTESIAN_POINT('',(6.5,8.88651760185943,2.38113521494319));
#27140=CARTESIAN_POINT('',(0.,8.88651760185943,2.38113521494319));
#27141=CARTESIAN_POINT('',(6.5,10.4391085074256,-0.144982546596809));
#27142=CARTESIAN_POINT('Origin',(0.3,8.67553317494525,2.15148163509972));
#27143=CARTESIAN_POINT('',(0.,9.64573388756855,-1.11022302462516E-15));
#27144=CARTESIAN_POINT('',(0.,9.64573388756855,-1.11022302462516E-15));
#27145=CARTESIAN_POINT('',(0.,8.41994796812825,1.99439502823489));
#27146=CARTESIAN_POINT('Origin',(0.3,7.94379197587497,-3.34204924257132));
#27147=CARTESIAN_POINT('',(0.6,8.88651760185943,-2.38113521494319));
#27148=CARTESIAN_POINT('',(0.6,8.19937718269197,-3.49913584943616));
#27149=CARTESIAN_POINT('',(0.,8.28183420045699,-2.2191107858609));
#27150=CARTESIAN_POINT('',(0.6,8.88651760185943,-2.38113521494319));
#27151=CARTESIAN_POINT('',(0.,7.68820676905796,-3.18496263570648));
#27152=CARTESIAN_POINT('Origin',(0.,8.73662794227019,-5.0440944942793));
#27153=CARTESIAN_POINT('',(0.376949928312602,8.73662794227019,-5.0440944942793));
#27154=CARTESIAN_POINT('',(0.6,8.94961561461769,-4.67518902438759));
#27155=CARTESIAN_POINT('',(0.770188275695484,9.11212623130119,-4.39371237952243));
#27156=CARTESIAN_POINT('',(6.5,8.94961561461769,-4.67518902438759));
#27157=CARTESIAN_POINT('',(0.,8.94961561461769,-4.67518902438759));
#27158=CARTESIAN_POINT('',(6.5,8.52364026992268,-5.41299996417101));
#27159=CARTESIAN_POINT('',(6.5,10.1116279422702,-2.6625246338721));
#27160=CARTESIAN_POINT('',(0.6,8.52364026992268,-5.41299996417102));
#27161=CARTESIAN_POINT('',(0.,8.52364026992268,-5.41299996417101));
#27162=CARTESIAN_POINT('',(1.01481910015687,8.12753479495326,-6.09907477197424));
#27163=CARTESIAN_POINT('Origin',(0.,8.96336292916894,-5.175));
#27164=CARTESIAN_POINT('',(0.6,8.88885952379457,-2.46628044696984));
#27165=CARTESIAN_POINT('',(6.5,8.88651760185943,-2.38113521494319));
#27166=CARTESIAN_POINT('',(0.,8.88651760185943,-2.38113521494319));
#27167=CARTESIAN_POINT('',(6.5,8.89301727425672,-2.61744373832382));
#27168=CARTESIAN_POINT('Origin',(0.3,8.58897293842712,-2.47452883570059));
#27169=CARTESIAN_POINT('',(0.,8.3534505847788,-4.82286694378428));
#27170=CARTESIAN_POINT('',(0.,8.3534505847788,-4.82286694378428));
#27171=CARTESIAN_POINT('',(0.,8.28908635305967,-2.48277722443133));
#27172=CARTESIAN_POINT('Origin',(0.,5.0440944942793,-8.73662794227019));
#27173=CARTESIAN_POINT('',(0.376949928312603,5.0440944942793,-8.73662794227019));
#27174=CARTESIAN_POINT('',(0.6,5.41299996417101,-8.52364026992269));
#27175=CARTESIAN_POINT('',(0.770188275695485,5.69447660903618,-8.36112965323919));
#27176=CARTESIAN_POINT('',(6.5,5.41299996417101,-8.52364026992269));
#27177=CARTESIAN_POINT('',(0.,5.41299996417101,-8.52364026992269));
#27178=CARTESIAN_POINT('',(6.5,4.67518902438759,-8.9496156146177));
#27179=CARTESIAN_POINT('',(6.5,9.1690944942793,-6.35505808186299));
#27180=CARTESIAN_POINT('',(0.6,4.67518902438759,-8.9496156146177));
#27181=CARTESIAN_POINT('',(0.,4.67518902438759,-8.9496156146177));
#27182=CARTESIAN_POINT('',(1.01481910015687,3.98911421658436,-9.34572108958711));
#27183=CARTESIAN_POINT('Origin',(0.,5.175,-8.96336292916894));
#27184=CARTESIAN_POINT('',(0.6,6.50538238691624,-6.50538238691624));
#27185=CARTESIAN_POINT('',(0.6,6.46483793479242,-6.58029128183));
#27186=CARTESIAN_POINT('',(6.5,6.50538238691624,-6.50538238691624));
#27187=CARTESIAN_POINT('',(0.,6.50538238691624,-6.50538238691624));
#27188=CARTESIAN_POINT('',(6.5,7.71100555959128,-4.27790378462261));
#27189=CARTESIAN_POINT('Origin',(0.3,6.20100433924467,-6.43749130332739));
#27190=CARTESIAN_POINT('',(0.,4.82286694378428,-8.3534505847788));
#27191=CARTESIAN_POINT('',(0.,4.82286694378428,-8.3534505847788));
#27192=CARTESIAN_POINT('',(0.,6.06272341459609,-6.06272341459609));
#27193=CARTESIAN_POINT('',(0.,5.93717074369692,-6.29469132482479));
#27194=CARTESIAN_POINT('',(0.,6.06272341459609,-6.06272341459609));
#27195=CARTESIAN_POINT('Origin',(0.3,1.07759644317218,-8.55055027477237));
#27196=CARTESIAN_POINT('',(0.6,2.38113521494319,-8.88651760185943));
#27197=CARTESIAN_POINT('',(0.6,1.06934805444143,-8.85043686013981));
#27198=CARTESIAN_POINT('',(0.,2.2191107858609,-8.281834200457));
#27199=CARTESIAN_POINT('',(0.,2.2191107858609,-8.281834200457));
#27200=CARTESIAN_POINT('',(0.,1.08584483190293,-8.25066368940492));
#27201=CARTESIAN_POINT('Origin',(0.,-3.53883589099269E-15,-10.0881889885586));
#27202=CARTESIAN_POINT('',(0.376949928312603,-1.0912875931293E-15,-10.0881889885586));
#27203=CARTESIAN_POINT('',(0.6,0.425975344695006,-10.0881889885586));
#27204=CARTESIAN_POINT('',(0.770188275695485,0.750996578061993,-10.0881889885586));
#27205=CARTESIAN_POINT('',(6.5,0.425975344695005,-10.0881889885586));
#27206=CARTESIAN_POINT('',(0.,0.425975344695005,-10.0881889885586));
#27207=CARTESIAN_POINT('',(6.5,-0.425975344695013,-10.0881889885586));
#27208=CARTESIAN_POINT('',(6.5,5.49999999999998,-10.0881889885586));
#27209=CARTESIAN_POINT('',(0.6,-0.425975344695012,-10.0881889885586));
#27210=CARTESIAN_POINT('',(0.,-0.425975344695013,-10.0881889885586));
#27211=CARTESIAN_POINT('',(1.01481910015687,-1.21818629463384,-10.0881889885586));
#27212=CARTESIAN_POINT('Origin',(0.,-1.90126415567627E-15,-10.35));
#27213=CARTESIAN_POINT('',(0.6,2.30856824196456,-8.93111838176226));
#27214=CARTESIAN_POINT('',(6.5,2.38113521494319,-8.88651760185943));
#27215=CARTESIAN_POINT('',(0.,2.38113521494319,-8.88651760185943));
#27216=CARTESIAN_POINT('',(6.5,6.30057811630126,-6.47756759320089));
#27217=CARTESIAN_POINT('Origin',(0.3,2.15148163509972,-8.67553317494525));
#27218=CARTESIAN_POINT('',(0.,0.,-9.64573388756855));
#27219=CARTESIAN_POINT('',(0.,2.77555756156289E-16,-9.64573388756855));
#27220=CARTESIAN_POINT('',(0.,1.99439502823488,-8.41994796812825));
#27221=CARTESIAN_POINT('Origin',(0.3,-3.34204924257132,-7.94379197587497));
#27222=CARTESIAN_POINT('',(0.6,-2.38113521494319,-8.88651760185943));
#27223=CARTESIAN_POINT('',(0.6,-3.49913584943616,-8.19937718269197));
#27224=CARTESIAN_POINT('',(0.,-2.2191107858609,-8.28183420045699));
#27225=CARTESIAN_POINT('',(0.,-2.2191107858609,-8.28183420045699));
#27226=CARTESIAN_POINT('',(0.,-3.18496263570648,-7.68820676905796));
#27227=CARTESIAN_POINT('Origin',(0.,-5.0440944942793,-8.73662794227019));
#27228=CARTESIAN_POINT('',(0.376949928312602,-5.0440944942793,-8.73662794227019));
#27229=CARTESIAN_POINT('',(0.6,-4.67518902438759,-8.94961561461769));
#27230=CARTESIAN_POINT('',(0.770188275695484,-4.39371237952243,-9.11212623130119));
#27231=CARTESIAN_POINT('',(6.5,-4.67518902438759,-8.94961561461769));
#27232=CARTESIAN_POINT('',(0.,-4.67518902438759,-8.94961561461769));
#27233=CARTESIAN_POINT('',(6.5,-5.41299996417102,-8.52364026992268));
#27234=CARTESIAN_POINT('',(6.5,-0.919094494279309,-11.1181978026774));
#27235=CARTESIAN_POINT('',(0.6,-5.41299996417101,-8.52364026992268));
#27236=CARTESIAN_POINT('',(0.,-5.41299996417101,-8.52364026992268));
#27237=CARTESIAN_POINT('',(1.01481910015687,-6.09907477197424,-8.12753479495327));
#27238=CARTESIAN_POINT('Origin',(0.,-5.175,-8.96336292916894));
#27239=CARTESIAN_POINT('',(0.6,-2.46628044696984,-8.88885952379457));
#27240=CARTESIAN_POINT('',(6.5,-2.38113521494319,-8.88651760185943));
#27241=CARTESIAN_POINT('',(0.,-2.38113521494319,-8.88651760185943));
#27242=CARTESIAN_POINT('',(6.5,3.029561802568,-8.73769623244058));
#27243=CARTESIAN_POINT('Origin',(0.3,-2.47452883570059,-8.58897293842712));
#27244=CARTESIAN_POINT('',(0.,-4.82286694378428,-8.3534505847788));
#27245=CARTESIAN_POINT('',(0.,-4.82286694378428,-8.3534505847788));
#27246=CARTESIAN_POINT('',(0.,-2.48277722443133,-8.28908635305967));
#27247=CARTESIAN_POINT('Origin',(0.3,-6.86619553270279,-5.20850103220104));
#27248=CARTESIAN_POINT('',(0.6,-6.50538238691624,-6.50538238691624));
#27249=CARTESIAN_POINT('',(0.6,-7.13002912825054,-5.35130101070365));
#27250=CARTESIAN_POINT('',(0.,-6.06272341459609,-6.06272341459609));
#27251=CARTESIAN_POINT('',(0.,-6.06272341459609,-6.06272341459609));
#27252=CARTESIAN_POINT('',(0.,-6.60236193715504,-5.06570105369843));
#27253=CARTESIAN_POINT('Origin',(0.,-8.73662794227019,-5.0440944942793));
#27254=CARTESIAN_POINT('',(0.376949928312602,-8.73662794227019,-5.0440944942793));
#27255=CARTESIAN_POINT('',(0.6,-8.52364026992268,-5.41299996417101));
#27256=CARTESIAN_POINT('',(0.770188275695484,-8.36112965323919,-5.69447660903617));
#27257=CARTESIAN_POINT('',(6.5,-8.52364026992268,-5.41299996417101));
#27258=CARTESIAN_POINT('',(0.,-8.52364026992268,-5.41299996417101));
#27259=CARTESIAN_POINT('',(6.5,-8.9496156146177,-4.67518902438759));
#27260=CARTESIAN_POINT('',(6.5,-7.36162794227019,-7.42566435468651));
#27261=CARTESIAN_POINT('',(0.6,-8.9496156146177,-4.67518902438759));
#27262=CARTESIAN_POINT('',(0.,-8.9496156146177,-4.67518902438759));
#27263=CARTESIAN_POINT('',(1.01481910015687,-9.34572108958711,-3.98911421658436));
#27264=CARTESIAN_POINT('Origin',(0.,-8.96336292916894,-5.175));
#27265=CARTESIAN_POINT('',(0.6,-6.58029128183,-6.46483793479242));
#27266=CARTESIAN_POINT('',(6.5,-6.50538238691624,-6.50538238691624));
#27267=CARTESIAN_POINT('',(0.,-6.50538238691624,-6.50538238691624));
#27268=CARTESIAN_POINT('',(6.5,-2.32645890662886,-8.76722543199981));
#27269=CARTESIAN_POINT('Origin',(0.3,-6.43749130332739,-6.20100433924467));
#27270=CARTESIAN_POINT('',(0.,-8.3534505847788,-4.82286694378428));
#27271=CARTESIAN_POINT('',(0.,-8.3534505847788,-4.82286694378428));
#27272=CARTESIAN_POINT('',(0.,-6.29469132482479,-5.93717074369692));
#27273=CARTESIAN_POINT('Origin',(0.3,-8.55055027477236,-1.07759644317218));
#27274=CARTESIAN_POINT('',(0.6,-8.88651760185943,-2.38113521494319));
#27275=CARTESIAN_POINT('',(0.6,-8.85043686013981,-1.06934805444143));
#27276=CARTESIAN_POINT('',(0.,-8.281834200457,-2.2191107858609));
#27277=CARTESIAN_POINT('',(0.,-8.281834200457,-2.2191107858609));
#27278=CARTESIAN_POINT('',(0.,-8.25066368940492,-1.08584483190293));
#27279=CARTESIAN_POINT('Origin',(0.,-10.0881889885586,1.04083408558608E-15));
#27280=CARTESIAN_POINT('',(0.376949928312603,-10.0881889885586,1.41540096550742E-15));
#27281=CARTESIAN_POINT('',(0.6,-10.0881889885586,-0.425975344695007));
#27282=CARTESIAN_POINT('',(0.770188275695486,-10.0881889885586,-0.750996578061997));
#27283=CARTESIAN_POINT('',(6.5,-10.0881889885586,-0.425975344695008));
#27284=CARTESIAN_POINT('',(0.,-10.0881889885586,-0.425975344695008));
#27285=CARTESIAN_POINT('',(6.5,-10.0881889885586,0.42597534469501));
#27286=CARTESIAN_POINT('',(6.5,-10.0881889885586,5.20417042793042E-16));
#27287=CARTESIAN_POINT('',(0.6,-10.0881889885586,0.425975344695009));
#27288=CARTESIAN_POINT('',(0.,-10.0881889885586,0.42597534469501));
#27289=CARTESIAN_POINT('',(1.01481910015687,-10.0881889885586,1.21818629463384));
#27290=CARTESIAN_POINT('Origin',(0.,-10.35,1.26750943711751E-15));
#27291=CARTESIAN_POINT('',(0.6,-8.93111838176226,-2.30856824196456));
#27292=CARTESIAN_POINT('',(6.5,-8.88651760185943,-2.38113521494319));
#27293=CARTESIAN_POINT('',(0.,-8.88651760185943,-2.38113521494319));
#27294=CARTESIAN_POINT('',(6.5,-7.42312825609896,-4.76211903052593));
#27295=CARTESIAN_POINT('Origin',(0.3,-8.67553317494525,-2.15148163509972));
#27296=CARTESIAN_POINT('',(0.,-9.64573388756855,2.22044604925031E-15));
#27297=CARTESIAN_POINT('',(0.,-9.64573388756855,1.66533453693773E-15));
#27298=CARTESIAN_POINT('',(0.,-8.41994796812825,-1.99439502823488));
#27299=CARTESIAN_POINT('Origin',(0.3,-7.94379197587497,3.34204924257132));
#27300=CARTESIAN_POINT('',(0.6,-8.19937718269197,3.49913584943616));
#27301=CARTESIAN_POINT('',(0.,-7.68820676905796,3.18496263570648));
#27302=CARTESIAN_POINT('Origin',(40.65,0.,0.));
#27303=CARTESIAN_POINT('',(40.4,34.9678423698117,1.5));
#27304=CARTESIAN_POINT('',(40.9,34.4673758792282,1.5));
#27305=CARTESIAN_POINT('Ctrl Pts',(40.4,34.9678423698117,1.5));
#27306=CARTESIAN_POINT('Ctrl Pts',(40.5666590135434,34.801030090909,1.5));
#27307=CARTESIAN_POINT('Ctrl Pts',(40.7333430449885,34.6341905786716,1.5));
#27308=CARTESIAN_POINT('Ctrl Pts',(40.9,34.4673758792282,1.5));
#27309=CARTESIAN_POINT('',(40.9,34.4673758792282,-1.50000000000001));
#27310=CARTESIAN_POINT('Origin',(40.9,0.,0.));
#27311=CARTESIAN_POINT('',(40.4,34.9678423698117,-1.5));
#27312=CARTESIAN_POINT('Ctrl Pts',(40.9,34.4673758792282,-1.5));
#27313=CARTESIAN_POINT('Ctrl Pts',(40.7333430449627,34.6341905786974,-1.5));
#27314=CARTESIAN_POINT('Ctrl Pts',(40.5666590137774,34.8010300906748,-1.5));
#27315=CARTESIAN_POINT('Ctrl Pts',(40.4,34.9678423698117,-1.5));
#27316=CARTESIAN_POINT('Origin',(40.4,0.,0.));
#27317=CARTESIAN_POINT('Origin',(35.7,0.,0.));
#27318=CARTESIAN_POINT('',(30.5,34.9656486014478,-1.55029606206997));
#27319=CARTESIAN_POINT('Ctrl Pts',(40.3999921398529,34.9678423429768,-1.49999538724755));
#27320=CARTESIAN_POINT('Ctrl Pts',(39.2499570215113,34.9678422244593,-1.49997501500716));
#27321=CARTESIAN_POINT('Ctrl Pts',(38.0998114916604,34.9678417480135,-1.49989311899335));
#27322=CARTESIAN_POINT('Ctrl Pts',(36.9497038557168,34.9678416168427,-1.49987059349837));
#27323=CARTESIAN_POINT('Ctrl Pts',(36.785105117964,34.96784159807,-1.49986736974093));
#27324=CARTESIAN_POINT('Ctrl Pts',(36.6205071563607,34.9678415863694,-1.49986536202073));
#27325=CARTESIAN_POINT('Ctrl Pts',(36.4559233022361,34.9678415707796,-1.49986268095531));
#27326=CARTESIAN_POINT('Ctrl Pts',(36.4193640724435,34.9678415673166,-1.4998620854067));
#27327=CARTESIAN_POINT('Ctrl Pts',(36.3828055387466,34.9678415636617,-1.49986145663366));
#27328=CARTESIAN_POINT('Ctrl Pts',(36.3462474593958,34.967841559861,-1.49986080263032));
#27329=CARTESIAN_POINT('Ctrl Pts',(36.0895450699579,34.967841533173,-1.49985621036995));
#27330=CARTESIAN_POINT('Ctrl Pts',(35.8501671305851,34.9678416196704,-1.49985084735668));
#27331=CARTESIAN_POINT('Ctrl Pts',(35.6266230092018,34.9678417642539,-1.49984692867086));
#27332=CARTESIAN_POINT('Ctrl Pts',(35.5729810992077,34.9678417989483,-1.49984598833841));
#27333=CARTESIAN_POINT('Ctrl Pts',(35.5202511626857,34.9678418369404,-1.49984512300934));
#27334=CARTESIAN_POINT('Ctrl Pts',(35.4684130151836,34.9678418773881,-1.4998443492858));
#27335=CARTESIAN_POINT('Ctrl Pts',(35.3128073279263,34.9678419988026,-1.49984202675329));
#27336=CARTESIAN_POINT('Ctrl Pts',(35.1652418679138,34.9678421408902,-1.49984027810624));
#27337=CARTESIAN_POINT('Ctrl Pts',(35.0252627275547,34.967842254217,-1.49983493809963));
#27338=CARTESIAN_POINT('Ctrl Pts',(35.0082618963838,34.9678422679808,-1.49983428954192));
#27339=CARTESIAN_POINT('Ctrl Pts',(34.9913729068342,34.9678422813397,-1.49983359135557));
#27340=CARTESIAN_POINT('Ctrl Pts',(34.9745948969331,34.9678422942204,-1.49983283870325));
#27341=CARTESIAN_POINT('Ctrl Pts',(34.8399133402553,34.9678423976168,-1.49982679696251));
#27342=CARTESIAN_POINT('Ctrl Pts',(34.7123780512931,34.9678424712592,-1.49981743040037));
#27343=CARTESIAN_POINT('Ctrl Pts',(34.591404591981,34.9678425127826,-1.49980840280397));
#27344=CARTESIAN_POINT('Ctrl Pts',(34.4539348326465,34.9678425599684,-1.49979814417771));
#27345=CARTESIAN_POINT('Ctrl Pts',(34.3249390274092,34.9678425655798,-1.49978830616204));
#27346=CARTESIAN_POINT('Ctrl Pts',(34.2036312646158,34.9678425105859,-1.49978156609768));
#27347=CARTESIAN_POINT('Ctrl Pts',(34.1284740534062,34.967842476514,-1.49977739023598));
#27348=CARTESIAN_POINT('Ctrl Pts',(34.0562692606603,34.9678424188851,-1.49977435262848));
#27349=CARTESIAN_POINT('Ctrl Pts',(33.9868395791739,34.9678423310509,-1.49977272195139));
#27350=CARTESIAN_POINT('Ctrl Pts',(33.944569913827,34.9678422775764,-1.49977172917461));
#27351=CARTESIAN_POINT('Ctrl Pts',(33.903332682828,34.9678422127028,-1.49977122168105));
#27352=CARTESIAN_POINT('Ctrl Pts',(33.8632274501546,34.9678421281365,-1.49977004757329));
#27353=CARTESIAN_POINT('Ctrl Pts',(33.8167531035319,34.9678420301403,-1.49976868700542));
#27354=CARTESIAN_POINT('Ctrl Pts',(33.771789463122,34.9678419060139,-1.49976648823776));
#27355=CARTESIAN_POINT('Ctrl Pts',(33.7281109635882,34.9678417565821,-1.49976414064438));
#27356=CARTESIAN_POINT('Ctrl Pts',(33.6812712011832,34.9678415963351,-1.49976162314223));
#27357=CARTESIAN_POINT('Ctrl Pts',(33.6359095723891,34.9678414069824,-1.49975893360226));
#27358=CARTESIAN_POINT('Ctrl Pts',(33.591810246565,34.9678411881909,-1.49975667024846));
#27359=CARTESIAN_POINT('Ctrl Pts',(33.5583448079856,34.9678410221577,-1.4997549526683));
#27360=CARTESIAN_POINT('Ctrl Pts',(33.5256076932742,34.9678408391413,-1.49975347489115));
#27361=CARTESIAN_POINT('Ctrl Pts',(33.4935243452377,34.9678406385663,-1.49975241817239));
#27362=CARTESIAN_POINT('Ctrl Pts',(33.4574180647961,34.9678404128412,-1.49975122895162));
#27363=CARTESIAN_POINT('Ctrl Pts',(33.4221459355308,34.9678401647559,-1.49975055002973));
#27364=CARTESIAN_POINT('Ctrl Pts',(33.3878318916215,34.9678398888653,-1.49974977143672));
#27365=CARTESIAN_POINT('Ctrl Pts',(33.3506903036195,34.9678395902407,-1.49974892868612));
#27366=CARTESIAN_POINT('Ctrl Pts',(33.3146710708563,34.9678392590421,-1.49974796966079));
#27367=CARTESIAN_POINT('Ctrl Pts',(33.2798677329257,34.967838889585,-1.49974635090117));
#27368=CARTESIAN_POINT('Ctrl Pts',(33.2432742079925,34.9678385011241,-1.49974464887706));
#27369=CARTESIAN_POINT('Ctrl Pts',(33.2080243245406,34.9678380703783,-1.49974221953694));
#27370=CARTESIAN_POINT('Ctrl Pts',(33.1741651388244,34.9678375919209,-1.4997386537707));
#27371=CARTESIAN_POINT('Ctrl Pts',(33.137063146823,34.96783706764,-1.49973474649923));
#27372=CARTESIAN_POINT('Ctrl Pts',(33.1016306515623,34.9678364860775,-1.49972947597288));
#27373=CARTESIAN_POINT('Ctrl Pts',(33.067864102108,34.9678358413429,-1.49972253958674));
#27374=CARTESIAN_POINT('Ctrl Pts',(33.0456526984032,34.967835417241,-1.49971797687971));
#27375=CARTESIAN_POINT('Ctrl Pts',(33.0241607955796,34.9678349658306,-1.49971269819094));
#27376=CARTESIAN_POINT('Ctrl Pts',(33.0033754048768,34.9678344856631,-1.49970666036488));
#27377=CARTESIAN_POINT('Ctrl Pts',(32.9442530209621,34.9678331198648,-1.49968948625086));
#27378=CARTESIAN_POINT('Ctrl Pts',(32.8887085075052,34.9678225692834,-1.49991335207053));
#27379=CARTESIAN_POINT('Ctrl Pts',(32.8362583193005,34.9678066670084,-1.50027559162313));
#27380=CARTESIAN_POINT('Ctrl Pts',(32.7773090712614,34.9677887942955,-1.50068271598181));
#27381=CARTESIAN_POINT('Ctrl Pts',(32.7222687069615,34.9677641462319,-1.50126502290934));
#27382=CARTESIAN_POINT('Ctrl Pts',(32.6704155259712,34.9677359487883,-1.50193537623735));
#27383=CARTESIAN_POINT('Ctrl Pts',(32.6144302418907,34.9677055043322,-1.50265914902788));
#27384=CARTESIAN_POINT('Ctrl Pts',(32.562160274654,34.967670888482,-1.50348644308881));
#27385=CARTESIAN_POINT('Ctrl Pts',(32.5126575741465,34.9676341575402,-1.50436077830378));
#27386=CARTESIAN_POINT('Ctrl Pts',(32.4592478825335,34.967594527616,-1.50530412025724));
#27387=CARTESIAN_POINT('Ctrl Pts',(32.4090594121702,34.9675524017484,-1.50630310623455));
#27388=CARTESIAN_POINT('Ctrl Pts',(32.3608584151774,34.9675086790575,-1.50733170420881));
#27389=CARTESIAN_POINT('Ctrl Pts',(32.3080624384018,34.9674607883018,-1.50845835797425));
#27390=CARTESIAN_POINT('Ctrl Pts',(32.2576510584103,34.9674109512874,-1.50962133088216));
#27391=CARTESIAN_POINT('Ctrl Pts',(32.2079531230124,34.9673589385144,-1.51082436306572));
#27392=CARTESIAN_POINT('Ctrl Pts',(32.1569814991446,34.9673055927269,-1.512058227279));
#27393=CARTESIAN_POINT('Ctrl Pts',(32.1067603493757,34.9672499217566,-1.51333518230822));
#27394=CARTESIAN_POINT('Ctrl Pts',(32.0554367657631,34.9671908102208,-1.51468303813505));
#27395=CARTESIAN_POINT('Ctrl Pts',(32.0053752916507,34.9671331523098,-1.51599774854364));
#27396=CARTESIAN_POINT('Ctrl Pts',(31.9542650752308,34.9670721879268,-1.51738077462803));
#27397=CARTESIAN_POINT('Ctrl Pts',(31.9003392718784,34.9670065776396,-1.51886693662987));
#27398=CARTESIAN_POINT('Ctrl Pts',(31.8778362033488,34.9669791986726,-1.51948710736994));
#27399=CARTESIAN_POINT('Ctrl Pts',(31.8548422465647,34.9669510097079,-1.52012527669195));
#27400=CARTESIAN_POINT('Ctrl Pts',(31.8312262657831,34.9669219190816,-1.5207838890893));
#27401=CARTESIAN_POINT('Ctrl Pts',(31.7273802318769,34.9667939995094,-1.52367999092727));
#27402=CARTESIAN_POINT('Ctrl Pts',(31.6210019634564,34.9666588880294,-1.52670831990391));
#27403=CARTESIAN_POINT('Ctrl Pts',(31.5129311113832,34.9665259706005,-1.52968152042074));
#27404=CARTESIAN_POINT('Ctrl Pts',(31.4048670765154,34.9663930615562,-1.53265453338543));
#27405=CARTESIAN_POINT('Ctrl Pts',(31.295110396828,34.9662624173991,-1.53557057541609));
#27406=CARTESIAN_POINT('Ctrl Pts',(31.1845493642852,34.9661438310284,-1.53823056067695));
#27407=CARTESIAN_POINT('Ctrl Pts',(31.1321570104766,34.9660876356498,-1.53949106707516));
#27408=CARTESIAN_POINT('Ctrl Pts',(31.0795847658967,34.9660341471942,-1.54069407696177));
#27409=CARTESIAN_POINT('Ctrl Pts',(31.0269312050905,34.9659843676727,-1.54181935957432));
#27410=CARTESIAN_POINT('Ctrl Pts',(30.9325025960689,34.9658950933502,-1.5438374352796));
#27411=CARTESIAN_POINT('Ctrl Pts',(30.8378102330027,34.9658178028119,-1.54560383003055));
#27412=CARTESIAN_POINT('Ctrl Pts',(30.743359924284,34.9657577677723,-1.54697518213503));
#27413=CARTESIAN_POINT('Ctrl Pts',(30.6608249248197,34.965705306409,-1.54817353232302));
#27414=CARTESIAN_POINT('Ctrl Pts',(30.5784749808876,34.9656660234083,-1.5490700665616));
#27415=CARTESIAN_POINT('Ctrl Pts',(30.4966730088978,34.9656427667437,-1.54959005157024));
#27416=CARTESIAN_POINT('',(30.5,34.9699609326822,1.44976976333442));
#27417=CARTESIAN_POINT('Origin',(30.5,0.,0.));
#27418=CARTESIAN_POINT('Ctrl Pts',(30.5051992612603,34.9699071381489,1.44903843638966));
#27419=CARTESIAN_POINT('Ctrl Pts',(30.6030952980657,34.9698787568567,1.44976082626916));
#27420=CARTESIAN_POINT('Ctrl Pts',(30.7001121880334,34.9698264221104,1.45104998650339));
#27421=CARTESIAN_POINT('Ctrl Pts',(30.7969947619801,34.9697577270266,1.45274237549662));
#27422=CARTESIAN_POINT('Ctrl Pts',(30.8545454823776,34.9697169203945,1.45374769773142));
#27423=CARTESIAN_POINT('Ctrl Pts',(30.9120492097055,34.9696702850817,1.45489634227782));
#27424=CARTESIAN_POINT('Ctrl Pts',(30.9696671110348,34.969619048359,1.45616096255286));
#27425=CARTESIAN_POINT('Ctrl Pts',(31.0687356284601,34.969530951673,1.45833535719175));
#27426=CARTESIAN_POINT('Ctrl Pts',(31.1681385828748,34.9694292858246,1.46085179879274));
#27427=CARTESIAN_POINT('Ctrl Pts',(31.2685908593294,34.9693191238307,1.46356721252908));
#27428=CARTESIAN_POINT('Ctrl Pts',(31.3711796386287,34.9692066188196,1.46634037995083));
#27429=CARTESIAN_POINT('Ctrl Pts',(31.4748629185041,34.9690851710715,1.46932276608686));
#27430=CARTESIAN_POINT('Ctrl Pts',(31.5804543970455,34.9689598486836,1.47236951553031));
#27431=CARTESIAN_POINT('Ctrl Pts',(31.6427002532107,34.9688859715163,1.47416556508136));
#27432=CARTESIAN_POINT('Ctrl Pts',(31.7056101943778,34.9688107472907,1.47598400420438));
#27433=CARTESIAN_POINT('Ctrl Pts',(31.7693590594472,34.9687353433411,1.47779256103941));
#27434=CARTESIAN_POINT('Ctrl Pts',(31.8369567664636,34.9686553868731,1.47971030961302));
#27435=CARTESIAN_POINT('Ctrl Pts',(31.8998289473024,34.9685826953726,1.4814535614827));
#27436=CARTESIAN_POINT('Ctrl Pts',(31.9584912820088,34.9685172658125,1.48302365833457));
#27437=CARTESIAN_POINT('Ctrl Pts',(32.0219681801222,34.9684464662861,1.484722616932));
#27438=CARTESIAN_POINT('Ctrl Pts',(32.0805160965731,34.9683841232146,1.48621979971339));
#27439=CARTESIAN_POINT('Ctrl Pts',(32.1348442130199,34.9683291276834,1.48754049944246));
#27440=CARTESIAN_POINT('Ctrl Pts',(32.1955320114797,34.9682676943423,1.48901580107678));
#27441=CARTESIAN_POINT('Ctrl Pts',(32.2509543450019,34.968215382145,1.49027186778443));
#27442=CARTESIAN_POINT('Ctrl Pts',(32.3021641802425,34.9681701141151,1.491355705848));
#27443=CARTESIAN_POINT('Ctrl Pts',(32.3568725417848,34.968121753488,1.49251358898425));
#27444=CARTESIAN_POINT('Ctrl Pts',(32.4067738547302,34.9680813901957,1.49347579219525));
#27445=CARTESIAN_POINT('Ctrl Pts',(32.4532143425731,34.9680466762593,1.49429647043739));
#27446=CARTESIAN_POINT('Ctrl Pts',(32.5024778890085,34.9680098521065,1.49516703667319));
#27447=CARTESIAN_POINT('Ctrl Pts',(32.5478477692412,34.9679793561973,1.49587895592534));
#27448=CARTESIAN_POINT('Ctrl Pts',(32.590987301899,34.9679531603257,1.49648137333632));
#27449=CARTESIAN_POINT('Ctrl Pts',(32.6362425762296,34.9679256796998,1.49711333579665));
#27450=CARTESIAN_POINT('Ctrl Pts',(32.6790438910131,34.9679029082458,1.49762527612465));
#27451=CARTESIAN_POINT('Ctrl Pts',(32.7213614276251,34.9678837287556,1.49804900699199));
#27452=CARTESIAN_POINT('Ctrl Pts',(32.7633326545624,34.9678647062227,1.49846927021659));
#27453=CARTESIAN_POINT('Ctrl Pts',(32.8048283340688,34.9678491963779,1.49880319667876));
#27454=CARTESIAN_POINT('Ctrl Pts',(32.8478112859608,34.9678375791943,1.49905168880693));
#27455=CARTESIAN_POINT('Ctrl Pts',(32.8880595868429,34.9678267011163,1.49928437142879));
#27456=CARTESIAN_POINT('Ctrl Pts',(32.9296120625591,34.9678192143483,1.49944259954572));
#27457=CARTESIAN_POINT('Ctrl Pts',(32.9741124736802,34.9678170031323,1.49949475964765));
#27458=CARTESIAN_POINT('Ctrl Pts',(32.9824658917578,34.9678165880528,1.49950455090861));
#27459=CARTESIAN_POINT('Ctrl Pts',(32.9909232824608,34.9678163642397,1.49951049395371));
#27460=CARTESIAN_POINT('Ctrl Pts',(32.9994956564548,34.9678163521984,1.49951221389311));
#27461=CARTESIAN_POINT('Ctrl Pts',(33.0359167076011,34.9678163010393,1.49951952132053));
#27462=CARTESIAN_POINT('Ctrl Pts',(33.0737648470632,34.9678163144542,1.49952600456098));
#27463=CARTESIAN_POINT('Ctrl Pts',(33.1138039348095,34.9678165569183,1.49953164904713));
#27464=CARTESIAN_POINT('Ctrl Pts',(33.2457861392316,34.9678173561608,1.49955025515846));
#27465=CARTESIAN_POINT('Ctrl Pts',(33.3718058092169,34.9678177616076,1.49955552940343));
#27466=CARTESIAN_POINT('Ctrl Pts',(33.4990121011461,34.9678181023248,1.49956083536768));
#27467=CARTESIAN_POINT('Ctrl Pts',(33.6624238693916,34.967818540017,1.49956765151637));
#27468=CARTESIAN_POINT('Ctrl Pts',(33.8277938592882,34.9678188708892,1.49957452000977));
#27469=CARTESIAN_POINT('Ctrl Pts',(33.9926457806312,34.9678194856963,1.49958605843696));
#27470=CARTESIAN_POINT('Ctrl Pts',(34.3223496233171,34.9678207153105,1.49960913529135));
#27471=CARTESIAN_POINT('Ctrl Pts',(34.6499811917881,34.9678230806641,1.49965089188094));
#27472=CARTESIAN_POINT('Ctrl Pts',(34.9787437607291,34.9678240597269,1.49966841302101));
#27473=CARTESIAN_POINT('Ctrl Pts',(35.1431250451996,34.9678245492583,1.49967717359104));
#27474=CARTESIAN_POINT('Ctrl Pts',(35.3077890797877,34.967824692217,1.4996798752987));
#27475=CARTESIAN_POINT('Ctrl Pts',(35.4723919953984,34.9678249110676,1.49968390458379));
#27476=CARTESIAN_POINT('Ctrl Pts',(35.9662007422305,34.9678255676193,1.49969599243905));
#27477=CARTESIAN_POINT('Ctrl Pts',(36.459459418267,34.9678269071983,1.49972002849123));
#27478=CARTESIAN_POINT('Ctrl Pts',(36.9527108273738,34.9678287658477,1.49975356610212));
#27479=CARTESIAN_POINT('Ctrl Pts',(38.1015495523822,34.9678330948538,1.49983167901864));
#27480=CARTESIAN_POINT('Ctrl Pts',(39.2503488559568,34.9678402396984,1.49996133572172));
#27481=CARTESIAN_POINT('Ctrl Pts',(40.4000634893725,34.9678419791559,1.49999290859453));
#27482=CARTESIAN_POINT('Ctrl Pts',(6.89999999997365,9.46599415780712,5.65979197164529));
#27483=CARTESIAN_POINT('Ctrl Pts',(6.99168932310453,9.49787619923353,5.60729410195164));
#27484=CARTESIAN_POINT('Ctrl Pts',(7.08405956072215,9.52934434473075,5.55450818731572));
#27485=CARTESIAN_POINT('Ctrl Pts',(8.15473535981985,9.88659437915723,4.94320927931173));
#27486=CARTESIAN_POINT('Ctrl Pts',(9.17052309187647,10.1553288976265,4.34956920012189));
#27487=CARTESIAN_POINT('Ctrl Pts',(11.249912418623,10.5681406908193,3.24757657546859));
#27488=CARTESIAN_POINT('Ctrl Pts',(12.2613271155137,10.7096926815135,2.71507294053767));
#27489=CARTESIAN_POINT('Ctrl Pts',(14.3530613265277,10.9182780492489,1.75089621035865));
#27490=CARTESIAN_POINT('Ctrl Pts',(15.3683896576347,10.9736589531833,1.30024364084097));
#27491=CARTESIAN_POINT('Ctrl Pts',(17.4699484560063,11.0479347559914,0.51160650808575));
#27492=CARTESIAN_POINT('Ctrl Pts',(18.4899441076999,11.0518486975415,0.154966618543408));
#27493=CARTESIAN_POINT('Ctrl Pts',(19.8459385111079,11.0525063200436,-0.227738630131172));
#27494=CARTESIAN_POINT('Ctrl Pts',(20.3436052070642,11.0499443867429,-0.364012293347548));
#27495=CARTESIAN_POINT('Ctrl Pts',(21.3765735172499,11.0391187302377,-0.626365466004486));
#27496=CARTESIAN_POINT('Ctrl Pts',(22.1786513408684,11.0271780970655,-0.80148237085404));
#27497=CARTESIAN_POINT('Ctrl Pts',(22.8524711894103,11.0190184236597,-0.927590054426941));
#27498=CARTESIAN_POINT('Ctrl Pts',(23.1034772575406,11.015636270466,-0.973361071581967));
#27499=CARTESIAN_POINT('Ctrl Pts',(23.6153488598143,11.0082046691873,-1.06157978958535));
#27500=CARTESIAN_POINT('Ctrl Pts',(24.2640912191231,10.9980907558832,-1.16309571993123));
#27501=CARTESIAN_POINT('Ctrl Pts',(24.9252112071703,10.9882975006411,-1.25112898708132));
#27502=CARTESIAN_POINT('Ctrl Pts',(25.3924209938587,10.9823391891697,-1.30426168416562));
#27503=CARTESIAN_POINT('Ctrl Pts',(25.6607104515486,10.9792975977554,-1.332046615497));
#27504=CARTESIAN_POINT('Ctrl Pts',(25.7950739758558,10.9779150347045,-1.34502686686554));
#27505=CARTESIAN_POINT('Ctrl Pts',(26.2512918422651,10.9735046934062,-1.38748529291552));
#27506=CARTESIAN_POINT('Ctrl Pts',(27.3073301682004,10.9653764904263,-1.45732017866833));
#27507=CARTESIAN_POINT('Ctrl Pts',(28.3319194320811,10.9609947024269,-1.48237708919284));
#27508=CARTESIAN_POINT('Ctrl Pts',(29.1280123944214,10.9582092660149,-1.50394716937725));
#27509=CARTESIAN_POINT('Ctrl Pts',(29.4779818455993,10.9573324846489,-1.51103964894258));
#27510=CARTESIAN_POINT('Ctrl Pts',(29.9466600480359,10.9567800220405,-1.51533483257754));
#27511=CARTESIAN_POINT('Ctrl Pts',(30.4585980273686,10.956656708735,-1.51632751174059));
#27512=CARTESIAN_POINT('Ctrl Pts',(31.4732549878281,10.9572594965941,-1.51158385370563));
#27513=CARTESIAN_POINT('Ctrl Pts',(32.3455845021632,10.95879335959,-1.4999511927851));
#27514=CARTESIAN_POINT('Ctrl Pts',(33.1628510802405,10.9587933798862,-1.49997453311311));
#27515=CARTESIAN_POINT('Ctrl Pts',(33.4532441810442,10.9587933789851,-1.49997366471359));
#27516=CARTESIAN_POINT('Ctrl Pts',(33.7813843869345,10.9587933812939,-1.49997637381128));
#27517=CARTESIAN_POINT('Ctrl Pts',(34.2755379701535,10.9587933817727,-1.49997699476315));
#27518=CARTESIAN_POINT('Ctrl Pts',(34.8102302793009,10.9587933869434,-1.49998326277599));
#27519=CARTESIAN_POINT('Ctrl Pts',(35.6332452367756,10.9587933876415,-1.49998412101817));
#27520=CARTESIAN_POINT('Ctrl Pts',(36.2915450349079,10.9587933890033,-1.49998577371297));
#27521=CARTESIAN_POINT('Ctrl Pts',(38.1020137670942,10.9587933908629,-1.49998803993575));
#27522=CARTESIAN_POINT('Ctrl Pts',(39.5833333333333,10.9587934006931,-1.5));
#27523=CARTESIAN_POINT('Ctrl Pts',(40.9,10.9587934006931,-1.5));
#27524=CARTESIAN_POINT('Ctrl Pts',(6.65963435785827,13.0027682689653,8.56288377493212));
#27525=CARTESIAN_POINT('Ctrl Pts',(6.7513219377677,13.050957789036,8.49067817166156));
#27526=CARTESIAN_POINT('Ctrl Pts',(6.84370278928156,13.0985893115687,8.41801298642698));
#27527=CARTESIAN_POINT('Ctrl Pts',(7.91483960325934,13.6397807532085,7.57680655910808));
#27528=CARTESIAN_POINT('Ctrl Pts',(8.9325509112231,14.0543934435321,6.75518385076231));
#27529=CARTESIAN_POINT('Ctrl Pts',(11.0192135814157,14.7040310435558,5.22065437877307));
#27530=CARTESIAN_POINT('Ctrl Pts',(12.0340542508324,14.9356992206141,4.4769598695545));
#27531=CARTESIAN_POINT('Ctrl Pts',(14.1407660172285,15.2883456800052,3.1214593369057));
#27532=CARTESIAN_POINT('Ctrl Pts',(15.1616568764318,15.3931503655329,2.48732138966201));
#27533=CARTESIAN_POINT('Ctrl Pts',(17.287218760307,15.5446125872455,1.36959877283814));
#27534=CARTESIAN_POINT('Ctrl Pts',(18.3145546794907,15.5707395254148,0.864902786641511));
#27535=CARTESIAN_POINT('Ctrl Pts',(19.6926214867647,15.5935126543779,0.318801403605146));
#27536=CARTESIAN_POINT('Ctrl Pts',(20.1945263626901,15.5977145841048,0.125373946234778));
#27537=CARTESIAN_POINT('Ctrl Pts',(21.2420076978203,15.5972978704292,-0.248868189963681));
#27538=CARTESIAN_POINT('Ctrl Pts',(22.0575126096201,15.5901933457539,-0.499284562147392));
#27539=CARTESIAN_POINT('Ctrl Pts',(22.7441078663834,15.5856475377419,-0.679992377552244));
#27540=CARTESIAN_POINT('Ctrl Pts',(22.9980856324395,15.5834353094767,-0.745267685418833));
#27541=CARTESIAN_POINT('Ctrl Pts',(23.5177883906687,15.5778337615218,-0.871419538176181));
#27542=CARTESIAN_POINT('Ctrl Pts',(24.1766640555165,15.569151455817,-1.01665680544524));
#27543=CARTESIAN_POINT('Ctrl Pts',(24.8496697365589,15.560128822227,-1.14287321247013));
#27544=CARTESIAN_POINT('Ctrl Pts',(25.3259254544069,15.554601684436,-1.2191404135396));
#27545=CARTESIAN_POINT('Ctrl Pts',(25.5996882691236,15.5518109321211,-1.2590574298324));
#27546=CARTESIAN_POINT('Ctrl Pts',(25.7368188560809,15.550561003587,-1.27770917936971));
#27547=CARTESIAN_POINT('Ctrl Pts',(26.2030586507879,15.5466206431081,-1.33878235986071));
#27548=CARTESIAN_POINT('Ctrl Pts',(27.2845562696213,15.5388831179539,-1.43928616936987));
#27549=CARTESIAN_POINT('Ctrl Pts',(28.3146233763975,15.534108117874,-1.47473229777557));
#27550=CARTESIAN_POINT('Ctrl Pts',(29.1121433593266,15.5313810124223,-1.5053783917148));
#27551=CARTESIAN_POINT('Ctrl Pts',(29.4693616319656,15.5305221749293,-1.51558516408219));
#27552=CARTESIAN_POINT('Ctrl Pts',(29.9425518103672,15.5299808253862,-1.52169686437909));
#27553=CARTESIAN_POINT('Ctrl Pts',(30.4595136734855,15.5298599056894,-1.52312339822457));
#27554=CARTESIAN_POINT('Ctrl Pts',(31.4800666545032,15.5304501241615,-1.51634797661239));
#27555=CARTESIAN_POINT('Ctrl Pts',(32.3507119180564,15.5319509809364,-1.4999128955352));
#27556=CARTESIAN_POINT('Ctrl Pts',(33.1621363777215,15.5319505779396,-1.49995461572564));
#27557=CARTESIAN_POINT('Ctrl Pts',(33.4535196029878,15.5319505880019,-1.49995304854269));
#27558=CARTESIAN_POINT('Ctrl Pts',(33.7812306484551,15.5319505396377,-1.49995788616631));
#27559=CARTESIAN_POINT('Ctrl Pts',(34.2755524327802,15.531950526851,-1.49995898984267));
#27560=CARTESIAN_POINT('Ctrl Pts',(34.8101578274898,15.5319504091692,-1.49997016508529));
#27561=CARTESIAN_POINT('Ctrl Pts',(35.6332135248365,15.5319503927198,-1.49997169422773));
#27562=CARTESIAN_POINT('Ctrl Pts',(36.2914988048216,15.5319503616369,-1.49997464065555));
#27563=CARTESIAN_POINT('Ctrl Pts',(38.1019885414694,15.5319503187541,-1.49997868009126));
#27564=CARTESIAN_POINT('Ctrl Pts',(39.5833333333333,15.5319500929849,-1.5));
#27565=CARTESIAN_POINT('Ctrl Pts',(40.9,15.5319500929849,-1.5));
#27566=CARTESIAN_POINT('Ctrl Pts',(6.47503677058814,19.2049631177014,13.6264850125633));
#27567=CARTESIAN_POINT('Ctrl Pts',(6.56582707216344,19.2807931407427,13.5206117629928));
#27568=CARTESIAN_POINT('Ctrl Pts',(6.65722187862393,19.3557456396964,13.4141026801341));
#27569=CARTESIAN_POINT('Ctrl Pts',(7.71979853459931,20.2113974185276,12.1774082172639));
#27570=CARTESIAN_POINT('Ctrl Pts',(8.72714740265586,20.876585861408,10.9649265084515));
#27571=CARTESIAN_POINT('Ctrl Pts',(10.792252425961,21.9312131301472,8.69413764846818));
#27572=CARTESIAN_POINT('Ctrl Pts',(11.8008983729842,22.3203974544121,7.58577239973431));
#27573=CARTESIAN_POINT('Ctrl Pts',(13.892634394048,22.9231109701401,5.56042793834188));
#27574=CARTESIAN_POINT('Ctrl Pts',(14.910936596525,23.1162450123325,4.60683703173286));
#27575=CARTESIAN_POINT('Ctrl Pts',(17.0374816014601,23.4053158267904,2.91606182242837));
#27576=CARTESIAN_POINT('Ctrl Pts',(18.0678529336714,23.4724397837998,2.15006970557796));
#27577=CARTESIAN_POINT('Ctrl Pts',(19.4632774216583,23.5361137002685,1.31129970902877));
#27578=CARTESIAN_POINT('Ctrl Pts',(19.9690853949367,23.5527456051548,1.01646669656859));
#27579=CARTESIAN_POINT('Ctrl Pts',(21.0306109698709,23.5717577824589,0.441678056412672));
#27580=CARTESIAN_POINT('Ctrl Pts',(21.8626014988188,23.5739085372705,0.0543003442681426));
#27581=CARTESIAN_POINT('Ctrl Pts',(22.5665651705189,23.5761789143631,-0.226484889079843));
#27582=CARTESIAN_POINT('Ctrl Pts',(22.8246411038756,23.5761448043361,-0.326902916553465));
#27583=CARTESIAN_POINT('Ctrl Pts',(23.3554232774669,23.5740054132278,-0.522054743089693));
#27584=CARTESIAN_POINT('Ctrl Pts',(24.0293769285439,23.5680817805141,-0.747005858788648));
#27585=CARTESIAN_POINT('Ctrl Pts',(24.7209631427047,23.560586503548,-0.94339358139433));
#27586=CARTESIAN_POINT('Ctrl Pts',(25.2118242719342,23.5558940963915,-1.06233480615607));
#27587=CARTESIAN_POINT('Ctrl Pts',(25.4945546545947,23.5535795021665,-1.12470144437592));
#27588=CARTESIAN_POINT('Ctrl Pts',(25.6362544160062,23.5525764277764,-1.15385183559377));
#27589=CARTESIAN_POINT('Ctrl Pts',(26.1191683853685,23.5495095529483,-1.24953281052836));
#27590=CARTESIAN_POINT('Ctrl Pts',(27.244410780189,23.5425023713064,-1.40715534997208));
#27591=CARTESIAN_POINT('Ctrl Pts',(28.2843056152442,23.5370396227258,-1.46065929315376));
#27592=CARTESIAN_POINT('Ctrl Pts',(29.0843244121809,23.5344215873996,-1.50737208683505));
#27593=CARTESIAN_POINT('Ctrl Pts',(29.4542021761287,23.5335942286398,-1.52336782189617));
#27594=CARTESIAN_POINT('Ctrl Pts',(29.9352997409898,23.5330734925559,-1.53271512054377));
#27595=CARTESIAN_POINT('Ctrl Pts',(30.4610555884278,23.532957187389,-1.5349453613852));
#27596=CARTESIAN_POINT('Ctrl Pts',(31.4919316519535,23.5335262680548,-1.52450364515754));
#27597=CARTESIAN_POINT('Ctrl Pts',(32.3596576160514,23.5349731541844,-1.49979324124413));
#27598=CARTESIAN_POINT('Ctrl Pts',(33.1608710165812,23.5349736853906,-1.49989213988255));
#27599=CARTESIAN_POINT('Ctrl Pts',(33.4539865796869,23.5349736699323,-1.49988845489238));
#27600=CARTESIAN_POINT('Ctrl Pts',(33.780948091659,23.5349737329761,-1.49989993226727));
#27601=CARTESIAN_POINT('Ctrl Pts',(34.275564602361,23.5349737489117,-1.49990256114204));
#27602=CARTESIAN_POINT('Ctrl Pts',(34.810021467207,23.5349738998239,-1.49992910993535));
#27603=CARTESIAN_POINT('Ctrl Pts',(35.6331489543767,23.5349739207807,-1.49993274473985));
#27604=CARTESIAN_POINT('Ctrl Pts',(36.2914097700016,23.5349739606187,-1.4999397448351));
#27605=CARTESIAN_POINT('Ctrl Pts',(38.1019375614968,23.5349740154737,-1.49994934328327));
#27606=CARTESIAN_POINT('Ctrl Pts',(39.5833333333333,23.5349743044955,-1.5));
#27607=CARTESIAN_POINT('Ctrl Pts',(40.9,23.5349743044955,-1.5));
#27608=CARTESIAN_POINT('Ctrl Pts',(6.39840282685635,25.4797798158266,18.5950148818));
#27609=CARTESIAN_POINT('Ctrl Pts',(6.48879582230594,25.5825069307027,18.455456538043));
#27610=CARTESIAN_POINT('Ctrl Pts',(6.57973810483189,25.684006582131,18.3151558806717));
#27611=CARTESIAN_POINT('Ctrl Pts',(7.63881202209714,26.8457843562122,16.6821095714367));
#27612=CARTESIAN_POINT('Ctrl Pts',(8.64206536867565,27.7524045864227,15.0805562774161));
#27613=CARTESIAN_POINT('Ctrl Pts',(10.6943835463645,29.194220471563,12.08639394536));
#27614=CARTESIAN_POINT('Ctrl Pts',(11.6986850371144,29.7340826089764,10.6188960618635));
#27615=CARTESIAN_POINT('Ctrl Pts',(13.7736723466472,30.5724457120527,7.9480571508383));
#27616=CARTESIAN_POINT('Ctrl Pts',(14.7865355152845,30.8496813329458,6.68379951334874));
#27617=CARTESIAN_POINT('Ctrl Pts',(16.895644387614,31.2681094727719,4.44867953439714));
#27618=CARTESIAN_POINT('Ctrl Pts',(17.921113585793,31.3748718553479,3.42955614780409));
#27619=CARTESIAN_POINT('Ctrl Pts',(19.3111115725317,31.4778602005301,2.31180057560694));
#27620=CARTESIAN_POINT('Ctrl Pts',(19.8164097330209,31.5068304778962,1.91755167896536));
#27621=CARTESIAN_POINT('Ctrl Pts',(20.8772665291465,31.5450009606978,1.14804732053491));
#27622=CARTESIAN_POINT('Ctrl Pts',(21.7126526899651,31.5565752055434,0.625757760628938));
#27623=CARTESIAN_POINT('Ctrl Pts',(22.4233939916368,31.5658469864011,0.244774266221906));
#27624=CARTESIAN_POINT('Ctrl Pts',(22.68321700305,31.568070163829,0.109074102068986));
#27625=CARTESIAN_POINT('Ctrl Pts',(23.2191843843282,31.5695528321153,-0.155714853804433));
#27626=CARTESIAN_POINT('Ctrl Pts',(23.9014490792895,31.5665856540486,-0.461901703286707));
#27627=CARTESIAN_POINT('Ctrl Pts',(24.6052033552109,31.5607844376464,-0.730987709817266));
#27628=CARTESIAN_POINT('Ctrl Pts',(25.1069219885717,31.5570192016244,-0.89479518126793));
#27629=CARTESIAN_POINT('Ctrl Pts',(25.3966703145091,31.5552253028176,-0.980957842597307));
#27630=CARTESIAN_POINT('Ctrl Pts',(25.5420691491796,31.5544886793522,-1.02128571697646));
#27631=CARTESIAN_POINT('Ctrl Pts',(26.0386675456483,31.5523567719375,-1.15405115562806));
#27632=CARTESIAN_POINT('Ctrl Pts',(27.2041996425261,31.5461367082151,-1.37405103438868));
#27633=CARTESIAN_POINT('Ctrl Pts',(28.254481539011,31.5399727189289,-1.44553527377015));
#27634=CARTESIAN_POINT('Ctrl Pts',(29.0567817440806,31.5374655658645,-1.50856328668891));
#27635=CARTESIAN_POINT('Ctrl Pts',(29.4392037716731,31.5366692491296,-1.53093305020556));
#27636=CARTESIAN_POINT('Ctrl Pts',(29.9281985709061,31.536168682902,-1.54360558359609));
#27637=CARTESIAN_POINT('Ctrl Pts',(30.4627354290944,31.5360567738141,-1.54671304059522));
#27638=CARTESIAN_POINT('Ctrl Pts',(31.5039222132187,31.5366047697957,-1.53240580330097));
#27639=CARTESIAN_POINT('Ctrl Pts',(32.3686614831274,31.5379963364647,-1.49961223537188));
#27640=CARTESIAN_POINT('Ctrl Pts',(33.1596379899179,31.5379973429874,-1.49979803313558));
#27641=CARTESIAN_POINT('Ctrl Pts',(33.4544864001145,31.5379973136915,-1.49979103760183));
#27642=CARTESIAN_POINT('Ctrl Pts',(33.7806952343975,31.5379974331442,-1.49981257637976));
#27643=CARTESIAN_POINT('Ctrl Pts',(34.2756055948936,31.5379974633363,-1.49981748473541));
#27644=CARTESIAN_POINT('Ctrl Pts',(34.8099061252942,31.5379977492716,-1.49986722177693));
#27645=CARTESIAN_POINT('Ctrl Pts',(35.6331043028646,31.5379977889784,-1.49987402634112));
#27646=CARTESIAN_POINT('Ctrl Pts',(36.2913385913736,31.5379978644599,-1.49988713966987));
#27647=CARTESIAN_POINT('Ctrl Pts',(38.1019015852784,31.537997968394,-1.49990511666357));
#27648=CARTESIAN_POINT('Ctrl Pts',(39.5833333333333,31.5379985160061,-1.5));
#27649=CARTESIAN_POINT('Ctrl Pts',(40.9,31.5379985160061,-1.5));
#27650=CARTESIAN_POINT('Ctrl Pts',(6.37427268165564,28.1741189428499,20.7176664141567));
#27651=CARTESIAN_POINT('Ctrl Pts',(6.46448755772838,28.2883460540946,20.5636424771022));
#27652=CARTESIAN_POINT('Ctrl Pts',(6.55522687426754,28.4011972468989,20.4088293925213));
#27653=CARTESIAN_POINT('Ctrl Pts',(7.61282240204204,29.693787896276,18.6056139772311));
#27654=CARTESIAN_POINT('Ctrl Pts',(8.61454082730176,30.703424507615,16.8370699794085));
#27655=CARTESIAN_POINT('Ctrl Pts',(10.6618274824665,32.3104201819496,13.5325068155167));
#27656=CARTESIAN_POINT('Ctrl Pts',(11.6645377987076,32.9144254040795,11.9110180488694));
#27657=CARTESIAN_POINT('Ctrl Pts',(13.7331445959134,33.8529424117878,8.96386257277559));
#27658=CARTESIAN_POINT('Ctrl Pts',(14.7439932704909,34.1658004948675,7.56674532731095));
#27659=CARTESIAN_POINT('Ctrl Pts',(16.8461035490385,34.6388264066738,5.10012840374637));
#27660=CARTESIAN_POINT('Ctrl Pts',(17.8695058124616,34.7622645166785,3.97333364734334));
#27661=CARTESIAN_POINT('Ctrl Pts',(19.2561174443541,34.8817349492475,2.73821070416469));
#27662=CARTESIAN_POINT('Ctrl Pts',(19.7609345646798,34.9159214541564,2.30176586395499));
#27663=CARTESIAN_POINT('Ctrl Pts',(20.8205141053453,34.9621410370326,1.45015687002429));
#27664=CARTESIAN_POINT('Ctrl Pts',(21.6560023791939,34.9776907709078,0.871078443387));
#27665=CARTESIAN_POINT('Ctrl Pts',(22.3682688599883,34.989939594886,0.44777828592714));
#27666=CARTESIAN_POINT('Ctrl Pts',(22.6285200842947,34.9931281975259,0.297086276283266));
#27667=CARTESIAN_POINT('Ctrl Pts',(23.1658603614091,34.9961605697035,0.00273379297028335));
#27668=CARTESIAN_POINT('Ctrl Pts',(23.8505975407037,34.9944676948756,-0.338068372298848));
#27669=CARTESIAN_POINT('Ctrl Pts',(24.5583968797874,34.9894056975888,-0.638319272935672));
#27670=CARTESIAN_POINT('Ctrl Pts',(25.0640148551739,34.9860476379143,-0.821498314632837));
#27671=CARTESIAN_POINT('Ctrl Pts',(25.3563632502514,34.9844821378475,-0.917977493583088));
#27672=CARTESIAN_POINT('Ctrl Pts',(25.503160007456,34.9838621425449,-0.963163948801062));
#27673=CARTESIAN_POINT('Ctrl Pts',(26.0049713545738,34.982139121313,-1.11209382847183));
#27674=CARTESIAN_POINT('Ctrl Pts',(27.1869304722337,34.9762666166019,-1.35965020681435));
#27675=CARTESIAN_POINT('Ctrl Pts',(28.2418054197051,34.9698003983093,-1.43886806122646));
#27676=CARTESIAN_POINT('Ctrl Pts',(29.0450356043991,34.9673414359535,-1.50892754055989));
#27677=CARTESIAN_POINT('Ctrl Pts',(29.4328041419752,34.9665583691038,-1.53413528152412));
#27678=CARTESIAN_POINT('Ctrl Pts',(29.9251825362975,34.9660664512209,-1.54824951859995));
#27679=CARTESIAN_POINT('Ctrl Pts',(30.4634799414205,34.9659564211645,-1.55174636239756));
#27680=CARTESIAN_POINT('Ctrl Pts',(31.5090833787051,34.9664954410524,-1.53574598606795));
#27681=CARTESIAN_POINT('Ctrl Pts',(32.3725304400172,34.9678633362529,-1.49952340891733));
#27682=CARTESIAN_POINT('Ctrl Pts',(33.1591152593399,34.9678645826042,-1.49975189997365));
#27683=CARTESIAN_POINT('Ctrl Pts',(33.4547063903441,34.9678645463389,-1.49974326694615));
#27684=CARTESIAN_POINT('Ctrl Pts',(33.7805921021893,34.9678646942577,-1.49976974530861));
#27685=CARTESIAN_POINT('Ctrl Pts',(34.2756282408745,34.9678647316484,-1.49977576894615));
#27686=CARTESIAN_POINT('Ctrl Pts',(34.8098603973427,34.967865085736,-1.49983687714898));
#27687=CARTESIAN_POINT('Ctrl Pts',(35.6330886763766,34.9678651349076,-1.49984523535833));
#27688=CARTESIAN_POINT('Ctrl Pts',(36.2913112329655,34.9678652283802,-1.49986134640235));
#27689=CARTESIAN_POINT('Ctrl Pts',(38.1018888107018,34.9678653570876,-1.49988343135295));
#27690=CARTESIAN_POINT('Ctrl Pts',(39.5833333333333,34.9678660352249,-1.5));
#27691=CARTESIAN_POINT('Ctrl Pts',(40.9,34.9678660352249,-1.5));
#27692=CARTESIAN_POINT('',(40.9,32.9658914637539,-1.50000000000001));
#27693=CARTESIAN_POINT('Ctrl Pts',(40.9,32.9658914637539,-1.50000000000001));
#27694=CARTESIAN_POINT('Ctrl Pts',(40.9,33.466386268912,-1.50000000000001));
#27695=CARTESIAN_POINT('Ctrl Pts',(40.9,33.9668810740701,-1.50000000000001));
#27696=CARTESIAN_POINT('Ctrl Pts',(40.9,34.4673758792282,-1.50000000000001));
#27697=CARTESIAN_POINT('',(38.,32.9658914637539,-1.5));
#27698=CARTESIAN_POINT('Ctrl Pts',(38.,32.9658914637539,-1.5));
#27699=CARTESIAN_POINT('Ctrl Pts',(38.9666666666667,32.9658914637539,-1.5));
#27700=CARTESIAN_POINT('Ctrl Pts',(39.9333333333333,32.9658914637539,-1.5));
#27701=CARTESIAN_POINT('Ctrl Pts',(40.9,32.9658914637539,-1.5));
#27702=CARTESIAN_POINT('',(37.5,32.3652591523689,-1.49999999999999));
#27703=CARTESIAN_POINT('Ctrl Pts',(37.4997714574611,32.3652585803353,-1.49990106437152));
#27704=CARTESIAN_POINT('Ctrl Pts',(37.6667294826964,32.5658056765353,-1.4999047077905));
#27705=CARTESIAN_POINT('Ctrl Pts',(37.8334450600884,32.7660568372679,-1.49990923999261));
#27706=CARTESIAN_POINT('Ctrl Pts',(37.9998166694663,32.9658909678229,-1.49991439209149));
#27707=CARTESIAN_POINT('Ctrl Pts',(20.644698628669,15.8947820241755,4.30211422042248E-15));
#27708=CARTESIAN_POINT('Ctrl Pts',(21.3839825863869,16.36544922962,-0.225731928831263));
#27709=CARTESIAN_POINT('Ctrl Pts',(22.0257484868013,16.806097479622,-0.406661554463689));
#27710=CARTESIAN_POINT('Ctrl Pts',(22.5801728644232,17.2054177529787,-0.547761868179738));
#27711=CARTESIAN_POINT('Ctrl Pts',(23.3331120273116,17.7477169095115,-0.739383947548498));
#27712=CARTESIAN_POINT('Ctrl Pts',(23.9218122708631,18.2069240887503,-0.875125428914569));
#27713=CARTESIAN_POINT('Ctrl Pts',(24.4823254534451,18.6644103290309,-0.991025114746261));
#27714=CARTESIAN_POINT('Ctrl Pts',(24.9418997081724,19.0395110482618,-1.0860532307557));
#27715=CARTESIAN_POINT('Ctrl Pts',(25.3626371148051,19.3999354975894,-1.16248640886278));
#27716=CARTESIAN_POINT('Ctrl Pts',(25.7525302890143,19.7463071016619,-1.22321331868058));
#27717=CARTESIAN_POINT('Ctrl Pts',(26.1776080056329,20.123935796648,-1.28942031554581));
#27718=CARTESIAN_POINT('Ctrl Pts',(26.5661459571655,20.485239616978,-1.3329732143938));
#27719=CARTESIAN_POINT('Ctrl Pts',(26.9267016831473,20.8313979297641,-1.36638815233963));
#27720=CARTESIAN_POINT('Ctrl Pts',(27.1778777842812,21.0725442744629,-1.38966620127371));
#27721=CARTESIAN_POINT('Ctrl Pts',(27.415486111974,21.306416246323,-1.40780557011307));
#27722=CARTESIAN_POINT('Ctrl Pts',(27.6422281942519,21.533988872658,-1.42326116565051));
#27723=CARTESIAN_POINT('Ctrl Pts',(27.8555559933386,21.7480980800036,-1.43780239305062));
#27724=CARTESIAN_POINT('Ctrl Pts',(28.1190837193165,22.0160369614212,-1.45368682614543));
#27725=CARTESIAN_POINT('Ctrl Pts',(28.4603051775928,22.3749799381825,-1.47251023690728));
#27726=CARTESIAN_POINT('Ctrl Pts',(28.6017730832564,22.5237950550031,-1.48031428449378));
#27727=CARTESIAN_POINT('Ctrl Pts',(28.7540286646466,22.6856884569089,-1.48853267939435));
#27728=CARTESIAN_POINT('Ctrl Pts',(28.9157341130969,22.8599017516109,-1.49763121638955));
#27729=CARTESIAN_POINT('Ctrl Pts',(29.4787137469343,23.4664276157722,-1.52930789194508));
#27730=CARTESIAN_POINT('Ctrl Pts',(30.1711677436424,24.2477248210898,-1.53976925233531));
#27731=CARTESIAN_POINT('Ctrl Pts',(30.8055547543771,24.9885333989172,-1.53340754825751));
#27732=CARTESIAN_POINT('Ctrl Pts',(31.1893125644442,25.4366684847488,-1.52955918190719));
#27733=CARTESIAN_POINT('Ctrl Pts',(31.5650207099053,25.8828713567937,-1.52122455967934));
#27734=CARTESIAN_POINT('Ctrl Pts',(31.9311744366546,26.3192346641773,-1.51382648741803));
#27735=CARTESIAN_POINT('Ctrl Pts',(32.1142513000292,26.5374163178691,-1.51012745128737));
#27736=CARTESIAN_POINT('Ctrl Pts',(32.2949430642633,26.7531357746899,-1.50666813405654));
#27737=CARTESIAN_POINT('Ctrl Pts',(32.4730466959744,26.9654180603387,-1.50413682057756));
#27738=CARTESIAN_POINT('Ctrl Pts',(32.5932788659896,27.108723166552,-1.50242801032117));
#27739=CARTESIAN_POINT('Ctrl Pts',(32.7123311761215,27.2504621964592,-1.50114220273815));
#27740=CARTESIAN_POINT('Ctrl Pts',(32.8301302693916,27.3903440145187,-1.50048655910759));
#27741=CARTESIAN_POINT('Ctrl Pts',(32.8868306160054,27.457673459498,-1.50017097755194));
#27742=CARTESIAN_POINT('Ctrl Pts',(32.9387123022831,27.5192120661962,-1.5));
#27743=CARTESIAN_POINT('Ctrl Pts',(33.,27.5917792275077,-1.5));
#27744=CARTESIAN_POINT('Ctrl Pts',(33.0955022515694,27.704857831427,-1.5));
#27745=CARTESIAN_POINT('Ctrl Pts',(33.2417478452381,27.8775886864723,-1.5));
#27746=CARTESIAN_POINT('Ctrl Pts',(33.3688392457043,28.0268611297194,-1.5));
#27747=CARTESIAN_POINT('Ctrl Pts',(34.266193218837,29.0808287430714,-1.5));
#27748=CARTESIAN_POINT('Ctrl Pts',(35.2319960543079,30.1809662912372,-1.49999999999999));
#27749=CARTESIAN_POINT('Ctrl Pts',(36.3004607333105,31.2401426718444,-1.49999999999999));
#27750=CARTESIAN_POINT('Ctrl Pts',(36.6891719086848,31.6254747318792,-1.49999999999999));
#27751=CARTESIAN_POINT('Ctrl Pts',(37.0893059758979,32.0028866146556,-1.49999999999999));
#27752=CARTESIAN_POINT('Ctrl Pts',(37.5,32.3652591523689,-1.49999999999999));
#27753=CARTESIAN_POINT('',(6.9,24.7737885487526,16.9192021366758));
#27754=CARTESIAN_POINT('Ctrl Pts',(6.9,24.7737885487526,16.9192021366758));
#27755=CARTESIAN_POINT('Ctrl Pts',(6.9,22.6454446228759,15.3881766950258));
#27756=CARTESIAN_POINT('Ctrl Pts',(6.90000000000115,20.4978726403359,13.8353835251886));
#27757=CARTESIAN_POINT('Ctrl Pts',(6.90000000000115,15.662481608859,10.3082122779765));
#27758=CARTESIAN_POINT('Ctrl Pts',(6.9,12.4764228571341,7.95935811114668));
#27759=CARTESIAN_POINT('Ctrl Pts',(6.9,9.46599415782504,5.6597919716369));
#27760=CARTESIAN_POINT('',(22.9245129145126,31.7706052331164,0.));
#27761=CARTESIAN_POINT('Ctrl Pts',(22.9245129145126,31.7706052331164,-4.30711063480545E-15));
#27762=CARTESIAN_POINT('Ctrl Pts',(22.7202811020963,31.7014549124251,0.0979233563002647));
#27763=CARTESIAN_POINT('Ctrl Pts',(22.5089075447093,31.6320805544326,0.203440182623873));
#27764=CARTESIAN_POINT('Ctrl Pts',(22.2913349439917,31.5632247707622,0.316637134194167));
#27765=CARTESIAN_POINT('Ctrl Pts',(21.4451770585291,31.2954389184983,0.756869465221241));
#27766=CARTESIAN_POINT('Ctrl Pts',(20.5220951556665,31.047510614715,1.35418571023244));
#27767=CARTESIAN_POINT('Ctrl Pts',(19.7671428819535,30.8612920963157,1.89915402350731));
#27768=CARTESIAN_POINT('Ctrl Pts',(19.5194773058389,30.8002022522971,2.0779333927085));
#27769=CARTESIAN_POINT('Ctrl Pts',(19.286571638609,30.7444068279677,2.25204835959331));
#27770=CARTESIAN_POINT('Ctrl Pts',(19.0728538401323,30.6939488833522,2.41532203906683));
#27771=CARTESIAN_POINT('Ctrl Pts',(18.7028555998035,30.6065937315988,2.69798906318813));
#27772=CARTESIAN_POINT('Ctrl Pts',(18.4144703596235,30.539966063932,2.93373938287718));
#27773=CARTESIAN_POINT('Ctrl Pts',(18.0642874871537,30.4582462938821,3.23398234069995));
#27774=CARTESIAN_POINT('Ctrl Pts',(17.4420927116721,30.3130489756353,3.76744532366923));
#27775=CARTESIAN_POINT('Ctrl Pts',(16.7224564418218,30.1446863488622,4.43872907330234));
#27776=CARTESIAN_POINT('Ctrl Pts',(15.9202806616111,29.9321297384067,5.24401550821529));
#27777=CARTESIAN_POINT('Ctrl Pts',(15.4090529834515,29.7966671314303,5.75722561070153));
#27778=CARTESIAN_POINT('Ctrl Pts',(14.8739602945708,29.6418940055913,6.33424649579734));
#27779=CARTESIAN_POINT('Ctrl Pts',(14.3169794331144,29.4557634846119,6.96996102647337));
#27780=CARTESIAN_POINT('Ctrl Pts',(13.8864206762829,29.3118803976566,7.46138268378477));
#27781=CARTESIAN_POINT('Ctrl Pts',(13.3867890027799,29.1311705407937,8.05270459512057));
#27782=CARTESIAN_POINT('Ctrl Pts',(12.8146824059514,28.8915984033895,8.75043091662868));
#27783=CARTESIAN_POINT('Ctrl Pts',(12.2526665517595,28.6562518085588,9.4358508309389));
#27784=CARTESIAN_POINT('Ctrl Pts',(11.6379478462804,28.3625845909803,10.231366276768));
#27785=CARTESIAN_POINT('Ctrl Pts',(10.9739250490309,27.981021293096,11.1267230319105));
#27786=CARTESIAN_POINT('Ctrl Pts',(10.5683455447964,27.747965660321,11.6735993596027));
#27787=CARTESIAN_POINT('Ctrl Pts',(10.1437415406956,27.4801235315866,12.2581093618546));
#27788=CARTESIAN_POINT('Ctrl Pts',(9.74137929176525,27.2046666925187,12.8142541611144));
#27789=CARTESIAN_POINT('Ctrl Pts',(8.72285779294234,26.5073877769786,14.2220538143138));
#27790=CARTESIAN_POINT('Ctrl Pts',(7.81323138778195,25.7100913255874,15.580948814124));
#27791=CARTESIAN_POINT('Ctrl Pts',(6.9,24.7737885487526,16.9192021366758));
#27792=CARTESIAN_POINT('Ctrl Pts',(30.5,34.9656486014478,-1.55029606206997));
#27793=CARTESIAN_POINT('Ctrl Pts',(29.9560179420817,34.7222276068062,-1.55343104498103));
#27794=CARTESIAN_POINT('Ctrl Pts',(29.4152668325132,34.4790656554127,-1.54030953139106));
#27795=CARTESIAN_POINT('Ctrl Pts',(28.8740459957565,34.2361296888632,-1.49470250846617));
#27796=CARTESIAN_POINT('Ctrl Pts',(28.3535277923439,34.0024864433252,-1.4508400330705));
#27797=CARTESIAN_POINT('Ctrl Pts',(27.8179515912466,33.7608540997398,-1.40923473841146));
#27798=CARTESIAN_POINT('Ctrl Pts',(27.2695051149491,33.5168388499063,-1.33972398862116));
#27799=CARTESIAN_POINT('Ctrl Pts',(26.9554553615883,33.3771115796287,-1.29992095446742));
#27800=CARTESIAN_POINT('Ctrl Pts',(26.6378099296971,33.2369493090937,-1.25106463707208));
#27801=CARTESIAN_POINT('Ctrl Pts',(26.3179304017917,33.0983258448229,-1.18777049128279));
#27802=CARTESIAN_POINT('Ctrl Pts',(26.1078196745982,33.0072719500184,-1.14619615520081));
#27803=CARTESIAN_POINT('Ctrl Pts',(25.8967402232745,32.9168907470981,-1.09839525532296));
#27804=CARTESIAN_POINT('Ctrl Pts',(25.6850706236774,32.8277596053404,-1.04282885388104));
#27805=CARTESIAN_POINT('Ctrl Pts',(25.6562210027417,32.8156114288513,-1.03525540156946));
#27806=CARTESIAN_POINT('Ctrl Pts',(25.6277737638215,32.8036595933923,-1.02765061224339));
#27807=CARTESIAN_POINT('Ctrl Pts',(25.5983858063598,32.7913423709803,-1.01964325944536));
#27808=CARTESIAN_POINT('Ctrl Pts',(25.1249357452756,32.5929076988546,-0.890642063078171));
#27809=CARTESIAN_POINT('Ctrl Pts',(24.1510084067019,32.1858811669087,-0.588069770626602));
#27810=CARTESIAN_POINT('Ctrl Pts',(22.9245129145126,31.7706052331164,-4.30711063480545E-15));
#27811=CARTESIAN_POINT('Origin',(40.65,0.,0.));
#27812=CARTESIAN_POINT('',(40.4,29.5330398077868,18.7829592905825));
#27813=CARTESIAN_POINT('',(40.9,29.0996231131986,18.5327260452907));
#27814=CARTESIAN_POINT('Ctrl Pts',(40.4,29.5330398077868,18.7829592905825));
#27815=CARTESIAN_POINT('Ctrl Pts',(40.5666590139515,29.3885761362401,18.6995531509269));
#27816=CARTESIAN_POINT('Ctrl Pts',(40.7333430451841,29.2440888804717,18.6161333949145));
#27817=CARTESIAN_POINT('Ctrl Pts',(40.9,29.0996231131986,18.5327260452907));
#27818=CARTESIAN_POINT('',(40.9,30.5996231131986,15.9346498339374));
#27819=CARTESIAN_POINT('Origin',(40.9,0.,0.));
#27820=CARTESIAN_POINT('',(40.4,31.0330398077868,16.1848830792292));
#27821=CARTESIAN_POINT('Ctrl Pts',(40.9,30.5996231131986,15.9346498339374));
#27822=CARTESIAN_POINT('Ctrl Pts',(40.7333430442943,30.744088881243,16.0180571840065));
#27823=CARTESIAN_POINT('Ctrl Pts',(40.5666590123842,30.8885761375987,16.101476940358));
#27824=CARTESIAN_POINT('Ctrl Pts',(40.4,31.0330398077868,16.1848830792292));
#27825=CARTESIAN_POINT('Origin',(40.4,0.,0.));
#27826=CARTESIAN_POINT('Origin',(35.7,0.,0.));
#27827=CARTESIAN_POINT('',(30.5,31.0562879796886,16.1402285275843));
#27828=CARTESIAN_POINT('Ctrl Pts',(40.3999012894849,31.0330346270951,16.1848928782182));
#27829=CARTESIAN_POINT('Ctrl Pts',(39.2494626810401,31.0330116996609,16.1849362443212));
#27830=CARTESIAN_POINT('Ctrl Pts',(38.0976708836828,31.0329190263647,16.1851115327779));
#27831=CARTESIAN_POINT('Ctrl Pts',(36.9467340384723,31.0328856894588,16.1851746119074));
#27832=CARTESIAN_POINT('Ctrl Pts',(36.745427730736,31.032879858618,16.1851856448557));
#27833=CARTESIAN_POINT('Ctrl Pts',(36.5441475779313,31.0328758430124,16.1851932450653));
#27834=CARTESIAN_POINT('Ctrl Pts',(36.3429119519248,31.0328722727086,16.1852000001162));
#27835=CARTESIAN_POINT('Ctrl Pts',(36.2102758775794,31.0328699194916,16.1852044524265));
#27836=CARTESIAN_POINT('Ctrl Pts',(36.0822774296293,31.0328678560427,16.1852084224022));
#27837=CARTESIAN_POINT('Ctrl Pts',(35.9587202262686,31.0328657167445,16.1852125810274));
#27838=CARTESIAN_POINT('Ctrl Pts',(35.7925662245335,31.0328628399153,16.1852181733537));
#27839=CARTESIAN_POINT('Ctrl Pts',(35.6344388155487,31.0328598211429,16.1852241162452));
#27840=CARTESIAN_POINT('Ctrl Pts',(35.4837714463449,31.032856216152,16.1852312078526));
#27841=CARTESIAN_POINT('Ctrl Pts',(35.3175474553595,31.0328522389406,16.1852390316786));
#27842=CARTESIAN_POINT('Ctrl Pts',(35.1604041224851,31.0328475520712,16.1852482463284));
#27843=CARTESIAN_POINT('Ctrl Pts',(35.011642794874,31.0328419178902,16.1852592402397));
#27844=CARTESIAN_POINT('Ctrl Pts',(34.9979272091186,31.0328413984266,16.1852602538629));
#27845=CARTESIAN_POINT('Ctrl Pts',(34.9842829110392,31.0328408711132,16.1852612822246));
#27846=CARTESIAN_POINT('Ctrl Pts',(34.9707093736272,31.0328403358797,16.1852623254084));
#27847=CARTESIAN_POINT('Ctrl Pts',(34.8522491799023,31.0328356647415,16.1852714295754));
#27848=CARTESIAN_POINT('Ctrl Pts',(34.7391835006529,31.0328304196803,16.1852816068676));
#27849=CARTESIAN_POINT('Ctrl Pts',(34.6312849042887,31.0328252639047,16.1852915612823));
#27850=CARTESIAN_POINT('Ctrl Pts',(34.5096795260851,31.0328194531708,16.1853027802453));
#27851=CARTESIAN_POINT('Ctrl Pts',(34.3946370581326,31.0328137541413,16.1853137193614));
#27852=CARTESIAN_POINT('Ctrl Pts',(34.2857585821188,31.0328086821746,16.1853233495613));
#27853=CARTESIAN_POINT('Ctrl Pts',(34.1786801908151,31.0328036940625,16.1853328205454));
#27854=CARTESIAN_POINT('Ctrl Pts',(34.0775620514827,31.0327993031901,16.185341043166));
#27855=CARTESIAN_POINT('Ctrl Pts',(33.9819758246427,31.0327957057952,16.1853475980775));
#27856=CARTESIAN_POINT('Ctrl Pts',(33.9184449689727,31.0327933148067,16.1853519547631));
#27857=CARTESIAN_POINT('Ctrl Pts',(33.8573517602305,31.0327912624254,16.1853555977387));
#27858=CARTESIAN_POINT('Ctrl Pts',(33.7984399511826,31.0327894081824,16.1853587887284));
#27859=CARTESIAN_POINT('Ctrl Pts',(33.7337970612213,31.0327873735543,16.1853622901453));
#27860=CARTESIAN_POINT('Ctrl Pts',(33.6717809742681,31.0327855776264,16.1853652470742));
#27861=CARTESIAN_POINT('Ctrl Pts',(33.6121191806454,31.0327838881567,16.1853678991828));
#27862=CARTESIAN_POINT('Ctrl Pts',(33.5695978710648,31.0327826840617,16.1853697893561));
#27863=CARTESIAN_POINT('Ctrl Pts',(33.5282738752657,31.0327815352149,16.185371522363));
#27864=CARTESIAN_POINT('Ctrl Pts',(33.4880643388298,31.032780407062,16.1853731585247));
#27865=CARTESIAN_POINT('Ctrl Pts',(33.4508270573206,31.0327793623013,16.1853746737428));
#27866=CARTESIAN_POINT('Ctrl Pts',(33.4145509216558,31.0327783314862,16.1853761126592));
#27867=CARTESIAN_POINT('Ctrl Pts',(33.3793439789548,31.0327771639657,16.1853777420673));
#27868=CARTESIAN_POINT('Ctrl Pts',(33.3411337035362,31.0327758968498,16.1853795104722));
#27869=CARTESIAN_POINT('Ctrl Pts',(33.3041826660689,31.0327744688781,16.1853815029502));
#27870=CARTESIAN_POINT('Ctrl Pts',(33.2685652776782,31.0327727495066,16.1853839484229));
#27871=CARTESIAN_POINT('Ctrl Pts',(33.231009447455,31.0327709365599,16.1853865269881));
#27872=CARTESIAN_POINT('Ctrl Pts',(33.1949357943681,31.0327688002292,16.185389608116));
#27873=CARTESIAN_POINT('Ctrl Pts',(33.1603699172393,31.0327662471215,16.1853933524012));
#27874=CARTESIAN_POINT('Ctrl Pts',(33.1223715679418,31.0327634404841,16.1853974685027));
#27875=CARTESIAN_POINT('Ctrl Pts',(33.0861949166475,31.0327601306123,16.1854023852333));
#27876=CARTESIAN_POINT('Ctrl Pts',(33.0518089354073,31.0327562557942,16.1854082033113));
#27877=CARTESIAN_POINT('Ctrl Pts',(33.0341030813059,31.0327542605926,16.1854111991264));
#27878=CARTESIAN_POINT('Ctrl Pts',(33.0168710360021,31.032752116523,16.1854144322605));
#27879=CARTESIAN_POINT('Ctrl Pts',(33.0001033802535,31.0327498200704,16.1854179076007));
#27880=CARTESIAN_POINT('Ctrl Pts',(32.9420348133412,31.0327418671573,16.1854299431544));
#27881=CARTESIAN_POINT('Ctrl Pts',(32.8874145324497,31.0328461364757,16.1852296143114));
#27882=CARTESIAN_POINT('Ctrl Pts',(32.8357863520582,31.0330149777623,16.1849068811705));
#27883=CARTESIAN_POINT('Ctrl Pts',(32.7779739682632,31.0332040434467,16.1845454899291));
#27884=CARTESIAN_POINT('Ctrl Pts',(32.7239136589685,31.0334742654593,16.1840302574575));
#27885=CARTESIAN_POINT('Ctrl Pts',(32.6729278684755,31.033785409572,16.1834371021678));
#27886=CARTESIAN_POINT('Ctrl Pts',(32.6180801336262,31.0341201214522,16.1827990180322));
#27887=CARTESIAN_POINT('Ctrl Pts',(32.5667902508433,31.0345025939175,16.1820699950122));
#27888=CARTESIAN_POINT('Ctrl Pts',(32.5181731636799,31.034906696383,16.1812992842338));
#27889=CARTESIAN_POINT('Ctrl Pts',(32.4659536029869,31.0353407424038,16.1804714646211));
#27890=CARTESIAN_POINT('Ctrl Pts',(32.416817513625,31.0358001425894,16.1795947944396));
#27891=CARTESIAN_POINT('Ctrl Pts',(32.3696233879015,31.0362725138779,16.1786925325962));
#27892=CARTESIAN_POINT('Ctrl Pts',(32.3182581618433,31.0367866341767,16.1777105272546));
#27893=CARTESIAN_POINT('Ctrl Pts',(32.2691934412649,31.0373164741888,16.1766975364929));
#27894=CARTESIAN_POINT('Ctrl Pts',(32.2209064724825,31.0378627004433,16.1756521425246));
#27895=CARTESIAN_POINT('Ctrl Pts',(32.1715370438648,31.0384211715746,16.1745833137248));
#27896=CARTESIAN_POINT('Ctrl Pts',(32.1229805798605,31.0389971805319,16.1734798401021));
#27897=CARTESIAN_POINT('Ctrl Pts',(32.0735591134784,31.039601856364,16.1723205501867));
#27898=CARTESIAN_POINT('Ctrl Pts',(32.0254239419648,31.0401907942692,16.1711914331653));
#27899=CARTESIAN_POINT('Ctrl Pts',(31.976468287942,31.04080728099,16.1700086968177));
#27900=CARTESIAN_POINT('Ctrl Pts',(31.9250947921535,31.041465759884,16.1687449477339));
#27901=CARTESIAN_POINT('Ctrl Pts',(31.8952919104891,31.0418477578044,16.1680118194191));
#27902=CARTESIAN_POINT('Ctrl Pts',(31.8646744620485,31.0422439429541,16.1672513233696));
#27903=CARTESIAN_POINT('Ctrl Pts',(31.8329224323944,31.0426570718779,16.1664582369103));
#27904=CARTESIAN_POINT('Ctrl Pts',(31.7319354368356,31.0439710240642,16.1639358337881));
#27905=CARTESIAN_POINT('Ctrl Pts',(31.6284526822057,31.0453389332579,16.1613063818566));
#27906=CARTESIAN_POINT('Ctrl Pts',(31.5232336354319,31.0466795487252,16.1587277943726));
#27907=CARTESIAN_POINT('Ctrl Pts',(31.418880786625,31.0480091278028,16.156170434673));
#27908=CARTESIAN_POINT('Ctrl Pts',(31.3128198672023,31.0493111005243,16.1536645426213));
#27909=CARTESIAN_POINT('Ctrl Pts',(31.2058402970406,31.0505011542277,16.1513736799427));
#27910=CARTESIAN_POINT('Ctrl Pts',(31.1464339374051,31.0511619977718,16.1501015509562));
#27911=CARTESIAN_POINT('Ctrl Pts',(31.0867451889514,31.051788304276,16.1488957763821));
#27912=CARTESIAN_POINT('Ctrl Pts',(31.0269161235859,31.052366291213,16.1477831210734));
#27913=CARTESIAN_POINT('Ctrl Pts',(30.9223727403119,31.0533762469848,16.1458389029967));
#27914=CARTESIAN_POINT('Ctrl Pts',(30.8173993541569,31.0542375463396,16.1441811147896));
#27915=CARTESIAN_POINT('Ctrl Pts',(30.7129204018003,31.0548748925162,16.1429541726495));
#27916=CARTESIAN_POINT('Ctrl Pts',(30.6397146645874,31.0553214647269,16.1420944855847));
#27917=CARTESIAN_POINT('Ctrl Pts',(30.5667525557982,31.0556583368409,16.1414458510595));
#27918=CARTESIAN_POINT('Ctrl Pts',(30.4943593393942,31.0558660149161,16.1410459118957));
#27919=CARTESIAN_POINT('',(30.5,29.559989655385,18.7405179110273));
#27920=CARTESIAN_POINT('Origin',(30.5,0.,0.));
#27921=CARTESIAN_POINT('Ctrl Pts',(30.5049791805002,29.5605178050972,18.7395177484757));
#27922=CARTESIAN_POINT('Ctrl Pts',(30.5973676827742,29.5601622646428,18.7400797009802));
#27923=CARTESIAN_POINT('Ctrl Pts',(30.6891105694844,29.5595425101548,18.7410567560112));
#27924=CARTESIAN_POINT('Ctrl Pts',(30.7806774793078,29.5587264396734,18.7423441244047));
#27925=CARTESIAN_POINT('Ctrl Pts',(30.8441888930627,29.5581604077946,18.7432370516297));
#27926=CARTESIAN_POINT('Ctrl Pts',(30.9076166453415,29.5574994222391,18.7442800408075));
#27927=CARTESIAN_POINT('Ctrl Pts',(30.9711288096738,29.5567612578199,18.745445599991));
#27928=CARTESIAN_POINT('Ctrl Pts',(31.0735567068109,29.5555707987954,18.7473253308647));
#27929=CARTESIAN_POINT('Ctrl Pts',(31.1762019082913,29.5541800414697,18.749523155664));
#27930=CARTESIAN_POINT('Ctrl Pts',(31.2798872709468,29.5526737444514,18.7519033574721));
#27931=CARTESIAN_POINT('Ctrl Pts',(31.3828989348253,29.5511772346434,18.7542680938471));
#27932=CARTESIAN_POINT('Ctrl Pts',(31.4869372222095,29.5495656759357,18.7568144117909));
#27933=CARTESIAN_POINT('Ctrl Pts',(31.5928574097401,29.5479181178243,18.7594156373082));
#27934=CARTESIAN_POINT('Ctrl Pts',(31.6516459294275,29.5470036792765,18.7608593866171));
#27935=CARTESIAN_POINT('Ctrl Pts',(31.71101503912,29.5460781618906,18.762320034785));
#27936=CARTESIAN_POINT('Ctrl Pts',(31.7711176725242,29.5451562912554,18.7637740491309));
#27937=CARTESIAN_POINT('Ctrl Pts',(31.8409082760364,29.5440858238841,18.7654624366935));
#27938=CARTESIAN_POINT('Ctrl Pts',(31.9056373311746,29.5431152615714,18.766993363124));
#27939=CARTESIAN_POINT('Ctrl Pts',(31.9658882086281,29.5422441375118,18.768367583494));
#27940=CARTESIAN_POINT('Ctrl Pts',(32.0341093482754,29.5412577771693,18.7699235920324));
#27941=CARTESIAN_POINT('Ctrl Pts',(32.0965888127921,29.5403982847665,18.7712796560442));
#27942=CARTESIAN_POINT('Ctrl Pts',(32.1542362617659,29.5396480149484,18.7724634074922));
#27943=CARTESIAN_POINT('Ctrl Pts',(32.2151538519828,29.5388551849074,18.773714309083));
#27944=CARTESIAN_POINT('Ctrl Pts',(32.2706761902186,29.5381836213573,18.7747738843964));
#27945=CARTESIAN_POINT('Ctrl Pts',(32.3219402247756,29.5376060245817,18.7756849339008));
#27946=CARTESIAN_POINT('Ctrl Pts',(32.3761674213252,29.5369950415769,18.7766486438579));
#27947=CARTESIAN_POINT('Ctrl Pts',(32.4256304058852,29.5364887148647,18.7774469218491));
#27948=CARTESIAN_POINT('Ctrl Pts',(32.4717350314086,29.5360572749796,18.7781265619113));
#27949=CARTESIAN_POINT('Ctrl Pts',(32.5214923281269,29.535591653968,18.7788600469326));
#27950=CARTESIAN_POINT('Ctrl Pts',(32.5673384642538,29.5352128774492,18.7794559410666));
#27951=CARTESIAN_POINT('Ctrl Pts',(32.6111004962939,29.5348934788927,18.7799576530151));
#27952=CARTESIAN_POINT('Ctrl Pts',(32.6551147163185,29.5345722397343,18.780462256185));
#27953=CARTESIAN_POINT('Ctrl Pts',(32.6970214084873,29.5343108907557,18.7808718608788));
#27954=CARTESIAN_POINT('Ctrl Pts',(32.7387279964579,29.5340950825231,18.7812095285094));
#27955=CARTESIAN_POINT('Ctrl Pts',(32.7800761354879,29.533881129063,18.781544294042));
#27956=CARTESIAN_POINT('Ctrl Pts',(32.8212277342352,29.5337116838823,18.7818087481602));
#27957=CARTESIAN_POINT('Ctrl Pts',(32.8640829337527,29.5335890251803,18.782000095504));
#27958=CARTESIAN_POINT('Ctrl Pts',(32.9037320332527,29.5334755428694,18.7821771276951));
#27959=CARTESIAN_POINT('Ctrl Pts',(32.9448394203909,29.5334018918636,18.782291920091));
#27960=CARTESIAN_POINT('Ctrl Pts',(32.9889438598236,29.5333868654405,18.7823158450367));
#27961=CARTESIAN_POINT('Ctrl Pts',(32.9925102269246,29.533385650376,18.7823177796523));
#27962=CARTESIAN_POINT('Ctrl Pts',(32.9960962106235,29.5333848297967,18.7823191027632));
#27963=CARTESIAN_POINT('Ctrl Pts',(32.9997026353888,29.5333844198653,18.7823197895505));
#27964=CARTESIAN_POINT('Ctrl Pts',(33.0361388185045,29.5333802782742,18.7823267282529));
#27965=CARTESIAN_POINT('Ctrl Pts',(33.0740002606604,29.5333765562528,18.7823330770045));
#27966=CARTESIAN_POINT('Ctrl Pts',(33.1140504028667,29.5333733966325,18.7823389179975));
#27967=CARTESIAN_POINT('Ctrl Pts',(33.2460690464807,29.5333629814689,18.7823581718611));
#27968=CARTESIAN_POINT('Ctrl Pts',(33.3720922029406,29.5333587011923,18.7823661897829));
#27969=CARTESIAN_POINT('Ctrl Pts',(33.4992849360725,29.5333546566755,18.7823737360729));
#27970=CARTESIAN_POINT('Ctrl Pts',(33.6626792864137,29.5333494610078,18.7823834301893));
#27971=CARTESIAN_POINT('Ctrl Pts',(33.8280037294636,29.5333446544025,18.7823923459959));
#27972=CARTESIAN_POINT('Ctrl Pts',(33.9928746198634,29.5333373313072,18.7824059536077));
#27973=CARTESIAN_POINT('Ctrl Pts',(34.322616400663,29.5333226851164,18.7824331688313));
#27974=CARTESIAN_POINT('Ctrl Pts',(34.650543970862,29.5332979729651,18.7824791512758));
#27975=CARTESIAN_POINT('Ctrl Pts',(34.979144925286,29.5332814027048,18.7825099763789));
#27976=CARTESIAN_POINT('Ctrl Pts',(35.30774587971,29.5332648324445,18.782540801482));
#27977=CARTESIAN_POINT('Ctrl Pts',(35.6370202183589,29.5332564040751,18.7825564692435));
#27978=CARTESIAN_POINT('Ctrl Pts',(35.9661418060973,29.5332492722834,18.7825697306317));
#27979=CARTESIAN_POINT('Ctrl Pts',(36.2952633938357,29.5332421404917,18.7825829920199));
#27980=CARTESIAN_POINT('Ctrl Pts',(36.6242322306637,29.5332363052776,18.7825938470347));
#27981=CARTESIAN_POINT('Ctrl Pts',(36.9531363303404,29.533224710841,18.782615411986));
#27982=CARTESIAN_POINT('Ctrl Pts',(38.1022190076918,29.5331842036954,18.7826907528288));
#27983=CARTESIAN_POINT('Ctrl Pts',(39.2505115204485,29.5330734009978,18.782896816333));
#27984=CARTESIAN_POINT('Ctrl Pts',(40.400093943525,29.533045998731,18.7829477771169));
#27985=CARTESIAN_POINT('Ctrl Pts',(6.89999999997365,5.3678954269134,9.63452070648359));
#27986=CARTESIAN_POINT('Ctrl Pts',(6.99168932310453,5.42175501956,9.60499723839754));
#27987=CARTESIAN_POINT('Ctrl Pts',(7.08383915760479,5.47527828673705,9.57508016834563));
#27988=CARTESIAN_POINT('Ctrl Pts',(8.15762752947027,6.09209251732962,9.22342495405908));
#27989=CARTESIAN_POINT('Ctrl Pts',(9.16608342448599,6.61836595106258,8.84591675027099));
#27990=CARTESIAN_POINT('Ctrl Pts',(11.2535425311854,7.53037930120419,8.09542754093137));
#27991=CARTESIAN_POINT('Ctrl Pts',(12.2577133097064,7.91666449612081,7.70725001371761));
#27992=CARTESIAN_POINT('Ctrl Pts',(14.356433377742,8.58141250110813,6.97440810645327));
#27993=CARTESIAN_POINT('Ctrl Pts',(15.3659105035251,8.85322312286061,6.61345583116597));
#27994=CARTESIAN_POINT('Ctrl Pts',(17.4728641219044,9.31281879192962,5.96623757129008));
#27995=CARTESIAN_POINT('Ctrl Pts',(18.4890996814195,9.49384943617778,5.66020885204394));
#27996=CARTESIAN_POINT('Ctrl Pts',(19.8476172011441,9.68599953593307,5.32865724601649));
#27997=CARTESIAN_POINT('Ctrl Pts',(20.3454889307686,9.75195458239818,5.2093054291626));
#27998=CARTESIAN_POINT('Ctrl Pts',(21.3782040612024,9.87366876552718,4.97678151322347));
#27999=CARTESIAN_POINT('Ctrl Pts',(22.1792648896895,9.95072592994714,4.81935607344487));
#28000=CARTESIAN_POINT('Ctrl Pts',(22.8542621828909,10.0067883222623,4.70591921690555));
#28001=CARTESIAN_POINT('Ctrl Pts',(23.1054579010968,10.0267605301623,4.66456206383029));
#28002=CARTESIAN_POINT('Ctrl Pts',(23.6171513959785,10.0644076466806,4.58448144656259));
#28003=CARTESIAN_POINT('Ctrl Pts',(24.1360713221937,10.0979855598765,4.51012725444835));
#28004=CARTESIAN_POINT('Ctrl Pts',(24.6624927871864,10.1277002159266,4.44285620865166));
#28005=CARTESIAN_POINT('Ctrl Pts',(25.1928168818088,10.154786256444,4.38095271718121));
#28006=CARTESIAN_POINT('Ctrl Pts',(25.5948982287615,10.1721457030179,4.34117176259644));
#28007=CARTESIAN_POINT('Ctrl Pts',(26.1232031889651,10.1922876384417,4.29604941535507));
#28008=CARTESIAN_POINT('Ctrl Pts',(27.1768897027567,10.2241871753182,4.22326129112041));
#28009=CARTESIAN_POINT('Ctrl Pts',(28.2111297865347,10.2325109692973,4.19969555688314));
#28010=CARTESIAN_POINT('Ctrl Pts',(29.1277555719713,10.2421056253618,4.17661492679514));
#28011=CARTESIAN_POINT('Ctrl Pts',(29.4767605677587,10.2448788784735,4.1700561490002));
#28012=CARTESIAN_POINT('Ctrl Pts',(30.1601418995912,10.2473221772452,4.16421367130872));
#28013=CARTESIAN_POINT('Ctrl Pts',(31.3500242312262,10.2457563290907,4.16794387579264));
#28014=CARTESIAN_POINT('Ctrl Pts',(32.3461596131128,10.2405791191157,4.18040640609127));
#28015=CARTESIAN_POINT('Ctrl Pts',(33.1614718826738,10.2405840900447,4.18039330945985));
#28016=CARTESIAN_POINT('Ctrl Pts',(33.4925794155279,10.2405841444578,4.18039253080268));
#28017=CARTESIAN_POINT('Ctrl Pts',(34.1499904318886,10.2405848392549,4.18039030822715));
#28018=CARTESIAN_POINT('Ctrl Pts',(34.9738731541179,10.2405865289644,4.18038393925505));
#28019=CARTESIAN_POINT('Ctrl Pts',(35.9612754428242,10.2405873001735,4.18038119412749));
#28020=CARTESIAN_POINT('Ctrl Pts',(37.936646788162,10.2405882857915,4.18037753677864));
#28021=CARTESIAN_POINT('Ctrl Pts',(39.5833333333333,10.2405934798255,4.18035859466987));
#28022=CARTESIAN_POINT('Ctrl Pts',(40.9,10.2405934798255,4.18035859466987));
#28023=CARTESIAN_POINT('Ctrl Pts',(6.71972576838711,6.5764381714634,12.8464244365415));
#28024=CARTESIAN_POINT('Ctrl Pts',(6.81144220747046,6.6482837686261,12.8102053989753));
#28025=CARTESIAN_POINT('Ctrl Pts',(6.90362823998598,6.71971524922859,12.7734498343709));
#28026=CARTESIAN_POINT('Ctrl Pts',(7.97787811486329,7.54294881554193,12.3410744046091));
#28027=CARTESIAN_POINT('Ctrl Pts',(8.98681832185142,8.24809748747637,11.871220138602));
#28028=CARTESIAN_POINT('Ctrl Pts',(11.0806583453373,9.47774891389534,10.9274240314556));
#28029=CARTESIAN_POINT('Ctrl Pts',(12.0862475175457,10.0005505115845,10.4368998098018));
#28030=CARTESIAN_POINT('Ctrl Pts',(14.197639322261,10.906656993414,9.50280276487818));
#28031=CARTESIAN_POINT('Ctrl Pts',(15.2100862637122,11.2785931828498,9.0420363325472));
#28032=CARTESIAN_POINT('Ctrl Pts',(17.3364698493954,11.9121957711898,8.20932952666153));
#28033=CARTESIAN_POINT('Ctrl Pts',(18.357279581038,12.1627870018009,7.81594677169139));
#28034=CARTESIAN_POINT('Ctrl Pts',(19.7331217809845,12.4307568384137,7.38628119283516));
#28035=CARTESIAN_POINT('Ctrl Pts',(20.2341927100358,12.5225360922774,7.23233618870704));
#28036=CARTESIAN_POINT('Ctrl Pts',(21.2777139275316,12.6928916013278,6.93114017240205));
#28037=CARTESIAN_POINT('Ctrl Pts',(22.0885637816418,12.8012350092453,6.72673758680647));
#28038=CARTESIAN_POINT('Ctrl Pts',(22.7734874647764,12.8801738355232,6.57909772915772));
#28039=CARTESIAN_POINT('Ctrl Pts',(23.0269571312139,12.9082278965574,6.52549682636868));
#28040=CARTESIAN_POINT('Ctrl Pts',(23.5444618566097,12.9612738268023,6.42148511325403));
#28041=CARTESIAN_POINT('Ctrl Pts',(24.0694383156461,13.0087020921734,6.32485290039694));
#28042=CARTESIAN_POINT('Ctrl Pts',(24.6027295908464,13.0507741241225,6.23730008137711));
#28043=CARTESIAN_POINT('Ctrl Pts',(25.1403192523141,13.0891677302172,6.15667530541499));
#28044=CARTESIAN_POINT('Ctrl Pts',(25.5484689870706,13.1137995888261,6.10479659087691));
#28045=CARTESIAN_POINT('Ctrl Pts',(26.0852808149067,13.1423647911197,6.04589855121055));
#28046=CARTESIAN_POINT('Ctrl Pts',(27.1586857291269,13.1877077660314,5.95074158602808));
#28047=CARTESIAN_POINT('Ctrl Pts',(28.1995312980844,13.1995114624862,5.92039197700573));
#28048=CARTESIAN_POINT('Ctrl Pts',(29.1157533315888,13.2130297822556,5.89061060808306));
#28049=CARTESIAN_POINT('Ctrl Pts',(29.4698938670486,13.2169740538762,5.88204921070823));
#28050=CARTESIAN_POINT('Ctrl Pts',(30.1587234046998,13.220429005539,5.8744768355958));
#28051=CARTESIAN_POINT('Ctrl Pts',(31.355731195606,13.2182120926509,5.87931523414859));
#28052=CARTESIAN_POINT('Ctrl Pts',(32.350180243561,13.2109234983782,5.89537176970751));
#28053=CARTESIAN_POINT('Ctrl Pts',(33.1605031382466,13.2109314016452,5.89535013085609));
#28054=CARTESIAN_POINT('Ctrl Pts',(33.4922179295252,13.2109314596682,5.89534881762645));
#28055=CARTESIAN_POINT('Ctrl Pts',(34.1493400019899,13.2109325467447,5.89534512891168));
#28056=CARTESIAN_POINT('Ctrl Pts',(34.9735241318652,13.2109351472382,5.8953345252407));
#28057=CARTESIAN_POINT('Ctrl Pts',(35.9608954520827,13.2109363413972,5.89532995964262));
#28058=CARTESIAN_POINT('Ctrl Pts',(37.9363824842976,13.2109378608691,5.8953238722353));
#28059=CARTESIAN_POINT('Ctrl Pts',(39.5833333333333,13.2109458830841,5.89529235427929));
#28060=CARTESIAN_POINT('Ctrl Pts',(40.9,13.2109458830841,5.89529235427929));
#28061=CARTESIAN_POINT('Ctrl Pts',(6.48177011792015,9.40621265917915,20.336764848396));
#28062=CARTESIAN_POINT('Ctrl Pts',(6.57271435585529,9.51911083717171,20.2851799357091));
#28063=CARTESIAN_POINT('Ctrl Pts',(6.66411141569866,9.63139437446865,20.2327517601296));
#28064=CARTESIAN_POINT('Ctrl Pts',(7.73048017258431,10.9276768808967,19.614616528956));
#28065=CARTESIAN_POINT('Ctrl Pts',(8.73292722985418,12.0456324995184,18.9319609573801));
#28066=CARTESIAN_POINT('Ctrl Pts',(10.8102906905198,14.0013807284478,17.5485371602851));
#28067=CARTESIAN_POINT('Ctrl Pts',(11.8125687231201,14.8418955382559,16.8218444562665));
#28068=CARTESIAN_POINT('Ctrl Pts',(13.9177445864075,16.3050153868123,15.4271303717406));
#28069=CARTESIAN_POINT('Ctrl Pts',(14.9296562678442,16.9116612373854,14.7350649820735));
#28070=CARTESIAN_POINT('Ctrl Pts',(17.0680844879216,17.9535844659564,13.4708635112562));
#28071=CARTESIAN_POINT('Ctrl Pts',(18.0932339179161,18.3688941094638,12.8729609429));
#28072=CARTESIAN_POINT('Ctrl Pts',(19.4933464326809,18.8183285494774,12.2099892645604));
#28073=CARTESIAN_POINT('Ctrl Pts',(19.9993272808496,18.971430097181,11.9744841299437));
#28074=CARTESIAN_POINT('Ctrl Pts',(21.0600020168761,19.2581324129063,11.5100300116438));
#28075=CARTESIAN_POINT('Ctrl Pts',(21.8888875769483,19.4420158954032,11.1928649299996));
#28076=CARTESIAN_POINT('Ctrl Pts',(22.5933490549503,19.5764520117208,10.962505511385));
#28077=CARTESIAN_POINT('Ctrl Pts',(22.8513437851799,19.6238525927722,10.8796937171906));
#28078=CARTESIAN_POINT('Ctrl Pts',(23.3805933886566,19.7139851739534,10.7182299385361));
#28079=CARTESIAN_POINT('Ctrl Pts',(23.9182257576785,19.7948254980796,10.5680285062335));
#28080=CARTESIAN_POINT('Ctrl Pts',(24.4662138806868,19.8668205194741,10.4315004891655));
#28081=CARTESIAN_POINT('Ctrl Pts',(25.0195744741822,19.9326328666884,10.3055778221167));
#28082=CARTESIAN_POINT('Ctrl Pts',(25.4412458088222,19.9749776253082,10.2242864909386));
#28083=CARTESIAN_POINT('Ctrl Pts',(25.9971983460992,20.0240850656221,10.131797107587));
#28084=CARTESIAN_POINT('Ctrl Pts',(27.1157050405652,20.102368552767,9.98182332250462));
#28085=CARTESIAN_POINT('Ctrl Pts',(28.1723100127449,20.1222437541335,9.93573708068025));
#28086=CARTESIAN_POINT('Ctrl Pts',(29.0876106506766,20.1449463132817,9.89029022572785));
#28087=CARTESIAN_POINT('Ctrl Pts',(29.4537207931442,20.1517438988729,9.87684873205164));
#28088=CARTESIAN_POINT('Ctrl Pts',(30.1552759232946,20.1576060163182,9.86516345924738));
#28089=CARTESIAN_POINT('Ctrl Pts',(31.368924127636,20.1538463873917,9.87263514017793));
#28090=CARTESIAN_POINT('Ctrl Pts',(32.3594787154311,20.1416711708076,9.89702302165624));
#28091=CARTESIAN_POINT('Ctrl Pts',(33.1581760188914,20.1416983285705,9.89696607979067));
#28092=CARTESIAN_POINT('Ctrl Pts',(33.4913102145729,20.1416998058431,9.89696201382195));
#28093=CARTESIAN_POINT('Ctrl Pts',(34.1477617736107,20.1417043298969,9.89695193052414));
#28094=CARTESIAN_POINT('Ctrl Pts',(34.9726616332633,20.1417171222835,9.89692218573783));
#28095=CARTESIAN_POINT('Ctrl Pts',(35.9599657908142,20.1417226604566,9.89690948638393));
#28096=CARTESIAN_POINT('Ctrl Pts',(37.9357298104643,20.1417300151411,9.89689244880616));
#28097=CARTESIAN_POINT('Ctrl Pts',(39.5833333333333,20.1417681573542,9.89680446003461));
#28098=CARTESIAN_POINT('Ctrl Pts',(40.9,20.1417681573542,9.89680446003461));
#28099=CARTESIAN_POINT('Ctrl Pts',(6.40644620858992,12.3446157076951,27.7818319413302));
#28100=CARTESIAN_POINT('Ctrl Pts',(6.49686818484384,12.4976194141968,27.7146057723315));
#28101=CARTESIAN_POINT('Ctrl Pts',(6.58771883172007,12.6497754970257,27.6462615383487));
#28102=CARTESIAN_POINT('Ctrl Pts',(7.64885870107047,14.4089312086777,26.8389674658771));
#28103=CARTESIAN_POINT('Ctrl Pts',(8.64786699401839,15.9309901815184,25.9406999974138));
#28104=CARTESIAN_POINT('Ctrl Pts',(10.7071344443812,18.5841088194585,24.1258468463739));
#28105=CARTESIAN_POINT('Ctrl Pts',(11.7059636153277,19.7351568023896,23.1640388241121));
#28106=CARTESIAN_POINT('Ctrl Pts',(13.7894167134297,21.7274097031724,21.32755345859));
#28107=CARTESIAN_POINT('Ctrl Pts',(14.7964804448639,22.5625068415354,20.40896606215));
#28108=CARTESIAN_POINT('Ctrl Pts',(16.9150096963281,23.9923642448819,18.734786787185));
#28109=CARTESIAN_POINT('Ctrl Pts',(17.9356563974909,24.568778311437,17.9376031564435));
#28110=CARTESIAN_POINT('Ctrl Pts',(19.3316378726113,25.1942531765859,17.0495061236355));
#28111=CARTESIAN_POINT('Ctrl Pts',(19.8373783148988,25.4080883980548,16.733671277521));
#28112=CARTESIAN_POINT('Ctrl Pts',(20.8986146451321,25.8097110946141,16.1088561234904));
#28113=CARTESIAN_POINT('Ctrl Pts',(21.7322089233615,26.0695581056351,15.6790344990822));
#28114=CARTESIAN_POINT('Ctrl Pts',(22.4452152218927,26.2607608176432,15.3644450466695));
#28115=CARTESIAN_POINT('Ctrl Pts',(22.7053175952387,26.3278633535721,15.2520352575855));
#28116=CARTESIAN_POINT('Ctrl Pts',(23.2405350109147,26.4560495577169,15.0319031635372));
#28117=CARTESIAN_POINT('Ctrl Pts',(23.7856351879594,26.5714803865859,14.8265027181049));
#28118=CARTESIAN_POINT('Ctrl Pts',(24.3434088150882,26.6748081507042,14.6389049166987));
#28119=CARTESIAN_POINT('Ctrl Pts',(24.9080926446007,26.7695587595052,14.4653482504621));
#28120=CARTESIAN_POINT('Ctrl Pts',(25.3404979553364,26.8308622015487,14.3526452692475));
#28121=CARTESIAN_POINT('Ctrl Pts',(25.9125607075504,26.9021372597287,14.2239063651395));
#28122=CARTESIAN_POINT('Ctrl Pts',(27.0720378258712,27.0165941086124,14.0136986134135));
#28123=CARTESIAN_POINT('Ctrl Pts',(28.1454151442859,27.0445191043407,13.9518646781025));
#28124=CARTESIAN_POINT('Ctrl Pts',(29.0596751952944,27.0764264216485,13.890725520751));
#28125=CARTESIAN_POINT('Ctrl Pts',(29.4376599373188,27.0863532011149,13.8719255145712));
#28126=CARTESIAN_POINT('Ctrl Pts',(30.1519376760718,27.0947220176404,13.855954576287));
#28127=CARTESIAN_POINT('Ctrl Pts',(31.3821999577689,27.0893514143296,13.8661782937677));
#28128=CARTESIAN_POINT('Ctrl Pts',(32.3688386893657,27.0723527225427,13.8987881217581));
#28129=CARTESIAN_POINT('Ctrl Pts',(33.1558986739574,27.0724155351932,13.8986675947835));
#28130=CARTESIAN_POINT('Ctrl Pts',(33.49045038666,27.072419804706,13.8986584195583));
#28131=CARTESIAN_POINT('Ctrl Pts',(34.1462287076184,27.0724307945236,13.8986367255003));
#28132=CARTESIAN_POINT('Ctrl Pts',(34.9718350023128,27.0724629552156,13.8985720488061));
#28133=CARTESIAN_POINT('Ctrl Pts',(35.9590682028415,27.0724767217601,13.8985445297568));
#28134=CARTESIAN_POINT('Ctrl Pts',(37.9351039480424,27.072495155898,13.8985075170899));
#28135=CARTESIAN_POINT('Ctrl Pts',(39.5833333333333,27.0725904316243,13.8983165657899));
#28136=CARTESIAN_POINT('Ctrl Pts',(40.9,27.0725904316243,13.8983165657899));
#28137=CARTESIAN_POINT('Ctrl Pts',(6.37427268165564,14.0406695266741,32.0290848932163));
#28138=CARTESIAN_POINT('Ctrl Pts',(6.46448755772839,14.2166050753401,31.9528098065586));
#28139=CARTESIAN_POINT('Ctrl Pts',(6.55512327887566,14.3915605358513,31.8752581000468));
#28140=CARTESIAN_POINT('Ctrl Pts',(7.61410360785656,16.4151695040826,30.958672886913));
#28141=CARTESIAN_POINT('Ctrl Pts',(8.61142775869687,18.1677152487792,29.9361952854453));
#28142=CARTESIAN_POINT('Ctrl Pts',(10.6634825022472,21.2183968262284,27.8730682250753));
#28143=CARTESIAN_POINT('Ctrl Pts',(11.6607542873627,22.5462154536683,26.7761583709752));
#28144=CARTESIAN_POINT('Ctrl Pts',(13.7353039743977,24.8383185913233,24.6873364683673));
#28145=CARTESIAN_POINT('Ctrl Pts',(14.7402095633116,25.802985911944,23.6392130729629));
#28146=CARTESIAN_POINT('Ctrl Pts',(16.8490881066137,27.450307490631,21.733995182915));
#28147=CARTESIAN_POINT('Ctrl Pts',(17.8672038783315,28.117536242687,20.8239061433235));
#28148=CARTESIAN_POINT('Ctrl Pts',(19.2585933984997,28.8404836901117,19.811022849419));
#28149=CARTESIAN_POINT('Ctrl Pts',(19.7636418533908,29.0884650342026,19.4499572035579));
#28150=CARTESIAN_POINT('Ctrl Pts',(20.8231816497994,29.5540603372584,18.7357747989968));
#28151=CARTESIAN_POINT('Ctrl Pts',(21.6568670511735,29.8562628482713,18.2431916560479));
#28152=CARTESIAN_POINT('Ctrl Pts',(22.3720072062877,30.0792593376712,17.8815051531588));
#28153=CARTESIAN_POINT('Ctrl Pts',(22.6326824787813,30.1574913312728,17.7523977438431));
#28154=CARTESIAN_POINT('Ctrl Pts',(23.1697036949937,30.3071564102286,17.4991937768336));
#28155=CARTESIAN_POINT('Ctrl Pts',(23.7174377716562,30.4422233412819,17.2625030946595));
#28156=CARTESIAN_POINT('Ctrl Pts',(24.2790946262572,30.5634410393028,17.0457855087881));
#28157=CARTESIAN_POINT('Ctrl Pts',(24.8485847331463,30.6748008187179,16.8449230908939));
#28158=CARTESIAN_POINT('Ctrl Pts',(25.2859632686137,30.7471152582869,16.714000734413));
#28159=CARTESIAN_POINT('Ctrl Pts',(25.8659001690755,30.8313513860032,16.5640760155963));
#28160=CARTESIAN_POINT('Ctrl Pts',(27.0467877055032,30.9672841404844,16.3181083484215));
#28161=CARTESIAN_POINT('Ctrl Pts',(28.1301993946288,30.9999203594232,16.2470842981322));
#28162=CARTESIAN_POINT('Ctrl Pts',(29.0438132065911,31.0370949113971,16.1769735529556));
#28163=CARTESIAN_POINT('Ctrl Pts',(29.4285323170642,31.0489002942269,16.1549555741443));
#28164=CARTESIAN_POINT('Ctrl Pts',(30.1500796604944,31.0587367393328,16.1364761766636));
#28165=CARTESIAN_POINT('Ctrl Pts',(31.3898224001987,31.0524272220083,16.1483068856791));
#28166=CARTESIAN_POINT('Ctrl Pts',(32.3742147772173,31.0327017051641,16.1855693458549));
#28167=CARTESIAN_POINT('Ctrl Pts',(33.1546196294426,31.0327939306214,16.1853991323255));
#28168=CARTESIAN_POINT('Ctrl Pts',(33.4899805045662,31.0328008093452,16.185385634532));
#28169=CARTESIAN_POINT('Ctrl Pts',(34.1453728987309,31.0328173216774,16.1853546639146));
#28170=CARTESIAN_POINT('Ctrl Pts',(34.9713787068036,31.0328663827335,16.1852616946182));
#28171=CARTESIAN_POINT('Ctrl Pts',(35.9585696612047,31.0328872804502,16.1852222245757));
#28172=CARTESIAN_POINT('Ctrl Pts',(37.9347583211501,31.0329153648958,16.1851690519237));
#28173=CARTESIAN_POINT('Ctrl Pts',(39.5833333333333,31.0330603026358,16.1848949119358));
#28174=CARTESIAN_POINT('Ctrl Pts',(40.9,31.0330603026358,16.1848949119358));
#28175=CARTESIAN_POINT('',(40.9,29.2992994660114,15.1839076262003));
#28176=CARTESIAN_POINT('Ctrl Pts',(40.9,29.2992994660114,15.1839076262003));
#28177=CARTESIAN_POINT('Ctrl Pts',(40.9,29.7327406817405,15.4341550287793));
#28178=CARTESIAN_POINT('Ctrl Pts',(40.9,30.1661818974696,15.6844024313584));
#28179=CARTESIAN_POINT('Ctrl Pts',(40.9,30.5996231131986,15.9346498339374));
#28180=CARTESIAN_POINT('',(38.,29.2992994660114,15.1839076262003));
#28181=CARTESIAN_POINT('Ctrl Pts',(38.,29.2992994660114,15.1839076262003));
#28182=CARTESIAN_POINT('Ctrl Pts',(38.9666666666667,29.2992994660114,15.1839076262003));
#28183=CARTESIAN_POINT('Ctrl Pts',(39.9333333333333,29.2992994660114,15.1839076262003));
#28184=CARTESIAN_POINT('Ctrl Pts',(40.9,29.2992994660114,15.1839076262003));
#28185=CARTESIAN_POINT('Ctrl Pts',(37.4974382384971,28.7790269720418,14.8838038109906));
#28186=CARTESIAN_POINT('Ctrl Pts',(37.6645213547146,28.9527098777879,14.9840691120819));
#28187=CARTESIAN_POINT('Ctrl Pts',(37.8313739960416,29.1261374112004,15.084184715056));
#28188=CARTESIAN_POINT('Ctrl Pts',(37.9978889629903,29.2992044501375,15.1840905833949));
#28189=CARTESIAN_POINT('',(6.9,12.9951291628659,27.0393531365015));
#28190=CARTESIAN_POINT('Ctrl Pts',(6.9,12.9951291628659,27.0393531365015));
#28191=CARTESIAN_POINT('Ctrl Pts',(6.9,11.9174419758914,24.649274247254));
#28192=CARTESIAN_POINT('Ctrl Pts',(6.90000000000115,10.8339866674746,22.230729924082));
#28193=CARTESIAN_POINT('Ctrl Pts',(6.90000000000115,8.41000082059024,16.7584145047598));
#28194=CARTESIAN_POINT('Ctrl Pts',(6.9,6.82522008706163,13.1312177506378));
#28195=CARTESIAN_POINT('Ctrl Pts',(6.9,5.36789542693312,9.63452070648529));
#28196=CARTESIAN_POINT('',(22.9245129145126,27.5141512254856,15.8853026165582));
#28197=CARTESIAN_POINT('Ctrl Pts',(22.9245129145126,27.5141512254856,15.8853026165582));
#28198=CARTESIAN_POINT('Ctrl Pts',(22.7202811020963,27.405303612937,15.9355315703924));
#28199=CARTESIAN_POINT('Ctrl Pts',(22.5089075447093,27.2924652433825,15.9922246435191));
#28200=CARTESIAN_POINT('Ctrl Pts',(22.2913349439917,27.1762359097412,16.0558281873748));
#28201=CARTESIAN_POINT('Ctrl Pts',(21.4451770585293,26.7242103933933,16.3031876434794));
#28202=CARTESIAN_POINT('Ctrl Pts',(20.522095155667,26.2108400614943,16.6965145338605));
#28203=CARTESIAN_POINT('Ctrl Pts',(19.7671428819541,25.777085937268,17.0753616782143));
#28204=CARTESIAN_POINT('Ctrl Pts',(19.5194773058393,25.634790895834,17.1996442316059));
#28205=CARTESIAN_POINT('Ctrl Pts',(19.2865716386092,25.4994131575073,17.3225345039426));
#28206=CARTESIAN_POINT('Ctrl Pts',(19.0728538401323,25.3740784559106,17.4387046858284));
#28207=CARTESIAN_POINT('Ctrl Pts',(18.7028555998037,25.1570931632801,17.6398239336528));
#28208=CARTESIAN_POINT('Ctrl Pts',(18.4144703596238,24.9815167506413,17.8106758656204));
#28209=CARTESIAN_POINT('Ctrl Pts',(18.0642874871542,24.7606238748754,18.0298340093772));
#28210=CARTESIAN_POINT('Ctrl Pts',(17.4420927116724,24.3681478172276,18.4192278454838));
#28211=CARTESIAN_POINT('Ctrl Pts',(16.722456441822,23.8866996305776,18.9163953124274));
#28212=CARTESIAN_POINT('Ctrl Pts',(15.9202806616111,23.2999769887242,19.5075155171573));
#28213=CARTESIAN_POINT('Ctrl Pts',(15.4090529834523,22.9260578785773,19.8842371999004));
#28214=CARTESIAN_POINT('Ctrl Pts',(14.8739602945725,22.5035099772305,20.3065653819873));
#28215=CARTESIAN_POINT('Ctrl Pts',(14.3169794331172,22.0244589523056,20.7640450546171));
#28216=CARTESIAN_POINT('Ctrl Pts',(13.8864206762848,21.6541417151711,21.1176871503417));
#28217=CARTESIAN_POINT('Ctrl Pts',(13.3867890027812,21.2019814327451,21.5394320189419));
#28218=CARTESIAN_POINT('Ctrl Pts',(12.8146824059514,20.6456427149589,22.0238946695559));
#28219=CARTESIAN_POINT('Ctrl Pts',(12.2526665517595,20.0991166279862,22.499812430193));
#28220=CARTESIAN_POINT('Ctrl Pts',(11.6379478462803,19.44703563439,23.0419154065947));
#28221=CARTESIAN_POINT('Ctrl Pts',(10.9739250490308,18.6689137476991,23.6265354530559));
#28222=CARTESIAN_POINT('Ctrl Pts',(10.5683455447963,18.1936434853748,23.9836164291782));
#28223=CARTESIAN_POINT('Ctrl Pts',(10.1437415406956,17.6694303965612,24.3558958755273));
#28224=CARTESIAN_POINT('Ctrl Pts',(9.74137929176525,17.1528053766524,24.6998029803349));
#28225=CARTESIAN_POINT('Ctrl Pts',(8.72285779294234,15.8450442956717,25.5703537856744));
#28226=CARTESIAN_POINT('Ctrl Pts',(7.81323138778194,14.4751178145147,26.3485431508902));
#28227=CARTESIAN_POINT('Ctrl Pts',(6.9,12.9951291628659,27.0393531365015));
#28228=CARTESIAN_POINT('Ctrl Pts',(30.5,31.0562879796886,16.1402285275843));
#28229=CARTESIAN_POINT('Ctrl Pts',(29.9560179420817,30.8470467059701,16.0158030554221));
#28230=CARTESIAN_POINT('Ctrl Pts',(29.4152668325132,30.6299015220344,15.9055856438304));
#28231=CARTESIAN_POINT('Ctrl Pts',(28.8740459957565,30.3967092920472,15.8236145009996));
#28232=CARTESIAN_POINT('Ctrl Pts',(28.353527792344,30.1724370682909,15.7447788961961));
#28233=CARTESIAN_POINT('Ctrl Pts',(27.8179515912467,29.9423746730404,15.65999396651));
#28234=CARTESIAN_POINT('Ctrl Pts',(27.2695051149491,29.6962958928787,15.5981844167478));
#28235=CARTESIAN_POINT('Ctrl Pts',(26.9554553615883,29.5553870101399,15.5627912203338));
#28236=CARTESIAN_POINT('Ctrl Pts',(26.6378099296971,29.4095747645068,15.5350208970661));
#28237=CARTESIAN_POINT('Ctrl Pts',(26.3179304017917,29.2578762499931,15.520523503095));
#28238=CARTESIAN_POINT('Ctrl Pts',(26.1078196745982,29.1582340959378,15.5110009868852));
#28239=CARTESIAN_POINT('Ctrl Pts',(25.8967402232745,29.0560612282453,15.5072071790431));
#28240=CARTESIAN_POINT('Ctrl Pts',(25.6850706236774,28.9510881944939,15.5107635234098));
#28241=CARTESIAN_POINT('Ctrl Pts',(25.6562210027417,28.9367808388889,15.5112482372614));
#28242=CARTESIAN_POINT('Ctrl Pts',(25.6277737638215,28.9226278510966,15.5118582602788));
#28243=CARTESIAN_POINT('Ctrl Pts',(25.5983858063598,28.9079571471847,15.5126342200129));
#28244=CARTESIAN_POINT('Ctrl Pts',(25.1249357452756,28.6716070819486,15.5251351971226));
#28245=CARTESIAN_POINT('Ctrl Pts',(24.1510084067019,28.1678256190434,15.583657222894));
#28246=CARTESIAN_POINT('Ctrl Pts',(22.9245129145126,27.5141512254856,15.8853026165582));
#28247=CARTESIAN_POINT('Origin',(40.65,0.,0.));
#28248=CARTESIAN_POINT('',(40.4,16.1848830792292,31.0330398077868));
#28249=CARTESIAN_POINT('',(40.9,15.9346498339374,30.5996231131986));
#28250=CARTESIAN_POINT('Ctrl Pts',(40.4,16.1848830792292,31.0330398077868));
#28251=CARTESIAN_POINT('Ctrl Pts',(40.5666590127278,16.101476940186,30.8885761373009));
#28252=CARTESIAN_POINT('Ctrl Pts',(40.7333430445956,16.0180571838558,30.7440888809818));
#28253=CARTESIAN_POINT('Ctrl Pts',(40.9,15.9346498339374,30.5996231131986));
#28254=CARTESIAN_POINT('',(40.9,18.5327260452908,29.0996231131986));
#28255=CARTESIAN_POINT('Origin',(40.9,0.,0.));
#28256=CARTESIAN_POINT('',(40.4,18.7829592905825,29.5330398077868));
#28257=CARTESIAN_POINT('Ctrl Pts',(40.9,18.5327260452907,29.0996231131986));
#28258=CARTESIAN_POINT('Ctrl Pts',(40.7333430449886,18.6161333950124,29.2440888806411));
#28259=CARTESIAN_POINT('Ctrl Pts',(40.5666590138314,18.699553150987,29.3885761363442));
#28260=CARTESIAN_POINT('Ctrl Pts',(40.4,18.7829592905825,29.5330398077868));
#28261=CARTESIAN_POINT('Origin',(40.4,0.,0.));
#28262=CARTESIAN_POINT('Origin',(35.7,0.,0.));
#28263=CARTESIAN_POINT('',(30.5,18.8254200738635,29.5059919176187));
#28264=CARTESIAN_POINT('Ctrl Pts',(40.3998805977105,18.7829479019259,29.5330468723878));
#28265=CARTESIAN_POINT('Ctrl Pts',(39.2493532038275,18.7828975281295,29.5330781201994));
#28266=CARTESIAN_POINT('Ctrl Pts',(38.0972325173599,18.7826942098824,29.5332042421555));
#28267=CARTESIAN_POINT('Ctrl Pts',(36.9466403234098,18.782625610211,29.5332467931397));
#28268=CARTESIAN_POINT('Ctrl Pts',(36.745394297411,18.7826136116842,29.5332542355824));
#28269=CARTESIAN_POINT('Ctrl Pts',(36.5441950314761,18.7826057345052,29.5332591213989));
#28270=CARTESIAN_POINT('Ctrl Pts',(36.3429831482489,18.7825981392881,29.5332638326403));
#28271=CARTESIAN_POINT('Ctrl Pts',(36.2103627229667,18.7825931332173,29.5332669378586));
#28272=CARTESIAN_POINT('Ctrl Pts',(36.0823539051257,18.7825884046849,29.5332699079689));
#28273=CARTESIAN_POINT('Ctrl Pts',(35.9587472612939,18.782583031639,29.5332733040083));
#28274=CARTESIAN_POINT('Ctrl Pts',(35.7554552091559,18.7825741947555,29.5332788893702));
#28275=CARTESIAN_POINT('Ctrl Pts',(35.5640774639574,18.7825638026986,29.5332855100023));
#28276=CARTESIAN_POINT('Ctrl Pts',(35.3838244596789,18.7825536728019,29.5332919882553));
#28277=CARTESIAN_POINT('Ctrl Pts',(35.2391029657187,18.7825455397126,29.5332971895137));
#28278=CARTESIAN_POINT('Ctrl Pts',(35.1015509582107,18.7825375448577,29.5333023181014));
#28279=CARTESIAN_POINT('Ctrl Pts',(34.9707359993668,18.7825301857251,29.53330703978));
#28280=CARTESIAN_POINT('Ctrl Pts',(34.8578981782319,18.7825238379151,29.5333111125858));
#28281=CARTESIAN_POINT('Ctrl Pts',(34.7500670454682,18.7825179390022,29.5333148977088));
#28282=CARTESIAN_POINT('Ctrl Pts',(34.6468496336312,18.7825123391989,29.5333184739616));
#28283=CARTESIAN_POINT('Ctrl Pts',(34.5887227637979,18.7825091856706,29.5333204879278));
#28284=CARTESIAN_POINT('Ctrl Pts',(34.5320601650638,18.7825061280823,29.5333224349598));
#28285=CARTESIAN_POINT('Ctrl Pts',(34.4767987085459,18.7825031467929,29.5333243245742));
#28286=CARTESIAN_POINT('Ctrl Pts',(34.3959515551432,18.7824987851858,29.5333270890679));
#28287=CARTESIAN_POINT('Ctrl Pts',(34.3181086379449,18.7824945796072,29.533329735068));
#28288=CARTESIAN_POINT('Ctrl Pts',(34.2432236356779,18.7824903289018,29.5333323757534));
#28289=CARTESIAN_POINT('Ctrl Pts',(34.1622675304667,18.7824857335818,29.5333352305253));
#28290=CARTESIAN_POINT('Ctrl Pts',(34.0847679660317,18.7824810863437,29.5333380785848));
#28291=CARTESIAN_POINT('Ctrl Pts',(34.0106064145688,18.7824762391415,29.533340998409));
#28292=CARTESIAN_POINT('Ctrl Pts',(34.0011740964176,18.7824756226447,29.53334136977));
#28293=CARTESIAN_POINT('Ctrl Pts',(33.9917957065817,18.7824750030335,29.5333417422189));
#28294=CARTESIAN_POINT('Ctrl Pts',(33.9824709442606,18.7824743801028,29.5333421158564));
#28295=CARTESIAN_POINT('Ctrl Pts',(33.9223617768599,18.7824703645751,29.533344524394));
#28296=CARTESIAN_POINT('Ctrl Pts',(33.8644761964479,18.7824662176988,29.5333469783448));
#28297=CARTESIAN_POINT('Ctrl Pts',(33.8085662292048,18.7824621301166,29.5333493560321));
#28298=CARTESIAN_POINT('Ctrl Pts',(33.747423701629,18.7824576599816,29.533351956245));
#28299=CARTESIAN_POINT('Ctrl Pts',(33.6886441629997,18.782453260435,29.5333544654464));
#28300=CARTESIAN_POINT('Ctrl Pts',(33.6319696815839,18.7824490897764,29.5333567795391));
#28301=CARTESIAN_POINT('Ctrl Pts',(33.5826925637838,18.7824454634877,29.5333587915877));
#28302=CARTESIAN_POINT('Ctrl Pts',(33.535008342921,18.7824420082021,29.5333606573655));
#28303=CARTESIAN_POINT('Ctrl Pts',(33.4887791610839,18.7824387840041,29.5333623350385));
#28304=CARTESIAN_POINT('Ctrl Pts',(33.4518540160536,18.7824362087047,29.5333636750648));
#28305=CARTESIAN_POINT('Ctrl Pts',(33.4158630419527,18.7824337707087,29.5333649012377));
#28306=CARTESIAN_POINT('Ctrl Pts',(33.3809178974527,18.7824311830501,29.5333661853037));
#28307=CARTESIAN_POINT('Ctrl Pts',(33.3430135142413,18.7824283762623,29.5333675781075));
#28308=CARTESIAN_POINT('Ctrl Pts',(33.3063394414416,18.7824253936822,29.5333690388471));
#28309=CARTESIAN_POINT('Ctrl Pts',(33.2709744550635,18.7824219844966,29.5333707164935));
#28310=CARTESIAN_POINT('Ctrl Pts',(33.2337091834358,18.7824183921235,29.5333724842856));
#28311=CARTESIAN_POINT('Ctrl Pts',(33.1978968817731,18.7824143271502,29.5333744922618));
#28312=CARTESIAN_POINT('Ctrl Pts',(33.1635680440817,18.7824096073364,29.5333768470679));
#28313=CARTESIAN_POINT('Ctrl Pts',(33.1258517953345,18.7824044217933,29.5333794342353));
#28314=CARTESIAN_POINT('Ctrl Pts',(33.0899258347186,18.7823984465448,29.5333824396031));
#28315=CARTESIAN_POINT('Ctrl Pts',(33.0557653925385,18.7823915567442,29.5333859335397));
#28316=CARTESIAN_POINT('Ctrl Pts',(33.0368719877468,18.7823877461438,29.5333878659608));
#28317=CARTESIAN_POINT('Ctrl Pts',(33.0185175727354,18.7823836577058,29.5333899466652));
#28318=CARTESIAN_POINT('Ctrl Pts',(33.0006913489163,18.7823792820484,29.5333921804186));
#28319=CARTESIAN_POINT('Ctrl Pts',(32.9433364918127,18.7823652036207,29.5333993673924));
#28320=CARTESIAN_POINT('Ctrl Pts',(32.889323201888,18.78254762761,29.5332829792211));
#28321=CARTESIAN_POINT('Ctrl Pts',(32.8382230276383,18.7828441879673,29.5330947066102));
#28322=CARTESIAN_POINT('Ctrl Pts',(32.7810653124614,18.7831759033221,29.5328841156987));
#28323=CARTESIAN_POINT('Ctrl Pts',(32.7275524567343,18.7836507315896,29.5325833908465));
#28324=CARTESIAN_POINT('Ctrl Pts',(32.6770430180207,18.7841988326963,29.532236338609));
#28325=CARTESIAN_POINT('Ctrl Pts',(32.6227203152385,18.7847883132819,29.5318630852917));
#28326=CARTESIAN_POINT('Ctrl Pts',(32.5718714572482,18.785463223046,29.5314358211882));
#28327=CARTESIAN_POINT('Ctrl Pts',(32.5236533105898,18.7861776883227,29.5309832901274));
#28328=CARTESIAN_POINT('Ctrl Pts',(32.4718100172058,18.7869458686764,29.5304967367823));
#28329=CARTESIAN_POINT('Ctrl Pts',(32.4230076638019,18.7877604440451,29.5299805544879));
#28330=CARTESIAN_POINT('Ctrl Pts',(32.3761512174013,18.7885990068259,29.5294487410664));
#28331=CARTESIAN_POINT('Ctrl Pts',(32.3248096593255,18.789517837062,29.5288660223209));
#28332=CARTESIAN_POINT('Ctrl Pts',(32.2758043952282,18.7904660501636,29.5282641699575));
#28333=CARTESIAN_POINT('Ctrl Pts',(32.2276418902258,18.7914438969209,29.5276429421487));
#28334=CARTESIAN_POINT('Ctrl Pts',(32.1780484881801,18.7924507952825,29.5270032578033));
#28335=CARTESIAN_POINT('Ctrl Pts',(32.1293485209749,18.7934898292201,29.5263425802702));
#28336=CARTESIAN_POINT('Ctrl Pts',(32.0798596724235,18.7945806304077,29.525648507911));
#28337=CARTESIAN_POINT('Ctrl Pts',(32.0310319729845,18.7956568589742,29.5249637080513));
#28338=CARTESIAN_POINT('Ctrl Pts',(31.9814363681892,18.7967841298918,29.5242459916461));
#28339=CARTESIAN_POINT('Ctrl Pts',(31.9294088358077,18.7979897030586,29.5234781935337));
#28340=CARTESIAN_POINT('Ctrl Pts',(31.8980169364549,18.7987171108326,29.523014926491));
#28341=CARTESIAN_POINT('Ctrl Pts',(31.8657387727397,18.7994731540541,29.5225333463335));
#28342=CARTESIAN_POINT('Ctrl Pts',(31.8321995512669,18.8002637764333,29.5220297160307));
#28343=CARTESIAN_POINT('Ctrl Pts',(31.7313430764711,18.8026412730643,29.5205152391074));
#28344=CARTESIAN_POINT('Ctrl Pts',(31.6280303047182,18.8051208626313,29.5189339807854));
#28345=CARTESIAN_POINT('Ctrl Pts',(31.5230436279567,18.8075570028382,29.5173797885034));
#28346=CARTESIAN_POINT('Ctrl Pts',(31.4165412786076,18.8100283131358,29.5158031586445));
#28347=CARTESIAN_POINT('Ctrl Pts',(31.3083161729143,18.8124535008248,29.5142552682412));
#28348=CARTESIAN_POINT('Ctrl Pts',(31.1992361814709,18.8146708543331,29.512840201736));
#28349=CARTESIAN_POINT('Ctrl Pts',(31.1417800745717,18.8158388091388,29.5120948385276));
#28350=CARTESIAN_POINT('Ctrl Pts',(31.0840876480107,18.8169490689289,29.5113863465313));
#28351=CARTESIAN_POINT('Ctrl Pts',(31.0262914639722,18.8179790482415,29.5107292749178));
#28352=CARTESIAN_POINT('Ctrl Pts',(30.9238422544136,18.8198047841132,29.5095645532577));
#28353=CARTESIAN_POINT('Ctrl Pts',(30.8210652532058,18.8213763539421,29.5085625948816));
#28354=CARTESIAN_POINT('Ctrl Pts',(30.7187655074561,18.8225556950176,29.507810834769));
#28355=CARTESIAN_POINT('Ctrl Pts',(30.6466529343875,18.82338702963,29.5072809081729));
#28356=CARTESIAN_POINT('Ctrl Pts',(30.5747782907563,18.8240238717387,29.5068750504575));
#28357=CARTESIAN_POINT('Ctrl Pts',(30.5034323951389,18.8244289981691,29.5066169468345));
#28358=CARTESIAN_POINT('Ctrl Pts',(30.5006731185506,18.8244446662866,29.5066069647706));
#28359=CARTESIAN_POINT('Ctrl Pts',(30.497914633606,18.8244599892393,29.5065972028236));
#28360=CARTESIAN_POINT('Ctrl Pts',(30.4951569527683,18.8244749650172,29.5065876622663));
#28361=CARTESIAN_POINT('',(30.5,16.229443021655,31.0097594187194));
#28362=CARTESIAN_POINT('Origin',(30.5,0.,0.));
#28363=CARTESIAN_POINT('Ctrl Pts',(30.5049076308142,16.2304573503027,31.009123868732));
#28364=CARTESIAN_POINT('Ctrl Pts',(30.5973062294347,16.2298682766553,31.0094328533549));
#28365=CARTESIAN_POINT('Ctrl Pts',(30.6890591585862,16.2288427503287,31.009969267703));
#28366=CARTESIAN_POINT('Ctrl Pts',(30.7806364364921,16.2274919709622,31.0106763092386));
#28367=CARTESIAN_POINT('Ctrl Pts',(30.8441456090294,16.2265552005995,31.0111666450937));
#28368=CARTESIAN_POINT('Ctrl Pts',(30.9075713010185,16.2254611740685,31.0117394593185));
#28369=CARTESIAN_POINT('Ctrl Pts',(30.9710816356705,16.2242390174925,31.012379837551));
#28370=CARTESIAN_POINT('Ctrl Pts',(31.0734991469997,16.2222681534488,31.0134125190073));
#28371=CARTESIAN_POINT('Ctrl Pts',(31.1761345288069,16.2199648111637,31.0146205155169));
#28372=CARTESIAN_POINT('Ctrl Pts',(31.2798100568472,16.2174702047239,31.0159286966546));
#28373=CARTESIAN_POINT('Ctrl Pts',(31.3828326297121,16.2149913094767,31.017228638783));
#28374=CARTESIAN_POINT('Ctrl Pts',(31.4868822244314,16.2123218973816,31.0186283615543));
#28375=CARTESIAN_POINT('Ctrl Pts',(31.5928140565566,16.2095937955792,31.0200576696061));
#28376=CARTESIAN_POINT('Ctrl Pts',(31.6516194621086,16.2080793581371,31.0208511142012));
#28377=CARTESIAN_POINT('Ctrl Pts',(31.711005767608,16.2065468518029,31.0216536678952));
#28378=CARTESIAN_POINT('Ctrl Pts',(31.771125977653,16.205020814195,31.0224523036439));
#28379=CARTESIAN_POINT('Ctrl Pts',(31.8409078613428,16.2032495333099,31.023379284885));
#28380=CARTESIAN_POINT('Ctrl Pts',(31.9056298453965,16.2016434584278,31.0242198767435));
#28381=CARTESIAN_POINT('Ctrl Pts',(31.9658749467866,16.2002018139143,31.0249744961548));
#28382=CARTESIAN_POINT('Ctrl Pts',(32.0341046687229,16.198569100183,31.025829129501));
#28383=CARTESIAN_POINT('Ctrl Pts',(32.0965918298942,16.1971462744692,31.0265740158192));
#28384=CARTESIAN_POINT('Ctrl Pts',(32.1542461945015,16.195904238954,31.0272242625031));
#28385=CARTESIAN_POINT('Ctrl Pts',(32.2151665953518,16.1945918439259,31.0279113447198));
#28386=CARTESIAN_POINT('Ctrl Pts',(32.2706916712559,16.1934801514052,31.0284933558529));
#28387=CARTESIAN_POINT('Ctrl Pts',(32.3219582775156,16.1925241206213,31.0289937114783));
#28388=CARTESIAN_POINT('Ctrl Pts',(32.3761916324766,16.1915127652647,31.0295230221977));
#28389=CARTESIAN_POINT('Ctrl Pts',(32.4256599862214,16.1906748064837,31.0299613681538));
#28390=CARTESIAN_POINT('Ctrl Pts',(32.4717693483768,16.1899610544419,31.0303343957025));
#28391=CARTESIAN_POINT('Ctrl Pts',(32.5215332003052,16.1891907325538,31.030736988296));
#28392=CARTESIAN_POINT('Ctrl Pts',(32.5673849287937,16.1885644631732,31.0310638203077));
#28393=CARTESIAN_POINT('Ctrl Pts',(32.6111519417706,16.1880367365759,31.0313387615315));
#28394=CARTESIAN_POINT('Ctrl Pts',(32.655174121074,16.1875059332765,31.0316153056917));
#28395=CARTESIAN_POINT('Ctrl Pts',(32.6970878717828,16.1870745377529,31.0318395012597));
#28396=CARTESIAN_POINT('Ctrl Pts',(32.7388013470518,16.18671857384,31.0320241553174));
#28397=CARTESIAN_POINT('Ctrl Pts',(32.7801521457877,16.1863657048444,31.032207203906));
#28398=CARTESIAN_POINT('Ctrl Pts',(32.8213062770016,16.186086545466,31.0323516104908));
#28399=CARTESIAN_POINT('Ctrl Pts',(32.8641640035295,16.1858844594635,31.0324560971771));
#28400=CARTESIAN_POINT('Ctrl Pts',(32.9038200784534,16.1856974701314,31.0325527782704));
#28401=CARTESIAN_POINT('Ctrl Pts',(32.9449347772907,16.1855761117062,31.0326154655021));
#28402=CARTESIAN_POINT('Ctrl Pts',(32.9890474705827,16.1855509840874,31.0326287580454));
#28403=CARTESIAN_POINT('Ctrl Pts',(32.9926089293378,16.1855489553974,31.032629831225));
#28404=CARTESIAN_POINT('Ctrl Pts',(32.9961899495412,16.1855475722578,31.0326305730129));
#28405=CARTESIAN_POINT('Ctrl Pts',(32.9997913521116,16.185546860962,31.0326309700539));
#28406=CARTESIAN_POINT('Ctrl Pts',(33.0362292496773,16.1855396642873,31.0326349871948));
#28407=CARTESIAN_POINT('Ctrl Pts',(33.0740922921121,16.1855331333215,31.0326386992186));
#28408=CARTESIAN_POINT('Ctrl Pts',(33.1141439185632,16.1855273500632,31.032642249087));
#28409=CARTESIAN_POINT('Ctrl Pts',(33.2461674547435,16.1855082865123,31.0326539506384));
#28410=CARTESIAN_POINT('Ctrl Pts',(33.3721931286569,16.1855003220479,31.0326588963954));
#28411=CARTESIAN_POINT('Ctrl Pts',(33.499387920745,16.185492813855,31.0326635427517));
#28412=CARTESIAN_POINT('Ctrl Pts',(33.6627849160626,16.185483168679,31.0326695115548));
#28413=CARTESIAN_POINT('Ctrl Pts',(33.828111247454,16.1854742764645,31.0326749862724));
#28414=CARTESIAN_POINT('Ctrl Pts',(33.9929845306744,16.1854606405094,31.0326833946006));
#28415=CARTESIAN_POINT('Ctrl Pts',(34.3227310971152,16.1854333685993,31.032700211257));
#28416=CARTESIAN_POINT('Ctrl Pts',(34.650665470872,16.185387121727,31.0327287623561));
#28417=CARTESIAN_POINT('Ctrl Pts',(34.9792693636211,16.1853559472169,31.0327480042371));
#28418=CARTESIAN_POINT('Ctrl Pts',(35.3078732563702,16.1853247727069,31.0327672461181));
#28419=CARTESIAN_POINT('Ctrl Pts',(35.6371466681117,16.185308670559,31.0327771787811));
#28420=CARTESIAN_POINT('Ctrl Pts',(35.9662682695209,16.1852951338217,31.0327855310263));
#28421=CARTESIAN_POINT('Ctrl Pts',(36.2953898709301,16.1852815970843,31.0327938832715));
#28422=CARTESIAN_POINT('Ctrl Pts',(36.624359662007,16.1852706257574,31.0328006550989));
#28423=CARTESIAN_POINT('Ctrl Pts',(36.9532592751493,16.185248102247,31.032814555176));
#28424=CARTESIAN_POINT('Ctrl Pts',(38.1023262780261,16.1851694125147,31.0328631174706));
#28425=CARTESIAN_POINT('Ctrl Pts',(39.2505367075415,16.184949719878,31.0329986853002));
#28426=CARTESIAN_POINT('Ctrl Pts',(40.4000986012038,16.1848953623403,31.0330322281526));
#28427=CARTESIAN_POINT('Ctrl Pts',(6.89999999997365,-0.168526548676479,
11.0276873985587));
#28428=CARTESIAN_POINT('Ctrl Pts',(6.99168932310453,-0.107121039164011,
11.0290491215116));
#28429=CARTESIAN_POINT('Ctrl Pts',(7.08383940291242,-0.0458098125994647,
11.0299018391088));
#28430=CARTESIAN_POINT('Ctrl Pts',(8.15761824498006,0.664186592400573,11.0337651740187));
#28431=CARTESIAN_POINT('Ctrl Pts',(9.166078574375,1.30870352701556,10.9699676285446));
#28432=CARTESIAN_POINT('Ctrl Pts',(11.2535171643192,2.47376106241927,10.7760330567599));
#28433=CARTESIAN_POINT('Ctrl Pts',(12.2576790632369,3.00237606292525,10.6330057282434));
#28434=CARTESIAN_POINT('Ctrl Pts',(14.3563663857894,3.94447005883399,10.3307260661656));
#28435=CARTESIAN_POINT('Ctrl Pts',(15.3658129161116,4.36032593857961,10.1540434041659));
#28436=CARTESIAN_POINT('Ctrl Pts',(17.4727193021212,5.08193366885831,9.82334300624282));
#28437=CARTESIAN_POINT('Ctrl Pts',(18.4888802671461,5.39169279079135,9.64884225911208));
#28438=CARTESIAN_POINT('Ctrl Pts',(19.8473882183425,5.72385817850076,9.45778984314826));
#28439=CARTESIAN_POINT('Ctrl Pts',(20.3451395577183,5.84063156394591,9.38741838105893));
#28440=CARTESIAN_POINT('Ctrl Pts',(21.1198641211409,6.00690103675047,9.28201599203949));
#28441=CARTESIAN_POINT('Ctrl Pts',(21.9116430735678,6.15921075032181,9.18172875488036));
#28442=CARTESIAN_POINT('Ctrl Pts',(22.4533884343746,6.25063668203687,9.12054551137775));
#28443=CARTESIAN_POINT('Ctrl Pts',(22.8546099577479,6.3132089675058,9.07881438233611));
#28444=CARTESIAN_POINT('Ctrl Pts',(23.1058218650381,6.35118260107244,9.05298395410355));
#28445=CARTESIAN_POINT('Ctrl Pts',(23.6175153199788,6.42382403760964,9.00245668094438));
#28446=CARTESIAN_POINT('Ctrl Pts',(24.1364702886545,6.49007583237978,8.95485371029555));
#28447=CARTESIAN_POINT('Ctrl Pts',(24.6629181373247,6.5494442392928,8.91145225308146));
#28448=CARTESIAN_POINT('Ctrl Pts',(25.0606678571037,6.59024788291776,8.88140293076166));
#28449=CARTESIAN_POINT('Ctrl Pts',(25.3945416155883,6.62099228309711,8.85873533710266));
#28450=CARTESIAN_POINT('Ctrl Pts',(25.6627586119465,6.64352323130155,8.84221409068035));
#28451=CARTESIAN_POINT('Ctrl Pts',(25.7972076165426,6.65408072739388,8.83452216013017));
#28452=CARTESIAN_POINT('Ctrl Pts',(26.3824137782947,6.69837697633854,8.80240169886325));
#28453=CARTESIAN_POINT('Ctrl Pts',(27.4369717967155,6.74704662082202,8.76563881905854));
#28454=CARTESIAN_POINT('Ctrl Pts',(28.4593635146676,6.76713562537253,8.74917816753948));
#28455=CARTESIAN_POINT('Ctrl Pts',(29.042748146989,6.7797450529872,8.73952198264541));
#28456=CARTESIAN_POINT('Ctrl Pts',(29.2174939164951,6.7830642423932,8.73701514175015));
#28457=CARTESIAN_POINT('Ctrl Pts',(29.5607048332278,6.78786835107259,8.7333656848919));
#28458=CARTESIAN_POINT('Ctrl Pts',(29.9899637006213,6.79106253935675,8.73093988338426));
#28459=CARTESIAN_POINT('Ctrl Pts',(30.5003627545717,6.79139754852946,8.7306825539187));
#28460=CARTESIAN_POINT('Ctrl Pts',(31.5152290141054,6.78728755019408,8.73381293113857));
#28461=CARTESIAN_POINT('Ctrl Pts',(32.346385618228,6.77838967797265,8.74063107149334));
#28462=CARTESIAN_POINT('Ctrl Pts',(33.1616392309915,6.77840182636605,8.74062146997073));
#28463=CARTESIAN_POINT('Ctrl Pts',(33.4928689770884,6.7784028418104,8.74062052628883));
#28464=CARTESIAN_POINT('Ctrl Pts',(33.9856875201801,6.77840526161274,8.74061852020512));
#28465=CARTESIAN_POINT('Ctrl Pts',(34.479956929609,6.7784068708528,8.74061713883255));
#28466=CARTESIAN_POINT('Ctrl Pts',(35.1382080085716,6.778409075901,8.74061527897129));
#28467=CARTESIAN_POINT('Ctrl Pts',(35.9613703496106,6.7784121544085,8.74061266742265));
#28468=CARTESIAN_POINT('Ctrl Pts',(37.9364530322258,6.77841531264166,8.74060999527038));
#28469=CARTESIAN_POINT('Ctrl Pts',(39.5833333333333,6.77843480602319,8.74059347982545));
#28470=CARTESIAN_POINT('Ctrl Pts',(40.9,6.77843480602319,8.74059347982545));
#28471=CARTESIAN_POINT('Ctrl Pts',(6.71972576838711,-0.727849695365753,
14.4135489955738));
#28472=CARTESIAN_POINT('Ctrl Pts',(6.81144220747046,-0.647520064289724,
14.4181051875223));
#28473=CARTESIAN_POINT('Ctrl Pts',(6.90362846895808,-0.567280569774696,
14.4219897194692));
#28474=CARTESIAN_POINT('Ctrl Pts',(7.97787094717212,0.361837668282342,14.4591555519285));
#28475=CARTESIAN_POINT('Ctrl Pts',(8.98682261267022,1.20743712855002,14.4048184698324));
#28476=CARTESIAN_POINT('Ctrl Pts',(11.0806424583842,2.7442230049829,14.2022941804566));
#28477=CARTESIAN_POINT('Ctrl Pts',(12.0862214600972,3.4422325745447,14.038891127913));
#28478=CARTESIAN_POINT('Ctrl Pts',(14.1975721203649,4.69396502652543,13.6830024292515));
#28479=CARTESIAN_POINT('Ctrl Pts',(15.2099789251839,5.24642829788654,13.4699449244818));
#28480=CARTESIAN_POINT('Ctrl Pts',(17.3362999248755,6.21145869787376,13.0656161985035));
#28481=CARTESIAN_POINT('Ctrl Pts',(18.357013455463,6.62511541331197,12.8502526120859));
#28482=CARTESIAN_POINT('Ctrl Pts',(19.7328409259837,7.07198752003368,12.6121436508471));
#28483=CARTESIAN_POINT('Ctrl Pts',(20.2337632876373,7.2284111452015,12.5247332071257));
#28484=CARTESIAN_POINT('Ctrl Pts',(21.0166345413949,7.45203181169806,12.3929576501156));
#28485=CARTESIAN_POINT('Ctrl Pts',(21.8175391230323,7.65714338227214,12.2672157657621));
#28486=CARTESIAN_POINT('Ctrl Pts',(22.3668263920487,7.7805494741423,12.190248920123));
#28487=CARTESIAN_POINT('Ctrl Pts',(22.7739396967848,7.8650629816421,12.1377120270328));
#28488=CARTESIAN_POINT('Ctrl Pts',(23.0274297041713,7.91615663273499,12.1053188608807));
#28489=CARTESIAN_POINT('Ctrl Pts',(23.5449351393661,8.01409846114017,12.0417665186343));
#28490=CARTESIAN_POINT('Ctrl Pts',(24.0699575659665,8.1034816713378,11.9817953425795));
#28491=CARTESIAN_POINT('Ctrl Pts',(24.6032835407751,8.18369268569516,11.9270075754273));
#28492=CARTESIAN_POINT('Ctrl Pts',(25.0064847905103,8.2388595218387,11.8890391550575));
#28493=CARTESIAN_POINT('Ctrl Pts',(25.3452465270806,8.28045801654028,11.8603696837558));
#28494=CARTESIAN_POINT('Ctrl Pts',(25.6175460563752,8.31095886138246,11.8394640015962));
#28495=CARTESIAN_POINT('Ctrl Pts',(25.7540942648801,8.3252551228897,11.829728241242));
#28496=CARTESIAN_POINT('Ctrl Pts',(26.3487780629201,8.38525559473469,11.7890598714194));
#28497=CARTESIAN_POINT('Ctrl Pts',(27.420647343066,8.4511591136706,11.7424863739248));
#28498=CARTESIAN_POINT('Ctrl Pts',(28.4470245212717,8.47809267828293,11.7218144944205));
#28499=CARTESIAN_POINT('Ctrl Pts',(29.0301431861017,8.49498332574133,11.7097207064843));
#28500=CARTESIAN_POINT('Ctrl Pts',(29.2075511609936,8.49948124637053,11.7065424548688));
#28501=CARTESIAN_POINT('Ctrl Pts',(29.5540559241345,8.50596054299456,11.7019389390663));
#28502=CARTESIAN_POINT('Ctrl Pts',(29.9873899374288,8.51027178683719,11.6988759349841));
#28503=CARTESIAN_POINT('Ctrl Pts',(30.5010585876109,8.51072031244604,11.698553559564));
#28504=CARTESIAN_POINT('Ctrl Pts',(31.520398261889,8.50519297418973,11.7024891534661));
#28505=CARTESIAN_POINT('Ctrl Pts',(32.3504760849347,8.49329404471494,11.7110091605269));
#28506=CARTESIAN_POINT('Ctrl Pts',(33.1607219786944,8.49331406281709,11.7109930603161));
#28507=CARTESIAN_POINT('Ctrl Pts',(33.4925972550183,8.49331574772296,11.7109914601493));
#28508=CARTESIAN_POINT('Ctrl Pts',(33.9851239882619,8.49331974280041,11.7109880844892));
#28509=CARTESIAN_POINT('Ctrl Pts',(34.4795557496198,8.49332240354984,11.7109857543654));
#28510=CARTESIAN_POINT('Ctrl Pts',(35.1377808103951,8.49332604669792,11.7109826209376));
#28511=CARTESIAN_POINT('Ctrl Pts',(35.9610196518539,8.49333113419868,11.7109782193289));
#28512=CARTESIAN_POINT('Ctrl Pts',(37.9361278153251,8.49333635287233,11.7109737164008));
#28513=CARTESIAN_POINT('Ctrl Pts',(39.5833333333333,8.49336856563261,11.7109458830841));
#28514=CARTESIAN_POINT('Ctrl Pts',(40.9,8.49336856563261,11.7109458830841));
#28515=CARTESIAN_POINT('Ctrl Pts',(6.48175880232276,-2.0223358101383,22.3152648782349));
#28516=CARTESIAN_POINT('Ctrl Pts',(6.5727030402579,-1.89877066361229,22.3270401223923));
#28517=CARTESIAN_POINT('Ctrl Pts',(6.66410021308729,-1.77531589258794,22.3377778183098));
#28518=CARTESIAN_POINT('Ctrl Pts',(7.73046719612231,-0.343647388924402,
22.4505948584363));
#28519=CARTESIAN_POINT('Ctrl Pts',(8.73293490974101,0.965853752252133,22.4183684385317));
#28520=CARTESIAN_POINT('Ctrl Pts',(10.8102891123216,3.35126151217316,22.1981640385547));
#28521=CARTESIAN_POINT('Ctrl Pts',(11.8125652928685,4.44249581664875,21.9890905805955));
#28522=CARTESIAN_POINT('Ctrl Pts',(13.9177091187558,6.40690464277104,21.5128074248294));
#28523=CARTESIAN_POINT('Ctrl Pts',(14.9295907318602,7.27826244175742,21.2167997396941));
#28524=CARTESIAN_POINT('Ctrl Pts',(17.0679705254901,8.81262608188775,20.6429560449296));
#28525=CARTESIAN_POINT('Ctrl Pts',(18.0930327325161,9.47115000177602,20.3328482957164));
#28526=CARTESIAN_POINT('Ctrl Pts',(19.493165165493,10.1918150595347,19.9834260609174));
#28527=CARTESIAN_POINT('Ctrl Pts',(19.9989304172551,10.4420751188792,19.8560672526628));
#28528=CARTESIAN_POINT('Ctrl Pts',(20.7948115947079,10.8025573386247,19.6618467626018));
#28529=CARTESIAN_POINT('Ctrl Pts',(21.6117660259797,11.134285926341,19.4754657432765));
#28530=CARTESIAN_POINT('Ctrl Pts',(22.1753497026275,11.3349591405941,19.3605546952356));
#28531=CARTESIAN_POINT('Ctrl Pts',(22.5940479063322,11.47260657239,19.2819382297017));
#28532=CARTESIAN_POINT('Ctrl Pts',(22.8520812047022,11.5550617085391,19.2339198113556));
#28533=CARTESIAN_POINT('Ctrl Pts',(23.3813360719091,11.7138435277865,19.1391573021403));
#28534=CARTESIAN_POINT('Ctrl Pts',(23.9190563543678,11.8589452906513,19.0494991042743));
#28535=CARTESIAN_POINT('Ctrl Pts',(24.4671051082233,11.989559546254,18.9672572385016));
#28536=CARTESIAN_POINT('Ctrl Pts',(24.8821466483762,12.0795190000423,18.9101500634532));
#28537=CARTESIAN_POINT('Ctrl Pts',(25.2317043848842,12.1474851335067,18.8669280179622));
#28538=CARTESIAN_POINT('Ctrl Pts',(25.513095090024,12.1973721681455,18.8353673631032));
#28539=CARTESIAN_POINT('Ctrl Pts',(25.6543465475615,12.2207724172662,18.8206563371688));
#28540=CARTESIAN_POINT('Ctrl Pts',(26.2703768283174,12.3190725812828,18.7591443923488));
#28541=CARTESIAN_POINT('Ctrl Pts',(27.3823409200252,12.4269409232394,18.6887004197342));
#28542=CARTESIAN_POINT('Ctrl Pts',(28.4180912195453,12.4698946357076,18.6581821178487));
#28543=CARTESIAN_POINT('Ctrl Pts',(29.0006188348746,12.4967855079752,18.6404003655932));
#28544=CARTESIAN_POINT('Ctrl Pts',(29.1842244806991,12.5041566301776,18.6355848623939));
#28545=CARTESIAN_POINT('Ctrl Pts',(29.5384110471464,12.5146498740616,18.6286952117012));
#28546=CARTESIAN_POINT('Ctrl Pts',(29.9812601150293,12.5216494975055,18.6240999155071));
#28547=CARTESIAN_POINT('Ctrl Pts',(30.5025631839301,12.5223645690812,18.6236255844565));
#28548=CARTESIAN_POINT('Ctrl Pts',(31.5323495650756,12.5134871029148,18.6294670720537));
#28549=CARTESIAN_POINT('Ctrl Pts',(32.3599484134841,12.4946603930139,18.6419219593216));
#28550=CARTESIAN_POINT('Ctrl Pts',(33.1585258504257,12.4947174829697,18.6418830267369));
#28551=CARTESIAN_POINT('Ctrl Pts',(33.4919095878066,12.4947228565318,18.6418790995137));
#28552=CARTESIAN_POINT('Ctrl Pts',(33.9837592380106,12.4947346270607,18.6418708983646));
#28553=CARTESIAN_POINT('Ctrl Pts',(34.4785726427749,12.4947426563109,18.6418652189505));
#28554=CARTESIAN_POINT('Ctrl Pts',(35.1367406589071,12.4947535178469,18.6418575939256));
#28555=CARTESIAN_POINT('Ctrl Pts',(35.9601632093982,12.4947687456191,18.641846877137));
#28556=CARTESIAN_POINT('Ctrl Pts',(37.9353361278946,12.4947843377882,18.6418359163297));
#28557=CARTESIAN_POINT('Ctrl Pts',(39.5833333333333,12.4948806713879,18.6417681573542));
#28558=CARTESIAN_POINT('Ctrl Pts',(40.9,12.4948806713879,18.6417681573542));
#28559=CARTESIAN_POINT('Ctrl Pts',(6.40644620858992,-3.20016516784476,30.2320800787095));
#28560=CARTESIAN_POINT('Ctrl Pts',(6.49686818484384,-3.03404698664168,30.2503623618083));
#28561=CARTESIAN_POINT('Ctrl Pts',(6.58771890650217,-2.86810360702044,30.2672526113879));
#28562=CARTESIAN_POINT('Ctrl Pts',(7.64885862899863,-0.940991822615552,
30.4476905739237));
#28563=CARTESIAN_POINT('Ctrl Pts',(8.64788707329235,0.826287776604457,30.430792173042));
#28564=CARTESIAN_POINT('Ctrl Pts',(10.707154859542,4.03135720303698,30.1856445659011));
#28565=CARTESIAN_POINT('Ctrl Pts',(11.7059935225822,5.50908116677457,29.9282222211751));
#28566=CARTESIAN_POINT('Ctrl Pts',(13.7894394913649,8.15261547988189,29.3339211293756));
#28567=CARTESIAN_POINT('Ctrl Pts',(14.7965025532944,9.33507154947814,28.9559671306032));
#28568=CARTESIAN_POINT('Ctrl Pts',(16.9150296648081,11.4103698853377,28.2210428396417));
#28569=CARTESIAN_POINT('Ctrl Pts',(17.9356459667172,12.3080290796725,27.8189128366825));
#28570=CARTESIAN_POINT('Ctrl Pts',(19.3316976380886,13.2937048286053,27.3625462801585));
#28571=CARTESIAN_POINT('Ctrl Pts',(19.8372125803626,13.6366910969767,27.1960046691454));
#28572=CARTESIAN_POINT('Ctrl Pts',(20.6335801906183,14.1320040365234,26.9406914971977));
#28573=CARTESIAN_POINT('Ctrl Pts',(21.4537597225929,14.5899345529251,26.6943052661746));
#28574=CARTESIAN_POINT('Ctrl Pts',(22.0223258890083,14.8686659459061,26.5413031957662));
#28575=CARTESIAN_POINT('Ctrl Pts',(22.4461030502075,15.0605640384028,26.436200781156));
#28576=CARTESIAN_POINT('Ctrl Pts',(22.7062608359972,15.1748824403433,26.3723989822776));
#28577=CARTESIAN_POINT('Ctrl Pts',(23.2414929286472,15.3959532265256,26.2458547955408));
#28578=CARTESIAN_POINT('Ctrl Pts',(23.7867279834487,15.5986167246948,26.1256827576298));
#28579=CARTESIAN_POINT('Ctrl Pts',(24.3445890668936,15.7819085569279,26.0148742888258));
#28580=CARTESIAN_POINT('Ctrl Pts',(24.7681394700222,15.9085256074862,25.9376795444546));
#28581=CARTESIAN_POINT('Ctrl Pts',(25.1260106169384,16.0045350828092,25.8790242908719));
#28582=CARTESIAN_POINT('Ctrl Pts',(25.4147345926425,16.0751760807979,25.8360764159908));
#28583=CARTESIAN_POINT('Ctrl Pts',(25.5598889289847,16.1083660281042,25.8160190309821));
#28584=CARTESIAN_POINT('Ctrl Pts',(26.1939339115031,16.2480157393789,25.7320023110876));
#28585=CARTESIAN_POINT('Ctrl Pts',(27.3441597812047,16.4017510524694,25.6354753903564));
#28586=CARTESIAN_POINT('Ctrl Pts',(28.3894038584673,16.4608066876633,25.5950614103761));
#28587=CARTESIAN_POINT('Ctrl Pts',(28.9713246547181,16.4977059168026,25.5715886293348));
#28588=CARTESIAN_POINT('Ctrl Pts',(29.1610585442185,16.5082319208974,25.5649734110424));
#28589=CARTESIAN_POINT('Ctrl Pts',(29.5228882487203,16.5229807852931,25.555658015613));
#28590=CARTESIAN_POINT('Ctrl Pts',(29.9752283100297,16.5328527231063,25.5494240137561));
#28591=CARTESIAN_POINT('Ctrl Pts',(30.5041683224499,16.5338357099673,25.5487969550271));
#28592=CARTESIAN_POINT('Ctrl Pts',(31.5443819697417,16.521500293953,25.5566068476797));
#28593=CARTESIAN_POINT('Ctrl Pts',(32.369479464394,16.4958953935747,25.5729102090687));
#28594=CARTESIAN_POINT('Ctrl Pts',(33.1563754893963,16.4960222658506,25.5728296448089));
#28595=CARTESIAN_POINT('Ctrl Pts',(33.4912658278754,16.4960347835491,25.572821407314));
#28596=CARTESIAN_POINT('Ctrl Pts',(33.9824352992262,16.4960613233721,25.5728043629855));
#28597=CARTESIAN_POINT('Ctrl Pts',(34.4776280283123,16.4960796138348,25.5727925244551));
#28598=CARTESIAN_POINT('Ctrl Pts',(35.1357360035508,16.4961042295225,25.5727766538609));
#28599=CARTESIAN_POINT('Ctrl Pts',(35.9593379975622,16.4961387987433,25.5727543372373));
#28600=CARTESIAN_POINT('Ctrl Pts',(37.9345713338106,16.4961741679457,25.5727315175493));
#28601=CARTESIAN_POINT('Ctrl Pts',(39.5833333333333,16.4963927771432,25.5725904316243));
#28602=CARTESIAN_POINT('Ctrl Pts',(40.9,16.4963927771432,25.5725904316243));
#28603=CARTESIAN_POINT('Ctrl Pts',(6.37427268165564,-3.85496595036638,34.7583359408307));
#28604=CARTESIAN_POINT('Ctrl Pts',(6.46448755772839,-3.664463752464,34.7802475524424));
#28605=CARTESIAN_POINT('Ctrl Pts',(6.55512331969025,-3.47417181608894,34.8005635888992));
#28606=CARTESIAN_POINT('Ctrl Pts',(7.61410548625795,-1.26339052014806,35.0185788676572));
#28607=CARTESIAN_POINT('Ctrl Pts',(8.61145388480625,0.765602457207675,35.0093532870147));
#28608=CARTESIAN_POINT('Ctrl Pts',(10.6635149436019,4.43910992978123,34.747974440135));
#28609=CARTESIAN_POINT('Ctrl Pts',(11.6608017032625,6.13747453196183,34.4619345886989));
#28610=CARTESIAN_POINT('Ctrl Pts',(13.7353542747945,9.16685810272321,33.7990269238398));
#28611=CARTESIAN_POINT('Ctrl Pts',(14.7402715202385,10.5262979552789,33.3736740493576));
#28612=CARTESIAN_POINT('Ctrl Pts',(16.8491677832146,12.9054531131771,32.5473921410153));
#28613=CARTESIAN_POINT('Ctrl Pts',(17.8672809631135,13.938220333161,32.0928860415559));
#28614=CARTESIAN_POINT('Ctrl Pts',(19.2587625104672,15.0707179501981,31.5771798698669));
#28615=CARTESIAN_POINT('Ctrl Pts',(19.7635899403542,15.4658689812883,31.3885503410944));
#28616=CARTESIAN_POINT('Ctrl Pts',(20.5586991602296,16.0362969262866,31.0991569516509));
#28617=CARTESIAN_POINT('Ctrl Pts',(21.3785272493018,16.5645337867929,30.819343278526));
#28618=CARTESIAN_POINT('Ctrl Pts',(21.9479176287994,16.8867906552356,30.6451300260617));
#28619=CARTESIAN_POINT('Ctrl Pts',(22.3729695502115,17.1090467735267,30.5252344400129));
#28620=CARTESIAN_POINT('Ctrl Pts',(22.6337096028248,17.2413581349254,30.45253373981));
#28621=CARTESIAN_POINT('Ctrl Pts',(23.170751986421,17.4975676797996,30.3080867629257));
#28622=CARTESIAN_POINT('Ctrl Pts',(23.7186485394885,17.7328951431605,30.1706268071311));
#28623=CARTESIAN_POINT('Ctrl Pts',(24.2804077704386,17.9462491604951,30.0435395405948));
#28624=CARTESIAN_POINT('Ctrl Pts',(24.7075732751059,18.093896808302,29.9548357769836));
#28625=CARTESIAN_POINT('Ctrl Pts',(25.0692008252976,18.2061112471098,29.8872739715488));
#28626=CARTESIAN_POINT('Ctrl Pts',(25.3613771492326,18.2888047627701,29.8377189043885));
#28627=CARTESIAN_POINT('Ctrl Pts',(25.5084154817281,18.3277015544067,29.8145466170754));
#28628=CARTESIAN_POINT('Ctrl Pts',(26.1512870025444,18.4915385207408,29.7173716879778));
#28629=CARTESIAN_POINT('Ctrl Pts',(27.3223884400173,18.6726738474942,29.6052740416531));
#28630=CARTESIAN_POINT('Ctrl Pts',(28.373139604832,18.7409825767551,29.559177524821));
#28631=CARTESIAN_POINT('Ctrl Pts',(28.9547046473314,18.7836137746098,29.5324480977278));
#28632=CARTESIAN_POINT('Ctrl Pts',(29.1479037067737,18.7960320303041,29.5247529606443));
#28633=CARTESIAN_POINT('Ctrl Pts',(29.514080236792,18.8132921881813,29.51400582112));
#28634=CARTESIAN_POINT('Ctrl Pts',(29.9718311305157,18.8248686377542,29.5067996680496));
#28635=CARTESIAN_POINT('Ctrl Pts',(30.5051365276118,18.8260067178222,29.5060845192011));
#28636=CARTESIAN_POINT('Ctrl Pts',(31.551298475448,18.8116639693828,29.5150383037988));
#28637=CARTESIAN_POINT('Ctrl Pts',(32.3749555043413,18.7822473977007,29.5335081969198));
#28638=CARTESIAN_POINT('Ctrl Pts',(33.1551698865007,18.7824304492383,29.5333957726549));
#28639=CARTESIAN_POINT('Ctrl Pts',(33.4909201969602,18.782448957068,29.5333841560219));
#28640=CARTESIAN_POINT('Ctrl Pts',(33.981699427726,18.7824875453787,29.5333602907362));
#28641=CARTESIAN_POINT('Ctrl Pts',(34.4771077390558,18.7825142819534,29.533343676228));
#28642=CARTESIAN_POINT('Ctrl Pts',(35.1351798881798,18.7825501686284,29.5333214285967));
#28643=CARTESIAN_POINT('Ctrl Pts',(35.958882261465,18.7826006107083,29.5332901329543));
#28644=CARTESIAN_POINT('Ctrl Pts',(37.9341479260215,18.7826521993715,29.5332581373787));
#28645=CARTESIAN_POINT('Ctrl Pts',(39.5833333333333,18.7829711232891,29.5330603026358));
#28646=CARTESIAN_POINT('Ctrl Pts',(40.9,18.7829711232891,29.5330603026358));
#28647=CARTESIAN_POINT('',(40.9,17.7819838375536,27.7992994660114));
#28648=CARTESIAN_POINT('Ctrl Pts',(40.9,17.7819838375536,27.7992994660114));
#28649=CARTESIAN_POINT('Ctrl Pts',(40.9,18.0322312401327,28.2327406817405));
#28650=CARTESIAN_POINT('Ctrl Pts',(40.9,18.2824786427117,28.6661818974695));
#28651=CARTESIAN_POINT('Ctrl Pts',(40.9,18.5327260452908,29.0996231131986));
#28652=CARTESIAN_POINT('',(38.,17.7819838375536,27.7992994660114));
#28653=CARTESIAN_POINT('Ctrl Pts',(38.,17.7819838375536,27.7992994660114));
#28654=CARTESIAN_POINT('Ctrl Pts',(38.9666666666667,17.7819838375536,27.7992994660114));
#28655=CARTESIAN_POINT('Ctrl Pts',(39.9333333333333,17.7819838375536,27.7992994660114));
#28656=CARTESIAN_POINT('Ctrl Pts',(40.9,17.7819838375536,27.7992994660114));
#28657=CARTESIAN_POINT('Ctrl Pts',(37.4972421947179,17.4814252073799,27.2792895089189));
#28658=CARTESIAN_POINT('Ctrl Pts',(37.6643036200225,17.5817077438357,27.4529624980705));
#28659=CARTESIAN_POINT('Ctrl Pts',(37.8311445342373,17.6818443698597,27.6263779214721));
#28660=CARTESIAN_POINT('Ctrl Pts',(37.9976555467136,17.7817739539416,27.7994312893194));
#28661=CARTESIAN_POINT('',(6.9,-2.26556458774885,29.9143312995417));
#28662=CARTESIAN_POINT('Ctrl Pts',(6.9,-2.26556458774884,29.9143312995417));
#28663=CARTESIAN_POINT('Ctrl Pts',(6.9,-2.00382962437803,27.3056186709172));
#28664=CARTESIAN_POINT('Ctrl Pts',(6.90000000000115,-1.73285728374609,24.6693701926632));
#28665=CARTESIAN_POINT('Ctrl Pts',(6.90000000000115,-1.09593289590079,18.7182130985667));
#28666=CARTESIAN_POINT('Ctrl Pts',(6.9,-0.654794893503693,14.7845781982083));
#28667=CARTESIAN_POINT('Ctrl Pts',(6.9,-0.168526548660249,11.02768739857));
#28668=CARTESIAN_POINT('',(22.9245129145126,15.8853026165582,27.5141512254856));
#28669=CARTESIAN_POINT('Ctrl Pts',(22.9245129145126,15.8853026165582,27.5141512254856));
#28670=CARTESIAN_POINT('Ctrl Pts',(22.7202811020963,15.7659233420327,27.5032269692373));
#28671=CARTESIAN_POINT('Ctrl Pts',(22.5089075447093,15.6398559109135,27.4959054260063));
#28672=CARTESIAN_POINT('Ctrl Pts',(22.2913349439917,15.5073965833875,27.4928730439354));
#28673=CARTESIAN_POINT('Ctrl Pts',(21.4451770585292,14.9922512750189,27.4810798586143));
#28674=CARTESIAN_POINT('Ctrl Pts',(20.5220951556666,14.3509960808545,27.5650257717264));
#28675=CARTESIAN_POINT('Ctrl Pts',(19.7671428819537,13.7859304181012,27.6762399607749));
#28676=CARTESIAN_POINT('Ctrl Pts',(19.519477305839,13.6005580206911,27.7127242885422));
#28677=CARTESIAN_POINT('Ctrl Pts',(19.286571638609,13.421872324025,27.7514615171004));
#28678=CARTESIAN_POINT('Ctrl Pts',(19.0728538401323,13.2552441975238,27.7894004949774));
#28679=CARTESIAN_POINT('Ctrl Pts',(18.7028555998035,12.9667697979459,27.8550822264681));
#28680=CARTESIAN_POINT('Ctrl Pts',(18.4144703596235,12.7292901983115,27.9152561335183));
#28681=CARTESIAN_POINT('Ctrl Pts',(18.0642874871537,12.4284122845046,27.9946062155751));
#28682=CARTESIAN_POINT('Ctrl Pts',(17.4420927116721,11.8938211301512,28.1355931408966));
#28683=CARTESIAN_POINT('Ctrl Pts',(16.7224564418218,11.2282910364347,28.3254287038798));
#28684=CARTESIAN_POINT('Ctrl Pts',(15.9202806616111,10.4246142212493,28.5439924969395));
#28685=CARTESIAN_POINT('Ctrl Pts',(15.409052983451,9.91242993152873,28.6832834892783));
#28686=CARTESIAN_POINT('Ctrl Pts',(14.8739602945697,9.33532862360144,28.8377564730268));
#28687=CARTESIAN_POINT('Ctrl Pts',(14.3169794331127,8.69171842999057,28.9944199787771));
#28688=CARTESIAN_POINT('Ctrl Pts',(13.8864206762817,8.19419324731197,29.1155243989544));
#28689=CARTESIAN_POINT('Ctrl Pts',(13.3867890027792,7.59173852184979,29.2546860278647));
#28690=CARTESIAN_POINT('Ctrl Pts',(12.8146824059514,6.86770373383357,29.3960736315876));
#28691=CARTESIAN_POINT('Ctrl Pts',(12.2526665517594,6.15643937836573,29.5349674589251));
#28692=CARTESIAN_POINT('Ctrl Pts',(11.6379478462802,5.32066918438549,29.678401911158));
#28693=CARTESIAN_POINT('Ctrl Pts',(10.9739250490306,4.35448584003976,29.7956367796097));
#28694=CARTESIAN_POINT('Ctrl Pts',(10.5683455447962,3.76434923114256,29.8672428449776));
#28695=CARTESIAN_POINT('Ctrl Pts',(10.1437415406955,3.12422765605926,29.9275397584159));
#28696=CARTESIAN_POINT('Ctrl Pts',(9.74137929176525,2.50486371218384,29.9670595377668));
#28697=CARTESIAN_POINT('Ctrl Pts',(8.72285779294234,0.937033991304201,30.0670981099855));
#28698=CARTESIAN_POINT('Ctrl Pts',(7.81323138778195,-0.63845182530268,30.0560666286387));
#28699=CARTESIAN_POINT('Ctrl Pts',(6.9,-2.26556458774884,29.9143312995417));
#28700=CARTESIAN_POINT('Ctrl Pts',(30.5,18.8254200738635,29.5059919176187));
#28701=CARTESIAN_POINT('Ctrl Pts',(29.9560179420816,18.7064245513841,29.293615660989));
#28702=CARTESIAN_POINT('Ctrl Pts',(29.4152668325132,18.5734800115823,29.0895919906434));
#28703=CARTESIAN_POINT('Ctrl Pts',(28.8740459957565,18.4125151878636,28.9020067835811));
#28704=CARTESIAN_POINT('Ctrl Pts',(28.353527792344,18.2577075471291,28.7215970352204));
#28705=CARTESIAN_POINT('Ctrl Pts',(27.8179515912466,18.1008601332297,28.5331399346289));
#28706=CARTESIAN_POINT('Ctrl Pts',(27.2695051149491,17.9186544331585,28.3565719042575));
#28707=CARTESIAN_POINT('Ctrl Pts',(26.9554553615883,17.8143203592948,28.2554660556725));
#28708=CARTESIAN_POINT('Ctrl Pts',(26.637809929697,17.7019284120276,28.1585101274348));
#28709=CARTESIAN_POINT('Ctrl Pts',(26.3179304017917,17.5778023417279,28.0701057587103));
#28710=CARTESIAN_POINT('Ctrl Pts',(26.1078196745982,17.4962709631331,28.012037940737));
#28711=CARTESIAN_POINT('Ctrl Pts',(25.8967402232745,17.409683568055,27.9576659729224));
#28712=CARTESIAN_POINT('Ctrl Pts',(25.6850706236774,17.3169960819306,27.9082593406129));
#28713=CARTESIAN_POINT('Ctrl Pts',(25.6562210027417,17.3043631915899,27.9015254373195));
#28714=CARTESIAN_POINT('Ctrl Pts',(25.6277737638215,17.2918013331136,27.8949772388532));
#28715=CARTESIAN_POINT('Ctrl Pts',(25.5983858063598,17.2787081509674,27.8883138877393));
#28716=CARTESIAN_POINT('Ctrl Pts',(25.1249357452756,17.067772501732,27.7809650188704));
#28717=CARTESIAN_POINT('Ctrl Pts',(24.1510084067019,16.6022239440147,27.5797558484168));
#28718=CARTESIAN_POINT('Ctrl Pts',(22.9245129145126,15.8853026165582,27.5141512254856));
#28719=CARTESIAN_POINT('Origin',(40.65,0.,0.));
#28720=CARTESIAN_POINT('',(40.4,-1.5,34.9678423698117));
#28721=CARTESIAN_POINT('',(40.9,-1.5,34.4673758792282));
#28722=CARTESIAN_POINT('Ctrl Pts',(40.4,-1.5,34.9678423698117));
#28723=CARTESIAN_POINT('Ctrl Pts',(40.5666590135434,-1.5,34.801030090909));
#28724=CARTESIAN_POINT('Ctrl Pts',(40.7333430449885,-1.5,34.6341905786716));
#28725=CARTESIAN_POINT('Ctrl Pts',(40.9,-1.5,34.4673758792282));
#28726=CARTESIAN_POINT('',(40.9,1.50000000000002,34.4673758792282));
#28727=CARTESIAN_POINT('Origin',(40.9,0.,0.));
#28728=CARTESIAN_POINT('',(40.4,1.5,34.9678423698117));
#28729=CARTESIAN_POINT('Ctrl Pts',(40.9,1.5,34.4673758792282));
#28730=CARTESIAN_POINT('Ctrl Pts',(40.7333430449643,1.5,34.6341905786958));
#28731=CARTESIAN_POINT('Ctrl Pts',(40.566659013779,1.5,34.8010300906732));
#28732=CARTESIAN_POINT('Ctrl Pts',(40.4,1.5,34.9678423698117));
#28733=CARTESIAN_POINT('Origin',(40.4,0.,0.));
#28734=CARTESIAN_POINT('Origin',(35.7,0.,0.));
#28735=CARTESIAN_POINT('',(30.5,1.55029606206997,34.9656486014478));
#28736=CARTESIAN_POINT('Ctrl Pts',(40.3999921398529,1.49999538724755,34.9678423429768));
#28737=CARTESIAN_POINT('Ctrl Pts',(39.2499570215113,1.49997501500716,34.9678422244593));
#28738=CARTESIAN_POINT('Ctrl Pts',(38.0998114916604,1.49989311899335,34.9678417480135));
#28739=CARTESIAN_POINT('Ctrl Pts',(36.9497038557168,1.49987059349837,34.9678416168427));
#28740=CARTESIAN_POINT('Ctrl Pts',(36.785105117964,1.49986736974093,34.96784159807));
#28741=CARTESIAN_POINT('Ctrl Pts',(36.6205071563607,1.49986536202073,34.9678415863694));
#28742=CARTESIAN_POINT('Ctrl Pts',(36.4559233022361,1.49986268095531,34.9678415707796));
#28743=CARTESIAN_POINT('Ctrl Pts',(36.4193640724435,1.4998620854067,34.9678415673166));
#28744=CARTESIAN_POINT('Ctrl Pts',(36.3828055387466,1.49986145663366,34.9678415636617));
#28745=CARTESIAN_POINT('Ctrl Pts',(36.3462474593958,1.49986080263033,34.967841559861));
#28746=CARTESIAN_POINT('Ctrl Pts',(36.0895450699579,1.49985621036995,34.967841533173));
#28747=CARTESIAN_POINT('Ctrl Pts',(35.8501671305851,1.49985084735668,34.9678416196704));
#28748=CARTESIAN_POINT('Ctrl Pts',(35.6266230092018,1.49984692867086,34.9678417642539));
#28749=CARTESIAN_POINT('Ctrl Pts',(35.5729810992077,1.49984598833841,34.9678417989483));
#28750=CARTESIAN_POINT('Ctrl Pts',(35.5202511626857,1.49984512300934,34.9678418369404));
#28751=CARTESIAN_POINT('Ctrl Pts',(35.4684130151836,1.4998443492858,34.9678418773881));
#28752=CARTESIAN_POINT('Ctrl Pts',(35.3128073279263,1.49984202675329,34.9678419988026));
#28753=CARTESIAN_POINT('Ctrl Pts',(35.1652418679138,1.49984027810624,34.9678421408902));
#28754=CARTESIAN_POINT('Ctrl Pts',(35.0252627275547,1.49983493809963,34.967842254217));
#28755=CARTESIAN_POINT('Ctrl Pts',(35.0082618963838,1.49983428954192,34.9678422679808));
#28756=CARTESIAN_POINT('Ctrl Pts',(34.9913729068342,1.49983359135557,34.9678422813397));
#28757=CARTESIAN_POINT('Ctrl Pts',(34.9745948969331,1.49983283870325,34.9678422942204));
#28758=CARTESIAN_POINT('Ctrl Pts',(34.8399133402553,1.49982679696251,34.9678423976168));
#28759=CARTESIAN_POINT('Ctrl Pts',(34.7123780512931,1.49981743040037,34.9678424712592));
#28760=CARTESIAN_POINT('Ctrl Pts',(34.591404591981,1.49980840280397,34.9678425127827));
#28761=CARTESIAN_POINT('Ctrl Pts',(34.4539348326462,1.49979814417772,34.9678425599684));
#28762=CARTESIAN_POINT('Ctrl Pts',(34.3249390274086,1.49978830616204,34.9678425655798));
#28763=CARTESIAN_POINT('Ctrl Pts',(34.203631264615,1.49978156609768,34.9678425105859));
#28764=CARTESIAN_POINT('Ctrl Pts',(34.1284740534057,1.49977739023598,34.967842476514));
#28765=CARTESIAN_POINT('Ctrl Pts',(34.0562692606601,1.49977435262848,34.9678424188851));
#28766=CARTESIAN_POINT('Ctrl Pts',(33.9868395791739,1.49977272195139,34.9678423310509));
#28767=CARTESIAN_POINT('Ctrl Pts',(33.944569913827,1.49977172917462,34.9678422775764));
#28768=CARTESIAN_POINT('Ctrl Pts',(33.903332682828,1.49977122168105,34.9678422127028));
#28769=CARTESIAN_POINT('Ctrl Pts',(33.8632274501546,1.49977004757329,34.9678421281365));
#28770=CARTESIAN_POINT('Ctrl Pts',(33.8167531035319,1.49976868700542,34.9678420301403));
#28771=CARTESIAN_POINT('Ctrl Pts',(33.771789463122,1.49976648823776,34.9678419060139));
#28772=CARTESIAN_POINT('Ctrl Pts',(33.7281109635882,1.49976414064438,34.9678417565821));
#28773=CARTESIAN_POINT('Ctrl Pts',(33.6812712011832,1.49976162314223,34.9678415963351));
#28774=CARTESIAN_POINT('Ctrl Pts',(33.6359095723891,1.49975893360226,34.9678414069824));
#28775=CARTESIAN_POINT('Ctrl Pts',(33.591810246565,1.49975667024847,34.9678411881909));
#28776=CARTESIAN_POINT('Ctrl Pts',(33.5583448079856,1.4997549526683,34.9678410221577));
#28777=CARTESIAN_POINT('Ctrl Pts',(33.5256076932742,1.49975347489115,34.9678408391413));
#28778=CARTESIAN_POINT('Ctrl Pts',(33.4935243452377,1.49975241817239,34.9678406385663));
#28779=CARTESIAN_POINT('Ctrl Pts',(33.4574180647961,1.49975122895162,34.9678404128412));
#28780=CARTESIAN_POINT('Ctrl Pts',(33.4221459355308,1.49975055002974,34.9678401647559));
#28781=CARTESIAN_POINT('Ctrl Pts',(33.3878318916215,1.49974977143672,34.9678398888653));
#28782=CARTESIAN_POINT('Ctrl Pts',(33.3506903036195,1.49974892868613,34.9678395902407));
#28783=CARTESIAN_POINT('Ctrl Pts',(33.3146710708563,1.49974796966079,34.9678392590421));
#28784=CARTESIAN_POINT('Ctrl Pts',(33.2798677329257,1.49974635090117,34.967838889585));
#28785=CARTESIAN_POINT('Ctrl Pts',(33.2432742079925,1.49974464887706,34.9678385011241));
#28786=CARTESIAN_POINT('Ctrl Pts',(33.2080243245406,1.49974221953694,34.9678380703783));
#28787=CARTESIAN_POINT('Ctrl Pts',(33.1741651388244,1.49973865377071,34.9678375919209));
#28788=CARTESIAN_POINT('Ctrl Pts',(33.137063146823,1.49973474649923,34.96783706764));
#28789=CARTESIAN_POINT('Ctrl Pts',(33.1016306515623,1.49972947597288,34.9678364860775));
#28790=CARTESIAN_POINT('Ctrl Pts',(33.0678641021079,1.49972253958675,34.967835841343));
#28791=CARTESIAN_POINT('Ctrl Pts',(33.0456526984032,1.49971797687971,34.967835417241));
#28792=CARTESIAN_POINT('Ctrl Pts',(33.0241607955796,1.49971269819094,34.9678349658306));
#28793=CARTESIAN_POINT('Ctrl Pts',(33.0033754048768,1.49970666036489,34.9678344856631));
#28794=CARTESIAN_POINT('Ctrl Pts',(32.9442530209621,1.49968948625086,34.9678331198648));
#28795=CARTESIAN_POINT('Ctrl Pts',(32.8887085075052,1.49991335207053,34.9678225692835));
#28796=CARTESIAN_POINT('Ctrl Pts',(32.8362583193005,1.50027559162313,34.9678066670084));
#28797=CARTESIAN_POINT('Ctrl Pts',(32.7773090712613,1.50068271598182,34.9677887942955));
#28798=CARTESIAN_POINT('Ctrl Pts',(32.7222687069613,1.50126502290935,34.9677641462319));
#28799=CARTESIAN_POINT('Ctrl Pts',(32.6704155259709,1.50193537623736,34.9677359487883));
#28800=CARTESIAN_POINT('Ctrl Pts',(32.6144302418904,1.50265914902788,34.9677055043322));
#28801=CARTESIAN_POINT('Ctrl Pts',(32.5621602746537,1.50348644308882,34.967670888482));
#28802=CARTESIAN_POINT('Ctrl Pts',(32.512657574146,1.50436077830379,34.9676341575402));
#28803=CARTESIAN_POINT('Ctrl Pts',(32.4592478825331,1.50530412025725,34.967594527616));
#28804=CARTESIAN_POINT('Ctrl Pts',(32.4090594121698,1.50630310623457,34.9675524017484));
#28805=CARTESIAN_POINT('Ctrl Pts',(32.360858415177,1.50733170420882,34.9675086790575));
#28806=CARTESIAN_POINT('Ctrl Pts',(32.308062438401,1.50845835797427,34.9674607883018));
#28807=CARTESIAN_POINT('Ctrl Pts',(32.2576510584091,1.50962133088219,34.9674109512874));
#28808=CARTESIAN_POINT('Ctrl Pts',(32.2079531230108,1.51082436306576,34.9673589385144));
#28809=CARTESIAN_POINT('Ctrl Pts',(32.1569814991429,1.51205822727904,34.9673055927269));
#28810=CARTESIAN_POINT('Ctrl Pts',(32.1067603493739,1.51333518230827,34.9672499217566));
#28811=CARTESIAN_POINT('Ctrl Pts',(32.0554367657612,1.5146830381351,34.9671908102209));
#28812=CARTESIAN_POINT('Ctrl Pts',(32.0053752916488,1.5159977485437,34.9671331523098));
#28813=CARTESIAN_POINT('Ctrl Pts',(31.954265075229,1.51738077462808,34.9670721879268));
#28814=CARTESIAN_POINT('Ctrl Pts',(31.9003392718766,1.51886693662993,34.9670065776396));
#28815=CARTESIAN_POINT('Ctrl Pts',(31.8778362033475,1.51948710736998,34.9669791986726));
#28816=CARTESIAN_POINT('Ctrl Pts',(31.8548422465641,1.52012527669197,34.9669510097079));
#28817=CARTESIAN_POINT('Ctrl Pts',(31.8312262657831,1.52078388908931,34.9669219190816));
#28818=CARTESIAN_POINT('Ctrl Pts',(31.7273802318769,1.52367999092728,34.9667939995094));
#28819=CARTESIAN_POINT('Ctrl Pts',(31.6210019634565,1.52670831990391,34.9666588880294));
#28820=CARTESIAN_POINT('Ctrl Pts',(31.5129311113833,1.52968152042074,34.9665259706005));
#28821=CARTESIAN_POINT('Ctrl Pts',(31.4048670765162,1.53265453338541,34.9663930615562));
#28822=CARTESIAN_POINT('Ctrl Pts',(31.2951103968296,1.53557057541605,34.9662624173991));
#28823=CARTESIAN_POINT('Ctrl Pts',(31.1845493642875,1.5382305606769,34.9661438310284));
#28824=CARTESIAN_POINT('Ctrl Pts',(31.1321570104782,1.53949106707513,34.9660876356498));
#28825=CARTESIAN_POINT('Ctrl Pts',(31.0795847658975,1.54069407696176,34.9660341471942));
#28826=CARTESIAN_POINT('Ctrl Pts',(31.0269312050905,1.54181935957432,34.9659843676727));
#28827=CARTESIAN_POINT('Ctrl Pts',(30.9325025960689,1.5438374352796,34.9658950933502));
#28828=CARTESIAN_POINT('Ctrl Pts',(30.8378102330027,1.54560383003055,34.9658178028119));
#28829=CARTESIAN_POINT('Ctrl Pts',(30.7433599242841,1.54697518213503,34.9657577677723));
#28830=CARTESIAN_POINT('Ctrl Pts',(30.6608249248197,1.54817353232302,34.965705306409));
#28831=CARTESIAN_POINT('Ctrl Pts',(30.5784749808876,1.5490700665616,34.9656660234083));
#28832=CARTESIAN_POINT('Ctrl Pts',(30.4966730088978,1.54959005157024,34.9656427667437));
#28833=CARTESIAN_POINT('',(30.5,-1.44976976333441,34.9699609326822));
#28834=CARTESIAN_POINT('Origin',(30.5,0.,0.));
#28835=CARTESIAN_POINT('Ctrl Pts',(30.5054746968959,-1.44895568092928,34.9699078679682));
#28836=CARTESIAN_POINT('Ctrl Pts',(30.6033610779518,-1.44967958189436,34.9698794984549));
#28837=CARTESIAN_POINT('Ctrl Pts',(30.700368212004,-1.45097025371839,34.9698271758096));
#28838=CARTESIAN_POINT('Ctrl Pts',(30.7972404545925,-1.4526642529085,34.9697584928139));
#28839=CARTESIAN_POINT('Ctrl Pts',(30.8547901090085,-1.45367062031951,34.9697176897669));
#28840=CARTESIAN_POINT('Ctrl Pts',(30.912292559737,-1.45482036974536,34.9696710570157));
#28841=CARTESIAN_POINT('Ctrl Pts',(30.9699089182993,-1.45608616697457,34.9696198221059));
#28842=CARTESIAN_POINT('Ctrl Pts',(31.0689868417091,-1.45826285019539,34.9695317178142));
#28843=CARTESIAN_POINT('Ctrl Pts',(31.1683984987081,-1.4607818754806,34.969430038865));
#28844=CARTESIAN_POINT('Ctrl Pts',(31.2688593849665,-1.46350004288006,34.9693198609858));
#28845=CARTESIAN_POINT('Ctrl Pts',(31.3714336749603,-1.46627539258549,34.9692073652856));
#28846=CARTESIAN_POINT('Ctrl Pts',(31.47510187112,-1.4692600451563,34.9690859279462));
#28847=CARTESIAN_POINT('Ctrl Pts',(31.580677770035,-1.47230911796257,34.9689606163935));
#28848=CARTESIAN_POINT('Ctrl Pts',(31.6429045255873,-1.47410625073745,34.9688867573836));
#28849=CARTESIAN_POINT('Ctrl Pts',(31.705794981891,-1.47592578560654,34.9688115519007));
#28850=CARTESIAN_POINT('Ctrl Pts',(31.7695239145147,-1.477735460163,34.9687361665656));
#28851=CARTESIAN_POINT('Ctrl Pts',(31.8371287126756,-1.47965519548713,34.968656196446));
#28852=CARTESIAN_POINT('Ctrl Pts',(31.9000064968246,-1.48140024645571,34.9685834938761));
#28853=CARTESIAN_POINT('Ctrl Pts',(31.9586732749497,-1.48297195975084,34.968518055841));
#28854=CARTESIAN_POINT('Ctrl Pts',(32.0221536851646,-1.48467263273653,34.9684472485894));
#28855=CARTESIAN_POINT('Ctrl Pts',(32.0807039557236,-1.48617132572194,34.968384900435));
#28856=CARTESIAN_POINT('Ctrl Pts',(32.1350336259587,-1.48749336426716,34.9683299017682));
#28857=CARTESIAN_POINT('Ctrl Pts',(32.1957172192665,-1.48897001687831,34.9682684709384));
#28858=CARTESIAN_POINT('Ctrl Pts',(32.2511353794558,-1.49022726489916,34.9682161618562));
#28859=CARTESIAN_POINT('Ctrl Pts',(32.3023412619544,-1.49131215660691,34.9681708970554));
#28860=CARTESIAN_POINT('Ctrl Pts',(32.3570408527793,-1.49247106901321,34.9681225438983));
#28861=CARTESIAN_POINT('Ctrl Pts',(32.4069344452281,-1.49343418875215,34.9680821868754));
#28862=CARTESIAN_POINT('Ctrl Pts',(32.4533681563833,-1.49425570426041,34.9680474782494));
#28863=CARTESIAN_POINT('Ctrl Pts',(32.5026204371887,-1.49512708652756,34.9680106627774));
#28864=CARTESIAN_POINT('Ctrl Pts',(32.5479807574602,-1.49583975877307,34.9679801734415));
#28865=CARTESIAN_POINT('Ctrl Pts',(32.5911118987537,-1.4964428881441,34.9679539828988));
#28866=CARTESIAN_POINT('Ctrl Pts',(32.636353739081,-1.49707553272253,34.9679265106753));
#28867=CARTESIAN_POINT('Ctrl Pts',(32.6791434072979,-1.49758813414905,34.9679037453221));
#28868=CARTESIAN_POINT('Ctrl Pts',(32.721449867613,-1.4980125210104,34.9678845705529));
#28869=CARTESIAN_POINT('Ctrl Pts',(32.7634085003555,-1.49843341872493,34.9678655534314));
#28870=CARTESIAN_POINT('Ctrl Pts',(32.804892182072,-1.498767980885,34.9678500473991));
#28871=CARTESIAN_POINT('Ctrl Pts',(32.8478623301446,-1.49901713688919,34.9678384322062));
#28872=CARTESIAN_POINT('Ctrl Pts',(32.8880980033236,-1.49925043744794,34.9678275561649));
#28873=CARTESIAN_POINT('Ctrl Pts',(32.9296371024713,-1.4994093100348,34.9678200697633));
#28874=CARTESIAN_POINT('Ctrl Pts',(32.974122177228,-1.49946218333186,34.9678178555004));
#28875=CARTESIAN_POINT('Ctrl Pts',(32.9824896509787,-1.49947212859839,34.967817439006));
#28876=CARTESIAN_POINT('Ctrl Pts',(32.9909614502058,-1.49947821255296,34.9678172144271));
#28877=CARTESIAN_POINT('Ctrl Pts',(32.9995486448024,-1.49948005835563,34.967817202377));
#28878=CARTESIAN_POINT('Ctrl Pts',(33.0359672905901,-1.49948788648071,34.9678171512721));
#28879=CARTESIAN_POINT('Ctrl Pts',(33.0738131854325,-1.49949485271612,34.9678171646432));
#28880=CARTESIAN_POINT('Ctrl Pts',(33.113850191809,-1.49950094200878,34.9678174069563));
#28881=CARTESIAN_POINT('Ctrl Pts',(33.2458255353411,-1.49952101435093,34.9678182057012));
#28882=CARTESIAN_POINT('Ctrl Pts',(33.3718416807702,-1.49952700620476,34.9678186096024));
#28883=CARTESIAN_POINT('Ctrl Pts',(33.4990450828556,-1.49953291477053,34.9678189489946));
#28884=CARTESIAN_POINT('Ctrl Pts',(33.6624531387496,-1.49954050503329,34.9678193849847));
#28885=CARTESIAN_POINT('Ctrl Pts',(33.8278204637282,-1.49954795785001,34.9678197145189));
#28886=CARTESIAN_POINT('Ctrl Pts',(33.9926680821625,-1.4995605226248,34.9678203238631));
#28887=CARTESIAN_POINT('Ctrl Pts',(34.322363319031,-1.49958565217439,34.9678215425514));
#28888=CARTESIAN_POINT('Ctrl Pts',(34.649979729722,-1.49963122955625,34.9678238804795));
#28889=CARTESIAN_POINT('Ctrl Pts',(34.9787365315426,-1.49965028313962,34.9678248457331));
#28890=CARTESIAN_POINT('Ctrl Pts',(35.1431149324529,-1.49965980993131,34.9678253283599));
#28891=CARTESIAN_POINT('Ctrl Pts',(35.3077784311456,-1.49966270577337,34.9678254678181));
#28892=CARTESIAN_POINT('Ctrl Pts',(35.4723805288558,-1.4996670374846,34.9678256815692));
#28893=CARTESIAN_POINT('Ctrl Pts',(35.9661868219866,-1.49968003261829,34.9678263228224));
#28894=CARTESIAN_POINT('Ctrl Pts',(36.4594405062758,-1.49970595057452,34.9678276327118));
#28895=CARTESIAN_POINT('Ctrl Pts',(36.9526906817966,-1.49974153069046,34.9678294216938));
#28896=CARTESIAN_POINT('Ctrl Pts',(38.1015265336426,-1.4998244008339,34.9678335884367));
#28897=CARTESIAN_POINT('Ctrl Pts',(39.2503433512219,-1.49995968598758,34.9678403541474));
#28898=CARTESIAN_POINT('Ctrl Pts',(40.4000624645996,-1.4999926075592,34.9678420002216));
#28899=CARTESIAN_POINT('Ctrl Pts',(6.89999999997365,-5.65979197164529,9.46599415780712));
#28900=CARTESIAN_POINT('Ctrl Pts',(6.99168932310453,-5.60729410195165,9.49787619923353));
#28901=CARTESIAN_POINT('Ctrl Pts',(7.08405956072215,-5.55450818731572,9.52934434473076));
#28902=CARTESIAN_POINT('Ctrl Pts',(8.15473535981986,-4.94320927931174,9.88659437915724));
#28903=CARTESIAN_POINT('Ctrl Pts',(9.17052309187647,-4.34956920012189,10.1553288976265));
#28904=CARTESIAN_POINT('Ctrl Pts',(11.249912418623,-3.2475765754686,10.5681406908193));
#28905=CARTESIAN_POINT('Ctrl Pts',(12.2613271155137,-2.71507294053767,10.7096926815135));
#28906=CARTESIAN_POINT('Ctrl Pts',(14.3530613265277,-1.75089621035865,10.9182780492489));
#28907=CARTESIAN_POINT('Ctrl Pts',(15.3683896576347,-1.30024364084097,10.9736589531833));
#28908=CARTESIAN_POINT('Ctrl Pts',(17.4699484560063,-0.51160650808575,11.0479347559914));
#28909=CARTESIAN_POINT('Ctrl Pts',(18.4899441076999,-0.154966618543408,
11.0518486975415));
#28910=CARTESIAN_POINT('Ctrl Pts',(19.8459385111079,0.227738630131172,11.0525063200436));
#28911=CARTESIAN_POINT('Ctrl Pts',(20.3436052070642,0.364012293347549,11.0499443867429));
#28912=CARTESIAN_POINT('Ctrl Pts',(21.3765735172499,0.626365466004486,11.0391187302377));
#28913=CARTESIAN_POINT('Ctrl Pts',(22.1786513408684,0.80148237085404,11.0271780970656));
#28914=CARTESIAN_POINT('Ctrl Pts',(22.8524711894103,0.927590054426942,11.0190184236597));
#28915=CARTESIAN_POINT('Ctrl Pts',(23.1034772575406,0.973361071581968,11.015636270466));
#28916=CARTESIAN_POINT('Ctrl Pts',(23.6153488598143,1.06157978958535,11.0082046691873));
#28917=CARTESIAN_POINT('Ctrl Pts',(24.2640912191231,1.16309571993124,10.9980907558832));
#28918=CARTESIAN_POINT('Ctrl Pts',(24.9252112071703,1.25112898708133,10.9882975006411));
#28919=CARTESIAN_POINT('Ctrl Pts',(25.3924209938587,1.30426168416562,10.9823391891697));
#28920=CARTESIAN_POINT('Ctrl Pts',(25.6607104515486,1.332046615497,10.9792975977554));
#28921=CARTESIAN_POINT('Ctrl Pts',(25.7950739758558,1.34502686686554,10.9779150347045));
#28922=CARTESIAN_POINT('Ctrl Pts',(26.2512918422651,1.38748529291552,10.9735046934062));
#28923=CARTESIAN_POINT('Ctrl Pts',(27.3073301682004,1.45732017866833,10.9653764904263));
#28924=CARTESIAN_POINT('Ctrl Pts',(28.3319194320811,1.48237708919284,10.9609947024269));
#28925=CARTESIAN_POINT('Ctrl Pts',(29.1280123944214,1.50394716937725,10.9582092660149));
#28926=CARTESIAN_POINT('Ctrl Pts',(29.4779818455993,1.51103964894258,10.9573324846489));
#28927=CARTESIAN_POINT('Ctrl Pts',(29.9466600480359,1.51533483257754,10.9567800220405));
#28928=CARTESIAN_POINT('Ctrl Pts',(30.4585980273686,1.51632751174059,10.956656708735));
#28929=CARTESIAN_POINT('Ctrl Pts',(31.4732549878281,1.51158385370564,10.9572594965941));
#28930=CARTESIAN_POINT('Ctrl Pts',(32.3455845021632,1.4999511927851,10.95879335959));
#28931=CARTESIAN_POINT('Ctrl Pts',(33.1628510802405,1.49997453311311,10.9587933798862));
#28932=CARTESIAN_POINT('Ctrl Pts',(33.4532441810442,1.49997366471359,10.9587933789851));
#28933=CARTESIAN_POINT('Ctrl Pts',(33.7813843869345,1.49997637381128,10.9587933812939));
#28934=CARTESIAN_POINT('Ctrl Pts',(34.2755379701535,1.49997699476315,10.9587933817727));
#28935=CARTESIAN_POINT('Ctrl Pts',(34.8102302793009,1.49998326277599,10.9587933869434));
#28936=CARTESIAN_POINT('Ctrl Pts',(35.6332452367756,1.49998412101817,10.9587933876415));
#28937=CARTESIAN_POINT('Ctrl Pts',(36.2915450349079,1.49998577371297,10.9587933890033));
#28938=CARTESIAN_POINT('Ctrl Pts',(38.1020137670942,1.49998803993575,10.9587933908629));
#28939=CARTESIAN_POINT('Ctrl Pts',(39.5833333333333,1.5,10.9587934006931));
#28940=CARTESIAN_POINT('Ctrl Pts',(40.9,1.5,10.9587934006931));
#28941=CARTESIAN_POINT('Ctrl Pts',(6.65963435785827,-8.56288377493212,13.0027682689653));
#28942=CARTESIAN_POINT('Ctrl Pts',(6.7513219377677,-8.49067817166156,13.050957789036));
#28943=CARTESIAN_POINT('Ctrl Pts',(6.84370278928156,-8.41801298642698,13.0985893115687));
#28944=CARTESIAN_POINT('Ctrl Pts',(7.91483960325935,-7.57680655910808,13.6397807532085));
#28945=CARTESIAN_POINT('Ctrl Pts',(8.9325509112231,-6.75518385076231,14.0543934435321));
#28946=CARTESIAN_POINT('Ctrl Pts',(11.0192135814157,-5.22065437877307,14.7040310435559));
#28947=CARTESIAN_POINT('Ctrl Pts',(12.0340542508324,-4.4769598695545,14.9356992206141));
#28948=CARTESIAN_POINT('Ctrl Pts',(14.1407660172285,-3.1214593369057,15.2883456800052));
#28949=CARTESIAN_POINT('Ctrl Pts',(15.1616568764318,-2.48732138966201,15.3931503655329));
#28950=CARTESIAN_POINT('Ctrl Pts',(17.287218760307,-1.36959877283814,15.5446125872455));
#28951=CARTESIAN_POINT('Ctrl Pts',(18.3145546794907,-0.86490278664151,15.5707395254148));
#28952=CARTESIAN_POINT('Ctrl Pts',(19.6926214867647,-0.318801403605146,
15.5935126543779));
#28953=CARTESIAN_POINT('Ctrl Pts',(20.19452636269,-0.125373946234777,15.5977145841048));
#28954=CARTESIAN_POINT('Ctrl Pts',(21.2420076978203,0.248868189963681,15.5972978704292));
#28955=CARTESIAN_POINT('Ctrl Pts',(22.0575126096201,0.499284562147392,15.5901933457539));
#28956=CARTESIAN_POINT('Ctrl Pts',(22.7441078663834,0.679992377552245,15.5856475377419));
#28957=CARTESIAN_POINT('Ctrl Pts',(22.9980856324395,0.745267685418834,15.5834353094767));
#28958=CARTESIAN_POINT('Ctrl Pts',(23.5177883906687,0.871419538176182,15.5778337615218));
#28959=CARTESIAN_POINT('Ctrl Pts',(24.1766640555165,1.01665680544524,15.569151455817));
#28960=CARTESIAN_POINT('Ctrl Pts',(24.8496697365589,1.14287321247013,15.560128822227));
#28961=CARTESIAN_POINT('Ctrl Pts',(25.3259254544069,1.2191404135396,15.554601684436));
#28962=CARTESIAN_POINT('Ctrl Pts',(25.5996882691236,1.2590574298324,15.5518109321211));
#28963=CARTESIAN_POINT('Ctrl Pts',(25.7368188560809,1.27770917936971,15.550561003587));
#28964=CARTESIAN_POINT('Ctrl Pts',(26.2030586507879,1.33878235986071,15.5466206431081));
#28965=CARTESIAN_POINT('Ctrl Pts',(27.2845562696213,1.43928616936987,15.5388831179539));
#28966=CARTESIAN_POINT('Ctrl Pts',(28.3146233763975,1.47473229777557,15.534108117874));
#28967=CARTESIAN_POINT('Ctrl Pts',(29.1121433593266,1.5053783917148,15.5313810124223));
#28968=CARTESIAN_POINT('Ctrl Pts',(29.4693616319656,1.51558516408219,15.5305221749293));
#28969=CARTESIAN_POINT('Ctrl Pts',(29.9425518103672,1.5216968643791,15.5299808253862));
#28970=CARTESIAN_POINT('Ctrl Pts',(30.4595136734855,1.52312339822457,15.5298599056894));
#28971=CARTESIAN_POINT('Ctrl Pts',(31.4800666545032,1.51634797661239,15.5304501241615));
#28972=CARTESIAN_POINT('Ctrl Pts',(32.3507119180564,1.4999128955352,15.5319509809364));
#28973=CARTESIAN_POINT('Ctrl Pts',(33.1621363777215,1.49995461572564,15.5319505779396));
#28974=CARTESIAN_POINT('Ctrl Pts',(33.4535196029878,1.49995304854269,15.5319505880019));
#28975=CARTESIAN_POINT('Ctrl Pts',(33.7812306484551,1.49995788616631,15.5319505396377));
#28976=CARTESIAN_POINT('Ctrl Pts',(34.2755524327802,1.49995898984267,15.531950526851));
#28977=CARTESIAN_POINT('Ctrl Pts',(34.8101578274898,1.49997016508529,15.5319504091692));
#28978=CARTESIAN_POINT('Ctrl Pts',(35.6332135248365,1.49997169422773,15.5319503927198));
#28979=CARTESIAN_POINT('Ctrl Pts',(36.2914988048216,1.49997464065555,15.5319503616369));
#28980=CARTESIAN_POINT('Ctrl Pts',(38.1019885414694,1.49997868009126,15.5319503187541));
#28981=CARTESIAN_POINT('Ctrl Pts',(39.5833333333333,1.5,15.5319500929849));
#28982=CARTESIAN_POINT('Ctrl Pts',(40.9,1.5,15.5319500929849));
#28983=CARTESIAN_POINT('Ctrl Pts',(6.47503677058814,-13.6264850125633,19.2049631177014));
#28984=CARTESIAN_POINT('Ctrl Pts',(6.56582707216344,-13.5206117629928,19.2807931407427));
#28985=CARTESIAN_POINT('Ctrl Pts',(6.65722187862393,-13.4141026801341,19.3557456396964));
#28986=CARTESIAN_POINT('Ctrl Pts',(7.71979853459931,-12.1774082172639,20.2113974185276));
#28987=CARTESIAN_POINT('Ctrl Pts',(8.72714740265586,-10.9649265084515,20.876585861408));
#28988=CARTESIAN_POINT('Ctrl Pts',(10.792252425961,-8.69413764846818,21.9312131301472));
#28989=CARTESIAN_POINT('Ctrl Pts',(11.8008983729842,-7.58577239973431,22.3203974544121));
#28990=CARTESIAN_POINT('Ctrl Pts',(13.892634394048,-5.56042793834188,22.9231109701401));
#28991=CARTESIAN_POINT('Ctrl Pts',(14.910936596525,-4.60683703173286,23.1162450123325));
#28992=CARTESIAN_POINT('Ctrl Pts',(17.0374816014601,-2.91606182242837,23.4053158267904));
#28993=CARTESIAN_POINT('Ctrl Pts',(18.0678529336714,-2.15006970557795,23.4724397837998));
#28994=CARTESIAN_POINT('Ctrl Pts',(19.4632774216583,-1.31129970902877,23.5361137002685));
#28995=CARTESIAN_POINT('Ctrl Pts',(19.9690853949367,-1.01646669656859,23.5527456051548));
#28996=CARTESIAN_POINT('Ctrl Pts',(21.0306109698709,-0.441678056412671,
23.5717577824589));
#28997=CARTESIAN_POINT('Ctrl Pts',(21.8626014988188,-0.054300344268142,
23.5739085372705));
#28998=CARTESIAN_POINT('Ctrl Pts',(22.5665651705188,0.226484889079844,23.576178914363));
#28999=CARTESIAN_POINT('Ctrl Pts',(22.8246411038756,0.326902916553466,23.5761448043361));
#29000=CARTESIAN_POINT('Ctrl Pts',(23.3554232774669,0.522054743089693,23.5740054132278));
#29001=CARTESIAN_POINT('Ctrl Pts',(24.0293769285439,0.747005858788649,23.5680817805141));
#29002=CARTESIAN_POINT('Ctrl Pts',(24.7209631427047,0.943393581394331,23.560586503548));
#29003=CARTESIAN_POINT('Ctrl Pts',(25.2118242719342,1.06233480615607,23.5558940963915));
#29004=CARTESIAN_POINT('Ctrl Pts',(25.4945546545947,1.12470144437592,23.5535795021665));
#29005=CARTESIAN_POINT('Ctrl Pts',(25.6362544160062,1.15385183559377,23.5525764277763));
#29006=CARTESIAN_POINT('Ctrl Pts',(26.1191683853685,1.24953281052836,23.5495095529483));
#29007=CARTESIAN_POINT('Ctrl Pts',(27.244410780189,1.40715534997208,23.5425023713064));
#29008=CARTESIAN_POINT('Ctrl Pts',(28.2843056152442,1.46065929315376,23.5370396227258));
#29009=CARTESIAN_POINT('Ctrl Pts',(29.0843244121809,1.50737208683505,23.5344215873996));
#29010=CARTESIAN_POINT('Ctrl Pts',(29.4542021761287,1.52336782189617,23.5335942286398));
#29011=CARTESIAN_POINT('Ctrl Pts',(29.9352997409898,1.53271512054377,23.5330734925559));
#29012=CARTESIAN_POINT('Ctrl Pts',(30.4610555884278,1.5349453613852,23.532957187389));
#29013=CARTESIAN_POINT('Ctrl Pts',(31.4919316519535,1.52450364515754,23.5335262680548));
#29014=CARTESIAN_POINT('Ctrl Pts',(32.3596576160514,1.49979324124413,23.5349731541844));
#29015=CARTESIAN_POINT('Ctrl Pts',(33.1608710165812,1.49989213988255,23.5349736853906));
#29016=CARTESIAN_POINT('Ctrl Pts',(33.4539865796869,1.49988845489238,23.5349736699323));
#29017=CARTESIAN_POINT('Ctrl Pts',(33.780948091659,1.49989993226727,23.5349737329761));
#29018=CARTESIAN_POINT('Ctrl Pts',(34.275564602361,1.49990256114204,23.5349737489117));
#29019=CARTESIAN_POINT('Ctrl Pts',(34.8100214672069,1.49992910993535,23.5349738998239));
#29020=CARTESIAN_POINT('Ctrl Pts',(35.6331489543767,1.49993274473985,23.5349739207807));
#29021=CARTESIAN_POINT('Ctrl Pts',(36.2914097700016,1.4999397448351,23.5349739606187));
#29022=CARTESIAN_POINT('Ctrl Pts',(38.1019375614968,1.49994934328327,23.5349740154737));
#29023=CARTESIAN_POINT('Ctrl Pts',(39.5833333333333,1.5,23.5349743044955));
#29024=CARTESIAN_POINT('Ctrl Pts',(40.9,1.5,23.5349743044955));
#29025=CARTESIAN_POINT('Ctrl Pts',(6.39840282685635,-18.5950148818,25.4797798158266));
#29026=CARTESIAN_POINT('Ctrl Pts',(6.48879582230594,-18.455456538043,25.5825069307027));
#29027=CARTESIAN_POINT('Ctrl Pts',(6.57973810483189,-18.3151558806717,25.684006582131));
#29028=CARTESIAN_POINT('Ctrl Pts',(7.63881202209716,-16.6821095714367,26.8457843562122));
#29029=CARTESIAN_POINT('Ctrl Pts',(8.64206536867565,-15.0805562774161,27.7524045864227));
#29030=CARTESIAN_POINT('Ctrl Pts',(10.6943835463645,-12.08639394536,29.194220471563));
#29031=CARTESIAN_POINT('Ctrl Pts',(11.6986850371145,-10.6188960618635,29.7340826089764));
#29032=CARTESIAN_POINT('Ctrl Pts',(13.7736723466472,-7.9480571508383,30.5724457120527));
#29033=CARTESIAN_POINT('Ctrl Pts',(14.7865355152845,-6.68379951334874,30.8496813329458));
#29034=CARTESIAN_POINT('Ctrl Pts',(16.895644387614,-4.44867953439714,31.2681094727719));
#29035=CARTESIAN_POINT('Ctrl Pts',(17.921113585793,-3.42955614780409,31.3748718553479));
#29036=CARTESIAN_POINT('Ctrl Pts',(19.3111115725317,-2.31180057560694,31.4778602005301));
#29037=CARTESIAN_POINT('Ctrl Pts',(19.8164097330209,-1.91755167896535,31.5068304778962));
#29038=CARTESIAN_POINT('Ctrl Pts',(20.8772665291465,-1.14804732053491,31.5450009606978));
#29039=CARTESIAN_POINT('Ctrl Pts',(21.7126526899651,-0.625757760628936,
31.5565752055434));
#29040=CARTESIAN_POINT('Ctrl Pts',(22.4233939916368,-0.244774266221903,
31.5658469864011));
#29041=CARTESIAN_POINT('Ctrl Pts',(22.68321700305,-0.109074102068984,31.568070163829));
#29042=CARTESIAN_POINT('Ctrl Pts',(23.2191843843282,0.155714853804436,31.5695528321153));
#29043=CARTESIAN_POINT('Ctrl Pts',(23.9014490792895,0.461901703286709,31.5665856540486));
#29044=CARTESIAN_POINT('Ctrl Pts',(24.6052033552109,0.730987709817267,31.5607844376464));
#29045=CARTESIAN_POINT('Ctrl Pts',(25.1069219885717,0.894795181267931,31.5570192016244));
#29046=CARTESIAN_POINT('Ctrl Pts',(25.3966703145091,0.980957842597309,31.5552253028176));
#29047=CARTESIAN_POINT('Ctrl Pts',(25.5420691491796,1.02128571697646,31.5544886793522));
#29048=CARTESIAN_POINT('Ctrl Pts',(26.0386675456483,1.15405115562807,31.5523567719375));
#29049=CARTESIAN_POINT('Ctrl Pts',(27.2041996425261,1.37405103438869,31.5461367082151));
#29050=CARTESIAN_POINT('Ctrl Pts',(28.254481539011,1.44553527377015,31.5399727189289));
#29051=CARTESIAN_POINT('Ctrl Pts',(29.0567817440806,1.50856328668891,31.5374655658645));
#29052=CARTESIAN_POINT('Ctrl Pts',(29.4392037716731,1.53093305020556,31.5366692491296));
#29053=CARTESIAN_POINT('Ctrl Pts',(29.9281985709061,1.54360558359609,31.536168682902));
#29054=CARTESIAN_POINT('Ctrl Pts',(30.4627354290944,1.54671304059522,31.5360567738141));
#29055=CARTESIAN_POINT('Ctrl Pts',(31.5039222132188,1.53240580330097,31.5366047697957));
#29056=CARTESIAN_POINT('Ctrl Pts',(32.3686614831274,1.49961223537188,31.5379963364647));
#29057=CARTESIAN_POINT('Ctrl Pts',(33.1596379899179,1.49979803313559,31.5379973429874));
#29058=CARTESIAN_POINT('Ctrl Pts',(33.4544864001145,1.49979103760184,31.5379973136915));
#29059=CARTESIAN_POINT('Ctrl Pts',(33.7806952343975,1.49981257637976,31.5379974331442));
#29060=CARTESIAN_POINT('Ctrl Pts',(34.2756055948936,1.49981748473541,31.5379974633363));
#29061=CARTESIAN_POINT('Ctrl Pts',(34.8099061252942,1.49986722177693,31.5379977492716));
#29062=CARTESIAN_POINT('Ctrl Pts',(35.6331043028646,1.49987402634112,31.5379977889784));
#29063=CARTESIAN_POINT('Ctrl Pts',(36.2913385913736,1.49988713966987,31.5379978644599));
#29064=CARTESIAN_POINT('Ctrl Pts',(38.1019015852784,1.49990511666357,31.537997968394));
#29065=CARTESIAN_POINT('Ctrl Pts',(39.5833333333333,1.5,31.5379985160061));
#29066=CARTESIAN_POINT('Ctrl Pts',(40.9,1.5,31.5379985160061));
#29067=CARTESIAN_POINT('Ctrl Pts',(6.37427268165564,-20.7176664141567,28.1741189428499));
#29068=CARTESIAN_POINT('Ctrl Pts',(6.46448755772839,-20.5636424771022,28.2883460540946));
#29069=CARTESIAN_POINT('Ctrl Pts',(6.55522687426754,-20.4088293925213,28.4011972468989));
#29070=CARTESIAN_POINT('Ctrl Pts',(7.61282240204205,-18.6056139772311,29.693787896276));
#29071=CARTESIAN_POINT('Ctrl Pts',(8.61454082730176,-16.8370699794085,30.703424507615));
#29072=CARTESIAN_POINT('Ctrl Pts',(10.6618274824665,-13.5325068155167,32.3104201819496));
#29073=CARTESIAN_POINT('Ctrl Pts',(11.6645377987076,-11.9110180488694,32.9144254040795));
#29074=CARTESIAN_POINT('Ctrl Pts',(13.7331445959134,-8.96386257277558,33.8529424117878));
#29075=CARTESIAN_POINT('Ctrl Pts',(14.7439932704909,-7.56674532731094,34.1658004948675));
#29076=CARTESIAN_POINT('Ctrl Pts',(16.8461035490385,-5.10012840374637,34.6388264066738));
#29077=CARTESIAN_POINT('Ctrl Pts',(17.8695058124616,-3.97333364734334,34.7622645166785));
#29078=CARTESIAN_POINT('Ctrl Pts',(19.2561174443541,-2.73821070416468,34.8817349492475));
#29079=CARTESIAN_POINT('Ctrl Pts',(19.7609345646798,-2.30176586395498,34.9159214541564));
#29080=CARTESIAN_POINT('Ctrl Pts',(20.8205141053453,-1.45015687002429,34.9621410370326));
#29081=CARTESIAN_POINT('Ctrl Pts',(21.6560023791939,-0.871078443386998,
34.9776907709078));
#29082=CARTESIAN_POINT('Ctrl Pts',(22.3682688599883,-0.447778285927138,
34.989939594886));
#29083=CARTESIAN_POINT('Ctrl Pts',(22.6285200842947,-0.297086276283264,
34.9931281975259));
#29084=CARTESIAN_POINT('Ctrl Pts',(23.1658603614091,-0.00273379297028158,
34.9961605697035));
#29085=CARTESIAN_POINT('Ctrl Pts',(23.8505975407037,0.338068372298849,34.9944676948756));
#29086=CARTESIAN_POINT('Ctrl Pts',(24.5583968797874,0.638319272935674,34.9894056975888));
#29087=CARTESIAN_POINT('Ctrl Pts',(25.0640148551739,0.821498314632839,34.9860476379143));
#29088=CARTESIAN_POINT('Ctrl Pts',(25.3563632502514,0.917977493583091,34.9844821378475));
#29089=CARTESIAN_POINT('Ctrl Pts',(25.503160007456,0.963163948801064,34.9838621425449));
#29090=CARTESIAN_POINT('Ctrl Pts',(26.0049713545738,1.11209382847184,34.982139121313));
#29091=CARTESIAN_POINT('Ctrl Pts',(27.1869304722337,1.35965020681436,34.9762666166019));
#29092=CARTESIAN_POINT('Ctrl Pts',(28.2418054197051,1.43886806122646,34.9698003983093));
#29093=CARTESIAN_POINT('Ctrl Pts',(29.0450356043991,1.5089275405599,34.9673414359535));
#29094=CARTESIAN_POINT('Ctrl Pts',(29.4328041419752,1.53413528152413,34.9665583691038));
#29095=CARTESIAN_POINT('Ctrl Pts',(29.9251825362975,1.54824951859995,34.9660664512209));
#29096=CARTESIAN_POINT('Ctrl Pts',(30.4634799414205,1.55174636239756,34.9659564211645));
#29097=CARTESIAN_POINT('Ctrl Pts',(31.5090833787051,1.53574598606795,34.9664954410524));
#29098=CARTESIAN_POINT('Ctrl Pts',(32.3725304400172,1.49952340891733,34.9678633362529));
#29099=CARTESIAN_POINT('Ctrl Pts',(33.1591152593399,1.49975189997366,34.9678645826042));
#29100=CARTESIAN_POINT('Ctrl Pts',(33.4547063903441,1.49974326694616,34.9678645463389));
#29101=CARTESIAN_POINT('Ctrl Pts',(33.7805921021893,1.49976974530861,34.9678646942577));
#29102=CARTESIAN_POINT('Ctrl Pts',(34.2756282408745,1.49977576894615,34.9678647316484));
#29103=CARTESIAN_POINT('Ctrl Pts',(34.8098603973427,1.49983687714898,34.967865085736));
#29104=CARTESIAN_POINT('Ctrl Pts',(35.6330886763766,1.49984523535833,34.9678651349076));
#29105=CARTESIAN_POINT('Ctrl Pts',(36.2913112329655,1.49986134640235,34.9678652283802));
#29106=CARTESIAN_POINT('Ctrl Pts',(38.1018888107018,1.49988343135295,34.9678653570876));
#29107=CARTESIAN_POINT('Ctrl Pts',(39.5833333333333,1.5,34.9678660352249));
#29108=CARTESIAN_POINT('Ctrl Pts',(40.9,1.5,34.9678660352249));
#29109=CARTESIAN_POINT('',(40.9,1.50000000000002,32.9658914637539));
#29110=CARTESIAN_POINT('Ctrl Pts',(40.9,1.50000000000002,32.9658914637539));
#29111=CARTESIAN_POINT('Ctrl Pts',(40.9,1.50000000000002,33.466386268912));
#29112=CARTESIAN_POINT('Ctrl Pts',(40.9,1.50000000000002,33.9668810740701));
#29113=CARTESIAN_POINT('Ctrl Pts',(40.9,1.50000000000002,34.4673758792282));
#29114=CARTESIAN_POINT('',(38.,1.50000000000001,32.9658914637539));
#29115=CARTESIAN_POINT('Ctrl Pts',(38.,1.5,32.9658914637539));
#29116=CARTESIAN_POINT('Ctrl Pts',(38.9666666666667,1.5,32.9658914637539));
#29117=CARTESIAN_POINT('Ctrl Pts',(39.9333333333333,1.5,32.9658914637539));
#29118=CARTESIAN_POINT('Ctrl Pts',(40.9,1.5,32.9658914637539));
#29119=CARTESIAN_POINT('Ctrl Pts',(37.4997714574611,1.49990106437153,32.3652585803353));
#29120=CARTESIAN_POINT('Ctrl Pts',(37.6667294826965,1.4999047077905,32.5658056765355));
#29121=CARTESIAN_POINT('Ctrl Pts',(37.8334450600885,1.49990923999261,32.7660568372681));
#29122=CARTESIAN_POINT('Ctrl Pts',(37.9998166694663,1.49991439209149,32.9658909678229));
#29123=CARTESIAN_POINT('',(6.9,-16.9192021366758,24.7737885487526));
#29124=CARTESIAN_POINT('Ctrl Pts',(6.9,-16.9192021366758,24.7737885487526));
#29125=CARTESIAN_POINT('Ctrl Pts',(6.9,-15.3881766950258,22.6454446228759));
#29126=CARTESIAN_POINT('Ctrl Pts',(6.90000000000115,-13.8353835251886,20.4978726403359));
#29127=CARTESIAN_POINT('Ctrl Pts',(6.90000000000115,-10.3082122779765,15.662481608859));
#29128=CARTESIAN_POINT('Ctrl Pts',(6.9,-7.95935811114668,12.4764228571341));
#29129=CARTESIAN_POINT('Ctrl Pts',(6.9,-5.6597919716369,9.46599415782505));
#29130=CARTESIAN_POINT('',(22.9245129145126,1.94538850028551E-15,31.7706052331164));
#29131=CARTESIAN_POINT('Ctrl Pts',(22.9245129145126,6.11247215341707E-15,
31.7706052331164));
#29132=CARTESIAN_POINT('Ctrl Pts',(22.7202811020963,-0.0979233563002629,
31.7014549124251));
#29133=CARTESIAN_POINT('Ctrl Pts',(22.5089075447093,-0.203440182623871,
31.6320805544326));
#29134=CARTESIAN_POINT('Ctrl Pts',(22.2913349439917,-0.316637134194165,
31.5632247707622));
#29135=CARTESIAN_POINT('Ctrl Pts',(21.4451770585292,-0.756869465221198,
31.2954389184983));
#29136=CARTESIAN_POINT('Ctrl Pts',(20.5220951556666,-1.35418571023233,31.0475106147151));
#29137=CARTESIAN_POINT('Ctrl Pts',(19.7671428819537,-1.89915402350715,30.8612920963157));
#29138=CARTESIAN_POINT('Ctrl Pts',(19.519477305839,-2.07793339270839,30.8002022522972));
#29139=CARTESIAN_POINT('Ctrl Pts',(19.286571638609,-2.25204835959326,30.7444068279677));
#29140=CARTESIAN_POINT('Ctrl Pts',(19.0728538401323,-2.41532203906683,30.6939488833522));
#29141=CARTESIAN_POINT('Ctrl Pts',(18.7028555998035,-2.69798906318815,30.6065937315987));
#29142=CARTESIAN_POINT('Ctrl Pts',(18.4144703596235,-2.93373938287723,30.5399660639319));
#29143=CARTESIAN_POINT('Ctrl Pts',(18.0642874871537,-3.23398234070002,30.4582462938821));
#29144=CARTESIAN_POINT('Ctrl Pts',(17.442092711672,-3.76744532366929,30.3130489756353));
#29145=CARTESIAN_POINT('Ctrl Pts',(16.7224564418218,-4.43872907330236,30.1446863488622));
#29146=CARTESIAN_POINT('Ctrl Pts',(15.9202806616111,-5.24401550821529,29.9321297384067));
#29147=CARTESIAN_POINT('Ctrl Pts',(15.4090529834516,-5.75722561070139,29.7966671314304));
#29148=CARTESIAN_POINT('Ctrl Pts',(14.8739602945711,-6.33424649579702,29.6418940055914));
#29149=CARTESIAN_POINT('Ctrl Pts',(14.3169794331149,-6.96996102647284,29.455763484612));
#29150=CARTESIAN_POINT('Ctrl Pts',(13.8864206762832,-7.4613826837844,29.3118803976567));
#29151=CARTESIAN_POINT('Ctrl Pts',(13.3867890027802,-8.05270459512032,29.1311705407938));
#29152=CARTESIAN_POINT('Ctrl Pts',(12.8146824059514,-8.75043091662868,28.8915984033895));
#29153=CARTESIAN_POINT('Ctrl Pts',(12.2526665517595,-9.43585083093891,28.6562518085588));
#29154=CARTESIAN_POINT('Ctrl Pts',(11.6379478462804,-10.231366276768,28.3625845909803));
#29155=CARTESIAN_POINT('Ctrl Pts',(10.9739250490308,-11.1267230319105,27.981021293096));
#29156=CARTESIAN_POINT('Ctrl Pts',(10.5683455447963,-11.6735993596027,27.747965660321));
#29157=CARTESIAN_POINT('Ctrl Pts',(10.1437415406956,-12.2581093618546,27.4801235315866));
#29158=CARTESIAN_POINT('Ctrl Pts',(9.74137929176525,-12.8142541611144,27.2046666925187));
#29159=CARTESIAN_POINT('Ctrl Pts',(8.72285779294234,-14.2220538143138,26.5073877769786));
#29160=CARTESIAN_POINT('Ctrl Pts',(7.81323138778195,-15.580948814124,25.7100913255874));
#29161=CARTESIAN_POINT('Ctrl Pts',(6.9,-16.9192021366758,24.7737885487526));
#29162=CARTESIAN_POINT('Ctrl Pts',(30.5,1.55029606206997,34.9656486014478));
#29163=CARTESIAN_POINT('Ctrl Pts',(29.9560179420817,1.55343104498103,34.7222276068062));
#29164=CARTESIAN_POINT('Ctrl Pts',(29.4152668325132,1.54030953139106,34.4790656554127));
#29165=CARTESIAN_POINT('Ctrl Pts',(28.8740459957565,1.49470250846617,34.2361296888632));
#29166=CARTESIAN_POINT('Ctrl Pts',(28.3535277923439,1.4508400330705,34.0024864433252));
#29167=CARTESIAN_POINT('Ctrl Pts',(27.8179515912466,1.40923473841146,33.7608540997398));
#29168=CARTESIAN_POINT('Ctrl Pts',(27.2695051149491,1.33972398862116,33.5168388499063));
#29169=CARTESIAN_POINT('Ctrl Pts',(26.9554553615883,1.29992095446743,33.3771115796287));
#29170=CARTESIAN_POINT('Ctrl Pts',(26.6378099296971,1.25106463707208,33.2369493090937));
#29171=CARTESIAN_POINT('Ctrl Pts',(26.3179304017917,1.18777049128279,33.0983258448229));
#29172=CARTESIAN_POINT('Ctrl Pts',(26.1078196745982,1.14619615520081,33.0072719500184));
#29173=CARTESIAN_POINT('Ctrl Pts',(25.8967402232745,1.09839525532296,32.9168907470981));
#29174=CARTESIAN_POINT('Ctrl Pts',(25.6850706236774,1.04282885388104,32.8277596053404));
#29175=CARTESIAN_POINT('Ctrl Pts',(25.6562210027417,1.03525540156946,32.8156114288513));
#29176=CARTESIAN_POINT('Ctrl Pts',(25.6277737638215,1.0276506122434,32.8036595933923));
#29177=CARTESIAN_POINT('Ctrl Pts',(25.5983858063598,1.01964325944536,32.7913423709803));
#29178=CARTESIAN_POINT('Ctrl Pts',(25.1249357452756,0.890642063078173,32.5929076988546));
#29179=CARTESIAN_POINT('Ctrl Pts',(24.1510084067019,0.588069770626604,32.1858811669087));
#29180=CARTESIAN_POINT('Ctrl Pts',(22.9245129145126,6.11247215341707E-15,
31.7706052331164));
#29181=CARTESIAN_POINT('Origin',(40.65,0.,0.));
#29182=CARTESIAN_POINT('',(40.4,-18.7829592905825,29.5330398077868));
#29183=CARTESIAN_POINT('',(40.9,-18.5327260452907,29.0996231131986));
#29184=CARTESIAN_POINT('Ctrl Pts',(40.4,-18.7829592905825,29.5330398077868));
#29185=CARTESIAN_POINT('Ctrl Pts',(40.5666590136477,-18.6995531510789,29.3885761365034));
#29186=CARTESIAN_POINT('Ctrl Pts',(40.733343045036,-18.6161333949886,29.2440888806));
#29187=CARTESIAN_POINT('Ctrl Pts',(40.9,-18.5327260452907,29.0996231131986));
#29188=CARTESIAN_POINT('',(40.9,-15.9346498339374,30.5996231131986));
#29189=CARTESIAN_POINT('Origin',(40.9,0.,0.));
#29190=CARTESIAN_POINT('',(40.4,-16.1848830792292,31.0330398077868));
#29191=CARTESIAN_POINT('Ctrl Pts',(40.9,-15.9346498339374,30.5996231131986));
#29192=CARTESIAN_POINT('Ctrl Pts',(40.7333430442473,-16.0180571840301,30.7440888812837));
#29193=CARTESIAN_POINT('Ctrl Pts',(40.5666590122953,-16.1014769404025,30.8885761376758));
#29194=CARTESIAN_POINT('Ctrl Pts',(40.4,-16.1848830792292,31.0330398077868));
#29195=CARTESIAN_POINT('Origin',(40.4,0.,0.));
#29196=CARTESIAN_POINT('Origin',(35.7,0.,0.));
#29197=CARTESIAN_POINT('',(30.5,-16.1402285275843,31.0562879796886));
#29198=CARTESIAN_POINT('Ctrl Pts',(40.3999012894849,-16.1848928782182,31.0330346270951));
#29199=CARTESIAN_POINT('Ctrl Pts',(39.2494626810401,-16.1849362443212,31.0330116996609));
#29200=CARTESIAN_POINT('Ctrl Pts',(38.0976708836828,-16.1851115327779,31.0329190263647));
#29201=CARTESIAN_POINT('Ctrl Pts',(36.9467340384723,-16.1851746119074,31.0328856894588));
#29202=CARTESIAN_POINT('Ctrl Pts',(36.745427730736,-16.1851856448557,31.032879858618));
#29203=CARTESIAN_POINT('Ctrl Pts',(36.5441475779313,-16.1851932450653,31.0328758430125));
#29204=CARTESIAN_POINT('Ctrl Pts',(36.3429119519248,-16.1852000001162,31.0328722727086));
#29205=CARTESIAN_POINT('Ctrl Pts',(36.2102758775794,-16.1852044524265,31.0328699194916));
#29206=CARTESIAN_POINT('Ctrl Pts',(36.0822774296293,-16.1852084224022,31.0328678560427));
#29207=CARTESIAN_POINT('Ctrl Pts',(35.9587202262686,-16.1852125810274,31.0328657167445));
#29208=CARTESIAN_POINT('Ctrl Pts',(35.7925662245336,-16.1852181733537,31.0328628399153));
#29209=CARTESIAN_POINT('Ctrl Pts',(35.6344388155489,-16.1852241162452,31.0328598211429));
#29210=CARTESIAN_POINT('Ctrl Pts',(35.4837714463452,-16.1852312078526,31.032856216152));
#29211=CARTESIAN_POINT('Ctrl Pts',(35.3175474553577,-16.1852390316786,31.0328522389407));
#29212=CARTESIAN_POINT('Ctrl Pts',(35.1604041224813,-16.1852482463284,31.0328475520712));
#29213=CARTESIAN_POINT('Ctrl Pts',(35.0116427948686,-16.1852592402397,31.0328419178902));
#29214=CARTESIAN_POINT('Ctrl Pts',(34.997927209115,-16.1852602538629,31.0328413984267));
#29215=CARTESIAN_POINT('Ctrl Pts',(34.9842829110374,-16.1852612822246,31.0328408711132));
#29216=CARTESIAN_POINT('Ctrl Pts',(34.9707093736272,-16.1852623254084,31.0328403358797));
#29217=CARTESIAN_POINT('Ctrl Pts',(34.8522491799023,-16.1852714295754,31.0328356647415));
#29218=CARTESIAN_POINT('Ctrl Pts',(34.7391835006529,-16.1852816068676,31.0328304196803));
#29219=CARTESIAN_POINT('Ctrl Pts',(34.6312849042887,-16.1852915612823,31.0328252639047));
#29220=CARTESIAN_POINT('Ctrl Pts',(34.5096795260853,-16.1853027802453,31.0328194531708));
#29221=CARTESIAN_POINT('Ctrl Pts',(34.394637058133,-16.1853137193614,31.0328137541413));
#29222=CARTESIAN_POINT('Ctrl Pts',(34.2857585821194,-16.1853233495613,31.0328086821746));
#29223=CARTESIAN_POINT('Ctrl Pts',(34.1786801908155,-16.1853328205454,31.0328036940625));
#29224=CARTESIAN_POINT('Ctrl Pts',(34.0775620514829,-16.185341043166,31.0327993031901));
#29225=CARTESIAN_POINT('Ctrl Pts',(33.9819758246427,-16.1853475980775,31.0327957057953));
#29226=CARTESIAN_POINT('Ctrl Pts',(33.9184449689727,-16.1853519547631,31.0327933148067));
#29227=CARTESIAN_POINT('Ctrl Pts',(33.8573517602305,-16.1853555977387,31.0327912624254));
#29228=CARTESIAN_POINT('Ctrl Pts',(33.7984399511826,-16.1853587887284,31.0327894081824));
#29229=CARTESIAN_POINT('Ctrl Pts',(33.7337970612213,-16.1853622901453,31.0327873735543));
#29230=CARTESIAN_POINT('Ctrl Pts',(33.6717809742681,-16.1853652470742,31.0327855776265));
#29231=CARTESIAN_POINT('Ctrl Pts',(33.6121191806454,-16.1853678991828,31.0327838881567));
#29232=CARTESIAN_POINT('Ctrl Pts',(33.5695978710648,-16.1853697893561,31.0327826840617));
#29233=CARTESIAN_POINT('Ctrl Pts',(33.5282738752657,-16.185371522363,31.0327815352149));
#29234=CARTESIAN_POINT('Ctrl Pts',(33.4880643388298,-16.1853731585247,31.032780407062));
#29235=CARTESIAN_POINT('Ctrl Pts',(33.4508270573206,-16.1853746737428,31.0327793623013));
#29236=CARTESIAN_POINT('Ctrl Pts',(33.4145509216558,-16.1853761126592,31.0327783314862));
#29237=CARTESIAN_POINT('Ctrl Pts',(33.3793439789548,-16.1853777420673,31.0327771639657));
#29238=CARTESIAN_POINT('Ctrl Pts',(33.3411337035362,-16.1853795104722,31.0327758968498));
#29239=CARTESIAN_POINT('Ctrl Pts',(33.3041826660689,-16.1853815029502,31.0327744688781));
#29240=CARTESIAN_POINT('Ctrl Pts',(33.2685652776782,-16.1853839484229,31.0327727495066));
#29241=CARTESIAN_POINT('Ctrl Pts',(33.231009447455,-16.1853865269881,31.0327709365599));
#29242=CARTESIAN_POINT('Ctrl Pts',(33.1949357943681,-16.185389608116,31.0327688002293));
#29243=CARTESIAN_POINT('Ctrl Pts',(33.1603699172393,-16.1853933524012,31.0327662471215));
#29244=CARTESIAN_POINT('Ctrl Pts',(33.122371567942,-16.1853974685027,31.0327634404841));
#29245=CARTESIAN_POINT('Ctrl Pts',(33.0861949166479,-16.1854023852333,31.0327601306123));
#29246=CARTESIAN_POINT('Ctrl Pts',(33.0518089354078,-16.1854082033113,31.0327562557942));
#29247=CARTESIAN_POINT('Ctrl Pts',(33.0341030813062,-16.1854111991264,31.0327542605926));
#29248=CARTESIAN_POINT('Ctrl Pts',(33.0168710360023,-16.1854144322605,31.032752116523));
#29249=CARTESIAN_POINT('Ctrl Pts',(33.0001033802535,-16.1854179076007,31.0327498200704));
#29250=CARTESIAN_POINT('Ctrl Pts',(32.9420348133412,-16.1854299431544,31.0327418671573));
#29251=CARTESIAN_POINT('Ctrl Pts',(32.8874145324497,-16.1852296143114,31.0328461364757));
#29252=CARTESIAN_POINT('Ctrl Pts',(32.8357863520582,-16.1849068811705,31.0330149777623));
#29253=CARTESIAN_POINT('Ctrl Pts',(32.7779739682632,-16.1845454899291,31.0332040434467));
#29254=CARTESIAN_POINT('Ctrl Pts',(32.7239136589685,-16.1840302574575,31.0334742654593));
#29255=CARTESIAN_POINT('Ctrl Pts',(32.6729278684755,-16.1834371021678,31.033785409572));
#29256=CARTESIAN_POINT('Ctrl Pts',(32.6180801336262,-16.1827990180322,31.0341201214522));
#29257=CARTESIAN_POINT('Ctrl Pts',(32.5667902508432,-16.1820699950122,31.0345025939175));
#29258=CARTESIAN_POINT('Ctrl Pts',(32.5181731636797,-16.1812992842338,31.034906696383));
#29259=CARTESIAN_POINT('Ctrl Pts',(32.4659536029866,-16.1804714646211,31.0353407424038));
#29260=CARTESIAN_POINT('Ctrl Pts',(32.4168175136245,-16.1795947944396,31.0358001425894));
#29261=CARTESIAN_POINT('Ctrl Pts',(32.3696233879008,-16.1786925325962,31.0362725138779));
#29262=CARTESIAN_POINT('Ctrl Pts',(32.3182581618427,-16.1777105272546,31.0367866341767));
#29263=CARTESIAN_POINT('Ctrl Pts',(32.2691934412642,-16.1766975364928,31.0373164741889));
#29264=CARTESIAN_POINT('Ctrl Pts',(32.220906472482,-16.1756521425246,31.0378627004434));
#29265=CARTESIAN_POINT('Ctrl Pts',(32.1715370438644,-16.1745833137248,31.0384211715746));
#29266=CARTESIAN_POINT('Ctrl Pts',(32.1229805798603,-16.173479840102,31.0389971805319));
#29267=CARTESIAN_POINT('Ctrl Pts',(32.0735591134784,-16.1723205501867,31.039601856364));
#29268=CARTESIAN_POINT('Ctrl Pts',(32.0254239419646,-16.1711914331653,31.0401907942692));
#29269=CARTESIAN_POINT('Ctrl Pts',(31.9764682879417,-16.1700086968177,31.0408072809901));
#29270=CARTESIAN_POINT('Ctrl Pts',(31.925094792153,-16.1687449477339,31.041465759884));
#29271=CARTESIAN_POINT('Ctrl Pts',(31.8952919104888,-16.168011819419,31.0418477578044));
#29272=CARTESIAN_POINT('Ctrl Pts',(31.8646744620483,-16.1672513233696,31.0422439429542));
#29273=CARTESIAN_POINT('Ctrl Pts',(31.8329224323944,-16.1664582369103,31.0426570718779));
#29274=CARTESIAN_POINT('Ctrl Pts',(31.7319354368356,-16.1639358337881,31.0439710240642));
#29275=CARTESIAN_POINT('Ctrl Pts',(31.6284526822057,-16.1613063818566,31.0453389332579));
#29276=CARTESIAN_POINT('Ctrl Pts',(31.5232336354319,-16.1587277943726,31.0466795487252));
#29277=CARTESIAN_POINT('Ctrl Pts',(31.4188807866256,-16.156170434673,31.0480091278028));
#29278=CARTESIAN_POINT('Ctrl Pts',(31.3128198672035,-16.1536645426213,31.0493111005243));
#29279=CARTESIAN_POINT('Ctrl Pts',(31.2058402970424,-16.1513736799427,31.0505011542277));
#29280=CARTESIAN_POINT('Ctrl Pts',(31.1464339374063,-16.1501015509562,31.0511619977718));
#29281=CARTESIAN_POINT('Ctrl Pts',(31.086745188952,-16.1488957763821,31.051788304276));
#29282=CARTESIAN_POINT('Ctrl Pts',(31.0269161235859,-16.1477831210734,31.052366291213));
#29283=CARTESIAN_POINT('Ctrl Pts',(30.9223727403119,-16.1458389029967,31.0533762469848));
#29284=CARTESIAN_POINT('Ctrl Pts',(30.8173993541569,-16.1441811147896,31.0542375463396));
#29285=CARTESIAN_POINT('Ctrl Pts',(30.7129204018003,-16.1429541726495,31.0548748925162));
#29286=CARTESIAN_POINT('Ctrl Pts',(30.6397146645874,-16.1420944855847,31.0553214647269));
#29287=CARTESIAN_POINT('Ctrl Pts',(30.5667525557982,-16.1414458510595,31.0556583368409));
#29288=CARTESIAN_POINT('Ctrl Pts',(30.4943593393942,-16.1410459118957,31.0558660149161));
#29289=CARTESIAN_POINT('',(30.5,-18.7405179110273,29.559989655385));
#29290=CARTESIAN_POINT('Origin',(30.5,0.,0.));
#29291=CARTESIAN_POINT('Ctrl Pts',(30.5049791805003,-18.7395177484758,29.5605178050973));
#29292=CARTESIAN_POINT('Ctrl Pts',(30.5973676827744,-18.7400797009803,29.560162264643));
#29293=CARTESIAN_POINT('Ctrl Pts',(30.6891105694846,-18.7410567560113,29.559542510155));
#29294=CARTESIAN_POINT('Ctrl Pts',(30.7806774793081,-18.7423441244048,29.5587264396735));
#29295=CARTESIAN_POINT('Ctrl Pts',(30.8441888930629,-18.7432370516298,29.5581604077948));
#29296=CARTESIAN_POINT('Ctrl Pts',(30.9076166453417,-18.7442800408076,29.5574994222392));
#29297=CARTESIAN_POINT('Ctrl Pts',(30.971128809674,-18.7454455999911,29.5567612578201));
#29298=CARTESIAN_POINT('Ctrl Pts',(31.0735567068111,-18.7473253308648,29.5555707987956));
#29299=CARTESIAN_POINT('Ctrl Pts',(31.1762019082914,-18.7495231556641,29.5541800414699));
#29300=CARTESIAN_POINT('Ctrl Pts',(31.2798872709469,-18.7519033574722,29.5526737444515));
#29301=CARTESIAN_POINT('Ctrl Pts',(31.3828989348267,-18.7542680938472,29.5511772346436));
#29302=CARTESIAN_POINT('Ctrl Pts',(31.4869372222122,-18.756814411791,29.5495656759358));
#29303=CARTESIAN_POINT('Ctrl Pts',(31.5928574097442,-18.7594156373084,29.5479181178244));
#29304=CARTESIAN_POINT('Ctrl Pts',(31.6516459294303,-18.7608593866172,29.5470036792766));
#29305=CARTESIAN_POINT('Ctrl Pts',(31.7110150391215,-18.7623200347851,29.5460781618908));
#29306=CARTESIAN_POINT('Ctrl Pts',(31.7711176725243,-18.763774049131,29.5451562912556));
#29307=CARTESIAN_POINT('Ctrl Pts',(31.8409082760365,-18.7654624366936,29.5440858238842));
#29308=CARTESIAN_POINT('Ctrl Pts',(31.9056373311747,-18.7669933631241,29.5431152615715));
#29309=CARTESIAN_POINT('Ctrl Pts',(31.9658882086283,-18.7683675834941,29.5422441375119));
#29310=CARTESIAN_POINT('Ctrl Pts',(32.0341093482756,-18.7699235920325,29.5412577771694));
#29311=CARTESIAN_POINT('Ctrl Pts',(32.0965888127922,-18.7712796560443,29.5403982847666));
#29312=CARTESIAN_POINT('Ctrl Pts',(32.1542362617661,-18.7724634074923,29.5396480149485));
#29313=CARTESIAN_POINT('Ctrl Pts',(32.2151538519828,-18.773714309083,29.5388551849075));
#29314=CARTESIAN_POINT('Ctrl Pts',(32.2706761902186,-18.7747738843965,29.5381836213574));
#29315=CARTESIAN_POINT('Ctrl Pts',(32.3219402247755,-18.7756849339009,29.5376060245819));
#29316=CARTESIAN_POINT('Ctrl Pts',(32.3761674213235,-18.776648643858,29.536995041577));
#29317=CARTESIAN_POINT('Ctrl Pts',(32.4256304058823,-18.7774469218491,29.5364887148649));
#29318=CARTESIAN_POINT('Ctrl Pts',(32.4717350314044,-18.7781265619113,29.5360572749798));
#29319=CARTESIAN_POINT('Ctrl Pts',(32.5214923281234,-18.7788600469327,29.5355916539681));
#29320=CARTESIAN_POINT('Ctrl Pts',(32.5673384642507,-18.7794559410666,29.5352128774493));
#29321=CARTESIAN_POINT('Ctrl Pts',(32.6111004962912,-18.7799576530151,29.5348934788928));
#29322=CARTESIAN_POINT('Ctrl Pts',(32.6551147163156,-18.780462256185,29.5345722397345));
#29323=CARTESIAN_POINT('Ctrl Pts',(32.6970214084842,-18.7808718608789,29.5343108907558));
#29324=CARTESIAN_POINT('Ctrl Pts',(32.7387279964545,-18.7812095285095,29.5340950825232));
#29325=CARTESIAN_POINT('Ctrl Pts',(32.7800761354851,-18.7815442940421,29.5338811290631));
#29326=CARTESIAN_POINT('Ctrl Pts',(32.8212277342329,-18.7818087481603,29.5337116838824));
#29327=CARTESIAN_POINT('Ctrl Pts',(32.864082933751,-18.7820000955041,29.5335890251804));
#29328=CARTESIAN_POINT('Ctrl Pts',(32.903732033251,-18.7821771276952,29.5334755428695));
#29329=CARTESIAN_POINT('Ctrl Pts',(32.9448394203892,-18.7822919200911,29.5334018918637));
#29330=CARTESIAN_POINT('Ctrl Pts',(32.988943859822,-18.7823158450368,29.5333868654406));
#29331=CARTESIAN_POINT('Ctrl Pts',(32.9925102269236,-18.7823177796524,29.5333856503761));
#29332=CARTESIAN_POINT('Ctrl Pts',(32.996096210623,-18.7823191027633,29.5333848297968));
#29333=CARTESIAN_POINT('Ctrl Pts',(32.9997026353889,-18.7823197895506,29.5333844198654));
#29334=CARTESIAN_POINT('Ctrl Pts',(33.0361388185046,-18.782326728253,29.5333802782743));
#29335=CARTESIAN_POINT('Ctrl Pts',(33.0740002606605,-18.7823330770045,29.5333765562529));
#29336=CARTESIAN_POINT('Ctrl Pts',(33.1140504028668,-18.7823389179975,29.5333733966326));
#29337=CARTESIAN_POINT('Ctrl Pts',(33.2460690464808,-18.7823581718611,29.533362981469));
#29338=CARTESIAN_POINT('Ctrl Pts',(33.3720922029407,-18.782366189783,29.5333587011924));
#29339=CARTESIAN_POINT('Ctrl Pts',(33.4992849360726,-18.782373736073,29.5333546566756));
#29340=CARTESIAN_POINT('Ctrl Pts',(33.6626792864138,-18.7823834301894,29.5333494610079));
#29341=CARTESIAN_POINT('Ctrl Pts',(33.8280037294637,-18.7823923459959,29.5333446544026));
#29342=CARTESIAN_POINT('Ctrl Pts',(33.9928746198635,-18.7824059536077,29.5333373313073));
#29343=CARTESIAN_POINT('Ctrl Pts',(34.3226164006631,-18.7824331688313,29.5333226851165));
#29344=CARTESIAN_POINT('Ctrl Pts',(34.6505439708621,-18.7824791512759,29.5332979729652));
#29345=CARTESIAN_POINT('Ctrl Pts',(34.9791449252861,-18.7825099763789,29.5332814027049));
#29346=CARTESIAN_POINT('Ctrl Pts',(35.30774587971,-18.782540801482,29.5332648324445));
#29347=CARTESIAN_POINT('Ctrl Pts',(35.6370202183589,-18.7825564692435,29.5332564040752));
#29348=CARTESIAN_POINT('Ctrl Pts',(35.9661418060974,-18.7825697306317,29.5332492722835));
#29349=CARTESIAN_POINT('Ctrl Pts',(36.2952633938358,-18.7825829920199,29.5332421404918));
#29350=CARTESIAN_POINT('Ctrl Pts',(36.6242322306637,-18.7825938470347,29.5332363052777));
#29351=CARTESIAN_POINT('Ctrl Pts',(36.9531363303404,-18.7826154119861,29.5332247108411));
#29352=CARTESIAN_POINT('Ctrl Pts',(38.1022190076918,-18.7826907528289,29.5331842036954));
#29353=CARTESIAN_POINT('Ctrl Pts',(39.2505115204485,-18.782896816333,29.5330734009978));
#29354=CARTESIAN_POINT('Ctrl Pts',(40.400093943525,-18.7829477771169,29.533045998731));
#29355=CARTESIAN_POINT('Ctrl Pts',(6.89999999997365,-9.63452070648359,5.3678954269134));
#29356=CARTESIAN_POINT('Ctrl Pts',(6.99168932310453,-9.60499723839754,5.42175501956));
#29357=CARTESIAN_POINT('Ctrl Pts',(7.08383915760479,-9.57508016834563,5.47527828673705));
#29358=CARTESIAN_POINT('Ctrl Pts',(8.15762752947027,-9.22342495405908,6.09209251732962));
#29359=CARTESIAN_POINT('Ctrl Pts',(9.16608342448599,-8.84591675027098,6.61836595106259));
#29360=CARTESIAN_POINT('Ctrl Pts',(11.2535425311854,-8.09542754093136,7.53037930120419));
#29361=CARTESIAN_POINT('Ctrl Pts',(12.2577133097064,-7.70725001371761,7.91666449612081));
#29362=CARTESIAN_POINT('Ctrl Pts',(14.356433377742,-6.97440810645327,8.58141250110813));
#29363=CARTESIAN_POINT('Ctrl Pts',(15.3659105035251,-6.61345583116597,8.85322312286061));
#29364=CARTESIAN_POINT('Ctrl Pts',(17.4728641219044,-5.96623757129008,9.31281879192962));
#29365=CARTESIAN_POINT('Ctrl Pts',(18.4890996814195,-5.66020885204394,9.49384943617778));
#29366=CARTESIAN_POINT('Ctrl Pts',(19.8476172011441,-5.32865724601649,9.68599953593307));
#29367=CARTESIAN_POINT('Ctrl Pts',(20.3454889307686,-5.2093054291626,9.75195458239818));
#29368=CARTESIAN_POINT('Ctrl Pts',(21.3782040612024,-4.97678151322347,9.87366876552719));
#29369=CARTESIAN_POINT('Ctrl Pts',(22.1792648896895,-4.81935607344487,9.95072592994714));
#29370=CARTESIAN_POINT('Ctrl Pts',(22.8542621828909,-4.70591921690555,10.0067883222623));
#29371=CARTESIAN_POINT('Ctrl Pts',(23.1054579010968,-4.66456206383028,10.0267605301623));
#29372=CARTESIAN_POINT('Ctrl Pts',(23.6171513959785,-4.58448144656259,10.0644076466806));
#29373=CARTESIAN_POINT('Ctrl Pts',(24.1360713221937,-4.51012725444835,10.0979855598765));
#29374=CARTESIAN_POINT('Ctrl Pts',(24.6624927871864,-4.44285620865166,10.1277002159266));
#29375=CARTESIAN_POINT('Ctrl Pts',(25.1928168818088,-4.3809527171812,10.154786256444));
#29376=CARTESIAN_POINT('Ctrl Pts',(25.5948982287615,-4.34117176259643,10.1721457030179));
#29377=CARTESIAN_POINT('Ctrl Pts',(26.1232031889651,-4.29604941535507,10.1922876384417));
#29378=CARTESIAN_POINT('Ctrl Pts',(27.1768897027567,-4.2232612911204,10.2241871753182));
#29379=CARTESIAN_POINT('Ctrl Pts',(28.2111297865347,-4.19969555688313,10.2325109692973));
#29380=CARTESIAN_POINT('Ctrl Pts',(29.1277555719713,-4.17661492679514,10.2421056253618));
#29381=CARTESIAN_POINT('Ctrl Pts',(29.4767605677587,-4.1700561490002,10.2448788784735));
#29382=CARTESIAN_POINT('Ctrl Pts',(30.1601418995912,-4.16421367130872,10.2473221772452));
#29383=CARTESIAN_POINT('Ctrl Pts',(31.3500242312262,-4.16794387579264,10.2457563290907));
#29384=CARTESIAN_POINT('Ctrl Pts',(32.3461596131128,-4.18040640609126,10.2405791191157));
#29385=CARTESIAN_POINT('Ctrl Pts',(33.1614718826738,-4.18039330945984,10.2405840900447));
#29386=CARTESIAN_POINT('Ctrl Pts',(33.4925794155279,-4.18039253080268,10.2405841444578));
#29387=CARTESIAN_POINT('Ctrl Pts',(34.1499904318886,-4.18039030822715,10.2405848392549));
#29388=CARTESIAN_POINT('Ctrl Pts',(34.9738731541179,-4.18038393925505,10.2405865289644));
#29389=CARTESIAN_POINT('Ctrl Pts',(35.9612754428242,-4.18038119412748,10.2405873001735));
#29390=CARTESIAN_POINT('Ctrl Pts',(37.936646788162,-4.18037753677864,10.2405882857915));
#29391=CARTESIAN_POINT('Ctrl Pts',(39.5833333333333,-4.18035859466987,10.2405934798255));
#29392=CARTESIAN_POINT('Ctrl Pts',(40.9,-4.18035859466987,10.2405934798255));
#29393=CARTESIAN_POINT('Ctrl Pts',(6.71972576838711,-12.8464244365415,6.5764381714634));
#29394=CARTESIAN_POINT('Ctrl Pts',(6.81144220747046,-12.8102053989753,6.6482837686261));
#29395=CARTESIAN_POINT('Ctrl Pts',(6.90362823998598,-12.7734498343709,6.71971524922859));
#29396=CARTESIAN_POINT('Ctrl Pts',(7.97787811486329,-12.3410744046091,7.54294881554194));
#29397=CARTESIAN_POINT('Ctrl Pts',(8.98681832185142,-11.871220138602,8.24809748747637));
#29398=CARTESIAN_POINT('Ctrl Pts',(11.0806583453373,-10.9274240314556,9.47774891389534));
#29399=CARTESIAN_POINT('Ctrl Pts',(12.0862475175457,-10.4368998098018,10.0005505115845));
#29400=CARTESIAN_POINT('Ctrl Pts',(14.197639322261,-9.50280276487817,10.906656993414));
#29401=CARTESIAN_POINT('Ctrl Pts',(15.2100862637122,-9.0420363325472,11.2785931828498));
#29402=CARTESIAN_POINT('Ctrl Pts',(17.3364698493954,-8.20932952666153,11.9121957711898));
#29403=CARTESIAN_POINT('Ctrl Pts',(18.357279581038,-7.81594677169139,12.1627870018009));
#29404=CARTESIAN_POINT('Ctrl Pts',(19.7331217809845,-7.38628119283516,12.4307568384137));
#29405=CARTESIAN_POINT('Ctrl Pts',(20.2341927100358,-7.23233618870704,12.5225360922774));
#29406=CARTESIAN_POINT('Ctrl Pts',(21.2777139275316,-6.93114017240205,12.6928916013278));
#29407=CARTESIAN_POINT('Ctrl Pts',(22.0885637816418,-6.72673758680647,12.8012350092453));
#29408=CARTESIAN_POINT('Ctrl Pts',(22.7734874647764,-6.57909772915772,12.8801738355232));
#29409=CARTESIAN_POINT('Ctrl Pts',(23.0269571312139,-6.52549682636868,12.9082278965574));
#29410=CARTESIAN_POINT('Ctrl Pts',(23.5444618566097,-6.42148511325403,12.9612738268023));
#29411=CARTESIAN_POINT('Ctrl Pts',(24.0694383156461,-6.32485290039694,13.0087020921734));
#29412=CARTESIAN_POINT('Ctrl Pts',(24.6027295908464,-6.2373000813771,13.0507741241225));
#29413=CARTESIAN_POINT('Ctrl Pts',(25.1403192523141,-6.15667530541499,13.0891677302172));
#29414=CARTESIAN_POINT('Ctrl Pts',(25.5484689870706,-6.10479659087691,13.1137995888261));
#29415=CARTESIAN_POINT('Ctrl Pts',(26.0852808149067,-6.04589855121055,13.1423647911197));
#29416=CARTESIAN_POINT('Ctrl Pts',(27.1586857291269,-5.95074158602808,13.1877077660314));
#29417=CARTESIAN_POINT('Ctrl Pts',(28.1995312980844,-5.92039197700574,13.1995114624862));
#29418=CARTESIAN_POINT('Ctrl Pts',(29.1157533315888,-5.89061060808306,13.2130297822556));
#29419=CARTESIAN_POINT('Ctrl Pts',(29.4698938670486,-5.88204921070823,13.2169740538762));
#29420=CARTESIAN_POINT('Ctrl Pts',(30.1587234046998,-5.8744768355958,13.220429005539));
#29421=CARTESIAN_POINT('Ctrl Pts',(31.355731195606,-5.87931523414859,13.2182120926509));
#29422=CARTESIAN_POINT('Ctrl Pts',(32.350180243561,-5.89537176970751,13.2109234983782));
#29423=CARTESIAN_POINT('Ctrl Pts',(33.1605031382466,-5.89535013085609,13.2109314016452));
#29424=CARTESIAN_POINT('Ctrl Pts',(33.4922179295252,-5.89534881762644,13.2109314596682));
#29425=CARTESIAN_POINT('Ctrl Pts',(34.1493400019899,-5.89534512891168,13.2109325467447));
#29426=CARTESIAN_POINT('Ctrl Pts',(34.9735241318652,-5.89533452524069,13.2109351472382));
#29427=CARTESIAN_POINT('Ctrl Pts',(35.9608954520827,-5.89532995964262,13.2109363413972));
#29428=CARTESIAN_POINT('Ctrl Pts',(37.9363824842976,-5.8953238722353,13.2109378608691));
#29429=CARTESIAN_POINT('Ctrl Pts',(39.5833333333333,-5.89529235427929,13.2109458830841));
#29430=CARTESIAN_POINT('Ctrl Pts',(40.9,-5.89529235427929,13.2109458830841));
#29431=CARTESIAN_POINT('Ctrl Pts',(6.48177011792014,-20.336764848396,9.40621265917915));
#29432=CARTESIAN_POINT('Ctrl Pts',(6.57271435585528,-20.2851799357091,9.51911083717172));
#29433=CARTESIAN_POINT('Ctrl Pts',(6.66411141569866,-20.2327517601296,9.63139437446865));
#29434=CARTESIAN_POINT('Ctrl Pts',(7.73048017258431,-19.614616528956,10.9276768808967));
#29435=CARTESIAN_POINT('Ctrl Pts',(8.73292722985417,-18.9319609573801,12.0456324995184));
#29436=CARTESIAN_POINT('Ctrl Pts',(10.8102906905198,-17.5485371602851,14.0013807284478));
#29437=CARTESIAN_POINT('Ctrl Pts',(11.8125687231201,-16.8218444562665,14.8418955382559));
#29438=CARTESIAN_POINT('Ctrl Pts',(13.9177445864075,-15.4271303717407,16.3050153868123));
#29439=CARTESIAN_POINT('Ctrl Pts',(14.9296562678442,-14.7350649820735,16.9116612373854));
#29440=CARTESIAN_POINT('Ctrl Pts',(17.0680844879216,-13.4708635112562,17.9535844659564));
#29441=CARTESIAN_POINT('Ctrl Pts',(18.0932339179161,-12.8729609429,18.3688941094638));
#29442=CARTESIAN_POINT('Ctrl Pts',(19.4933464326809,-12.2099892645604,18.8183285494774));
#29443=CARTESIAN_POINT('Ctrl Pts',(19.9993272808496,-11.9744841299437,18.971430097181));
#29444=CARTESIAN_POINT('Ctrl Pts',(21.0600020168761,-11.5100300116438,19.2581324129064));
#29445=CARTESIAN_POINT('Ctrl Pts',(21.8888875769482,-11.1928649299996,19.4420158954032));
#29446=CARTESIAN_POINT('Ctrl Pts',(22.5933490549503,-10.962505511385,19.5764520117208));
#29447=CARTESIAN_POINT('Ctrl Pts',(22.8513437851799,-10.8796937171906,19.6238525927722));
#29448=CARTESIAN_POINT('Ctrl Pts',(23.3805933886566,-10.7182299385361,19.7139851739534));
#29449=CARTESIAN_POINT('Ctrl Pts',(23.9182257576784,-10.5680285062335,19.7948254980796));
#29450=CARTESIAN_POINT('Ctrl Pts',(24.4662138806867,-10.4315004891655,19.8668205194741));
#29451=CARTESIAN_POINT('Ctrl Pts',(25.0195744741822,-10.3055778221167,19.9326328666884));
#29452=CARTESIAN_POINT('Ctrl Pts',(25.4412458088222,-10.2242864909386,19.9749776253082));
#29453=CARTESIAN_POINT('Ctrl Pts',(25.9971983460992,-10.131797107587,20.0240850656221));
#29454=CARTESIAN_POINT('Ctrl Pts',(27.1157050405652,-9.98182332250462,20.102368552767));
#29455=CARTESIAN_POINT('Ctrl Pts',(28.1723100127449,-9.93573708068025,20.1222437541335));
#29456=CARTESIAN_POINT('Ctrl Pts',(29.0876106506766,-9.89029022572785,20.1449463132817));
#29457=CARTESIAN_POINT('Ctrl Pts',(29.4537207931442,-9.87684873205164,20.1517438988729));
#29458=CARTESIAN_POINT('Ctrl Pts',(30.1552759232946,-9.86516345924738,20.1576060163182));
#29459=CARTESIAN_POINT('Ctrl Pts',(31.368924127636,-9.87263514017793,20.1538463873917));
#29460=CARTESIAN_POINT('Ctrl Pts',(32.3594787154311,-9.89702302165624,20.1416711708076));
#29461=CARTESIAN_POINT('Ctrl Pts',(33.1581760188914,-9.89696607979067,20.1416983285705));
#29462=CARTESIAN_POINT('Ctrl Pts',(33.4913102145729,-9.89696201382195,20.1416998058431));
#29463=CARTESIAN_POINT('Ctrl Pts',(34.1477617736107,-9.89695193052414,20.1417043298969));
#29464=CARTESIAN_POINT('Ctrl Pts',(34.9726616332633,-9.89692218573783,20.1417171222835));
#29465=CARTESIAN_POINT('Ctrl Pts',(35.9599657908142,-9.89690948638392,20.1417226604566));
#29466=CARTESIAN_POINT('Ctrl Pts',(37.9357298104643,-9.89689244880616,20.1417300151411));
#29467=CARTESIAN_POINT('Ctrl Pts',(39.5833333333333,-9.8968044600346,20.1417681573542));
#29468=CARTESIAN_POINT('Ctrl Pts',(40.9,-9.8968044600346,20.1417681573542));
#29469=CARTESIAN_POINT('Ctrl Pts',(6.40644620858992,-27.7818319413302,12.3446157076951));
#29470=CARTESIAN_POINT('Ctrl Pts',(6.49686818484384,-27.7146057723315,12.4976194141968));
#29471=CARTESIAN_POINT('Ctrl Pts',(6.58771883172007,-27.6462615383487,12.6497754970257));
#29472=CARTESIAN_POINT('Ctrl Pts',(7.64885870107047,-26.8389674658771,14.4089312086777));
#29473=CARTESIAN_POINT('Ctrl Pts',(8.64786699401839,-25.9406999974138,15.9309901815184));
#29474=CARTESIAN_POINT('Ctrl Pts',(10.7071344443812,-24.1258468463739,18.5841088194585));
#29475=CARTESIAN_POINT('Ctrl Pts',(11.7059636153277,-23.1640388241121,19.7351568023896));
#29476=CARTESIAN_POINT('Ctrl Pts',(13.7894167134297,-21.32755345859,21.7274097031724));
#29477=CARTESIAN_POINT('Ctrl Pts',(14.7964804448639,-20.40896606215,22.5625068415354));
#29478=CARTESIAN_POINT('Ctrl Pts',(16.9150096963281,-18.734786787185,23.9923642448819));
#29479=CARTESIAN_POINT('Ctrl Pts',(17.9356563974909,-17.9376031564435,24.568778311437));
#29480=CARTESIAN_POINT('Ctrl Pts',(19.3316378726113,-17.0495061236355,25.1942531765859));
#29481=CARTESIAN_POINT('Ctrl Pts',(19.8373783148988,-16.733671277521,25.4080883980548));
#29482=CARTESIAN_POINT('Ctrl Pts',(20.8986146451321,-16.1088561234904,25.8097110946141));
#29483=CARTESIAN_POINT('Ctrl Pts',(21.7322089233615,-15.6790344990822,26.0695581056351));
#29484=CARTESIAN_POINT('Ctrl Pts',(22.4452152218927,-15.3644450466695,26.2607608176433));
#29485=CARTESIAN_POINT('Ctrl Pts',(22.7053175952387,-15.2520352575855,26.3278633535721));
#29486=CARTESIAN_POINT('Ctrl Pts',(23.2405350109147,-15.0319031635372,26.4560495577169));
#29487=CARTESIAN_POINT('Ctrl Pts',(23.7856351879594,-14.8265027181049,26.5714803865859));
#29488=CARTESIAN_POINT('Ctrl Pts',(24.3434088150882,-14.6389049166987,26.6748081507042));
#29489=CARTESIAN_POINT('Ctrl Pts',(24.9080926446007,-14.4653482504621,26.7695587595053));
#29490=CARTESIAN_POINT('Ctrl Pts',(25.3404979553364,-14.3526452692475,26.8308622015487));
#29491=CARTESIAN_POINT('Ctrl Pts',(25.9125607075504,-14.2239063651395,26.9021372597287));
#29492=CARTESIAN_POINT('Ctrl Pts',(27.0720378258712,-14.0136986134135,27.0165941086124));
#29493=CARTESIAN_POINT('Ctrl Pts',(28.1454151442859,-13.9518646781025,27.0445191043407));
#29494=CARTESIAN_POINT('Ctrl Pts',(29.0596751952944,-13.890725520751,27.0764264216485));
#29495=CARTESIAN_POINT('Ctrl Pts',(29.4376599373188,-13.8719255145712,27.0863532011149));
#29496=CARTESIAN_POINT('Ctrl Pts',(30.1519376760718,-13.855954576287,27.0947220176404));
#29497=CARTESIAN_POINT('Ctrl Pts',(31.3821999577689,-13.8661782937677,27.0893514143297));
#29498=CARTESIAN_POINT('Ctrl Pts',(32.3688386893657,-13.8987881217581,27.0723527225427));
#29499=CARTESIAN_POINT('Ctrl Pts',(33.1558986739574,-13.8986675947835,27.0724155351932));
#29500=CARTESIAN_POINT('Ctrl Pts',(33.49045038666,-13.8986584195583,27.072419804706));
#29501=CARTESIAN_POINT('Ctrl Pts',(34.1462287076184,-13.8986367255002,27.0724307945236));
#29502=CARTESIAN_POINT('Ctrl Pts',(34.9718350023128,-13.8985720488061,27.0724629552156));
#29503=CARTESIAN_POINT('Ctrl Pts',(35.9590682028415,-13.8985445297568,27.0724767217601));
#29504=CARTESIAN_POINT('Ctrl Pts',(37.9351039480424,-13.8985075170899,27.072495155898));
#29505=CARTESIAN_POINT('Ctrl Pts',(39.5833333333333,-13.8983165657899,27.0725904316243));
#29506=CARTESIAN_POINT('Ctrl Pts',(40.9,-13.8983165657899,27.0725904316243));
#29507=CARTESIAN_POINT('Ctrl Pts',(6.37427268165564,-32.0290848932163,14.0406695266741));
#29508=CARTESIAN_POINT('Ctrl Pts',(6.46448755772839,-31.9528098065586,14.2166050753401));
#29509=CARTESIAN_POINT('Ctrl Pts',(6.55512327887566,-31.8752581000468,14.3915605358513));
#29510=CARTESIAN_POINT('Ctrl Pts',(7.61410360785656,-30.958672886913,16.4151695040826));
#29511=CARTESIAN_POINT('Ctrl Pts',(8.61142775869687,-29.9361952854453,18.1677152487792));
#29512=CARTESIAN_POINT('Ctrl Pts',(10.6634825022472,-27.8730682250753,21.2183968262284));
#29513=CARTESIAN_POINT('Ctrl Pts',(11.6607542873627,-26.7761583709752,22.5462154536683));
#29514=CARTESIAN_POINT('Ctrl Pts',(13.7353039743977,-24.6873364683673,24.8383185913233));
#29515=CARTESIAN_POINT('Ctrl Pts',(14.7402095633116,-23.6392130729629,25.8029859119439));
#29516=CARTESIAN_POINT('Ctrl Pts',(16.8490881066137,-21.733995182915,27.450307490631));
#29517=CARTESIAN_POINT('Ctrl Pts',(17.8672038783315,-20.8239061433235,28.117536242687));
#29518=CARTESIAN_POINT('Ctrl Pts',(19.2585933984997,-19.811022849419,28.8404836901117));
#29519=CARTESIAN_POINT('Ctrl Pts',(19.7636418533908,-19.4499572035579,29.0884650342026));
#29520=CARTESIAN_POINT('Ctrl Pts',(20.8231816497994,-18.7357747989968,29.5540603372584));
#29521=CARTESIAN_POINT('Ctrl Pts',(21.6568670511735,-18.2431916560479,29.8562628482713));
#29522=CARTESIAN_POINT('Ctrl Pts',(22.3720072062877,-17.8815051531588,30.0792593376712));
#29523=CARTESIAN_POINT('Ctrl Pts',(22.6326824787813,-17.7523977438432,30.1574913312728));
#29524=CARTESIAN_POINT('Ctrl Pts',(23.1697036949937,-17.4991937768336,30.3071564102286));
#29525=CARTESIAN_POINT('Ctrl Pts',(23.7174377716562,-17.2625030946595,30.4422233412819));
#29526=CARTESIAN_POINT('Ctrl Pts',(24.2790946262572,-17.0457855087881,30.5634410393029));
#29527=CARTESIAN_POINT('Ctrl Pts',(24.8485847331463,-16.8449230908939,30.6748008187179));
#29528=CARTESIAN_POINT('Ctrl Pts',(25.2859632686137,-16.714000734413,30.7471152582869));
#29529=CARTESIAN_POINT('Ctrl Pts',(25.8659001690755,-16.5640760155963,30.8313513860032));
#29530=CARTESIAN_POINT('Ctrl Pts',(27.0467877055032,-16.3181083484215,30.9672841404844));
#29531=CARTESIAN_POINT('Ctrl Pts',(28.1301993946288,-16.2470842981322,30.9999203594232));
#29532=CARTESIAN_POINT('Ctrl Pts',(29.0438132065911,-16.1769735529556,31.0370949113971));
#29533=CARTESIAN_POINT('Ctrl Pts',(29.4285323170642,-16.1549555741443,31.0489002942269));
#29534=CARTESIAN_POINT('Ctrl Pts',(30.1500796604944,-16.1364761766636,31.0587367393328));
#29535=CARTESIAN_POINT('Ctrl Pts',(31.3898224001987,-16.1483068856791,31.0524272220083));
#29536=CARTESIAN_POINT('Ctrl Pts',(32.3742147772173,-16.1855693458549,31.0327017051641));
#29537=CARTESIAN_POINT('Ctrl Pts',(33.1546196294426,-16.1853991323255,31.0327939306214));
#29538=CARTESIAN_POINT('Ctrl Pts',(33.4899805045662,-16.185385634532,31.0328008093452));
#29539=CARTESIAN_POINT('Ctrl Pts',(34.1453728987309,-16.1853546639146,31.0328173216774));
#29540=CARTESIAN_POINT('Ctrl Pts',(34.9713787068036,-16.1852616946182,31.0328663827335));
#29541=CARTESIAN_POINT('Ctrl Pts',(35.9585696612047,-16.1852222245757,31.0328872804502));
#29542=CARTESIAN_POINT('Ctrl Pts',(37.9347583211501,-16.1851690519237,31.0329153648958));
#29543=CARTESIAN_POINT('Ctrl Pts',(39.5833333333333,-16.1848949119358,31.0330603026358));
#29544=CARTESIAN_POINT('Ctrl Pts',(40.9,-16.1848949119358,31.0330603026358));
#29545=CARTESIAN_POINT('',(40.9,-15.1839076262003,29.2992994660114));
#29546=CARTESIAN_POINT('Ctrl Pts',(40.9,-15.1839076262003,29.2992994660114));
#29547=CARTESIAN_POINT('Ctrl Pts',(40.9,-15.4341550287793,29.7327406817405));
#29548=CARTESIAN_POINT('Ctrl Pts',(40.9,-15.6844024313584,30.1661818974696));
#29549=CARTESIAN_POINT('Ctrl Pts',(40.9,-15.9346498339374,30.5996231131986));
#29550=CARTESIAN_POINT('',(38.,-15.1839076262003,29.2992994660114));
#29551=CARTESIAN_POINT('Ctrl Pts',(38.,-15.1839076262003,29.2992994660114));
#29552=CARTESIAN_POINT('Ctrl Pts',(38.9666666666667,-15.1839076262003,29.2992994660114));
#29553=CARTESIAN_POINT('Ctrl Pts',(39.9333333333333,-15.1839076262003,29.2992994660114));
#29554=CARTESIAN_POINT('Ctrl Pts',(40.9,-15.1839076262003,29.2992994660114));
#29555=CARTESIAN_POINT('Ctrl Pts',(37.4974382384971,-14.8838038109906,28.7790269720418));
#29556=CARTESIAN_POINT('Ctrl Pts',(37.6645213547142,-14.9840691120817,28.9527098777876));
#29557=CARTESIAN_POINT('Ctrl Pts',(37.8313739960413,-15.0841847150558,29.1261374112001));
#29558=CARTESIAN_POINT('Ctrl Pts',(37.9978889629903,-15.1840905833949,29.2992044501375));
#29559=CARTESIAN_POINT('',(6.9,-27.0393531365015,12.9951291628659));
#29560=CARTESIAN_POINT('Ctrl Pts',(6.9,-27.0393531365015,12.9951291628659));
#29561=CARTESIAN_POINT('Ctrl Pts',(6.9,-24.649274247254,11.9174419758914));
#29562=CARTESIAN_POINT('Ctrl Pts',(6.90000000000115,-22.230729924082,10.8339866674746));
#29563=CARTESIAN_POINT('Ctrl Pts',(6.90000000000115,-16.7584145047598,8.41000082059024));
#29564=CARTESIAN_POINT('Ctrl Pts',(6.9,-13.1312177506378,6.82522008706163));
#29565=CARTESIAN_POINT('Ctrl Pts',(6.9,-9.63452070648529,5.36789542693312));
#29566=CARTESIAN_POINT('',(22.9245129145126,-15.8853026165582,27.5141512254857));
#29567=CARTESIAN_POINT('Ctrl Pts',(22.9245129145126,-15.8853026165582,27.5141512254857));
#29568=CARTESIAN_POINT('Ctrl Pts',(22.7202811020963,-15.9355315703924,27.405303612937));
#29569=CARTESIAN_POINT('Ctrl Pts',(22.5089075447093,-15.9922246435191,27.2924652433825));
#29570=CARTESIAN_POINT('Ctrl Pts',(22.2913349439917,-16.0558281873747,27.1762359097413));
#29571=CARTESIAN_POINT('Ctrl Pts',(21.4451770585293,-16.3031876434794,26.7242103933932));
#29572=CARTESIAN_POINT('Ctrl Pts',(20.5220951556669,-16.6965145338605,26.2108400614943));
#29573=CARTESIAN_POINT('Ctrl Pts',(19.767142881954,-17.0753616782143,25.777085937268));
#29574=CARTESIAN_POINT('Ctrl Pts',(19.5194773058392,-17.1996442316059,25.634790895834));
#29575=CARTESIAN_POINT('Ctrl Pts',(19.2865716386091,-17.3225345039426,25.4994131575072));
#29576=CARTESIAN_POINT('Ctrl Pts',(19.0728538401323,-17.4387046858284,25.3740784559106));
#29577=CARTESIAN_POINT('Ctrl Pts',(18.7028555998035,-17.6398239336529,25.15709316328));
#29578=CARTESIAN_POINT('Ctrl Pts',(18.4144703596235,-17.8106758656205,24.9815167506411));
#29579=CARTESIAN_POINT('Ctrl Pts',(18.0642874871537,-18.0298340093775,24.7606238748751));
#29580=CARTESIAN_POINT('Ctrl Pts',(17.4420927116721,-18.4192278454841,24.3681478172274));
#29581=CARTESIAN_POINT('Ctrl Pts',(16.7224564418218,-18.9163953124275,23.8866996305775));
#29582=CARTESIAN_POINT('Ctrl Pts',(15.9202806616111,-19.5075155171573,23.2999769887242));
#29583=CARTESIAN_POINT('Ctrl Pts',(15.409052983452,-19.8842371999007,22.926057878577));
#29584=CARTESIAN_POINT('Ctrl Pts',(14.8739602945718,-20.3065653819879,22.5035099772299));
#29585=CARTESIAN_POINT('Ctrl Pts',(14.316979433116,-20.764045054618,22.0244589523046));
#29586=CARTESIAN_POINT('Ctrl Pts',(13.886420676284,-21.1176871503423,21.6541417151704));
#29587=CARTESIAN_POINT('Ctrl Pts',(13.3867890027807,-21.5394320189423,21.2019814327446));
#29588=CARTESIAN_POINT('Ctrl Pts',(12.8146824059514,-22.0238946695559,20.6456427149589));
#29589=CARTESIAN_POINT('Ctrl Pts',(12.2526665517595,-22.499812430193,20.0991166279862));
#29590=CARTESIAN_POINT('Ctrl Pts',(11.6379478462803,-23.0419154065947,19.44703563439));
#29591=CARTESIAN_POINT('Ctrl Pts',(10.9739250490308,-23.626535453056,18.6689137476991));
#29592=CARTESIAN_POINT('Ctrl Pts',(10.5683455447963,-23.9836164291782,18.1936434853748));
#29593=CARTESIAN_POINT('Ctrl Pts',(10.1437415406956,-24.3558958755273,17.6694303965612));
#29594=CARTESIAN_POINT('Ctrl Pts',(9.74137929176525,-24.6998029803349,17.1528053766524));
#29595=CARTESIAN_POINT('Ctrl Pts',(8.72285779294234,-25.5703537856744,15.8450442956717));
#29596=CARTESIAN_POINT('Ctrl Pts',(7.81323138778195,-26.3485431508901,14.4751178145147));
#29597=CARTESIAN_POINT('Ctrl Pts',(6.9,-27.0393531365015,12.9951291628659));
#29598=CARTESIAN_POINT('Ctrl Pts',(30.5,-16.1402285275843,31.0562879796886));
#29599=CARTESIAN_POINT('Ctrl Pts',(29.9560179420817,-16.0158030554221,30.8470467059701));
#29600=CARTESIAN_POINT('Ctrl Pts',(29.4152668325132,-15.9055856438304,30.6299015220344));
#29601=CARTESIAN_POINT('Ctrl Pts',(28.8740459957565,-15.8236145009996,30.3967092920472));
#29602=CARTESIAN_POINT('Ctrl Pts',(28.353527792344,-15.7447788961961,30.1724370682909));
#29603=CARTESIAN_POINT('Ctrl Pts',(27.8179515912467,-15.65999396651,29.9423746730404));
#29604=CARTESIAN_POINT('Ctrl Pts',(27.2695051149491,-15.5981844167478,29.6962958928787));
#29605=CARTESIAN_POINT('Ctrl Pts',(26.9554553615883,-15.5627912203338,29.5553870101399));
#29606=CARTESIAN_POINT('Ctrl Pts',(26.6378099296971,-15.5350208970661,29.4095747645068));
#29607=CARTESIAN_POINT('Ctrl Pts',(26.3179304017917,-15.5205235030951,29.2578762499931));
#29608=CARTESIAN_POINT('Ctrl Pts',(26.1078196745982,-15.5110009868853,29.1582340959379));
#29609=CARTESIAN_POINT('Ctrl Pts',(25.8967402232745,-15.507207179043,29.0560612282453));
#29610=CARTESIAN_POINT('Ctrl Pts',(25.6850706236774,-15.5107635234098,28.9510881944939));
#29611=CARTESIAN_POINT('Ctrl Pts',(25.6562210027417,-15.5112482372614,28.9367808388889));
#29612=CARTESIAN_POINT('Ctrl Pts',(25.6277737638215,-15.5118582602788,28.9226278510966));
#29613=CARTESIAN_POINT('Ctrl Pts',(25.5983858063598,-15.5126342200129,28.9079571471847));
#29614=CARTESIAN_POINT('Ctrl Pts',(25.1249357452756,-15.5251351971226,28.6716070819486));
#29615=CARTESIAN_POINT('Ctrl Pts',(24.1510084067019,-15.5836572228941,28.1678256190434));
#29616=CARTESIAN_POINT('Ctrl Pts',(22.9245129145126,-15.8853026165582,27.5141512254857));
#29617=CARTESIAN_POINT('Origin',(40.65,0.,0.));
#29618=CARTESIAN_POINT('',(40.4,-31.0330398077868,16.1848830792292));
#29619=CARTESIAN_POINT('',(40.9,-30.5996231131986,15.9346498339374));
#29620=CARTESIAN_POINT('Ctrl Pts',(40.4,-31.0330398077868,16.1848830792292));
#29621=CARTESIAN_POINT('Ctrl Pts',(40.5666590129021,-30.8885761371497,16.1014769400988));
#29622=CARTESIAN_POINT('Ctrl Pts',(40.7333430446799,-30.7440888809087,16.0180571838136));
#29623=CARTESIAN_POINT('Ctrl Pts',(40.9,-30.5996231131986,15.9346498339374));
#29624=CARTESIAN_POINT('',(40.9,-29.0996231131986,18.5327260452908));
#29625=CARTESIAN_POINT('Origin',(40.9,0.,0.));
#29626=CARTESIAN_POINT('',(40.4,-29.5330398077868,18.7829592905825));
#29627=CARTESIAN_POINT('Ctrl Pts',(40.9,-29.0996231131986,18.5327260452908));
#29628=CARTESIAN_POINT('Ctrl Pts',(40.7333430444293,-29.244088881126,18.6161333952923));
#29629=CARTESIAN_POINT('Ctrl Pts',(40.5666590126687,-29.3885761373521,18.6995531515689));
#29630=CARTESIAN_POINT('Ctrl Pts',(40.4,-29.5330398077868,18.7829592905825));
#29631=CARTESIAN_POINT('Origin',(40.4,0.,0.));
#29632=CARTESIAN_POINT('Origin',(35.7,0.,0.));
#29633=CARTESIAN_POINT('',(30.5,-29.5059919176187,18.8254200738635));
#29634=CARTESIAN_POINT('Ctrl Pts',(40.3998805977094,-29.5330468723883,18.7829479019245));
#29635=CARTESIAN_POINT('Ctrl Pts',(39.2493532038211,-29.5330781202017,18.7828975281218));
#29636=CARTESIAN_POINT('Ctrl Pts',(38.0972325173324,-29.5332042421652,18.7826942098493));
#29637=CARTESIAN_POINT('Ctrl Pts',(36.9466403233753,-29.5332467931519,18.7826256101695));
#29638=CARTESIAN_POINT('Ctrl Pts',(36.7453942973752,-29.533254235595,18.7826136116412));
#29639=CARTESIAN_POINT('Ctrl Pts',(36.5441950314395,-29.5332591214118,18.7826057344612));
#29640=CARTESIAN_POINT('Ctrl Pts',(36.3429831482115,-29.5332638326535,18.7825981392431));
#29641=CARTESIAN_POINT('Ctrl Pts',(36.2103627229288,-29.533266937872,18.7825931331717));
#29642=CARTESIAN_POINT('Ctrl Pts',(36.0823539050873,-29.5332699079824,18.7825884046388));
#29643=CARTESIAN_POINT('Ctrl Pts',(35.9587472612551,-29.533273304022,18.7825830315924));
#29644=CARTESIAN_POINT('Ctrl Pts',(35.7554552092488,-29.5332788893841,18.7825741947079));
#29645=CARTESIAN_POINT('Ctrl Pts',(35.5640774641664,-29.5332855100166,18.78256380265));
#29646=CARTESIAN_POINT('Ctrl Pts',(35.3838244599901,-29.5332919882698,18.7825536727525));
#29647=CARTESIAN_POINT('Ctrl Pts',(35.2391029659002,-29.5332971895284,18.7825455396624));
#29648=CARTESIAN_POINT('Ctrl Pts',(35.1015509582746,-29.5333023181163,18.7825375448068));
#29649=CARTESIAN_POINT('Ctrl Pts',(34.970735999324,-29.5333070397951,18.7825301856736));
#29650=CARTESIAN_POINT('Ctrl Pts',(34.857898178191,-29.533311112601,18.7825238378632));
#29651=CARTESIAN_POINT('Ctrl Pts',(34.7500670454289,-29.5333148977242,18.7825179389498));
#29652=CARTESIAN_POINT('Ctrl Pts',(34.6468496335934,-29.5333184739771,18.7825123391461));
#29653=CARTESIAN_POINT('Ctrl Pts',(34.5887227637577,-29.5333204879433,18.7825091856175));
#29654=CARTESIAN_POINT('Ctrl Pts',(34.5320601650214,-29.5333224349754,18.7825061280289));
#29655=CARTESIAN_POINT('Ctrl Pts',(34.4767987085013,-29.53332432459,18.7825031467392));
#29656=CARTESIAN_POINT('Ctrl Pts',(34.3959515550965,-29.5333270890838,18.7824987851317));
#29657=CARTESIAN_POINT('Ctrl Pts',(34.3181086378963,-29.533329735084,18.7824945795527));
#29658=CARTESIAN_POINT('Ctrl Pts',(34.2432236356273,-29.5333323757695,18.7824903288468));
#29659=CARTESIAN_POINT('Ctrl Pts',(34.162267530415,-29.5333352305416,18.7824857335262));
#29660=CARTESIAN_POINT('Ctrl Pts',(34.0847679659787,-29.5333380786013,18.7824810862876));
#29661=CARTESIAN_POINT('Ctrl Pts',(34.0106064145146,-29.5333409984257,18.7824762390846));
#29662=CARTESIAN_POINT('Ctrl Pts',(34.0011740963656,-29.5333413697867,18.7824756225878));
#29663=CARTESIAN_POINT('Ctrl Pts',(33.9917957065319,-29.5333417422357,18.7824750029764));
#29664=CARTESIAN_POINT('Ctrl Pts',(33.982470944213,-29.5333421158732,18.7824743800457));
#29665=CARTESIAN_POINT('Ctrl Pts',(33.9223617768103,-29.533344524411,18.7824703645173));
#29666=CARTESIAN_POINT('Ctrl Pts',(33.8644761963964,-29.5333469783619,18.7824662176402));
#29667=CARTESIAN_POINT('Ctrl Pts',(33.8085662291514,-29.5333493560496,18.7824621300573));
#29668=CARTESIAN_POINT('Ctrl Pts',(33.7474237015737,-29.5333519562627,18.7824576599214));
#29669=CARTESIAN_POINT('Ctrl Pts',(33.6886441629424,-29.5333544654644,18.7824532603738));
#29670=CARTESIAN_POINT('Ctrl Pts',(33.6319696815246,-29.5333567795574,18.7824490897141));
#29671=CARTESIAN_POINT('Ctrl Pts',(33.5826925637263,-29.5333587916063,18.7824454634244));
#29672=CARTESIAN_POINT('Ctrl Pts',(33.5350083428651,-29.5333606573844,18.7824420081377));
#29673=CARTESIAN_POINT('Ctrl Pts',(33.4887791610293,-29.5333623350578,18.7824387839385));
#29674=CARTESIAN_POINT('Ctrl Pts',(33.4518540159975,-29.5333636750843,18.7824362086383));
#29675=CARTESIAN_POINT('Ctrl Pts',(33.4158630418951,-29.5333649012576,18.7824337706412));
#29676=CARTESIAN_POINT('Ctrl Pts',(33.3809178973936,-29.5333661853239,18.7824311829815));
#29677=CARTESIAN_POINT('Ctrl Pts',(33.3430135141807,-29.533367578128,18.7824283761925));
#29678=CARTESIAN_POINT('Ctrl Pts',(33.3063394413795,-29.533369038868,18.7824253936111));
#29679=CARTESIAN_POINT('Ctrl Pts',(33.2709744549997,-29.5333707165148,18.782421984424));
#29680=CARTESIAN_POINT('Ctrl Pts',(33.2337091833705,-29.5333724843074,18.7824183920493));
#29681=CARTESIAN_POINT('Ctrl Pts',(33.1978968817061,-29.5333744922841,18.7824143270743));
#29682=CARTESIAN_POINT('Ctrl Pts',(33.163568044013,-29.5333768470907,18.7824096072586));
#29683=CARTESIAN_POINT('Ctrl Pts',(33.1258517952642,-29.5333794342588,18.7824044217133));
#29684=CARTESIAN_POINT('Ctrl Pts',(33.0899258346466,-29.5333824396273,18.7823984464624));
#29685=CARTESIAN_POINT('Ctrl Pts',(33.0557653924644,-29.5333859335647,18.782391556659));
#29686=CARTESIAN_POINT('Ctrl Pts',(33.0368719876726,-29.5333878659862,18.7823877460571));
#29687=CARTESIAN_POINT('Ctrl Pts',(33.0185175726609,-29.5333899466912,18.7823836576175));
#29688=CARTESIAN_POINT('Ctrl Pts',(33.0006913488414,-29.533392180445,18.7823792819583));
#29689=CARTESIAN_POINT('Ctrl Pts',(32.9433364917302,-29.5333993674205,18.782365203525));
#29690=CARTESIAN_POINT('Ctrl Pts',(32.8893232017973,-29.5332829792511,18.7825476275079));
#29691=CARTESIAN_POINT('Ctrl Pts',(32.8382230275391,-29.5330947066424,18.7828441878577));
#29692=CARTESIAN_POINT('Ctrl Pts',(32.7810653123535,-29.5328841157333,18.7831759032042));
#29693=CARTESIAN_POINT('Ctrl Pts',(32.7275524566169,-29.532583390884,18.783650731462));
#29694=CARTESIAN_POINT('Ctrl Pts',(32.6770430178928,-29.5322363386496,18.7841988325575));
#29695=CARTESIAN_POINT('Ctrl Pts',(32.6227203151,-29.5318630853359,18.7847883131312));
#29696=CARTESIAN_POINT('Ctrl Pts',(32.5718714570977,-29.5314358212365,18.7854632228815));
#29697=CARTESIAN_POINT('Ctrl Pts',(32.5236533104256,-29.5309832901803,18.7861776881423));
#29698=CARTESIAN_POINT('Ctrl Pts',(32.4718100170294,-29.5304967368402,18.7869458684789));
#29699=CARTESIAN_POINT('Ctrl Pts',(32.4230076636111,-29.5299805545515,18.787760443828));
#29700=CARTESIAN_POINT('Ctrl Pts',(32.3761512171934,-29.5294487411367,18.7885990065863));
#29701=CARTESIAN_POINT('Ctrl Pts',(32.3248096591137,-29.5288660223986,18.7895178367975));
#29702=CARTESIAN_POINT('Ctrl Pts',(32.275804395008,-29.5282641700436,18.7904660498706));
#29703=CARTESIAN_POINT('Ctrl Pts',(32.2276418899935,-29.5276429422446,18.7914438965952));
#29704=CARTESIAN_POINT('Ctrl Pts',(32.1780484879536,-29.5270032579094,18.7924507949227));
#29705=CARTESIAN_POINT('Ctrl Pts',(32.1293485207497,-29.5263425803878,18.7934898288216));
#29706=CARTESIAN_POINT('Ctrl Pts',(32.0798596721975,-29.5256485080419,18.7945806299648));
#29707=CARTESIAN_POINT('Ctrl Pts',(32.0310319727755,-29.5249637081956,18.7956568584871));
#29708=CARTESIAN_POINT('Ctrl Pts',(31.9814363679959,-29.5242459918056,18.7967841293549));
#29709=CARTESIAN_POINT('Ctrl Pts',(31.9294088356327,-29.5234781937104,18.7979897024648));
#29710=CARTESIAN_POINT('Ctrl Pts',(31.8980169361537,-29.523014926676,18.7987171102077));
#29711=CARTESIAN_POINT('Ctrl Pts',(31.8657387723057,-29.5225333465275,18.7994731533958));
#29712=CARTESIAN_POINT('Ctrl Pts',(31.8321995506891,-29.5220297162343,18.8002637757389));
#29713=CARTESIAN_POINT('Ctrl Pts',(31.7313430769548,-29.5205152393626,18.8026412722264));
#29714=CARTESIAN_POINT('Ctrl Pts',(31.6280303063015,-29.5189339811,18.8051208616255));
#29715=CARTESIAN_POINT('Ctrl Pts',(31.5230436306592,-29.5173797888792,18.8075570016556));
#29716=CARTESIAN_POINT('Ctrl Pts',(31.4165412834618,-29.5158031590973,18.8100283117502));
#29717=CARTESIAN_POINT('Ctrl Pts',(31.3083161799734,-29.5142552687721,18.8124534992282));
#29718=CARTESIAN_POINT('Ctrl Pts',(31.1992361907463,-29.5128402023347,18.8146708525443));
#29719=CARTESIAN_POINT('Ctrl Pts',(31.1417800802781,-29.5120948391006,18.815838807345));
#29720=CARTESIAN_POINT('Ctrl Pts',(31.0840876501124,-29.5113863470818,18.816949067126));
#29721=CARTESIAN_POINT('Ctrl Pts',(31.02629146246,-29.5107292754508,18.817979046424));
#29722=CARTESIAN_POINT('Ctrl Pts',(30.9238422517517,-29.5095645538193,18.8198047821761));
#29723=CARTESIAN_POINT('Ctrl Pts',(30.8210652493993,-29.5085625954711,18.8213763518943));
#29724=CARTESIAN_POINT('Ctrl Pts',(30.7187655025438,-29.5078108353849,18.8225556928751));
#29725=CARTESIAN_POINT('Ctrl Pts',(30.6466529304574,-29.5072809088203,18.8233870274004));
#29726=CARTESIAN_POINT('Ctrl Pts',(30.5747782878161,-29.5068750511296,18.8240238694395));
#29727=CARTESIAN_POINT('Ctrl Pts',(30.5034323931868,-29.5066169475224,18.824428995823));
#29728=CARTESIAN_POINT('Ctrl Pts',(30.5006731165971,-29.506606965459,18.8244446639389));
#29729=CARTESIAN_POINT('Ctrl Pts',(30.4979146316512,-29.5065972035125,18.82445998689));
#29730=CARTESIAN_POINT('Ctrl Pts',(30.4951569508122,-29.5065876629556,18.8244749626663));
#29731=CARTESIAN_POINT('',(30.5,-31.0097594187194,16.229443021655));
#29732=CARTESIAN_POINT('Origin',(30.5,0.,0.));
#29733=CARTESIAN_POINT('Ctrl Pts',(30.5049076308142,-31.009123868732,16.2304573503027));
#29734=CARTESIAN_POINT('Ctrl Pts',(30.5973062294346,-31.0094328533549,16.2298682766553));
#29735=CARTESIAN_POINT('Ctrl Pts',(30.6890591585861,-31.009969267703,16.2288427503287));
#29736=CARTESIAN_POINT('Ctrl Pts',(30.780636436492,-31.0106763092386,16.2274919709622));
#29737=CARTESIAN_POINT('Ctrl Pts',(30.8441456090293,-31.0111666450937,16.2265552005995));
#29738=CARTESIAN_POINT('Ctrl Pts',(30.9075713010185,-31.0117394593185,16.2254611740685));
#29739=CARTESIAN_POINT('Ctrl Pts',(30.9710816356705,-31.012379837551,16.2242390174925));
#29740=CARTESIAN_POINT('Ctrl Pts',(31.0734991469997,-31.0134125190072,16.2222681534488));
#29741=CARTESIAN_POINT('Ctrl Pts',(31.1761345288069,-31.0146205155169,16.2199648111637));
#29742=CARTESIAN_POINT('Ctrl Pts',(31.2798100568472,-31.0159286966546,16.2174702047239));
#29743=CARTESIAN_POINT('Ctrl Pts',(31.382832629713,-31.017228638783,16.2149913094767));
#29744=CARTESIAN_POINT('Ctrl Pts',(31.4868822244331,-31.0186283615543,16.2123218973815));
#29745=CARTESIAN_POINT('Ctrl Pts',(31.5928140565593,-31.0200576696061,16.2095937955791));
#29746=CARTESIAN_POINT('Ctrl Pts',(31.6516194621104,-31.0208511142012,16.2080793581371));
#29747=CARTESIAN_POINT('Ctrl Pts',(31.7110057676088,-31.0216536678952,16.2065468518028));
#29748=CARTESIAN_POINT('Ctrl Pts',(31.771125977653,-31.0224523036439,16.205020814195));
#29749=CARTESIAN_POINT('Ctrl Pts',(31.8409078613428,-31.023379284885,16.2032495333099));
#29750=CARTESIAN_POINT('Ctrl Pts',(31.9056298453965,-31.0242198767435,16.2016434584278));
#29751=CARTESIAN_POINT('Ctrl Pts',(31.9658749467866,-31.0249744961547,16.2002018139143));
#29752=CARTESIAN_POINT('Ctrl Pts',(32.0341046687229,-31.025829129501,16.198569100183));
#29753=CARTESIAN_POINT('Ctrl Pts',(32.0965918298942,-31.0265740158191,16.1971462744692));
#29754=CARTESIAN_POINT('Ctrl Pts',(32.1542461945015,-31.0272242625031,16.195904238954));
#29755=CARTESIAN_POINT('Ctrl Pts',(32.2151665953522,-31.0279113447197,16.1945918439259));
#29756=CARTESIAN_POINT('Ctrl Pts',(32.2706916712566,-31.0284933558528,16.1934801514052));
#29757=CARTESIAN_POINT('Ctrl Pts',(32.3219582775166,-31.0289937114783,16.1925241206213));
#29758=CARTESIAN_POINT('Ctrl Pts',(32.3761916324787,-31.0295230221977,16.1915127652646));
#29759=CARTESIAN_POINT('Ctrl Pts',(32.4256599862244,-31.0299613681538,16.1906748064836));
#29760=CARTESIAN_POINT('Ctrl Pts',(32.4717693483807,-31.0303343957025,16.1899610544419));
#29761=CARTESIAN_POINT('Ctrl Pts',(32.5215332003086,-31.030736988296,16.1891907325537));
#29762=CARTESIAN_POINT('Ctrl Pts',(32.5673849287966,-31.0310638203076,16.1885644631732));
#29763=CARTESIAN_POINT('Ctrl Pts',(32.6111519417731,-31.0313387615314,16.1880367365759));
#29764=CARTESIAN_POINT('Ctrl Pts',(32.6551741210764,-31.0316153056917,16.1875059332765));
#29765=CARTESIAN_POINT('Ctrl Pts',(32.6970878717851,-31.0318395012597,16.1870745377529));
#29766=CARTESIAN_POINT('Ctrl Pts',(32.7388013470541,-31.0320241553174,16.18671857384));
#29767=CARTESIAN_POINT('Ctrl Pts',(32.7801521457895,-31.032207203906,16.1863657048444));
#29768=CARTESIAN_POINT('Ctrl Pts',(32.8213062770031,-31.0323516104908,16.1860865454659));
#29769=CARTESIAN_POINT('Ctrl Pts',(32.8641640035306,-31.0324560971771,16.1858844594635));
#29770=CARTESIAN_POINT('Ctrl Pts',(32.9038200784547,-31.0325527782704,16.1856974701314));
#29771=CARTESIAN_POINT('Ctrl Pts',(32.9449347772922,-31.0326154655021,16.1855761117062));
#29772=CARTESIAN_POINT('Ctrl Pts',(32.9890474705844,-31.0326287580453,16.1855509840874));
#29773=CARTESIAN_POINT('Ctrl Pts',(32.992608929339,-31.032629831225,16.1855489553974));
#29774=CARTESIAN_POINT('Ctrl Pts',(32.9961899495417,-31.0326305730128,16.1855475722578));
#29775=CARTESIAN_POINT('Ctrl Pts',(32.9997913521115,-31.0326309700539,16.185546860962));
#29776=CARTESIAN_POINT('Ctrl Pts',(33.0362292496772,-31.0326349871947,16.1855396642873));
#29777=CARTESIAN_POINT('Ctrl Pts',(33.0740922921121,-31.0326386992186,16.1855331333215));
#29778=CARTESIAN_POINT('Ctrl Pts',(33.1141439185632,-31.0326422490869,16.1855273500632));
#29779=CARTESIAN_POINT('Ctrl Pts',(33.2461674547435,-31.0326539506384,16.1855082865123));
#29780=CARTESIAN_POINT('Ctrl Pts',(33.3721931286569,-31.0326588963954,16.1855003220479));
#29781=CARTESIAN_POINT('Ctrl Pts',(33.4993879207449,-31.0326635427517,16.185492813855));
#29782=CARTESIAN_POINT('Ctrl Pts',(33.6627849160626,-31.0326695115548,16.185483168679));
#29783=CARTESIAN_POINT('Ctrl Pts',(33.828111247454,-31.0326749862723,16.1854742764645));
#29784=CARTESIAN_POINT('Ctrl Pts',(33.9929845306744,-31.0326833946006,16.1854606405094));
#29785=CARTESIAN_POINT('Ctrl Pts',(34.3227310971152,-31.032700211257,16.1854333685993));
#29786=CARTESIAN_POINT('Ctrl Pts',(34.6506654708719,-31.0327287623561,16.185387121727));
#29787=CARTESIAN_POINT('Ctrl Pts',(34.9792693636211,-31.0327480042371,16.1853559472169));
#29788=CARTESIAN_POINT('Ctrl Pts',(35.3078732563702,-31.0327672461181,16.1853247727069));
#29789=CARTESIAN_POINT('Ctrl Pts',(35.6371466681117,-31.0327771787811,16.185308670559));
#29790=CARTESIAN_POINT('Ctrl Pts',(35.9662682695209,-31.0327855310262,16.1852951338217));
#29791=CARTESIAN_POINT('Ctrl Pts',(36.2953898709301,-31.0327938832714,16.1852815970843));
#29792=CARTESIAN_POINT('Ctrl Pts',(36.624359662007,-31.0328006550989,16.1852706257574));
#29793=CARTESIAN_POINT('Ctrl Pts',(36.9532592751492,-31.0328145551759,16.185248102247));
#29794=CARTESIAN_POINT('Ctrl Pts',(38.1023262780261,-31.0328631174705,16.1851694125147));
#29795=CARTESIAN_POINT('Ctrl Pts',(39.2505367075415,-31.0329986853002,16.184949719878));
#29796=CARTESIAN_POINT('Ctrl Pts',(40.4000986012038,-31.0330322281526,16.1848953623403));
#29797=CARTESIAN_POINT('Ctrl Pts',(6.89999999997365,-11.0276873985587,-0.168526548676476));
#29798=CARTESIAN_POINT('Ctrl Pts',(6.99168932310453,-11.0290491215116,-0.107121039164008));
#29799=CARTESIAN_POINT('Ctrl Pts',(7.08383940291242,-11.0299018391088,-0.0458098125994616));
#29800=CARTESIAN_POINT('Ctrl Pts',(8.15761824498006,-11.0337651740187,0.664186592400576));
#29801=CARTESIAN_POINT('Ctrl Pts',(9.166078574375,-10.9699676285446,1.30870352701556));
#29802=CARTESIAN_POINT('Ctrl Pts',(11.2535171643192,-10.77603305676,2.47376106241927));
#29803=CARTESIAN_POINT('Ctrl Pts',(12.2576790632369,-10.6330057282434,3.00237606292525));
#29804=CARTESIAN_POINT('Ctrl Pts',(14.3563663857894,-10.3307260661656,3.94447005883399));
#29805=CARTESIAN_POINT('Ctrl Pts',(15.3658129161116,-10.1540434041659,4.36032593857961));
#29806=CARTESIAN_POINT('Ctrl Pts',(17.4727193021212,-9.82334300624283,5.08193366885832));
#29807=CARTESIAN_POINT('Ctrl Pts',(18.4888802671462,-9.6488422591121,5.39169279079136));
#29808=CARTESIAN_POINT('Ctrl Pts',(19.8473882183426,-9.45778984314827,5.72385817850078));
#29809=CARTESIAN_POINT('Ctrl Pts',(20.3451395577184,-9.38741838105894,5.84063156394592));
#29810=CARTESIAN_POINT('Ctrl Pts',(21.119864121141,-9.28201599203951,6.00690103675049));
#29811=CARTESIAN_POINT('Ctrl Pts',(21.9116430735679,-9.18172875488037,6.15921075032182));
#29812=CARTESIAN_POINT('Ctrl Pts',(22.4533884343747,-9.12054551137776,6.25063668203688));
#29813=CARTESIAN_POINT('Ctrl Pts',(22.8546099577479,-9.07881438233612,6.31320896750581));
#29814=CARTESIAN_POINT('Ctrl Pts',(23.1058218650382,-9.05298395410356,6.35118260107245));
#29815=CARTESIAN_POINT('Ctrl Pts',(23.6175153199789,-9.00245668094438,6.42382403760964));
#29816=CARTESIAN_POINT('Ctrl Pts',(24.1364702886545,-8.95485371029556,6.49007583237978));
#29817=CARTESIAN_POINT('Ctrl Pts',(24.6629181373247,-8.91145225308146,6.54944423929281));
#29818=CARTESIAN_POINT('Ctrl Pts',(25.0606678571037,-8.88140293076166,6.59024788291776));
#29819=CARTESIAN_POINT('Ctrl Pts',(25.3945416155883,-8.85873533710267,6.62099228309712));
#29820=CARTESIAN_POINT('Ctrl Pts',(25.6627586119465,-8.84221409068036,6.64352323130155));
#29821=CARTESIAN_POINT('Ctrl Pts',(25.7972076165426,-8.83452216013017,6.65408072739389));
#29822=CARTESIAN_POINT('Ctrl Pts',(26.3824137782947,-8.80240169886326,6.69837697633856));
#29823=CARTESIAN_POINT('Ctrl Pts',(27.4369717967156,-8.76563881905857,6.74704662082205));
#29824=CARTESIAN_POINT('Ctrl Pts',(28.4593635146678,-8.74917816753953,6.76713562537257));
#29825=CARTESIAN_POINT('Ctrl Pts',(29.0427481469893,-8.73952198264548,6.77974505298725));
#29826=CARTESIAN_POINT('Ctrl Pts',(29.2174939164953,-8.73701514175021,6.78306424239326));
#29827=CARTESIAN_POINT('Ctrl Pts',(29.560704833228,-8.73336568489196,6.78786835107264));
#29828=CARTESIAN_POINT('Ctrl Pts',(29.9899637006215,-8.73093988338432,6.7910625393568));
#29829=CARTESIAN_POINT('Ctrl Pts',(30.5003627545719,-8.73068255391876,6.79139754852951));
#29830=CARTESIAN_POINT('Ctrl Pts',(31.5152290141056,-8.73381293113862,6.78728755019412));
#29831=CARTESIAN_POINT('Ctrl Pts',(32.346385618228,-8.74063107149336,6.77838967797267));
#29832=CARTESIAN_POINT('Ctrl Pts',(33.1616392309915,-8.74062146997074,6.77840182636606));
#29833=CARTESIAN_POINT('Ctrl Pts',(33.4928689770884,-8.74062052628884,6.77840284181041));
#29834=CARTESIAN_POINT('Ctrl Pts',(33.9856875201801,-8.74061852020513,6.77840526161275));
#29835=CARTESIAN_POINT('Ctrl Pts',(34.479956929609,-8.74061713883255,6.7784068708528));
#29836=CARTESIAN_POINT('Ctrl Pts',(35.1382080085716,-8.74061527897129,6.778409075901));
#29837=CARTESIAN_POINT('Ctrl Pts',(35.9613703496106,-8.74061266742265,6.7784121544085));
#29838=CARTESIAN_POINT('Ctrl Pts',(37.9364530322258,-8.74060999527037,6.77841531264166));
#29839=CARTESIAN_POINT('Ctrl Pts',(39.5833333333333,-8.74059347982545,6.77843480602319));
#29840=CARTESIAN_POINT('Ctrl Pts',(40.9,-8.74059347982545,6.77843480602319));
#29841=CARTESIAN_POINT('Ctrl Pts',(6.65963435785827,-15.5421695279122,-0.914290744262173));
#29842=CARTESIAN_POINT('Ctrl Pts',(6.7513219377677,-15.5478000748543,-0.827664097498932));
#29843=CARTESIAN_POINT('Ctrl Pts',(6.84347928233528,-15.552705535984,-0.741125593738216));
#29844=CARTESIAN_POINT('Ctrl Pts',(7.91768245328712,-15.6010379387116,0.260912141468049));
#29845=CARTESIAN_POINT('Ctrl Pts',(8.92716941433653,-15.5498192559038,1.17337698529147));
#29846=CARTESIAN_POINT('Ctrl Pts',(11.0226592374973,-15.3445243615387,2.83406080960164));
#29847=CARTESIAN_POINT('Ctrl Pts',(12.0289222513091,-15.174357849642,3.58841078209879));
#29848=CARTESIAN_POINT('Ctrl Pts',(14.1441326723881,-14.8006104561251,4.94359337154892));
#29849=CARTESIAN_POINT('Ctrl Pts',(15.1576282381579,-14.5754503759515,5.54148857510365));
#29850=CARTESIAN_POINT('Ctrl Pts',(17.2903455772588,-14.1464770374584,6.58799131832697));
#29851=CARTESIAN_POINT('Ctrl Pts',(18.3126565164254,-13.9174993841978,7.03615941125111));
#29852=CARTESIAN_POINT('Ctrl Pts',(19.6943886098338,-13.6636269320846,7.52140607073201));
#29853=CARTESIAN_POINT('Ctrl Pts',(20.1963997689949,-13.5705283753709,7.69105316997363));
#29854=CARTESIAN_POINT('Ctrl Pts',(20.9820476354982,-13.4299327266448,7.9338457745664));
#29855=CARTESIAN_POINT('Ctrl Pts',(21.7860719497258,-13.2956844767357,8.15658902665418));
#29856=CARTESIAN_POINT('Ctrl Pts',(22.337913112583,-13.2134517389134,8.29065006793576));
#29857=CARTESIAN_POINT('Ctrl Pts',(22.7470242103181,-13.1573095336481,8.38247788994951));
#29858=CARTESIAN_POINT('Ctrl Pts',(23.0012838485785,-13.1227286630507,8.43794163853499));
#29859=CARTESIAN_POINT('Ctrl Pts',(23.5207560883433,-13.0548326909721,8.54431696039333));
#29860=CARTESIAN_POINT('Ctrl Pts',(24.0478165510038,-12.9907421048667,8.6413962979357));
#29861=CARTESIAN_POINT('Ctrl Pts',(24.5834508086859,-12.9321620155412,8.72854413973127));
#29862=CARTESIAN_POINT('Ctrl Pts',(24.9884814516725,-12.8915554305395,8.78849484453726));
#29863=CARTESIAN_POINT('Ctrl Pts',(25.3288761766951,-12.8608881947636,8.83370307828864));
#29864=CARTESIAN_POINT('Ctrl Pts',(25.6025411192578,-12.8385223247212,8.86685769924433));
#29865=CARTESIAN_POINT('Ctrl Pts',(25.73979094788,-12.8281059147068,8.88239886754129));
#29866=CARTESIAN_POINT('Ctrl Pts',(26.3376341743262,-12.7845927902169,8.94762125697));
#29867=CARTESIAN_POINT('Ctrl Pts',(27.4152541470277,-12.7347557261565,9.01924678134855));
#29868=CARTESIAN_POINT('Ctrl Pts',(28.4429499146133,-12.7126826807293,9.04845162691347));
#29869=CARTESIAN_POINT('Ctrl Pts',(29.0259735124592,-12.6997781188676,9.06676270853369));
#29870=CARTESIAN_POINT('Ctrl Pts',(29.2042686472714,-12.6963761571783,9.07165323227908));
#29871=CARTESIAN_POINT('Ctrl Pts',(29.5518704410187,-12.6914548812216,9.07868995890017));
#29872=CARTESIAN_POINT('Ctrl Pts',(29.9865605489545,-12.6881801081657,9.08337117217634));
#29873=CARTESIAN_POINT('Ctrl Pts',(30.5013181269547,-12.6878363073061,9.08385656546482));
#29874=CARTESIAN_POINT('Ctrl Pts',(31.5221463919968,-12.692041007367,9.07785413361798));
#29875=CARTESIAN_POINT('Ctrl Pts',(32.3518561954418,-12.7011306199596,9.06494609970922));
#29876=CARTESIAN_POINT('Ctrl Pts',(33.1604291208178,-12.7011133788388,9.06496486760967));
#29877=CARTESIAN_POINT('Ctrl Pts',(33.4925190590671,-12.7011117013819,9.06496624091916));
#29878=CARTESIAN_POINT('Ctrl Pts',(33.9849476449336,-12.7011081104537,9.06496984963707));
#29879=CARTESIAN_POINT('Ctrl Pts',(34.4794328720439,-12.7011056432242,9.06497218408094));
#29880=CARTESIAN_POINT('Ctrl Pts',(35.1376484147356,-12.7011023177079,9.06497542847038));
#29881=CARTESIAN_POINT('Ctrl Pts',(35.9609115545804,-12.7010976498373,9.06497993729913));
#29882=CARTESIAN_POINT('Ctrl Pts',(37.9360269889122,-12.7010928728514,9.06498457262957));
#29883=CARTESIAN_POINT('Ctrl Pts',(39.5833333333333,-12.701063350837,9.06501315216909));
#29884=CARTESIAN_POINT('Ctrl Pts',(40.9,-12.701063350837,9.06501315216909));
#29885=CARTESIAN_POINT('Ctrl Pts',(6.47499700785697,-23.4452408248497,-2.19830497971403));
#29886=CARTESIAN_POINT('Ctrl Pts',(6.56578730943226,-23.4579749263878,-2.06870104448402));
#29887=CARTESIAN_POINT('Ctrl Pts',(6.65702462351448,-23.4696212195475,-1.93921681262018));
#29888=CARTESIAN_POINT('Ctrl Pts',(7.72175305647137,-23.5924911125725,-0.437116228582369));
#29889=CARTESIAN_POINT('Ctrl Pts',(8.72281885180382,-23.562968194923,0.93768014090861));
#29890=CARTESIAN_POINT('Ctrl Pts',(10.7949492361907,-23.3400040819286,3.44026704375966));
#29891=CARTESIAN_POINT('Ctrl Pts',(11.7960921547002,-23.1244337632637,4.58695803318564));
#29892=CARTESIAN_POINT('Ctrl Pts',(13.8958332645754,-22.6316660291752,6.64967501166335));
#29893=CARTESIAN_POINT('Ctrl Pts',(14.90655296446,-22.3241101177864,7.56603922905964));
#29894=CARTESIAN_POINT('Ctrl Pts',(17.0410718223018,-21.7268962408645,9.17994203101701));
#29895=CARTESIAN_POINT('Ctrl Pts',(18.0654584152639,-21.4035033181339,9.87337110606603));
#29896=CARTESIAN_POINT('Ctrl Pts',(19.4655915747002,-21.0382396447148,10.6334003056859));
#29897=CARTESIAN_POINT('Ctrl Pts',(19.9714665789849,-20.9051898734593,10.8971713557552));
#29898=CARTESIAN_POINT('Ctrl Pts',(20.7678306953019,-20.7020007981629,11.2774874271219));
#29899=CARTESIAN_POINT('Ctrl Pts',(21.5858101282049,-20.5068169170513,11.6277425327431));
#29900=CARTESIAN_POINT('Ctrl Pts',(22.1506096305012,-20.3863209191721,11.8398576536859));
#29901=CARTESIAN_POINT('Ctrl Pts',(22.5704199924792,-20.3038374401208,11.9854171937934));
#29902=CARTESIAN_POINT('Ctrl Pts',(22.8289065956908,-20.2535349220293,12.0724797867542));
#29903=CARTESIAN_POINT('Ctrl Pts',(23.3593853239227,-20.1541718428526,12.2402701514192));
#29904=CARTESIAN_POINT('Ctrl Pts',(23.8985486588058,-20.0601195256969,12.3936552183108));
#29905=CARTESIAN_POINT('Ctrl Pts',(24.4483714419234,-19.9737860075935,12.5318087211868));
#29906=CARTESIAN_POINT('Ctrl Pts',(24.8648919059684,-19.9138158121696,12.6269879069122));
#29907=CARTESIAN_POINT('Ctrl Pts',(25.2158455690757,-19.8684065291875,12.6989260386039));
#29908=CARTESIAN_POINT('Ctrl Pts',(25.4984343217207,-19.8352396029271,12.7517388774024));
#29909=CARTESIAN_POINT('Ctrl Pts',(25.6403132052064,-19.8197769054431,12.7765150372189));
#29910=CARTESIAN_POINT('Ctrl Pts',(26.2592160414081,-19.7551088720197,12.8806146990981));
#29911=CARTESIAN_POINT('Ctrl Pts',(27.3768446537005,-19.6810635867321,12.994818613011));
#29912=CARTESIAN_POINT('Ctrl Pts',(28.4139434096805,-19.6491350216629,13.0400692167481));
#29913=CARTESIAN_POINT('Ctrl Pts',(28.9963902080608,-19.6305403234117,13.0683908406421));
#29914=CARTESIAN_POINT('Ctrl Pts',(29.180878403009,-19.6254773891901,13.0761959447011));
#29915=CARTESIAN_POINT('Ctrl Pts',(29.5361613355606,-19.6182496508377,13.0872826938044));
#29916=CARTESIAN_POINT('Ctrl Pts',(29.9803701492975,-19.613426667661,13.0946820190499));
#29917=CARTESIAN_POINT('Ctrl Pts',(30.5027645652051,-19.6129305494837,13.0954354949456));
#29918=CARTESIAN_POINT('Ctrl Pts',(31.5340441540658,-19.619049331486,13.0860712826798));
#29919=CARTESIAN_POINT('Ctrl Pts',(32.361293357075,-19.6320590316267,13.0662692307128));
#29920=CARTESIAN_POINT('Ctrl Pts',(33.1582057305723,-19.6320151866218,13.0663352315321));
#29921=CARTESIAN_POINT('Ctrl Pts',(33.4918052160808,-19.6320107493385,13.0663415440457));
#29922=CARTESIAN_POINT('Ctrl Pts',(33.9835585756086,-19.6320015037508,13.0663552182345));
#29923=CARTESIAN_POINT('Ctrl Pts',(34.4784268233885,-19.6319950964453,13.0663645784942));
#29924=CARTESIAN_POINT('Ctrl Pts',(35.1365871092733,-19.6319864972548,13.0663772185058));
#29925=CARTESIAN_POINT('Ctrl Pts',(35.9600364992905,-19.631974409872,13.0663949498221));
#29926=CARTESIAN_POINT('Ctrl Pts',(37.935219274406,-19.6319620479287,13.0664131007023));
#29927=CARTESIAN_POINT('Ctrl Pts',(39.5833333333333,-19.6318856251071,13.0665252579244));
#29928=CARTESIAN_POINT('Ctrl Pts',(40.9,-19.6318856251071,13.0665252579244));
#29929=CARTESIAN_POINT('Ctrl Pts',(6.39840282685635,-31.3636440442398,-3.36386536347516));
#29930=CARTESIAN_POINT('Ctrl Pts',(6.48879582230594,-31.3828291635015,-3.19164073503352));
#29931=CARTESIAN_POINT('Ctrl Pts',(6.57961766269115,-31.4005708453189,-3.01959979440376));
#29932=CARTESIAN_POINT('Ctrl Pts',(7.64032554406628,-31.5903744166847,-1.0214771742003));
#29933=CARTESIAN_POINT('Ctrl Pts',(8.63867106160224,-31.5754173772483,0.811297807542586));
#29934=CARTESIAN_POINT('Ctrl Pts',(10.6964316380006,-31.3261515036618,4.13353910931635));
#29935=CARTESIAN_POINT('Ctrl Pts',(11.6947290441859,-31.0615534966588,5.66648609020814));
#29936=CARTESIAN_POINT('Ctrl Pts',(13.7762263687762,-30.4500782098735,8.40637303045944));
#29937=CARTESIAN_POINT('Ctrl Pts',(14.7826773906134,-30.0602543273649,9.63313444048393));
#29938=CARTESIAN_POINT('Ctrl Pts',(16.8988982405362,-29.3025485110513,11.7841821047735));
#29939=CARTESIAN_POINT('Ctrl Pts',(17.9188263508252,-28.8873179990429,12.7156877051221));
#29940=CARTESIAN_POINT('Ctrl Pts',(19.3136620513073,-28.4161739072999,13.7379571249216));
#29941=CARTESIAN_POINT('Ctrl Pts',(19.8189838754924,-28.2441169214324,14.0939758439964));
#29942=CARTESIAN_POINT('Ctrl Pts',(20.6150001505384,-27.9803060047161,14.6080226620617));
#29943=CARTESIAN_POINT('Ctrl Pts',(21.4350390683302,-27.7255808745093,15.0835002485375));
#29944=CARTESIAN_POINT('Ctrl Pts',(22.0037815933943,-27.5672808319298,15.3731124530265));
#29945=CARTESIAN_POINT('Ctrl Pts',(22.4278524797961,-27.4584837184542,15.5725968076267));
#29946=CARTESIAN_POINT('Ctrl Pts',(22.6881478873211,-27.3924576319504,15.6914147925573));
#29947=CARTESIAN_POINT('Ctrl Pts',(23.2238106344271,-27.2614400973337,15.921268075794));
#29948=CARTESIAN_POINT('Ctrl Pts',(23.7696978745005,-27.1369441741205,16.1321064141348));
#29949=CARTESIAN_POINT('Ctrl Pts',(24.3285206801333,-27.022064166134,16.3229204338608));
#29950=CARTESIAN_POINT('Ctrl Pts',(24.7529653140504,-26.9419913350362,16.4547973514759));
#29951=CARTESIAN_POINT('Ctrl Pts',(25.1117719491785,-26.8811074137509,16.554863796012));
#29952=CARTESIAN_POINT('Ctrl Pts',(25.4013553254924,-26.836506870562,16.6285198436922));
#29953=CARTESIAN_POINT('Ctrl Pts',(25.5469791293171,-26.8156703264605,16.6631374284086));
#29954=CARTESIAN_POINT('Ctrl Pts',(26.1832292898987,-26.7283606594225,16.8088431266916));
#29955=CARTESIAN_POINT('Ctrl Pts',(27.3386864567867,-26.6279357083785,16.9694451045118));
#29956=CARTESIAN_POINT('Ctrl Pts',(28.3853135289695,-26.5860990135272,17.0308214554548));
#29957=CARTESIAN_POINT('Ctrl Pts',(28.9671494424549,-26.5618106446087,17.0691585340134));
#29958=CARTESIAN_POINT('Ctrl Pts',(29.1577497745605,-26.5549253720648,17.0801578267592));
#29959=CARTESIAN_POINT('Ctrl Pts',(29.5206667657,-26.5452518307316,17.0955352214361));
#29960=CARTESIAN_POINT('Ctrl Pts',(29.9743609805096,-26.5387742795118,17.1058350294713));
#29961=CARTESIAN_POINT('Ctrl Pts',(30.5043929318942,-26.5381249904399,17.1068574997828));
#29962=CARTESIAN_POINT('Ctrl Pts',(31.5460952643805,-26.54622028874,17.0940221862975));
#29963=CARTESIAN_POINT('Ctrl Pts',(32.3708379684223,-26.5630634070367,17.0674707682792));
#29964=CARTESIAN_POINT('Ctrl Pts',(33.1560659395073,-26.5629740474711,17.0676145179389));
#29965=CARTESIAN_POINT('Ctrl Pts',(33.4911715963805,-26.5629648505727,17.0676289242213));
#29966=CARTESIAN_POINT('Ctrl Pts',(33.9822440621776,-26.5629459056337,17.0676591426917));
#29967=CARTESIAN_POINT('Ctrl Pts',(34.4774910986523,-26.5629327280363,17.0676800396183));
#29968=CARTESIAN_POINT('Ctrl Pts',(35.1355906516825,-26.5629150749568,17.0677081152075));
#29969=CARTESIAN_POINT('Ctrl Pts',(35.9592185001008,-26.5628902459987,17.0677475655254));
#29970=CARTESIAN_POINT('Ctrl Pts',(37.9344606912907,-26.5628648600815,17.067787918432));
#29971=CARTESIAN_POINT('Ctrl Pts',(39.5833333333333,-26.5627078993772,17.0680373636797));
#29972=CARTESIAN_POINT('Ctrl Pts',(40.9,-26.5627078993772,17.0680373636797));
#29973=CARTESIAN_POINT('Ctrl Pts',(6.37427268165564,-34.7583359408307,-3.85496595036637));
#29974=CARTESIAN_POINT('Ctrl Pts',(6.46448755772838,-34.7802475524424,-3.66446375246399));
#29975=CARTESIAN_POINT('Ctrl Pts',(6.55512331969025,-34.8005635888992,-3.47417181608893));
#29976=CARTESIAN_POINT('Ctrl Pts',(7.61410548625795,-35.0185788676572,-1.26339052014805));
#29977=CARTESIAN_POINT('Ctrl Pts',(8.61145388480624,-35.0093532870147,0.765602457207686));
#29978=CARTESIAN_POINT('Ctrl Pts',(10.6635149436019,-34.747974440135,4.43910992978124));
#29979=CARTESIAN_POINT('Ctrl Pts',(11.6608017032625,-34.4619345886989,6.13747453196185));
#29980=CARTESIAN_POINT('Ctrl Pts',(13.7353542747945,-33.7990269238398,9.16685810272323));
#29981=CARTESIAN_POINT('Ctrl Pts',(14.7402715202386,-33.3736740493576,10.5262979552789));
#29982=CARTESIAN_POINT('Ctrl Pts',(16.8491677832147,-32.5473921410153,12.9054531131771));
#29983=CARTESIAN_POINT('Ctrl Pts',(17.8672809631136,-32.092886041556,13.9382203331611));
#29984=CARTESIAN_POINT('Ctrl Pts',(19.2587625104673,-31.577179869867,15.0707179501981));
#29985=CARTESIAN_POINT('Ctrl Pts',(19.7635899403542,-31.3885503410944,15.4658689812884));
#29986=CARTESIAN_POINT('Ctrl Pts',(20.5586991602297,-31.0991569516509,16.0362969262867));
#29987=CARTESIAN_POINT('Ctrl Pts',(21.3785272493019,-30.819343278526,16.564533786793));
#29988=CARTESIAN_POINT('Ctrl Pts',(21.9479176287994,-30.6451300260617,16.8867906552356));
#29989=CARTESIAN_POINT('Ctrl Pts',(22.3729695502115,-30.525234440013,17.1090467735268));
#29990=CARTESIAN_POINT('Ctrl Pts',(22.6337096028249,-30.45253373981,17.2413581349254));
#29991=CARTESIAN_POINT('Ctrl Pts',(23.170751986421,-30.3080867629257,17.4975676797997));
#29992=CARTESIAN_POINT('Ctrl Pts',(23.7186485394885,-30.1706268071311,17.7328951431606));
#29993=CARTESIAN_POINT('Ctrl Pts',(24.2804077704386,-30.0435395405948,17.9462491604951));
#29994=CARTESIAN_POINT('Ctrl Pts',(24.7075732751059,-29.9548357769836,18.093896808302));
#29995=CARTESIAN_POINT('Ctrl Pts',(25.0692008252976,-29.8872739715488,18.2061112471098));
#29996=CARTESIAN_POINT('Ctrl Pts',(25.3613771492326,-29.8377189043885,18.2888047627701));
#29997=CARTESIAN_POINT('Ctrl Pts',(25.5084154817282,-29.8145466170754,18.3277015544067));
#29998=CARTESIAN_POINT('Ctrl Pts',(26.1512870025445,-29.7173716879778,18.4915385207408));
#29999=CARTESIAN_POINT('Ctrl Pts',(27.3223884400174,-29.6052740416532,18.6726738474943));
#30000=CARTESIAN_POINT('Ctrl Pts',(28.3731396048322,-29.5591775248211,18.7409825767552));
#30001=CARTESIAN_POINT('Ctrl Pts',(28.9547046473316,-29.532448097728,18.7836137746099));
#30002=CARTESIAN_POINT('Ctrl Pts',(29.1479037067739,-29.5247529606445,18.7960320303042));
#30003=CARTESIAN_POINT('Ctrl Pts',(29.5140802367922,-29.5140058211202,18.8132921881814));
#30004=CARTESIAN_POINT('Ctrl Pts',(29.9718311305159,-29.5067996680498,18.8248686377543));
#30005=CARTESIAN_POINT('Ctrl Pts',(30.505136527612,-29.5060845192012,18.8260067178223));
#30006=CARTESIAN_POINT('Ctrl Pts',(31.5512984754482,-29.515038303799,18.8116639693829));
#30007=CARTESIAN_POINT('Ctrl Pts',(32.3749555043413,-29.5335081969199,18.7822473977007));
#30008=CARTESIAN_POINT('Ctrl Pts',(33.1551698865007,-29.5333957726549,18.7824304492384));
#30009=CARTESIAN_POINT('Ctrl Pts',(33.4909201969602,-29.533384156022,18.782448957068));
#30010=CARTESIAN_POINT('Ctrl Pts',(33.981699427726,-29.5333602907363,18.7824875453788));
#30011=CARTESIAN_POINT('Ctrl Pts',(34.4771077390558,-29.533343676228,18.7825142819534));
#30012=CARTESIAN_POINT('Ctrl Pts',(35.1351798881798,-29.5333214285967,18.7825501686284));
#30013=CARTESIAN_POINT('Ctrl Pts',(35.958882261465,-29.5332901329543,18.7826006107083));
#30014=CARTESIAN_POINT('Ctrl Pts',(37.9341479260215,-29.5332581373787,18.7826521993715));
#30015=CARTESIAN_POINT('Ctrl Pts',(39.5833333333333,-29.5330603026358,18.7829711232891));
#30016=CARTESIAN_POINT('Ctrl Pts',(40.9,-29.5330603026358,18.7829711232891));
#30017=CARTESIAN_POINT('',(40.9,-27.7992994660114,17.7819838375536));
#30018=CARTESIAN_POINT('Ctrl Pts',(40.9,-27.7992994660114,17.7819838375536));
#30019=CARTESIAN_POINT('Ctrl Pts',(40.9,-28.2327406817405,18.0322312401327));
#30020=CARTESIAN_POINT('Ctrl Pts',(40.9,-28.6661818974695,18.2824786427117));
#30021=CARTESIAN_POINT('Ctrl Pts',(40.9,-29.0996231131986,18.5327260452908));
#30022=CARTESIAN_POINT('',(38.,-27.7992994660114,17.7819838375536));
#30023=CARTESIAN_POINT('Ctrl Pts',(38.,-27.7992994660114,17.7819838375536));
#30024=CARTESIAN_POINT('Ctrl Pts',(38.9666666666667,-27.7992994660114,17.7819838375536));
#30025=CARTESIAN_POINT('Ctrl Pts',(39.9333333333333,-27.7992994660114,17.7819838375536));
#30026=CARTESIAN_POINT('Ctrl Pts',(40.9,-27.7992994660114,17.7819838375536));
#30027=CARTESIAN_POINT('Ctrl Pts',(37.4972396727241,-27.2792903521173,17.4814222894395));
#30028=CARTESIAN_POINT('Ctrl Pts',(37.6643013627082,-27.4529632561665,17.581705123587));
#30029=CARTESIAN_POINT('Ctrl Pts',(37.8311425499703,-27.6263785906013,17.681842059693));
#30030=CARTESIAN_POINT('Ctrl Pts',(37.9976538234737,-27.7994318724651,17.7817719425585));
#30031=CARTESIAN_POINT('',(6.9,-29.9143312995417,-2.26556458774884));
#30032=CARTESIAN_POINT('Ctrl Pts',(6.9,-29.9143312995417,-2.26556458774883));
#30033=CARTESIAN_POINT('Ctrl Pts',(6.9,-27.3056186709172,-2.00382962437802));
#30034=CARTESIAN_POINT('Ctrl Pts',(6.90000000000115,-24.6693701926632,-1.73285728374608));
#30035=CARTESIAN_POINT('Ctrl Pts',(6.90000000000115,-18.7182130985667,-1.09593289590079));
#30036=CARTESIAN_POINT('Ctrl Pts',(6.9,-14.7845781982083,-0.65479489350369));
#30037=CARTESIAN_POINT('Ctrl Pts',(6.9,-11.02768739857,-0.168526548660246));
#30038=CARTESIAN_POINT('',(22.9245129145126,-27.5141512254856,15.8853026165582));
#30039=CARTESIAN_POINT('Ctrl Pts',(22.9245129145126,-27.5141512254856,15.8853026165582));
#30040=CARTESIAN_POINT('Ctrl Pts',(22.7202811020963,-27.5032269692373,15.7659233420327));
#30041=CARTESIAN_POINT('Ctrl Pts',(22.5089075447093,-27.4959054260063,15.6398559109135));
#30042=CARTESIAN_POINT('Ctrl Pts',(22.2913349439917,-27.4928730439354,15.5073965833875));
#30043=CARTESIAN_POINT('Ctrl Pts',(21.4451770585294,-27.4810798586144,14.992251275019));
#30044=CARTESIAN_POINT('Ctrl Pts',(20.522095155667,-27.5650257717264,14.3509960808547));
#30045=CARTESIAN_POINT('Ctrl Pts',(19.7671428819542,-27.6762399607748,13.7859304181016));
#30046=CARTESIAN_POINT('Ctrl Pts',(19.5194773058393,-27.7127242885422,13.6005580206914));
#30047=CARTESIAN_POINT('Ctrl Pts',(19.2865716386092,-27.7514615171004,13.4218723240252));
#30048=CARTESIAN_POINT('Ctrl Pts',(19.0728538401323,-27.7894004949774,13.2552441975238));
#30049=CARTESIAN_POINT('Ctrl Pts',(18.7028555998035,-27.8550822264681,12.9667697979459));
#30050=CARTESIAN_POINT('Ctrl Pts',(18.4144703596235,-27.9152561335183,12.7292901983115));
#30051=CARTESIAN_POINT('Ctrl Pts',(18.0642874871537,-27.9946062155751,12.4284122845046));
#30052=CARTESIAN_POINT('Ctrl Pts',(17.4420927116721,-28.1355931408966,11.8938211301512));
#30053=CARTESIAN_POINT('Ctrl Pts',(16.7224564418218,-28.3254287038798,11.2282910364347));
#30054=CARTESIAN_POINT('Ctrl Pts',(15.9202806616111,-28.5439924969395,10.4246142212493));
#30055=CARTESIAN_POINT('Ctrl Pts',(15.4090529834519,-28.6832834892781,9.91242993152971));
#30056=CARTESIAN_POINT('Ctrl Pts',(14.8739602945717,-28.8377564730262,9.33532862360362));
#30057=CARTESIAN_POINT('Ctrl Pts',(14.3169794331159,-28.9944199787762,8.69171842999422));
#30058=CARTESIAN_POINT('Ctrl Pts',(13.8864206762839,-29.1155243989539,8.19419324731461));
#30059=CARTESIAN_POINT('Ctrl Pts',(13.3867890027806,-29.2546860278643,7.59173852185157));
#30060=CARTESIAN_POINT('Ctrl Pts',(12.8146824059514,-29.3960736315876,6.86770373383358));
#30061=CARTESIAN_POINT('Ctrl Pts',(12.2526665517594,-29.5349674589251,6.15643937836574));
#30062=CARTESIAN_POINT('Ctrl Pts',(11.6379478462802,-29.678401911158,5.3206691843855));
#30063=CARTESIAN_POINT('Ctrl Pts',(10.9739250490306,-29.7956367796097,4.35448584003977));
#30064=CARTESIAN_POINT('Ctrl Pts',(10.5683455447962,-29.8672428449776,3.76434923114257));
#30065=CARTESIAN_POINT('Ctrl Pts',(10.1437415406955,-29.9275397584159,3.12422765605926));
#30066=CARTESIAN_POINT('Ctrl Pts',(9.74137929176525,-29.9670595377668,2.50486371218385));
#30067=CARTESIAN_POINT('Ctrl Pts',(8.72285779294234,-30.0670981099855,0.937033991304209));
#30068=CARTESIAN_POINT('Ctrl Pts',(7.81323138778195,-30.0560666286387,-0.638451825302673));
#30069=CARTESIAN_POINT('Ctrl Pts',(6.9,-29.9143312995417,-2.26556458774883));
#30070=CARTESIAN_POINT('Ctrl Pts',(30.5,-29.5059919176187,18.8254200738635));
#30071=CARTESIAN_POINT('Ctrl Pts',(29.9560179420816,-29.293615660989,18.7064245513841));
#30072=CARTESIAN_POINT('Ctrl Pts',(29.4152668325132,-29.0895919906434,18.5734800115823));
#30073=CARTESIAN_POINT('Ctrl Pts',(28.8740459957565,-28.9020067835811,18.4125151878636));
#30074=CARTESIAN_POINT('Ctrl Pts',(28.353527792344,-28.7215970352203,18.2577075471291));
#30075=CARTESIAN_POINT('Ctrl Pts',(27.8179515912467,-28.533139934629,18.1008601332298));
#30076=CARTESIAN_POINT('Ctrl Pts',(27.2695051149491,-28.3565719042575,17.9186544331585));
#30077=CARTESIAN_POINT('Ctrl Pts',(26.9554553615883,-28.2554660556725,17.8143203592948));
#30078=CARTESIAN_POINT('Ctrl Pts',(26.6378099296971,-28.1585101274347,17.7019284120276));
#30079=CARTESIAN_POINT('Ctrl Pts',(26.3179304017917,-28.0701057587103,17.5778023417279));
#30080=CARTESIAN_POINT('Ctrl Pts',(26.1078196745982,-28.012037940737,17.4962709631332));
#30081=CARTESIAN_POINT('Ctrl Pts',(25.8967402232745,-27.9576659729224,17.409683568055));
#30082=CARTESIAN_POINT('Ctrl Pts',(25.6850706236774,-27.9082593406129,17.3169960819306));
#30083=CARTESIAN_POINT('Ctrl Pts',(25.6562210027417,-27.9015254373195,17.3043631915899));
#30084=CARTESIAN_POINT('Ctrl Pts',(25.6277737638215,-27.8949772388532,17.2918013331136));
#30085=CARTESIAN_POINT('Ctrl Pts',(25.5983858063598,-27.8883138877393,17.2787081509674));
#30086=CARTESIAN_POINT('Ctrl Pts',(25.1249357452756,-27.7809650188704,17.067772501732));
#30087=CARTESIAN_POINT('Ctrl Pts',(24.1510084067019,-27.5797558484168,16.6022239440147));
#30088=CARTESIAN_POINT('Ctrl Pts',(22.9245129145126,-27.5141512254856,15.8853026165582));
#30089=CARTESIAN_POINT('Origin',(40.65,0.,0.));
#30090=CARTESIAN_POINT('',(40.4,-34.9678423698117,-1.5));
#30091=CARTESIAN_POINT('',(40.9,-34.4673758792282,-1.5));
#30092=CARTESIAN_POINT('Ctrl Pts',(40.4,-34.9678423698117,-1.5));
#30093=CARTESIAN_POINT('Ctrl Pts',(40.5666590142081,-34.8010300902437,-1.5));
#30094=CARTESIAN_POINT('Ctrl Pts',(40.7333430453063,-34.6341905783534,-1.5));
#30095=CARTESIAN_POINT('Ctrl Pts',(40.9,-34.4673758792282,-1.5));
#30096=CARTESIAN_POINT('',(40.9,-34.4673758792282,1.50000000000002));
#30097=CARTESIAN_POINT('Origin',(40.9,0.,0.));
#30098=CARTESIAN_POINT('',(40.4,-34.9678423698117,1.5));
#30099=CARTESIAN_POINT('Ctrl Pts',(40.9,-34.4673758792282,1.5));
#30100=CARTESIAN_POINT('Ctrl Pts',(40.7333430446438,-34.6341905790166,1.5));
#30101=CARTESIAN_POINT('Ctrl Pts',(40.5666590131148,-34.801030091338,1.5));
#30102=CARTESIAN_POINT('Ctrl Pts',(40.4,-34.9678423698117,1.5));
#30103=CARTESIAN_POINT('Origin',(40.4,0.,0.));
#30104=CARTESIAN_POINT('Origin',(35.7,0.,0.));
#30105=CARTESIAN_POINT('',(30.5,-34.9656486014478,1.55029606206997));
#30106=CARTESIAN_POINT('Ctrl Pts',(40.3999921398529,-34.9678423429768,1.49999538724756));
#30107=CARTESIAN_POINT('Ctrl Pts',(39.2499570215113,-34.9678422244593,1.49997501500716));
#30108=CARTESIAN_POINT('Ctrl Pts',(38.0998114916604,-34.9678417480135,1.49989311899335));
#30109=CARTESIAN_POINT('Ctrl Pts',(36.9497038557168,-34.9678416168427,1.49987059349837));
#30110=CARTESIAN_POINT('Ctrl Pts',(36.785105117964,-34.96784159807,1.49986736974094));
#30111=CARTESIAN_POINT('Ctrl Pts',(36.6205071563607,-34.9678415863694,1.49986536202073));
#30112=CARTESIAN_POINT('Ctrl Pts',(36.4559233022361,-34.9678415707796,1.49986268095532));
#30113=CARTESIAN_POINT('Ctrl Pts',(36.4193640724435,-34.9678415673166,1.4998620854067));
#30114=CARTESIAN_POINT('Ctrl Pts',(36.3828055387466,-34.9678415636617,1.49986145663366));
#30115=CARTESIAN_POINT('Ctrl Pts',(36.3462474593958,-34.967841559861,1.49986080263033));
#30116=CARTESIAN_POINT('Ctrl Pts',(36.0895450699579,-34.967841533173,1.49985621036996));
#30117=CARTESIAN_POINT('Ctrl Pts',(35.8501671305851,-34.9678416196704,1.49985084735669));
#30118=CARTESIAN_POINT('Ctrl Pts',(35.6266230092018,-34.9678417642539,1.49984692867087));
#30119=CARTESIAN_POINT('Ctrl Pts',(35.5729810992077,-34.9678417989483,1.49984598833841));
#30120=CARTESIAN_POINT('Ctrl Pts',(35.5202511626857,-34.9678418369404,1.49984512300934));
#30121=CARTESIAN_POINT('Ctrl Pts',(35.4684130151836,-34.9678418773881,1.49984434928581));
#30122=CARTESIAN_POINT('Ctrl Pts',(35.3128073279263,-34.9678419988026,1.49984202675329));
#30123=CARTESIAN_POINT('Ctrl Pts',(35.1652418679138,-34.9678421408902,1.49984027810625));
#30124=CARTESIAN_POINT('Ctrl Pts',(35.0252627275547,-34.967842254217,1.49983493809963));
#30125=CARTESIAN_POINT('Ctrl Pts',(35.0082618963838,-34.9678422679808,1.49983428954192));
#30126=CARTESIAN_POINT('Ctrl Pts',(34.9913729068342,-34.9678422813397,1.49983359135557));
#30127=CARTESIAN_POINT('Ctrl Pts',(34.9745948969331,-34.9678422942204,1.49983283870325));
#30128=CARTESIAN_POINT('Ctrl Pts',(34.8399133402553,-34.9678423976168,1.49982679696251));
#30129=CARTESIAN_POINT('Ctrl Pts',(34.7123780512931,-34.9678424712592,1.49981743040038));
#30130=CARTESIAN_POINT('Ctrl Pts',(34.591404591981,-34.9678425127826,1.49980840280397));
#30131=CARTESIAN_POINT('Ctrl Pts',(34.4539348326465,-34.9678425599684,1.49979814417772));
#30132=CARTESIAN_POINT('Ctrl Pts',(34.3249390274092,-34.9678425655798,1.49978830616205));
#30133=CARTESIAN_POINT('Ctrl Pts',(34.2036312646158,-34.9678425105859,1.49978156609768));
#30134=CARTESIAN_POINT('Ctrl Pts',(34.1284740534062,-34.967842476514,1.49977739023598));
#30135=CARTESIAN_POINT('Ctrl Pts',(34.0562692606603,-34.9678424188851,1.49977435262848));
#30136=CARTESIAN_POINT('Ctrl Pts',(33.9868395791739,-34.9678423310509,1.49977272195139));
#30137=CARTESIAN_POINT('Ctrl Pts',(33.944569913827,-34.9678422775764,1.49977172917462));
#30138=CARTESIAN_POINT('Ctrl Pts',(33.903332682828,-34.9678422127028,1.49977122168105));
#30139=CARTESIAN_POINT('Ctrl Pts',(33.8632274501546,-34.9678421281365,1.49977004757329));
#30140=CARTESIAN_POINT('Ctrl Pts',(33.8167531035319,-34.9678420301403,1.49976868700542));
#30141=CARTESIAN_POINT('Ctrl Pts',(33.771789463122,-34.9678419060139,1.49976648823776));
#30142=CARTESIAN_POINT('Ctrl Pts',(33.7281109635882,-34.9678417565821,1.49976414064438));
#30143=CARTESIAN_POINT('Ctrl Pts',(33.6812712011832,-34.9678415963351,1.49976162314223));
#30144=CARTESIAN_POINT('Ctrl Pts',(33.6359095723891,-34.9678414069824,1.49975893360226));
#30145=CARTESIAN_POINT('Ctrl Pts',(33.591810246565,-34.9678411881909,1.49975667024847));
#30146=CARTESIAN_POINT('Ctrl Pts',(33.5583448079856,-34.9678410221577,1.4997549526683));
#30147=CARTESIAN_POINT('Ctrl Pts',(33.5256076932742,-34.9678408391413,1.49975347489115));
#30148=CARTESIAN_POINT('Ctrl Pts',(33.4935243452377,-34.9678406385663,1.49975241817239));
#30149=CARTESIAN_POINT('Ctrl Pts',(33.4574180647961,-34.9678404128412,1.49975122895162));
#30150=CARTESIAN_POINT('Ctrl Pts',(33.4221459355308,-34.9678401647559,1.49975055002974));
#30151=CARTESIAN_POINT('Ctrl Pts',(33.3878318916215,-34.9678398888653,1.49974977143672));
#30152=CARTESIAN_POINT('Ctrl Pts',(33.3506903036195,-34.9678395902407,1.49974892868613));
#30153=CARTESIAN_POINT('Ctrl Pts',(33.3146710708563,-34.9678392590421,1.49974796966079));
#30154=CARTESIAN_POINT('Ctrl Pts',(33.2798677329257,-34.967838889585,1.49974635090117));
#30155=CARTESIAN_POINT('Ctrl Pts',(33.2432742079925,-34.9678385011241,1.49974464887706));
#30156=CARTESIAN_POINT('Ctrl Pts',(33.2080243245405,-34.9678380703783,1.49974221953695));
#30157=CARTESIAN_POINT('Ctrl Pts',(33.1741651388243,-34.9678375919209,1.49973865377071));
#30158=CARTESIAN_POINT('Ctrl Pts',(33.1370631468227,-34.96783706764,1.49973474649923));
#30159=CARTESIAN_POINT('Ctrl Pts',(33.101630651562,-34.9678364860775,1.49972947597289));
#30160=CARTESIAN_POINT('Ctrl Pts',(33.0678641021075,-34.9678358413429,1.49972253958675));
#30161=CARTESIAN_POINT('Ctrl Pts',(33.0456526984029,-34.967835417241,1.49971797687971));
#30162=CARTESIAN_POINT('Ctrl Pts',(33.0241607955795,-34.9678349658306,1.49971269819094));
#30163=CARTESIAN_POINT('Ctrl Pts',(33.0033754048768,-34.9678344856631,1.49970666036489));
#30164=CARTESIAN_POINT('Ctrl Pts',(32.9442530209621,-34.9678331198648,1.49968948625087));
#30165=CARTESIAN_POINT('Ctrl Pts',(32.8887085075052,-34.9678225692835,1.49991335207053));
#30166=CARTESIAN_POINT('Ctrl Pts',(32.8362583193005,-34.9678066670084,1.50027559162313));
#30167=CARTESIAN_POINT('Ctrl Pts',(32.7773090712612,-34.9677887942955,1.50068271598182));
#30168=CARTESIAN_POINT('Ctrl Pts',(32.7222687069611,-34.9677641462319,1.50126502290935));
#30169=CARTESIAN_POINT('Ctrl Pts',(32.6704155259707,-34.9677359487883,1.50193537623736));
#30170=CARTESIAN_POINT('Ctrl Pts',(32.6144302418903,-34.9677055043322,1.50265914902789));
#30171=CARTESIAN_POINT('Ctrl Pts',(32.5621602746537,-34.967670888482,1.50348644308882));
#30172=CARTESIAN_POINT('Ctrl Pts',(32.5126575741462,-34.9676341575402,1.50436077830379));
#30173=CARTESIAN_POINT('Ctrl Pts',(32.4592478825334,-34.967594527616,1.50530412025724));
#30174=CARTESIAN_POINT('Ctrl Pts',(32.4090594121703,-34.9675524017484,1.50630310623456));
#30175=CARTESIAN_POINT('Ctrl Pts',(32.3608584151776,-34.9675086790575,1.50733170420881));
#30176=CARTESIAN_POINT('Ctrl Pts',(32.3080624384018,-34.9674607883018,1.50845835797426));
#30177=CARTESIAN_POINT('Ctrl Pts',(32.2576510584102,-34.9674109512874,1.50962133088217));
#30178=CARTESIAN_POINT('Ctrl Pts',(32.2079531230122,-34.9673589385144,1.51082436306573));
#30179=CARTESIAN_POINT('Ctrl Pts',(32.1569814991443,-34.9673055927269,1.51205822727901));
#30180=CARTESIAN_POINT('Ctrl Pts',(32.1067603493753,-34.9672499217566,1.51333518230823));
#30181=CARTESIAN_POINT('Ctrl Pts',(32.0554367657627,-34.9671908102209,1.51468303813506));
#30182=CARTESIAN_POINT('Ctrl Pts',(32.0053752916503,-34.9671331523098,1.51599774854366));
#30183=CARTESIAN_POINT('Ctrl Pts',(31.9542650752303,-34.9670721879269,1.51738077462805));
#30184=CARTESIAN_POINT('Ctrl Pts',(31.9003392718779,-34.9670065776396,1.51886693662989));
#30185=CARTESIAN_POINT('Ctrl Pts',(31.8778362033484,-34.9669791986726,1.51948710736995));
#30186=CARTESIAN_POINT('Ctrl Pts',(31.8548422465646,-34.9669510097079,1.52012527669196));
#30187=CARTESIAN_POINT('Ctrl Pts',(31.8312262657831,-34.9669219190816,1.52078388908931));
#30188=CARTESIAN_POINT('Ctrl Pts',(31.7273802318769,-34.9667939995094,1.52367999092728));
#30189=CARTESIAN_POINT('Ctrl Pts',(31.6210019634565,-34.9666588880294,1.52670831990391));
#30190=CARTESIAN_POINT('Ctrl Pts',(31.5129311113833,-34.9665259706005,1.52968152042074));
#30191=CARTESIAN_POINT('Ctrl Pts',(31.4048670765169,-34.9663930615562,1.5326545333854));
#30192=CARTESIAN_POINT('Ctrl Pts',(31.295110396831,-34.9662624173991,1.53557057541601));
#30193=CARTESIAN_POINT('Ctrl Pts',(31.1845493642895,-34.9661438310284,1.53823056067685));
#30194=CARTESIAN_POINT('Ctrl Pts',(31.1321570104796,-34.9660876356498,1.5394910670751));
#30195=CARTESIAN_POINT('Ctrl Pts',(31.0795847658982,-34.9660341471942,1.54069407696174));
#30196=CARTESIAN_POINT('Ctrl Pts',(31.0269312050905,-34.9659843676727,1.54181935957433));
#30197=CARTESIAN_POINT('Ctrl Pts',(30.9325025960689,-34.9658950933502,1.5438374352796));
#30198=CARTESIAN_POINT('Ctrl Pts',(30.8378102330027,-34.9658178028119,1.54560383003055));
#30199=CARTESIAN_POINT('Ctrl Pts',(30.7433599242841,-34.9657577677723,1.54697518213503));
#30200=CARTESIAN_POINT('Ctrl Pts',(30.6608249248197,-34.965705306409,1.54817353232302));
#30201=CARTESIAN_POINT('Ctrl Pts',(30.5784749808876,-34.9656660234083,1.54907006656161));
#30202=CARTESIAN_POINT('Ctrl Pts',(30.4966730088978,-34.9656427667437,1.54959005157024));
#30203=CARTESIAN_POINT('',(30.5,-34.9699609326822,-1.44976976333441));
#30204=CARTESIAN_POINT('Origin',(30.5,0.,0.));
#30205=CARTESIAN_POINT('Ctrl Pts',(30.5051992612603,-34.9699071381489,-1.44903843638966));
#30206=CARTESIAN_POINT('Ctrl Pts',(30.6030952980657,-34.9698787568566,-1.44976082626917));
#30207=CARTESIAN_POINT('Ctrl Pts',(30.7001121880333,-34.9698264221104,-1.45104998650339));
#30208=CARTESIAN_POINT('Ctrl Pts',(30.7969947619801,-34.9697577270266,-1.45274237549662));
#30209=CARTESIAN_POINT('Ctrl Pts',(30.8545454823775,-34.9697169203944,-1.45374769773142));
#30210=CARTESIAN_POINT('Ctrl Pts',(30.9120492097055,-34.9696702850816,-1.45489634227782));
#30211=CARTESIAN_POINT('Ctrl Pts',(30.9696671110348,-34.9696190483589,-1.45616096255286));
#30212=CARTESIAN_POINT('Ctrl Pts',(31.0687356284601,-34.969530951673,-1.45833535719175));
#30213=CARTESIAN_POINT('Ctrl Pts',(31.1681385828748,-34.9694292858245,-1.46085179879274));
#30214=CARTESIAN_POINT('Ctrl Pts',(31.2685908593294,-34.9693191238307,-1.46356721252908));
#30215=CARTESIAN_POINT('Ctrl Pts',(31.3711796386319,-34.9692066188196,-1.46634037995092));
#30216=CARTESIAN_POINT('Ctrl Pts',(31.4748629185107,-34.9690851710714,-1.46932276608705));
#30217=CARTESIAN_POINT('Ctrl Pts',(31.5804543970555,-34.9689598486836,-1.4723695155306));
#30218=CARTESIAN_POINT('Ctrl Pts',(31.6427002532175,-34.9688859715162,-1.47416556508156));
#30219=CARTESIAN_POINT('Ctrl Pts',(31.7056101943812,-34.9688107472906,-1.47598400420448));
#30220=CARTESIAN_POINT('Ctrl Pts',(31.7693590594471,-34.9687353433411,-1.4777925610394));
#30221=CARTESIAN_POINT('Ctrl Pts',(31.8369567664635,-34.968655386873,-1.47971030961302));
#30222=CARTESIAN_POINT('Ctrl Pts',(31.8998289473023,-34.9685826953725,-1.48145356148269));
#30223=CARTESIAN_POINT('Ctrl Pts',(31.9584912820088,-34.9685172658125,-1.48302365833457));
#30224=CARTESIAN_POINT('Ctrl Pts',(32.0219681801233,-34.9684464662861,-1.48472261693203));
#30225=CARTESIAN_POINT('Ctrl Pts',(32.0805160965752,-34.9683841232145,-1.48621979971344));
#30226=CARTESIAN_POINT('Ctrl Pts',(32.1348442130228,-34.9683291276834,-1.48754049944253));
#30227=CARTESIAN_POINT('Ctrl Pts',(32.1955320114825,-34.9682676943422,-1.48901580107684));
#30228=CARTESIAN_POINT('Ctrl Pts',(32.2509543450045,-34.9682153821449,-1.49027186778449));
#30229=CARTESIAN_POINT('Ctrl Pts',(32.3021641802449,-34.968170114115,-1.49135570584805));
#30230=CARTESIAN_POINT('Ctrl Pts',(32.3568725417881,-34.9681217534879,-1.49251358898431));
#30231=CARTESIAN_POINT('Ctrl Pts',(32.4067738547341,-34.9680813901956,-1.49347579219532));
#30232=CARTESIAN_POINT('Ctrl Pts',(32.4532143425777,-34.9680466762592,-1.49429647043747));
#30233=CARTESIAN_POINT('Ctrl Pts',(32.5024778890134,-34.9680098521064,-1.49516703667327));
#30234=CARTESIAN_POINT('Ctrl Pts',(32.5478477692462,-34.9679793561973,-1.49587895592541));
#30235=CARTESIAN_POINT('Ctrl Pts',(32.5909873019042,-34.9679531603256,-1.49648137333639));
#30236=CARTESIAN_POINT('Ctrl Pts',(32.6362425762347,-34.9679256796997,-1.49711333579671));
#30237=CARTESIAN_POINT('Ctrl Pts',(32.6790438910183,-34.9679029082457,-1.49762527612471));
#30238=CARTESIAN_POINT('Ctrl Pts',(32.7213614276303,-34.9678837287556,-1.49804900699204));
#30239=CARTESIAN_POINT('Ctrl Pts',(32.7633326545687,-34.9678647062226,-1.49846927021664));
#30240=CARTESIAN_POINT('Ctrl Pts',(32.8048283340763,-34.9678491963778,-1.49880319667881));
#30241=CARTESIAN_POINT('Ctrl Pts',(32.8478112859697,-34.9678375791942,-1.49905168880698));
#30242=CARTESIAN_POINT('Ctrl Pts',(32.8880595868515,-34.9678267011162,-1.49928437142882));
#30243=CARTESIAN_POINT('Ctrl Pts',(32.9296120625675,-34.9678192143482,-1.49944259954574));
#30244=CARTESIAN_POINT('Ctrl Pts',(32.9741124736885,-34.9678170031322,-1.49949475964765));
#30245=CARTESIAN_POINT('Ctrl Pts',(32.9824658917633,-34.9678165880527,-1.49950455090861));
#30246=CARTESIAN_POINT('Ctrl Pts',(32.9909232824636,-34.9678163642396,-1.49951049395371));
#30247=CARTESIAN_POINT('Ctrl Pts',(32.9994956564547,-34.9678163521983,-1.4995122138931));
#30248=CARTESIAN_POINT('Ctrl Pts',(33.035916707601,-34.9678163010392,-1.49951952132052));
#30249=CARTESIAN_POINT('Ctrl Pts',(33.0737648470631,-34.9678163144541,-1.49952600456097));
#30250=CARTESIAN_POINT('Ctrl Pts',(33.1138039348094,-34.9678165569182,-1.49953164904712));
#30251=CARTESIAN_POINT('Ctrl Pts',(33.2457861392315,-34.9678173561608,-1.49955025515845));
#30252=CARTESIAN_POINT('Ctrl Pts',(33.3718058092168,-34.9678177616075,-1.49955552940343));
#30253=CARTESIAN_POINT('Ctrl Pts',(33.4990121011459,-34.9678181023247,-1.49956083536768));
#30254=CARTESIAN_POINT('Ctrl Pts',(33.6624238693915,-34.9678185400169,-1.49956765151637));
#30255=CARTESIAN_POINT('Ctrl Pts',(33.8277938592881,-34.9678188708891,-1.49957452000976));
#30256=CARTESIAN_POINT('Ctrl Pts',(33.9926457806311,-34.9678194856962,-1.49958605843696));
#30257=CARTESIAN_POINT('Ctrl Pts',(34.322349623317,-34.9678207153104,-1.49960913529135));
#30258=CARTESIAN_POINT('Ctrl Pts',(34.649981191788,-34.9678230806641,-1.49965089188094));
#30259=CARTESIAN_POINT('Ctrl Pts',(34.978743760729,-34.9678240597269,-1.499668413021));
#30260=CARTESIAN_POINT('Ctrl Pts',(35.1431250451995,-34.9678245492582,-1.49967717359104));
#30261=CARTESIAN_POINT('Ctrl Pts',(35.3077890797876,-34.9678246922169,-1.49967987529869));
#30262=CARTESIAN_POINT('Ctrl Pts',(35.4723919953983,-34.9678249110675,-1.49968390458378));
#30263=CARTESIAN_POINT('Ctrl Pts',(35.9662007422305,-34.9678255676192,-1.49969599243905));
#30264=CARTESIAN_POINT('Ctrl Pts',(36.4594594182669,-34.9678269071982,-1.49972002849122));
#30265=CARTESIAN_POINT('Ctrl Pts',(36.9527108273738,-34.9678287658476,-1.49975356610212));
#30266=CARTESIAN_POINT('Ctrl Pts',(38.1015495523822,-34.9678330948538,-1.49983167901864));
#30267=CARTESIAN_POINT('Ctrl Pts',(39.2503488559568,-34.9678402396984,-1.49996133572171));
#30268=CARTESIAN_POINT('Ctrl Pts',(40.4000634893725,-34.9678419791559,-1.49999290859452));
#30269=CARTESIAN_POINT('Ctrl Pts',(6.89999999997365,-9.46599415780712,-5.65979197164529));
#30270=CARTESIAN_POINT('Ctrl Pts',(6.99168932310453,-9.49787619923353,-5.60729410195164));
#30271=CARTESIAN_POINT('Ctrl Pts',(7.08405956072215,-9.52934434473076,-5.55450818731572));
#30272=CARTESIAN_POINT('Ctrl Pts',(8.15473535981986,-9.88659437915722,-4.94320927931172));
#30273=CARTESIAN_POINT('Ctrl Pts',(9.17052309187647,-10.1553288976265,-4.34956920012189));
#30274=CARTESIAN_POINT('Ctrl Pts',(11.249912418623,-10.5681406908193,-3.24757657546859));
#30275=CARTESIAN_POINT('Ctrl Pts',(12.2613271155137,-10.7096926815135,-2.71507294053766));
#30276=CARTESIAN_POINT('Ctrl Pts',(14.3530613265277,-10.9182780492489,-1.75089621035865));
#30277=CARTESIAN_POINT('Ctrl Pts',(15.3683896576347,-10.9736589531833,-1.30024364084097));
#30278=CARTESIAN_POINT('Ctrl Pts',(17.4699484560063,-11.0479347559914,-0.511606508085749));
#30279=CARTESIAN_POINT('Ctrl Pts',(18.4899441076999,-11.0518486975415,-0.154966618543406));
#30280=CARTESIAN_POINT('Ctrl Pts',(19.8459385111079,-11.0525063200436,0.227738630131173));
#30281=CARTESIAN_POINT('Ctrl Pts',(20.3436052070642,-11.0499443867429,0.36401229334755));
#30282=CARTESIAN_POINT('Ctrl Pts',(21.3765735172499,-11.0391187302377,0.626365466004487));
#30283=CARTESIAN_POINT('Ctrl Pts',(22.1786513408684,-11.0271780970655,0.801482370854041));
#30284=CARTESIAN_POINT('Ctrl Pts',(22.8524711894103,-11.0190184236597,0.927590054426943));
#30285=CARTESIAN_POINT('Ctrl Pts',(23.1034772575406,-11.015636270466,0.973361071581969));
#30286=CARTESIAN_POINT('Ctrl Pts',(23.6153488598143,-11.0082046691873,1.06157978958535));
#30287=CARTESIAN_POINT('Ctrl Pts',(24.2640912191231,-10.9980907558832,1.16309571993124));
#30288=CARTESIAN_POINT('Ctrl Pts',(24.9252112071703,-10.9882975006411,1.25112898708133));
#30289=CARTESIAN_POINT('Ctrl Pts',(25.3924209938587,-10.9823391891697,1.30426168416562));
#30290=CARTESIAN_POINT('Ctrl Pts',(25.6607104515486,-10.9792975977554,1.332046615497));
#30291=CARTESIAN_POINT('Ctrl Pts',(25.7950739758558,-10.9779150347045,1.34502686686554));
#30292=CARTESIAN_POINT('Ctrl Pts',(26.2512918422651,-10.9735046934062,1.38748529291552));
#30293=CARTESIAN_POINT('Ctrl Pts',(27.3073301682004,-10.9653764904263,1.45732017866833));
#30294=CARTESIAN_POINT('Ctrl Pts',(28.3319194320811,-10.9609947024269,1.48237708919284));
#30295=CARTESIAN_POINT('Ctrl Pts',(29.1280123944214,-10.9582092660149,1.50394716937725));
#30296=CARTESIAN_POINT('Ctrl Pts',(29.4779818455993,-10.9573324846489,1.51103964894258));
#30297=CARTESIAN_POINT('Ctrl Pts',(29.9466600480359,-10.9567800220405,1.51533483257754));
#30298=CARTESIAN_POINT('Ctrl Pts',(30.4585980273686,-10.956656708735,1.51632751174059));
#30299=CARTESIAN_POINT('Ctrl Pts',(31.4732549878281,-10.9572594965941,1.51158385370564));
#30300=CARTESIAN_POINT('Ctrl Pts',(32.3455845021632,-10.95879335959,1.4999511927851));
#30301=CARTESIAN_POINT('Ctrl Pts',(33.1628510802405,-10.9587933798862,1.49997453311311));
#30302=CARTESIAN_POINT('Ctrl Pts',(33.4532441810442,-10.9587933789851,1.49997366471359));
#30303=CARTESIAN_POINT('Ctrl Pts',(33.7813843869345,-10.9587933812939,1.49997637381128));
#30304=CARTESIAN_POINT('Ctrl Pts',(34.2755379701535,-10.9587933817727,1.49997699476315));
#30305=CARTESIAN_POINT('Ctrl Pts',(34.8102302793009,-10.9587933869434,1.49998326277599));
#30306=CARTESIAN_POINT('Ctrl Pts',(35.6332452367756,-10.9587933876415,1.49998412101817));
#30307=CARTESIAN_POINT('Ctrl Pts',(36.2915450349079,-10.9587933890033,1.49998577371297));
#30308=CARTESIAN_POINT('Ctrl Pts',(38.1020137670942,-10.9587933908629,1.49998803993575));
#30309=CARTESIAN_POINT('Ctrl Pts',(39.5833333333333,-10.9587934006931,1.5));
#30310=CARTESIAN_POINT('Ctrl Pts',(40.9,-10.9587934006931,1.5));
#30311=CARTESIAN_POINT('Ctrl Pts',(6.65963435785827,-13.0027682689653,-8.56288377493212));
#30312=CARTESIAN_POINT('Ctrl Pts',(6.7513219377677,-13.050957789036,-8.49067817166156));
#30313=CARTESIAN_POINT('Ctrl Pts',(6.84370278928156,-13.0985893115687,-8.41801298642698));
#30314=CARTESIAN_POINT('Ctrl Pts',(7.91483960325935,-13.6397807532085,-7.57680655910808));
#30315=CARTESIAN_POINT('Ctrl Pts',(8.9325509112231,-14.0543934435321,-6.75518385076231));
#30316=CARTESIAN_POINT('Ctrl Pts',(11.0192135814157,-14.7040310435559,-5.22065437877307));
#30317=CARTESIAN_POINT('Ctrl Pts',(12.0340542508324,-14.9356992206141,-4.4769598695545));
#30318=CARTESIAN_POINT('Ctrl Pts',(14.1407660172285,-15.2883456800052,-3.1214593369057));
#30319=CARTESIAN_POINT('Ctrl Pts',(15.1616568764318,-15.3931503655329,-2.48732138966201));
#30320=CARTESIAN_POINT('Ctrl Pts',(17.287218760307,-15.5446125872455,-1.36959877283814));
#30321=CARTESIAN_POINT('Ctrl Pts',(18.3145546794907,-15.5707395254148,-0.864902786641509));
#30322=CARTESIAN_POINT('Ctrl Pts',(19.6926214867647,-15.5935126543779,-0.318801403605145));
#30323=CARTESIAN_POINT('Ctrl Pts',(20.19452636269,-15.5977145841048,-0.125373946234776));
#30324=CARTESIAN_POINT('Ctrl Pts',(21.2420076978203,-15.5972978704292,0.248868189963684));
#30325=CARTESIAN_POINT('Ctrl Pts',(22.0575126096201,-15.5901933457539,0.499284562147393));
#30326=CARTESIAN_POINT('Ctrl Pts',(22.7441078663834,-15.5856475377419,0.679992377552246));
#30327=CARTESIAN_POINT('Ctrl Pts',(22.9980856324395,-15.5834353094767,0.745267685418835));
#30328=CARTESIAN_POINT('Ctrl Pts',(23.5177883906687,-15.5778337615218,0.871419538176182));
#30329=CARTESIAN_POINT('Ctrl Pts',(24.1766640555165,-15.569151455817,1.01665680544525));
#30330=CARTESIAN_POINT('Ctrl Pts',(24.8496697365589,-15.560128822227,1.14287321247013));
#30331=CARTESIAN_POINT('Ctrl Pts',(25.3259254544069,-15.554601684436,1.21914041353961));
#30332=CARTESIAN_POINT('Ctrl Pts',(25.5996882691236,-15.5518109321211,1.2590574298324));
#30333=CARTESIAN_POINT('Ctrl Pts',(25.7368188560809,-15.550561003587,1.27770917936971));
#30334=CARTESIAN_POINT('Ctrl Pts',(26.2030586507879,-15.5466206431081,1.33878235986071));
#30335=CARTESIAN_POINT('Ctrl Pts',(27.2845562696213,-15.5388831179539,1.43928616936987));
#30336=CARTESIAN_POINT('Ctrl Pts',(28.3146233763975,-15.534108117874,1.47473229777558));
#30337=CARTESIAN_POINT('Ctrl Pts',(29.1121433593266,-15.5313810124223,1.5053783917148));
#30338=CARTESIAN_POINT('Ctrl Pts',(29.4693616319656,-15.5305221749293,1.51558516408219));
#30339=CARTESIAN_POINT('Ctrl Pts',(29.9425518103672,-15.5299808253862,1.5216968643791));
#30340=CARTESIAN_POINT('Ctrl Pts',(30.4595136734855,-15.5298599056894,1.52312339822458));
#30341=CARTESIAN_POINT('Ctrl Pts',(31.4800666545032,-15.5304501241615,1.51634797661239));
#30342=CARTESIAN_POINT('Ctrl Pts',(32.3507119180564,-15.5319509809364,1.4999128955352));
#30343=CARTESIAN_POINT('Ctrl Pts',(33.1621363777215,-15.5319505779396,1.49995461572564));
#30344=CARTESIAN_POINT('Ctrl Pts',(33.4535196029878,-15.5319505880019,1.49995304854269));
#30345=CARTESIAN_POINT('Ctrl Pts',(33.7812306484551,-15.5319505396377,1.49995788616631));
#30346=CARTESIAN_POINT('Ctrl Pts',(34.2755524327802,-15.531950526851,1.49995898984267));
#30347=CARTESIAN_POINT('Ctrl Pts',(34.8101578274898,-15.5319504091692,1.4999701650853));
#30348=CARTESIAN_POINT('Ctrl Pts',(35.6332135248365,-15.5319503927198,1.49997169422773));
#30349=CARTESIAN_POINT('Ctrl Pts',(36.2914988048216,-15.5319503616369,1.49997464065556));
#30350=CARTESIAN_POINT('Ctrl Pts',(38.1019885414694,-15.5319503187541,1.49997868009126));
#30351=CARTESIAN_POINT('Ctrl Pts',(39.5833333333333,-15.5319500929849,1.5));
#30352=CARTESIAN_POINT('Ctrl Pts',(40.9,-15.5319500929849,1.5));
#30353=CARTESIAN_POINT('Ctrl Pts',(6.47503677058814,-19.2049631177014,-13.6264850125633));
#30354=CARTESIAN_POINT('Ctrl Pts',(6.56582707216344,-19.2807931407427,-13.5206117629928));
#30355=CARTESIAN_POINT('Ctrl Pts',(6.65722187862393,-19.3557456396964,-13.4141026801341));
#30356=CARTESIAN_POINT('Ctrl Pts',(7.71979853459931,-20.2113974185276,-12.1774082172639));
#30357=CARTESIAN_POINT('Ctrl Pts',(8.72714740265586,-20.876585861408,-10.9649265084515));
#30358=CARTESIAN_POINT('Ctrl Pts',(10.792252425961,-21.9312131301472,-8.69413764846817));
#30359=CARTESIAN_POINT('Ctrl Pts',(11.8008983729842,-22.3203974544121,-7.58577239973431));
#30360=CARTESIAN_POINT('Ctrl Pts',(13.892634394048,-22.9231109701401,-5.56042793834188));
#30361=CARTESIAN_POINT('Ctrl Pts',(14.910936596525,-23.1162450123325,-4.60683703173286));
#30362=CARTESIAN_POINT('Ctrl Pts',(17.0374816014601,-23.4053158267904,-2.91606182242837));
#30363=CARTESIAN_POINT('Ctrl Pts',(18.0678529336714,-23.4724397837998,-2.15006970557795));
#30364=CARTESIAN_POINT('Ctrl Pts',(19.4632774216583,-23.5361137002685,-1.31129970902877));
#30365=CARTESIAN_POINT('Ctrl Pts',(19.9690853949367,-23.5527456051548,-1.01646669656859));
#30366=CARTESIAN_POINT('Ctrl Pts',(21.0306109698709,-23.5717577824589,-0.441678056412671));
#30367=CARTESIAN_POINT('Ctrl Pts',(21.8626014988188,-23.5739085372705,-0.0543003442681394));
#30368=CARTESIAN_POINT('Ctrl Pts',(22.5665651705188,-23.576178914363,0.226484889079846));
#30369=CARTESIAN_POINT('Ctrl Pts',(22.8246411038756,-23.5761448043361,0.326902916553467));
#30370=CARTESIAN_POINT('Ctrl Pts',(23.3554232774669,-23.5740054132278,0.522054743089696));
#30371=CARTESIAN_POINT('Ctrl Pts',(24.0293769285439,-23.5680817805141,0.74700585878865));
#30372=CARTESIAN_POINT('Ctrl Pts',(24.7209631427047,-23.560586503548,0.943393581394333));
#30373=CARTESIAN_POINT('Ctrl Pts',(25.2118242719342,-23.5558940963915,1.06233480615607));
#30374=CARTESIAN_POINT('Ctrl Pts',(25.4945546545947,-23.5535795021665,1.12470144437592));
#30375=CARTESIAN_POINT('Ctrl Pts',(25.6362544160062,-23.5525764277763,1.15385183559377));
#30376=CARTESIAN_POINT('Ctrl Pts',(26.1191683853685,-23.5495095529483,1.24953281052836));
#30377=CARTESIAN_POINT('Ctrl Pts',(27.244410780189,-23.5425023713064,1.40715534997208));
#30378=CARTESIAN_POINT('Ctrl Pts',(28.2843056152442,-23.5370396227258,1.46065929315376));
#30379=CARTESIAN_POINT('Ctrl Pts',(29.0843244121809,-23.5344215873996,1.50737208683505));
#30380=CARTESIAN_POINT('Ctrl Pts',(29.4542021761287,-23.5335942286398,1.52336782189617));
#30381=CARTESIAN_POINT('Ctrl Pts',(29.9352997409898,-23.5330734925559,1.53271512054377));
#30382=CARTESIAN_POINT('Ctrl Pts',(30.4610555884278,-23.532957187389,1.5349453613852));
#30383=CARTESIAN_POINT('Ctrl Pts',(31.4919316519535,-23.5335262680548,1.52450364515754));
#30384=CARTESIAN_POINT('Ctrl Pts',(32.3596576160514,-23.5349731541844,1.49979324124414));
#30385=CARTESIAN_POINT('Ctrl Pts',(33.1608710165812,-23.5349736853906,1.49989213988255));
#30386=CARTESIAN_POINT('Ctrl Pts',(33.4539865796869,-23.5349736699323,1.49988845489238));
#30387=CARTESIAN_POINT('Ctrl Pts',(33.780948091659,-23.5349737329761,1.49989993226727));
#30388=CARTESIAN_POINT('Ctrl Pts',(34.275564602361,-23.5349737489117,1.49990256114204));
#30389=CARTESIAN_POINT('Ctrl Pts',(34.810021467207,-23.5349738998239,1.49992910993535));
#30390=CARTESIAN_POINT('Ctrl Pts',(35.6331489543767,-23.5349739207807,1.49993274473986));
#30391=CARTESIAN_POINT('Ctrl Pts',(36.2914097700016,-23.5349739606187,1.4999397448351));
#30392=CARTESIAN_POINT('Ctrl Pts',(38.1019375614968,-23.5349740154737,1.49994934328327));
#30393=CARTESIAN_POINT('Ctrl Pts',(39.5833333333333,-23.5349743044955,1.5));
#30394=CARTESIAN_POINT('Ctrl Pts',(40.9,-23.5349743044955,1.5));
#30395=CARTESIAN_POINT('Ctrl Pts',(6.39840282685635,-25.4797798158266,-18.5950148818));
#30396=CARTESIAN_POINT('Ctrl Pts',(6.48879582230594,-25.5825069307027,-18.455456538043));
#30397=CARTESIAN_POINT('Ctrl Pts',(6.57973810483189,-25.684006582131,-18.3151558806717));
#30398=CARTESIAN_POINT('Ctrl Pts',(7.63881202209715,-26.8457843562122,-16.6821095714367));
#30399=CARTESIAN_POINT('Ctrl Pts',(8.64206536867565,-27.7524045864227,-15.0805562774161));
#30400=CARTESIAN_POINT('Ctrl Pts',(10.6943835463645,-29.194220471563,-12.08639394536));
#30401=CARTESIAN_POINT('Ctrl Pts',(11.6986850371144,-29.7340826089764,-10.6188960618635));
#30402=CARTESIAN_POINT('Ctrl Pts',(13.7736723466472,-30.5724457120527,-7.9480571508383));
#30403=CARTESIAN_POINT('Ctrl Pts',(14.7865355152845,-30.8496813329458,-6.68379951334874));
#30404=CARTESIAN_POINT('Ctrl Pts',(16.895644387614,-31.2681094727719,-4.44867953439714));
#30405=CARTESIAN_POINT('Ctrl Pts',(17.921113585793,-31.3748718553479,-3.42955614780409));
#30406=CARTESIAN_POINT('Ctrl Pts',(19.3111115725317,-31.4778602005301,-2.31180057560694));
#30407=CARTESIAN_POINT('Ctrl Pts',(19.8164097330209,-31.5068304778962,-1.91755167896535));
#30408=CARTESIAN_POINT('Ctrl Pts',(20.8772665291465,-31.5450009606978,-1.1480473205349));
#30409=CARTESIAN_POINT('Ctrl Pts',(21.7126526899651,-31.5565752055434,-0.625757760628935));
#30410=CARTESIAN_POINT('Ctrl Pts',(22.4233939916368,-31.5658469864011,-0.244774266221902));
#30411=CARTESIAN_POINT('Ctrl Pts',(22.68321700305,-31.568070163829,-0.109074102068982));
#30412=CARTESIAN_POINT('Ctrl Pts',(23.2191843843282,-31.5695528321153,0.155714853804437));
#30413=CARTESIAN_POINT('Ctrl Pts',(23.9014490792895,-31.5665856540486,0.461901703286711));
#30414=CARTESIAN_POINT('Ctrl Pts',(24.6052033552109,-31.5607844376464,0.730987709817269));
#30415=CARTESIAN_POINT('Ctrl Pts',(25.1069219885717,-31.5570192016244,0.894795181267933));
#30416=CARTESIAN_POINT('Ctrl Pts',(25.3966703145091,-31.5552253028176,0.98095784259731));
#30417=CARTESIAN_POINT('Ctrl Pts',(25.5420691491796,-31.5544886793522,1.02128571697646));
#30418=CARTESIAN_POINT('Ctrl Pts',(26.0386675456483,-31.5523567719375,1.15405115562807));
#30419=CARTESIAN_POINT('Ctrl Pts',(27.2041996425261,-31.5461367082151,1.37405103438869));
#30420=CARTESIAN_POINT('Ctrl Pts',(28.254481539011,-31.5399727189289,1.44553527377015));
#30421=CARTESIAN_POINT('Ctrl Pts',(29.0567817440806,-31.5374655658645,1.50856328668892));
#30422=CARTESIAN_POINT('Ctrl Pts',(29.4392037716731,-31.5366692491296,1.53093305020556));
#30423=CARTESIAN_POINT('Ctrl Pts',(29.9281985709061,-31.536168682902,1.54360558359609));
#30424=CARTESIAN_POINT('Ctrl Pts',(30.4627354290944,-31.5360567738141,1.54671304059522));
#30425=CARTESIAN_POINT('Ctrl Pts',(31.5039222132188,-31.5366047697957,1.53240580330097));
#30426=CARTESIAN_POINT('Ctrl Pts',(32.3686614831274,-31.5379963364647,1.49961223537189));
#30427=CARTESIAN_POINT('Ctrl Pts',(33.1596379899179,-31.5379973429874,1.49979803313559));
#30428=CARTESIAN_POINT('Ctrl Pts',(33.4544864001145,-31.5379973136915,1.49979103760184));
#30429=CARTESIAN_POINT('Ctrl Pts',(33.7806952343975,-31.5379974331442,1.49981257637976));
#30430=CARTESIAN_POINT('Ctrl Pts',(34.2756055948936,-31.5379974633363,1.49981748473541));
#30431=CARTESIAN_POINT('Ctrl Pts',(34.8099061252942,-31.5379977492716,1.49986722177693));
#30432=CARTESIAN_POINT('Ctrl Pts',(35.6331043028646,-31.5379977889784,1.49987402634113));
#30433=CARTESIAN_POINT('Ctrl Pts',(36.2913385913736,-31.5379978644599,1.49988713966987));
#30434=CARTESIAN_POINT('Ctrl Pts',(38.1019015852784,-31.537997968394,1.49990511666357));
#30435=CARTESIAN_POINT('Ctrl Pts',(39.5833333333333,-31.5379985160061,1.5));
#30436=CARTESIAN_POINT('Ctrl Pts',(40.9,-31.5379985160061,1.5));
#30437=CARTESIAN_POINT('Ctrl Pts',(6.37427268165564,-28.1741189428499,-20.7176664141567));
#30438=CARTESIAN_POINT('Ctrl Pts',(6.46448755772838,-28.2883460540946,-20.5636424771022));
#30439=CARTESIAN_POINT('Ctrl Pts',(6.55522687426754,-28.4011972468989,-20.4088293925213));
#30440=CARTESIAN_POINT('Ctrl Pts',(7.61282240204204,-29.6937878962761,-18.6056139772311));
#30441=CARTESIAN_POINT('Ctrl Pts',(8.61454082730176,-30.703424507615,-16.8370699794085));
#30442=CARTESIAN_POINT('Ctrl Pts',(10.6618274824665,-32.3104201819496,-13.5325068155167));
#30443=CARTESIAN_POINT('Ctrl Pts',(11.6645377987076,-32.9144254040795,-11.9110180488693));
#30444=CARTESIAN_POINT('Ctrl Pts',(13.7331445959134,-33.8529424117878,-8.96386257277558));
#30445=CARTESIAN_POINT('Ctrl Pts',(14.7439932704909,-34.1658004948675,-7.56674532731094));
#30446=CARTESIAN_POINT('Ctrl Pts',(16.8461035490385,-34.6388264066738,-5.10012840374637));
#30447=CARTESIAN_POINT('Ctrl Pts',(17.8695058124616,-34.7622645166785,-3.97333364734334));
#30448=CARTESIAN_POINT('Ctrl Pts',(19.2561174443541,-34.8817349492475,-2.73821070416468));
#30449=CARTESIAN_POINT('Ctrl Pts',(19.7609345646798,-34.9159214541564,-2.30176586395498));
#30450=CARTESIAN_POINT('Ctrl Pts',(20.8205141053453,-34.9621410370326,-1.45015687002428));
#30451=CARTESIAN_POINT('Ctrl Pts',(21.6560023791939,-34.9776907709078,-0.871078443386996));
#30452=CARTESIAN_POINT('Ctrl Pts',(22.3682688599883,-34.989939594886,-0.447778285927136));
#30453=CARTESIAN_POINT('Ctrl Pts',(22.6285200842947,-34.9931281975259,-0.297086276283262));
#30454=CARTESIAN_POINT('Ctrl Pts',(23.1658603614091,-34.9961605697035,-0.00273379297027992));
#30455=CARTESIAN_POINT('Ctrl Pts',(23.8505975407037,-34.9944676948756,0.338068372298851));
#30456=CARTESIAN_POINT('Ctrl Pts',(24.5583968797874,-34.9894056975888,0.638319272935676));
#30457=CARTESIAN_POINT('Ctrl Pts',(25.0640148551739,-34.9860476379143,0.821498314632841));
#30458=CARTESIAN_POINT('Ctrl Pts',(25.3563632502514,-34.9844821378475,0.917977493583092));
#30459=CARTESIAN_POINT('Ctrl Pts',(25.503160007456,-34.9838621425449,0.963163948801066));
#30460=CARTESIAN_POINT('Ctrl Pts',(26.0049713545738,-34.982139121313,1.11209382847184));
#30461=CARTESIAN_POINT('Ctrl Pts',(27.1869304722337,-34.9762666166019,1.35965020681436));
#30462=CARTESIAN_POINT('Ctrl Pts',(28.2418054197051,-34.9698003983093,1.43886806122646));
#30463=CARTESIAN_POINT('Ctrl Pts',(29.0450356043991,-34.9673414359535,1.5089275405599));
#30464=CARTESIAN_POINT('Ctrl Pts',(29.4328041419752,-34.9665583691038,1.53413528152413));
#30465=CARTESIAN_POINT('Ctrl Pts',(29.9251825362975,-34.9660664512209,1.54824951859995));
#30466=CARTESIAN_POINT('Ctrl Pts',(30.4634799414205,-34.9659564211645,1.55174636239756));
#30467=CARTESIAN_POINT('Ctrl Pts',(31.5090833787051,-34.9664954410524,1.53574598606796));
#30468=CARTESIAN_POINT('Ctrl Pts',(32.3725304400172,-34.9678633362529,1.49952340891733));
#30469=CARTESIAN_POINT('Ctrl Pts',(33.1591152593399,-34.9678645826042,1.49975189997366));
#30470=CARTESIAN_POINT('Ctrl Pts',(33.4547063903441,-34.9678645463389,1.49974326694616));
#30471=CARTESIAN_POINT('Ctrl Pts',(33.7805921021893,-34.9678646942577,1.49976974530861));
#30472=CARTESIAN_POINT('Ctrl Pts',(34.2756282408745,-34.9678647316484,1.49977576894615));
#30473=CARTESIAN_POINT('Ctrl Pts',(34.8098603973427,-34.967865085736,1.49983687714898));
#30474=CARTESIAN_POINT('Ctrl Pts',(35.6330886763766,-34.9678651349076,1.49984523535833));
#30475=CARTESIAN_POINT('Ctrl Pts',(36.2913112329655,-34.9678652283802,1.49986134640235));
#30476=CARTESIAN_POINT('Ctrl Pts',(38.1018888107018,-34.9678653570876,1.49988343135295));
#30477=CARTESIAN_POINT('Ctrl Pts',(39.5833333333333,-34.9678660352249,1.5));
#30478=CARTESIAN_POINT('Ctrl Pts',(40.9,-34.9678660352249,1.5));
#30479=CARTESIAN_POINT('',(40.9,-32.9658914637539,1.50000000000002));
#30480=CARTESIAN_POINT('Ctrl Pts',(40.9,-32.9658914637539,1.50000000000002));
#30481=CARTESIAN_POINT('Ctrl Pts',(40.9,-33.466386268912,1.50000000000002));
#30482=CARTESIAN_POINT('Ctrl Pts',(40.9,-33.9668810740701,1.50000000000002));
#30483=CARTESIAN_POINT('Ctrl Pts',(40.9,-34.4673758792282,1.50000000000002));
#30484=CARTESIAN_POINT('',(38.,-32.9658914637539,1.49999999999999));
#30485=CARTESIAN_POINT('Ctrl Pts',(38.,-32.9658914637539,1.5));
#30486=CARTESIAN_POINT('Ctrl Pts',(38.9666666666667,-32.9658914637539,1.5));
#30487=CARTESIAN_POINT('Ctrl Pts',(39.9333333333333,-32.9658914637539,1.5));
#30488=CARTESIAN_POINT('Ctrl Pts',(40.9,-32.9658914637539,1.5));
#30489=CARTESIAN_POINT('Ctrl Pts',(37.4997714574611,-32.3652585803353,1.49990106437153));
#30490=CARTESIAN_POINT('Ctrl Pts',(37.6667294826967,-32.5658056765356,1.4999047077905));
#30491=CARTESIAN_POINT('Ctrl Pts',(37.8334450600886,-32.7660568372682,1.49990923999261));
#30492=CARTESIAN_POINT('Ctrl Pts',(37.9998166694663,-32.9658909678229,1.49991439209149));
#30493=CARTESIAN_POINT('',(6.9,-24.7737885487526,-16.9192021366758));
#30494=CARTESIAN_POINT('Ctrl Pts',(6.9,-24.7737885487526,-16.9192021366758));
#30495=CARTESIAN_POINT('Ctrl Pts',(6.9,-22.645444622876,-15.3881766950258));
#30496=CARTESIAN_POINT('Ctrl Pts',(6.90000000000115,-20.4978726403359,-13.8353835251886));
#30497=CARTESIAN_POINT('Ctrl Pts',(6.90000000000115,-15.662481608859,-10.3082122779765));
#30498=CARTESIAN_POINT('Ctrl Pts',(6.9,-12.4764228571341,-7.95935811114668));
#30499=CARTESIAN_POINT('Ctrl Pts',(6.9,-9.46599415782505,-5.6597919716369));
#30500=CARTESIAN_POINT('',(22.9245129145126,-31.7706052331164,3.89077700057102E-15));
#30501=CARTESIAN_POINT('Ctrl Pts',(22.9245129145126,-31.7706052331164,8.19538942818498E-15));
#30502=CARTESIAN_POINT('Ctrl Pts',(22.7202811020963,-31.7014549124251,-0.0979233563002608));
#30503=CARTESIAN_POINT('Ctrl Pts',(22.5089075447093,-31.6320805544326,-0.203440182623869));
#30504=CARTESIAN_POINT('Ctrl Pts',(22.2913349439917,-31.5632247707622,-0.316637134194163));
#30505=CARTESIAN_POINT('Ctrl Pts',(21.4451770585293,-31.2954389184984,-0.756869465221139));
#30506=CARTESIAN_POINT('Ctrl Pts',(20.5220951556669,-31.0475106147151,-1.35418571023217));
#30507=CARTESIAN_POINT('Ctrl Pts',(19.767142881954,-30.8612920963158,-1.89915402350694));
#30508=CARTESIAN_POINT('Ctrl Pts',(19.5194773058392,-30.8002022522972,-2.07793339270825));
#30509=CARTESIAN_POINT('Ctrl Pts',(19.2865716386091,-30.7444068279678,-2.2520483595932));
#30510=CARTESIAN_POINT('Ctrl Pts',(19.0728538401323,-30.6939488833522,-2.41532203906683));
#30511=CARTESIAN_POINT('Ctrl Pts',(18.7028555998036,-30.6065937315988,-2.69798906318808));
#30512=CARTESIAN_POINT('Ctrl Pts',(18.4144703596236,-30.539966063932,-2.9337393828771));
#30513=CARTESIAN_POINT('Ctrl Pts',(18.0642874871539,-30.4582462938821,-3.23398234069981));
#30514=CARTESIAN_POINT('Ctrl Pts',(17.4420927116722,-30.3130489756353,-3.76744532366912));
#30515=CARTESIAN_POINT('Ctrl Pts',(16.7224564418219,-30.1446863488622,-4.43872907330226));
#30516=CARTESIAN_POINT('Ctrl Pts',(15.9202806616111,-29.9321297384067,-5.24401550821529));
#30517=CARTESIAN_POINT('Ctrl Pts',(15.4090529834519,-29.7966671314304,-5.75722561070116));
#30518=CARTESIAN_POINT('Ctrl Pts',(14.8739602945715,-29.6418940055915,-6.33424649579652));
#30519=CARTESIAN_POINT('Ctrl Pts',(14.3169794331156,-29.4557634846122,-6.96996102647202));
#30520=CARTESIAN_POINT('Ctrl Pts',(13.8864206762837,-29.3118803976569,-7.4613826837838));
#30521=CARTESIAN_POINT('Ctrl Pts',(13.3867890027805,-29.1311705407939,-8.05270459511993));
#30522=CARTESIAN_POINT('Ctrl Pts',(12.8146824059514,-28.8915984033895,-8.75043091662868));
#30523=CARTESIAN_POINT('Ctrl Pts',(12.2526665517595,-28.6562518085588,-9.4358508309389));
#30524=CARTESIAN_POINT('Ctrl Pts',(11.6379478462804,-28.3625845909803,-10.231366276768));
#30525=CARTESIAN_POINT('Ctrl Pts',(10.9739250490309,-27.981021293096,-11.1267230319105));
#30526=CARTESIAN_POINT('Ctrl Pts',(10.5683455447964,-27.747965660321,-11.6735993596027));
#30527=CARTESIAN_POINT('Ctrl Pts',(10.1437415406956,-27.4801235315866,-12.2581093618546));
#30528=CARTESIAN_POINT('Ctrl Pts',(9.74137929176525,-27.2046666925187,-12.8142541611144));
#30529=CARTESIAN_POINT('Ctrl Pts',(8.72285779294234,-26.5073877769786,-14.2220538143138));
#30530=CARTESIAN_POINT('Ctrl Pts',(7.81323138778195,-25.7100913255874,-15.580948814124));
#30531=CARTESIAN_POINT('Ctrl Pts',(6.9,-24.7737885487526,-16.9192021366758));
#30532=CARTESIAN_POINT('Ctrl Pts',(30.5,-34.9656486014478,1.55029606206997));
#30533=CARTESIAN_POINT('Ctrl Pts',(29.9560179420817,-34.7222276068062,1.55343104498103));
#30534=CARTESIAN_POINT('Ctrl Pts',(29.4152668325132,-34.4790656554127,1.54030953139106));
#30535=CARTESIAN_POINT('Ctrl Pts',(28.8740459957565,-34.2361296888632,1.49470250846617));
#30536=CARTESIAN_POINT('Ctrl Pts',(28.3535277923439,-34.0024864433252,1.45084003307051));
#30537=CARTESIAN_POINT('Ctrl Pts',(27.8179515912466,-33.7608540997398,1.40923473841146));
#30538=CARTESIAN_POINT('Ctrl Pts',(27.2695051149491,-33.5168388499063,1.33972398862116));
#30539=CARTESIAN_POINT('Ctrl Pts',(26.9554553615883,-33.3771115796287,1.29992095446743));
#30540=CARTESIAN_POINT('Ctrl Pts',(26.6378099296971,-33.2369493090937,1.25106463707208));
#30541=CARTESIAN_POINT('Ctrl Pts',(26.3179304017917,-33.0983258448229,1.18777049128279));
#30542=CARTESIAN_POINT('Ctrl Pts',(26.1078196745982,-33.0072719500184,1.14619615520081));
#30543=CARTESIAN_POINT('Ctrl Pts',(25.8967402232745,-32.9168907470981,1.09839525532295));
#30544=CARTESIAN_POINT('Ctrl Pts',(25.6850706236774,-32.8277596053404,1.04282885388103));
#30545=CARTESIAN_POINT('Ctrl Pts',(25.6562210027417,-32.8156114288513,1.03525540156945));
#30546=CARTESIAN_POINT('Ctrl Pts',(25.6277737638215,-32.8036595933923,1.0276506122434));
#30547=CARTESIAN_POINT('Ctrl Pts',(25.5983858063598,-32.7913423709803,1.01964325944536));
#30548=CARTESIAN_POINT('Ctrl Pts',(25.1249357452756,-32.5929076988546,0.890642063078175));
#30549=CARTESIAN_POINT('Ctrl Pts',(24.1510084067019,-32.1858811669087,0.588069770626606));
#30550=CARTESIAN_POINT('Ctrl Pts',(22.9245129145126,-31.7706052331164,8.19538942818498E-15));
#30551=CARTESIAN_POINT('Origin',(40.65,0.,0.));
#30552=CARTESIAN_POINT('',(40.4,-29.5330398077868,-18.7829592905825));
#30553=CARTESIAN_POINT('',(40.9,-29.0996231131986,-18.5327260452907));
#30554=CARTESIAN_POINT('Ctrl Pts',(40.4,-29.5330398077868,-18.7829592905825));
#30555=CARTESIAN_POINT('Ctrl Pts',(40.5666590133561,-29.3885761367562,-18.6995531512249));
#30556=CARTESIAN_POINT('Ctrl Pts',(40.7333430448979,-29.2440888807198,-18.6161333950578));
#30557=CARTESIAN_POINT('Ctrl Pts',(40.9,-29.0996231131986,-18.5327260452907));
#30558=CARTESIAN_POINT('',(40.9,-30.5996231131986,-15.9346498339374));
#30559=CARTESIAN_POINT('Origin',(40.9,0.,0.));
#30560=CARTESIAN_POINT('',(40.4,-31.0330398077868,-16.1848830792292));
#30561=CARTESIAN_POINT('Ctrl Pts',(40.9,-30.5996231131986,-15.9346498339374));
#30562=CARTESIAN_POINT('Ctrl Pts',(40.7333430441722,-30.7440888813489,-16.0180571840677));
#30563=CARTESIAN_POINT('Ctrl Pts',(40.566659012132,-30.8885761378173,-16.1014769404842));
#30564=CARTESIAN_POINT('Ctrl Pts',(40.4,-31.0330398077868,-16.1848830792292));
#30565=CARTESIAN_POINT('Origin',(40.4,0.,0.));
#30566=CARTESIAN_POINT('Origin',(35.7,0.,0.));
#30567=CARTESIAN_POINT('',(30.5,-31.0562879796886,-16.1402285275843));
#30568=CARTESIAN_POINT('Ctrl Pts',(40.3999012894849,-31.0330346270951,-16.1848928782182));
#30569=CARTESIAN_POINT('Ctrl Pts',(39.2494626810401,-31.0330116996609,-16.1849362443212));
#30570=CARTESIAN_POINT('Ctrl Pts',(38.0976708836827,-31.0329190263647,-16.1851115327779));
#30571=CARTESIAN_POINT('Ctrl Pts',(36.9467340384722,-31.0328856894587,-16.1851746119074));
#30572=CARTESIAN_POINT('Ctrl Pts',(36.745427730736,-31.0328798586179,-16.1851856448556));
#30573=CARTESIAN_POINT('Ctrl Pts',(36.5441475779312,-31.0328758430124,-16.1851932450652));
#30574=CARTESIAN_POINT('Ctrl Pts',(36.3429119519248,-31.0328722727085,-16.1852000001162));
#30575=CARTESIAN_POINT('Ctrl Pts',(36.2102758775793,-31.0328699194915,-16.1852044524264));
#30576=CARTESIAN_POINT('Ctrl Pts',(36.0822774296292,-31.0328678560427,-16.1852084224022));
#30577=CARTESIAN_POINT('Ctrl Pts',(35.9587202262685,-31.0328657167444,-16.1852125810273));
#30578=CARTESIAN_POINT('Ctrl Pts',(35.7925662245339,-31.0328628399153,-16.1852181733537));
#30579=CARTESIAN_POINT('Ctrl Pts',(35.6344388155495,-31.0328598211428,-16.1852241162451));
#30580=CARTESIAN_POINT('Ctrl Pts',(35.4837714463462,-31.0328562161519,-16.1852312078525));
#30581=CARTESIAN_POINT('Ctrl Pts',(35.3175474553587,-31.0328522389406,-16.1852390316785));
#30582=CARTESIAN_POINT('Ctrl Pts',(35.1604041224823,-31.0328475520712,-16.1852482463283));
#30583=CARTESIAN_POINT('Ctrl Pts',(35.0116427948696,-31.0328419178902,-16.1852592402396));
#30584=CARTESIAN_POINT('Ctrl Pts',(34.9979272091156,-31.0328413984266,-16.1852602538628));
#30585=CARTESIAN_POINT('Ctrl Pts',(34.9842829110377,-31.0328408711131,-16.1852612822245));
#30586=CARTESIAN_POINT('Ctrl Pts',(34.9707093736271,-31.0328403358796,-16.1852623254083));
#30587=CARTESIAN_POINT('Ctrl Pts',(34.8522491799022,-31.0328356647415,-16.1852714295753));
#30588=CARTESIAN_POINT('Ctrl Pts',(34.7391835006528,-31.0328304196802,-16.1852816068676));
#30589=CARTESIAN_POINT('Ctrl Pts',(34.6312849042886,-31.0328252639046,-16.1852915612822));
#30590=CARTESIAN_POINT('Ctrl Pts',(34.509679526085,-31.0328194531707,-16.1853027802452));
#30591=CARTESIAN_POINT('Ctrl Pts',(34.3946370581325,-31.0328137541412,-16.1853137193613));
#30592=CARTESIAN_POINT('Ctrl Pts',(34.2857585821187,-31.0328086821745,-16.1853233495613));
#30593=CARTESIAN_POINT('Ctrl Pts',(34.178680190815,-31.0328036940624,-16.1853328205454));
#30594=CARTESIAN_POINT('Ctrl Pts',(34.0775620514826,-31.03279930319,-16.1853410431659));
#30595=CARTESIAN_POINT('Ctrl Pts',(33.9819758246426,-31.0327957057951,-16.1853475980774));
#30596=CARTESIAN_POINT('Ctrl Pts',(33.9184449689726,-31.0327933148066,-16.185351954763));
#30597=CARTESIAN_POINT('Ctrl Pts',(33.8573517602304,-31.0327912624253,-16.1853555977386));
#30598=CARTESIAN_POINT('Ctrl Pts',(33.7984399511825,-31.0327894081823,-16.1853587887284));
#30599=CARTESIAN_POINT('Ctrl Pts',(33.7337970612212,-31.0327873735542,-16.1853622901452));
#30600=CARTESIAN_POINT('Ctrl Pts',(33.671780974268,-31.0327855776264,-16.1853652470741));
#30601=CARTESIAN_POINT('Ctrl Pts',(33.6121191806453,-31.0327838881566,-16.1853678991827));
#30602=CARTESIAN_POINT('Ctrl Pts',(33.5695978710647,-31.0327826840616,-16.185369789356));
#30603=CARTESIAN_POINT('Ctrl Pts',(33.5282738752656,-31.0327815352148,-16.1853715223629));
#30604=CARTESIAN_POINT('Ctrl Pts',(33.4880643388297,-31.0327804070619,-16.1853731585247));
#30605=CARTESIAN_POINT('Ctrl Pts',(33.4508270573206,-31.0327793623012,-16.1853746737427));
#30606=CARTESIAN_POINT('Ctrl Pts',(33.4145509216557,-31.0327783314861,-16.1853761126591));
#30607=CARTESIAN_POINT('Ctrl Pts',(33.3793439789548,-31.0327771639656,-16.1853777420672));
#30608=CARTESIAN_POINT('Ctrl Pts',(33.3411337035362,-31.0327758968497,-16.1853795104722));
#30609=CARTESIAN_POINT('Ctrl Pts',(33.3041826660689,-31.032774468878,-16.1853815029501));
#30610=CARTESIAN_POINT('Ctrl Pts',(33.2685652776782,-31.0327727495065,-16.1853839484228));
#30611=CARTESIAN_POINT('Ctrl Pts',(33.2310094474552,-31.0327709365598,-16.185386526988));
#30612=CARTESIAN_POINT('Ctrl Pts',(33.1949357943683,-31.0327688002291,-16.1853896081159));
#30613=CARTESIAN_POINT('Ctrl Pts',(33.1603699172396,-31.0327662471214,-16.1853933524012));
#30614=CARTESIAN_POINT('Ctrl Pts',(33.1223715679422,-31.032763440484,-16.1853974685027));
#30615=CARTESIAN_POINT('Ctrl Pts',(33.0861949166479,-31.0327601306122,-16.1854023852332));
#30616=CARTESIAN_POINT('Ctrl Pts',(33.0518089354077,-31.0327562557941,-16.1854082033113));
#30617=CARTESIAN_POINT('Ctrl Pts',(33.0341030813061,-31.0327542605925,-16.1854111991264));
#30618=CARTESIAN_POINT('Ctrl Pts',(33.0168710360022,-31.0327521165229,-16.1854144322605));
#30619=CARTESIAN_POINT('Ctrl Pts',(33.0001033802534,-31.0327498200703,-16.1854179076006));
#30620=CARTESIAN_POINT('Ctrl Pts',(32.9420348133411,-31.0327418671572,-16.1854299431543));
#30621=CARTESIAN_POINT('Ctrl Pts',(32.8874145324496,-31.0328461364756,-16.1852296143113));
#30622=CARTESIAN_POINT('Ctrl Pts',(32.8357863520581,-31.0330149777622,-16.1849068811705));
#30623=CARTESIAN_POINT('Ctrl Pts',(32.7779739682631,-31.0332040434466,-16.1845454899291));
#30624=CARTESIAN_POINT('Ctrl Pts',(32.7239136589684,-31.0334742654592,-16.1840302574574));
#30625=CARTESIAN_POINT('Ctrl Pts',(32.6729278684753,-31.0337854095719,-16.1834371021678));
#30626=CARTESIAN_POINT('Ctrl Pts',(32.618080133626,-31.0341201214521,-16.1827990180322));
#30627=CARTESIAN_POINT('Ctrl Pts',(32.5667902508429,-31.0345025939174,-16.1820699950121));
#30628=CARTESIAN_POINT('Ctrl Pts',(32.5181731636795,-31.0349066963829,-16.1812992842338));
#30629=CARTESIAN_POINT('Ctrl Pts',(32.4659536029864,-31.0353407424037,-16.1804714646211));
#30630=CARTESIAN_POINT('Ctrl Pts',(32.4168175136244,-31.0358001425893,-16.1795947944395));
#30631=CARTESIAN_POINT('Ctrl Pts',(32.3696233879008,-31.0362725138778,-16.1786925325961));
#30632=CARTESIAN_POINT('Ctrl Pts',(32.3182581618429,-31.0367866341766,-16.1777105272545));
#30633=CARTESIAN_POINT('Ctrl Pts',(32.2691934412647,-31.0373164741887,-16.1766975364928));
#30634=CARTESIAN_POINT('Ctrl Pts',(32.2209064724826,-31.0378627004432,-16.1756521425246));
#30635=CARTESIAN_POINT('Ctrl Pts',(32.1715370438648,-31.0384211715745,-16.1745833137247));
#30636=CARTESIAN_POINT('Ctrl Pts',(32.1229805798606,-31.0389971805318,-16.173479840102));
#30637=CARTESIAN_POINT('Ctrl Pts',(32.0735591134784,-31.0396018563639,-16.1723205501866));
#30638=CARTESIAN_POINT('Ctrl Pts',(32.0254239419645,-31.0401907942691,-16.1711914331652));
#30639=CARTESIAN_POINT('Ctrl Pts',(31.9764682879415,-31.04080728099,-16.1700086968176));
#30640=CARTESIAN_POINT('Ctrl Pts',(31.9250947921527,-31.0414657598839,-16.1687449477338));
#30641=CARTESIAN_POINT('Ctrl Pts',(31.8952919104886,-31.0418477578043,-16.168011819419));
#30642=CARTESIAN_POINT('Ctrl Pts',(31.8646744620481,-31.0422439429541,-16.1672513233695));
#30643=CARTESIAN_POINT('Ctrl Pts',(31.8329224323944,-31.0426570718778,-16.1664582369103));
#30644=CARTESIAN_POINT('Ctrl Pts',(31.7319354368356,-31.0439710240641,-16.163935833788));
#30645=CARTESIAN_POINT('Ctrl Pts',(31.6284526822056,-31.0453389332578,-16.1613063818565));
#30646=CARTESIAN_POINT('Ctrl Pts',(31.5232336354318,-31.0466795487251,-16.1587277943726));
#30647=CARTESIAN_POINT('Ctrl Pts',(31.4188807866258,-31.0480091278027,-16.156170434673));
#30648=CARTESIAN_POINT('Ctrl Pts',(31.3128198672039,-31.0493111005242,-16.1536645426213));
#30649=CARTESIAN_POINT('Ctrl Pts',(31.205840297043,-31.0505011542276,-16.1513736799427));
#30650=CARTESIAN_POINT('Ctrl Pts',(31.1464339374067,-31.0511619977717,-16.1501015509562));
#30651=CARTESIAN_POINT('Ctrl Pts',(31.0867451889522,-31.0517883042759,-16.1488957763821));
#30652=CARTESIAN_POINT('Ctrl Pts',(31.0269161235858,-31.0523662912129,-16.1477831210733));
#30653=CARTESIAN_POINT('Ctrl Pts',(30.9223727403119,-31.0533762469847,-16.1458389029967));
#30654=CARTESIAN_POINT('Ctrl Pts',(30.8173993541569,-31.0542375463395,-16.1441811147896));
#30655=CARTESIAN_POINT('Ctrl Pts',(30.7129204018003,-31.0548748925162,-16.1429541726494));
#30656=CARTESIAN_POINT('Ctrl Pts',(30.6397146645873,-31.0553214647268,-16.1420944855846));
#30657=CARTESIAN_POINT('Ctrl Pts',(30.5667525557982,-31.0556583368408,-16.1414458510594));
#30658=CARTESIAN_POINT('Ctrl Pts',(30.4943593393941,-31.055866014916,-16.1410459118957));
#30659=CARTESIAN_POINT('',(30.5,-29.559989655385,-18.7405179110273));
#30660=CARTESIAN_POINT('Origin',(30.5,0.,0.));
#30661=CARTESIAN_POINT('Ctrl Pts',(30.5049791805003,-29.5605178050973,-18.7395177484758));
#30662=CARTESIAN_POINT('Ctrl Pts',(30.5973676827744,-29.560162264643,-18.7400797009803));
#30663=CARTESIAN_POINT('Ctrl Pts',(30.6891105694845,-29.559542510155,-18.7410567560113));
#30664=CARTESIAN_POINT('Ctrl Pts',(30.780677479308,-29.5587264396735,-18.7423441244048));
#30665=CARTESIAN_POINT('Ctrl Pts',(30.8441888930629,-29.5581604077948,-18.7432370516298));
#30666=CARTESIAN_POINT('Ctrl Pts',(30.9076166453417,-29.5574994222392,-18.7442800408076));
#30667=CARTESIAN_POINT('Ctrl Pts',(30.971128809674,-29.5567612578201,-18.7454455999911));
#30668=CARTESIAN_POINT('Ctrl Pts',(31.0735567068111,-29.5555707987955,-18.7473253308648));
#30669=CARTESIAN_POINT('Ctrl Pts',(31.1762019082914,-29.5541800414699,-18.7495231556641));
#30670=CARTESIAN_POINT('Ctrl Pts',(31.2798872709469,-29.5526737444515,-18.7519033574722));
#30671=CARTESIAN_POINT('Ctrl Pts',(31.3828989348284,-29.5511772346435,-18.7542680938472));
#30672=CARTESIAN_POINT('Ctrl Pts',(31.4869372222156,-29.5495656759358,-18.7568144117911));
#30673=CARTESIAN_POINT('Ctrl Pts',(31.5928574097494,-29.5479181178243,-18.7594156373086));
#30674=CARTESIAN_POINT('Ctrl Pts',(31.6516459294338,-29.5470036792766,-18.7608593866173));
#30675=CARTESIAN_POINT('Ctrl Pts',(31.7110150391233,-29.5460781618907,-18.7623200347852));
#30676=CARTESIAN_POINT('Ctrl Pts',(31.7711176725243,-29.5451562912556,-18.763774049131));
#30677=CARTESIAN_POINT('Ctrl Pts',(31.8409082760365,-29.5440858238842,-18.7654624366936));
#30678=CARTESIAN_POINT('Ctrl Pts',(31.9056373311747,-29.5431152615715,-18.7669933631241));
#30679=CARTESIAN_POINT('Ctrl Pts',(31.9658882086283,-29.5422441375119,-18.768367583494));
#30680=CARTESIAN_POINT('Ctrl Pts',(32.0341093482756,-29.5412577771694,-18.7699235920325));
#30681=CARTESIAN_POINT('Ctrl Pts',(32.0965888127923,-29.5403982847666,-18.7712796560443));
#30682=CARTESIAN_POINT('Ctrl Pts',(32.1542362617661,-29.5396480149485,-18.7724634074923));
#30683=CARTESIAN_POINT('Ctrl Pts',(32.2151538519835,-29.5388551849075,-18.773714309083));
#30684=CARTESIAN_POINT('Ctrl Pts',(32.2706761902198,-29.5381836213574,-18.7747738843965));
#30685=CARTESIAN_POINT('Ctrl Pts',(32.3219402247771,-29.5376060245818,-18.7756849339009));
#30686=CARTESIAN_POINT('Ctrl Pts',(32.3761674213258,-29.536995041577,-18.776648643858));
#30687=CARTESIAN_POINT('Ctrl Pts',(32.4256304058851,-29.5364887148648,-18.7774469218492));
#30688=CARTESIAN_POINT('Ctrl Pts',(32.4717350314077,-29.5360572749797,-18.7781265619113));
#30689=CARTESIAN_POINT('Ctrl Pts',(32.5214923281262,-29.5355916539681,-18.7788600469327));
#30690=CARTESIAN_POINT('Ctrl Pts',(32.5673384642532,-29.5352128774493,-18.7794559410667));
#30691=CARTESIAN_POINT('Ctrl Pts',(32.6111004962934,-29.5348934788928,-18.7799576530151));
#30692=CARTESIAN_POINT('Ctrl Pts',(32.6551147163181,-29.5345722397344,-18.780462256185));
#30693=CARTESIAN_POINT('Ctrl Pts',(32.6970214084871,-29.5343108907558,-18.7808718608789));
#30694=CARTESIAN_POINT('Ctrl Pts',(32.7387279964579,-29.5340950825232,-18.7812095285095));
#30695=CARTESIAN_POINT('Ctrl Pts',(32.7800761354879,-29.5338811290631,-18.781544294042));
#30696=CARTESIAN_POINT('Ctrl Pts',(32.8212277342351,-29.5337116838824,-18.7818087481603));
#30697=CARTESIAN_POINT('Ctrl Pts',(32.8640829337527,-29.5335890251804,-18.782000095504));
#30698=CARTESIAN_POINT('Ctrl Pts',(32.9037320332532,-29.5334755428695,-18.7821771276952));
#30699=CARTESIAN_POINT('Ctrl Pts',(32.9448394203921,-29.5334018918637,-18.7822919200911));
#30700=CARTESIAN_POINT('Ctrl Pts',(32.9889438598256,-29.5333868654406,-18.7823158450367));
#30701=CARTESIAN_POINT('Ctrl Pts',(32.992510226926,-29.5333856503761,-18.7823177796524));
#30702=CARTESIAN_POINT('Ctrl Pts',(32.9960962106242,-29.5333848297968,-18.7823191027633));
#30703=CARTESIAN_POINT('Ctrl Pts',(32.9997026353889,-29.5333844198653,-18.7823197895506));
#30704=CARTESIAN_POINT('Ctrl Pts',(33.0361388185046,-29.5333802782743,-18.7823267282529));
#30705=CARTESIAN_POINT('Ctrl Pts',(33.0740002606605,-29.5333765562528,-18.7823330770045));
#30706=CARTESIAN_POINT('Ctrl Pts',(33.1140504028668,-29.5333733966326,-18.7823389179975));
#30707=CARTESIAN_POINT('Ctrl Pts',(33.2460690464807,-29.5333629814689,-18.7823581718611));
#30708=CARTESIAN_POINT('Ctrl Pts',(33.3720922029406,-29.5333587011923,-18.7823661897829));
#30709=CARTESIAN_POINT('Ctrl Pts',(33.4992849360726,-29.5333546566756,-18.782373736073));
#30710=CARTESIAN_POINT('Ctrl Pts',(33.6626792864138,-29.5333494610079,-18.7823834301894));
#30711=CARTESIAN_POINT('Ctrl Pts',(33.8280037294637,-29.5333446544026,-18.7823923459959));
#30712=CARTESIAN_POINT('Ctrl Pts',(33.9928746198634,-29.5333373313072,-18.7824059536077));
#30713=CARTESIAN_POINT('Ctrl Pts',(34.322616400663,-29.5333226851165,-18.7824331688313));
#30714=CARTESIAN_POINT('Ctrl Pts',(34.6505439708621,-29.5332979729652,-18.7824791512758));
#30715=CARTESIAN_POINT('Ctrl Pts',(34.979144925286,-29.5332814027048,-18.7825099763789));
#30716=CARTESIAN_POINT('Ctrl Pts',(35.30774587971,-29.5332648324445,-18.782540801482));
#30717=CARTESIAN_POINT('Ctrl Pts',(35.6370202183589,-29.5332564040751,-18.7825564692435));
#30718=CARTESIAN_POINT('Ctrl Pts',(35.9661418060973,-29.5332492722834,-18.7825697306317));
#30719=CARTESIAN_POINT('Ctrl Pts',(36.2952633938358,-29.5332421404917,-18.7825829920199));
#30720=CARTESIAN_POINT('Ctrl Pts',(36.6242322306637,-29.5332363052777,-18.7825938470347));
#30721=CARTESIAN_POINT('Ctrl Pts',(36.9531363303404,-29.5332247108411,-18.7826154119861));
#30722=CARTESIAN_POINT('Ctrl Pts',(38.1022190076918,-29.5331842036954,-18.7826907528288));
#30723=CARTESIAN_POINT('Ctrl Pts',(39.2505115204485,-29.5330734009978,-18.782896816333));
#30724=CARTESIAN_POINT('Ctrl Pts',(40.400093943525,-29.533045998731,-18.7829477771169));
#30725=CARTESIAN_POINT('Ctrl Pts',(6.89999999997365,-5.3678954269134,-9.63452070648359));
#30726=CARTESIAN_POINT('Ctrl Pts',(6.99168932310453,-5.42175501956,-9.60499723839754));
#30727=CARTESIAN_POINT('Ctrl Pts',(7.08383915760479,-5.47527828673705,-9.57508016834563));
#30728=CARTESIAN_POINT('Ctrl Pts',(8.15762752947026,-6.09209251732962,-9.22342495405909));
#30729=CARTESIAN_POINT('Ctrl Pts',(9.16608342448598,-6.61836595106258,-8.84591675027098));
#30730=CARTESIAN_POINT('Ctrl Pts',(11.2535425311854,-7.53037930120419,-8.09542754093137));
#30731=CARTESIAN_POINT('Ctrl Pts',(12.2577133097063,-7.91666449612081,-7.7072500137176));
#30732=CARTESIAN_POINT('Ctrl Pts',(14.356433377742,-8.58141250110813,-6.97440810645327));
#30733=CARTESIAN_POINT('Ctrl Pts',(15.3659105035251,-8.8532231228606,-6.61345583116597));
#30734=CARTESIAN_POINT('Ctrl Pts',(17.4728641219044,-9.31281879192961,-5.96623757129007));
#30735=CARTESIAN_POINT('Ctrl Pts',(18.4890996814195,-9.49384943617776,-5.66020885204394));
#30736=CARTESIAN_POINT('Ctrl Pts',(19.8476172011441,-9.68599953593306,-5.32865724601648));
#30737=CARTESIAN_POINT('Ctrl Pts',(20.3454889307686,-9.75195458239816,-5.20930542916259));
#30738=CARTESIAN_POINT('Ctrl Pts',(21.3782040612024,-9.87366876552717,-4.97678151322346));
#30739=CARTESIAN_POINT('Ctrl Pts',(22.1792648896895,-9.95072592994711,-4.81935607344485));
#30740=CARTESIAN_POINT('Ctrl Pts',(22.8542621828908,-10.0067883222623,-4.70591921690553));
#30741=CARTESIAN_POINT('Ctrl Pts',(23.1054579010966,-10.0267605301623,-4.66456206383026));
#30742=CARTESIAN_POINT('Ctrl Pts',(23.6171513959784,-10.0644076466806,-4.58448144656257));
#30743=CARTESIAN_POINT('Ctrl Pts',(24.1360713221936,-10.0979855598765,-4.51012725444833));
#30744=CARTESIAN_POINT('Ctrl Pts',(24.6624927871863,-10.1277002159265,-4.44285620865164));
#30745=CARTESIAN_POINT('Ctrl Pts',(25.1928168818087,-10.1547862564439,-4.38095271718119));
#30746=CARTESIAN_POINT('Ctrl Pts',(25.5948982287614,-10.1721457030178,-4.34117176259642));
#30747=CARTESIAN_POINT('Ctrl Pts',(26.123203188965,-10.1922876384417,-4.29604941535506));
#30748=CARTESIAN_POINT('Ctrl Pts',(27.1768897027567,-10.2241871753182,-4.22326129112039));
#30749=CARTESIAN_POINT('Ctrl Pts',(28.2111297865347,-10.2325109692973,-4.19969555688312));
#30750=CARTESIAN_POINT('Ctrl Pts',(29.1277555719712,-10.2421056253617,-4.17661492679513));
#30751=CARTESIAN_POINT('Ctrl Pts',(29.4767605677586,-10.2448788784735,-4.17005614900019));
#30752=CARTESIAN_POINT('Ctrl Pts',(30.1601418995912,-10.2473221772452,-4.16421367130871));
#30753=CARTESIAN_POINT('Ctrl Pts',(31.3500242312262,-10.2457563290907,-4.16794387579263));
#30754=CARTESIAN_POINT('Ctrl Pts',(32.3461596131127,-10.2405791191156,-4.18040640609125));
#30755=CARTESIAN_POINT('Ctrl Pts',(33.1614718826737,-10.2405840900447,-4.18039330945983));
#30756=CARTESIAN_POINT('Ctrl Pts',(33.4925794155278,-10.2405841444578,-4.18039253080267));
#30757=CARTESIAN_POINT('Ctrl Pts',(34.1499904318885,-10.2405848392549,-4.18039030822713));
#30758=CARTESIAN_POINT('Ctrl Pts',(34.9738731541178,-10.2405865289643,-4.18038393925504));
#30759=CARTESIAN_POINT('Ctrl Pts',(35.9612754428241,-10.2405873001735,-4.18038119412747));
#30760=CARTESIAN_POINT('Ctrl Pts',(37.9366467881619,-10.2405882857914,-4.18037753677863));
#30761=CARTESIAN_POINT('Ctrl Pts',(39.5833333333333,-10.2405934798255,-4.18035859466987));
#30762=CARTESIAN_POINT('Ctrl Pts',(40.9,-10.2405934798255,-4.18035859466987));
#30763=CARTESIAN_POINT('Ctrl Pts',(6.71972576838711,-6.5764381714634,-12.8464244365415));
#30764=CARTESIAN_POINT('Ctrl Pts',(6.81144220747046,-6.6482837686261,-12.8102053989753));
#30765=CARTESIAN_POINT('Ctrl Pts',(6.90362823998598,-6.71971524922859,-12.7734498343709));
#30766=CARTESIAN_POINT('Ctrl Pts',(7.97787811486329,-7.54294881554194,-12.3410744046091));
#30767=CARTESIAN_POINT('Ctrl Pts',(8.98681832185142,-8.24809748747637,-11.871220138602));
#30768=CARTESIAN_POINT('Ctrl Pts',(11.0806583453373,-9.47774891389534,-10.9274240314556));
#30769=CARTESIAN_POINT('Ctrl Pts',(12.0862475175457,-10.0005505115845,-10.4368998098017));
#30770=CARTESIAN_POINT('Ctrl Pts',(14.197639322261,-10.906656993414,-9.50280276487817));
#30771=CARTESIAN_POINT('Ctrl Pts',(15.2100862637121,-11.2785931828498,-9.04203633254719));
#30772=CARTESIAN_POINT('Ctrl Pts',(17.3364698493953,-11.9121957711897,-8.20932952666152));
#30773=CARTESIAN_POINT('Ctrl Pts',(18.357279581038,-12.1627870018009,-7.81594677169137));
#30774=CARTESIAN_POINT('Ctrl Pts',(19.7331217809844,-12.4307568384137,-7.38628119283514));
#30775=CARTESIAN_POINT('Ctrl Pts',(20.2341927100357,-12.5225360922773,-7.23233618870703));
#30776=CARTESIAN_POINT('Ctrl Pts',(21.2777139275315,-12.6928916013278,-6.93114017240203));
#30777=CARTESIAN_POINT('Ctrl Pts',(22.0885637816417,-12.8012350092453,-6.72673758680645));
#30778=CARTESIAN_POINT('Ctrl Pts',(22.7734874647763,-12.8801738355232,-6.57909772915769));
#30779=CARTESIAN_POINT('Ctrl Pts',(23.0269571312138,-12.9082278965573,-6.52549682636865));
#30780=CARTESIAN_POINT('Ctrl Pts',(23.5444618566096,-12.9612738268022,-6.421485113254));
#30781=CARTESIAN_POINT('Ctrl Pts',(24.069438315646,-13.0087020921734,-6.32485290039691));
#30782=CARTESIAN_POINT('Ctrl Pts',(24.6027295908464,-13.0507741241225,-6.23730008137708));
#30783=CARTESIAN_POINT('Ctrl Pts',(25.140319252314,-13.0891677302171,-6.15667530541497));
#30784=CARTESIAN_POINT('Ctrl Pts',(25.5484689870705,-13.1137995888261,-6.1047965908769));
#30785=CARTESIAN_POINT('Ctrl Pts',(26.0852808149066,-13.1423647911197,-6.04589855121053));
#30786=CARTESIAN_POINT('Ctrl Pts',(27.1586857291268,-13.1877077660313,-5.95074158602806));
#30787=CARTESIAN_POINT('Ctrl Pts',(28.1995312980844,-13.1995114624862,-5.92039197700572));
#30788=CARTESIAN_POINT('Ctrl Pts',(29.1157533315887,-13.2130297822556,-5.89061060808304));
#30789=CARTESIAN_POINT('Ctrl Pts',(29.4698938670485,-13.2169740538761,-5.88204921070821));
#30790=CARTESIAN_POINT('Ctrl Pts',(30.1587234046997,-13.220429005539,-5.87447683559578));
#30791=CARTESIAN_POINT('Ctrl Pts',(31.3557311956059,-13.2182120926508,-5.87931523414857));
#30792=CARTESIAN_POINT('Ctrl Pts',(32.3501802435609,-13.2109234983781,-5.89537176970749));
#30793=CARTESIAN_POINT('Ctrl Pts',(33.1605031382465,-13.2109314016451,-5.89535013085606));
#30794=CARTESIAN_POINT('Ctrl Pts',(33.4922179295251,-13.2109314596682,-5.89534881762642));
#30795=CARTESIAN_POINT('Ctrl Pts',(34.1493400019897,-13.2109325467446,-5.89534512891166));
#30796=CARTESIAN_POINT('Ctrl Pts',(34.9735241318651,-13.2109351472382,-5.89533452524068));
#30797=CARTESIAN_POINT('Ctrl Pts',(35.9608954520826,-13.2109363413972,-5.8953299596426));
#30798=CARTESIAN_POINT('Ctrl Pts',(37.9363824842975,-13.2109378608691,-5.89532387223529));
#30799=CARTESIAN_POINT('Ctrl Pts',(39.5833333333333,-13.2109458830841,-5.89529235427929));
#30800=CARTESIAN_POINT('Ctrl Pts',(40.9,-13.2109458830841,-5.89529235427929));
#30801=CARTESIAN_POINT('Ctrl Pts',(6.48177011792014,-9.40621265917915,-20.336764848396));
#30802=CARTESIAN_POINT('Ctrl Pts',(6.57271435585529,-9.51911083717172,-20.2851799357091));
#30803=CARTESIAN_POINT('Ctrl Pts',(6.66411141569866,-9.63139437446865,-20.2327517601295));
#30804=CARTESIAN_POINT('Ctrl Pts',(7.73048017258431,-10.9276768808967,-19.614616528956));
#30805=CARTESIAN_POINT('Ctrl Pts',(8.73292722985417,-12.0456324995183,-18.9319609573801));
#30806=CARTESIAN_POINT('Ctrl Pts',(10.8102906905198,-14.0013807284478,-17.5485371602851));
#30807=CARTESIAN_POINT('Ctrl Pts',(11.8125687231201,-14.8418955382559,-16.8218444562665));
#30808=CARTESIAN_POINT('Ctrl Pts',(13.9177445864075,-16.3050153868123,-15.4271303717406));
#30809=CARTESIAN_POINT('Ctrl Pts',(14.9296562678442,-16.9116612373854,-14.7350649820735));
#30810=CARTESIAN_POINT('Ctrl Pts',(17.0680844879216,-17.9535844659564,-13.4708635112562));
#30811=CARTESIAN_POINT('Ctrl Pts',(18.0932339179161,-18.3688941094638,-12.8729609429));
#30812=CARTESIAN_POINT('Ctrl Pts',(19.4933464326808,-18.8183285494773,-12.2099892645604));
#30813=CARTESIAN_POINT('Ctrl Pts',(19.9993272808496,-18.971430097181,-11.9744841299437));
#30814=CARTESIAN_POINT('Ctrl Pts',(21.0600020168761,-19.2581324129063,-11.5100300116438));
#30815=CARTESIAN_POINT('Ctrl Pts',(21.8888875769482,-19.4420158954032,-11.1928649299996));
#30816=CARTESIAN_POINT('Ctrl Pts',(22.5933490549502,-19.5764520117207,-10.9625055113849));
#30817=CARTESIAN_POINT('Ctrl Pts',(22.8513437851798,-19.6238525927721,-10.8796937171905));
#30818=CARTESIAN_POINT('Ctrl Pts',(23.3805933886565,-19.7139851739533,-10.7182299385361));
#30819=CARTESIAN_POINT('Ctrl Pts',(23.9182257576784,-19.7948254980796,-10.5680285062335));
#30820=CARTESIAN_POINT('Ctrl Pts',(24.4662138806867,-19.8668205194741,-10.4315004891655));
#30821=CARTESIAN_POINT('Ctrl Pts',(25.0195744741821,-19.9326328666884,-10.3055778221167));
#30822=CARTESIAN_POINT('Ctrl Pts',(25.4412458088222,-19.9749776253081,-10.2242864909386));
#30823=CARTESIAN_POINT('Ctrl Pts',(25.9971983460992,-20.0240850656221,-10.1317971075869));
#30824=CARTESIAN_POINT('Ctrl Pts',(27.1157050405651,-20.102368552767,-9.98182332250459));
#30825=CARTESIAN_POINT('Ctrl Pts',(28.1723100127449,-20.1222437541334,-9.93573708068021));
#30826=CARTESIAN_POINT('Ctrl Pts',(29.0876106506765,-20.1449463132816,-9.89029022572782));
#30827=CARTESIAN_POINT('Ctrl Pts',(29.4537207931442,-20.1517438988728,-9.87684873205161));
#30828=CARTESIAN_POINT('Ctrl Pts',(30.1552759232945,-20.1576060163182,-9.86516345924734));
#30829=CARTESIAN_POINT('Ctrl Pts',(31.3689241276359,-20.1538463873916,-9.87263514017789));
#30830=CARTESIAN_POINT('Ctrl Pts',(32.359478715431,-20.1416711708076,-9.8970230216562));
#30831=CARTESIAN_POINT('Ctrl Pts',(33.1581760188913,-20.1416983285704,-9.89696607979063));
#30832=CARTESIAN_POINT('Ctrl Pts',(33.4913102145728,-20.141699805843,-9.89696201382191));
#30833=CARTESIAN_POINT('Ctrl Pts',(34.1477617736106,-20.1417043298969,-9.8969519305241));
#30834=CARTESIAN_POINT('Ctrl Pts',(34.9726616332632,-20.1417171222834,-9.8969221857378));
#30835=CARTESIAN_POINT('Ctrl Pts',(35.9599657908141,-20.1417226604566,-9.8969094863839));
#30836=CARTESIAN_POINT('Ctrl Pts',(37.9357298104642,-20.1417300151411,-9.89689244880614));
#30837=CARTESIAN_POINT('Ctrl Pts',(39.5833333333333,-20.1417681573542,-9.8968044600346));
#30838=CARTESIAN_POINT('Ctrl Pts',(40.9,-20.1417681573542,-9.8968044600346));
#30839=CARTESIAN_POINT('Ctrl Pts',(6.40644620858992,-12.3446157076951,-27.7818319413302));
#30840=CARTESIAN_POINT('Ctrl Pts',(6.49686818484384,-12.4976194141968,-27.7146057723315));
#30841=CARTESIAN_POINT('Ctrl Pts',(6.58771883172007,-12.6497754970257,-27.6462615383487));
#30842=CARTESIAN_POINT('Ctrl Pts',(7.64885870107047,-14.4089312086777,-26.838967465877));
#30843=CARTESIAN_POINT('Ctrl Pts',(8.64786699401838,-15.9309901815184,-25.9406999974137));
#30844=CARTESIAN_POINT('Ctrl Pts',(10.7071344443812,-18.5841088194585,-24.1258468463739));
#30845=CARTESIAN_POINT('Ctrl Pts',(11.7059636153276,-19.7351568023896,-23.1640388241121));
#30846=CARTESIAN_POINT('Ctrl Pts',(13.7894167134297,-21.7274097031724,-21.32755345859));
#30847=CARTESIAN_POINT('Ctrl Pts',(14.7964804448639,-22.5625068415353,-20.4089660621499));
#30848=CARTESIAN_POINT('Ctrl Pts',(16.9150096963281,-23.9923642448818,-18.7347867871849));
#30849=CARTESIAN_POINT('Ctrl Pts',(17.9356563974909,-24.568778311437,-17.9376031564435));
#30850=CARTESIAN_POINT('Ctrl Pts',(19.3316378726113,-25.1942531765858,-17.0495061236354));
#30851=CARTESIAN_POINT('Ctrl Pts',(19.8373783148987,-25.4080883980548,-16.733671277521));
#30852=CARTESIAN_POINT('Ctrl Pts',(20.898614645132,-25.8097110946141,-16.1088561234904));
#30853=CARTESIAN_POINT('Ctrl Pts',(21.7322089233614,-26.069558105635,-15.6790344990821));
#30854=CARTESIAN_POINT('Ctrl Pts',(22.4452152218926,-26.2607608176431,-15.3644450466694));
#30855=CARTESIAN_POINT('Ctrl Pts',(22.7053175952386,-26.327863353572,-15.2520352575854));
#30856=CARTESIAN_POINT('Ctrl Pts',(23.2405350109147,-26.4560495577168,-15.0319031635371));
#30857=CARTESIAN_POINT('Ctrl Pts',(23.7856351879594,-26.5714803865858,-14.8265027181048));
#30858=CARTESIAN_POINT('Ctrl Pts',(24.3434088150881,-26.6748081507041,-14.6389049166986));
#30859=CARTESIAN_POINT('Ctrl Pts',(24.9080926446007,-26.7695587595052,-14.4653482504621));
#30860=CARTESIAN_POINT('Ctrl Pts',(25.3404979553363,-26.8308622015487,-14.3526452692475));
#30861=CARTESIAN_POINT('Ctrl Pts',(25.9125607075503,-26.9021372597286,-14.2239063651395));
#30862=CARTESIAN_POINT('Ctrl Pts',(27.0720378258712,-27.0165941086124,-14.0136986134134));
#30863=CARTESIAN_POINT('Ctrl Pts',(28.1454151442858,-27.0445191043407,-13.9518646781024));
#30864=CARTESIAN_POINT('Ctrl Pts',(29.0596751952943,-27.0764264216484,-13.890725520751));
#30865=CARTESIAN_POINT('Ctrl Pts',(29.4376599373187,-27.0863532011148,-13.8719255145711));
#30866=CARTESIAN_POINT('Ctrl Pts',(30.1519376760717,-27.0947220176403,-13.855954576287));
#30867=CARTESIAN_POINT('Ctrl Pts',(31.3821999577688,-27.0893514143296,-13.8661782937676));
#30868=CARTESIAN_POINT('Ctrl Pts',(32.3688386893656,-27.0723527225426,-13.898788121758));
#30869=CARTESIAN_POINT('Ctrl Pts',(33.1558986739573,-27.0724155351931,-13.8986675947835));
#30870=CARTESIAN_POINT('Ctrl Pts',(33.4904503866599,-27.0724198047059,-13.8986584195583));
#30871=CARTESIAN_POINT('Ctrl Pts',(34.1462287076183,-27.0724307945235,-13.8986367255002));
#30872=CARTESIAN_POINT('Ctrl Pts',(34.9718350023127,-27.0724629552155,-13.898572048806));
#30873=CARTESIAN_POINT('Ctrl Pts',(35.9590682028414,-27.07247672176,-13.8985445297567));
#30874=CARTESIAN_POINT('Ctrl Pts',(37.9351039480424,-27.0724951558979,-13.8985075170898));
#30875=CARTESIAN_POINT('Ctrl Pts',(39.5833333333333,-27.0725904316243,-13.8983165657899));
#30876=CARTESIAN_POINT('Ctrl Pts',(40.9,-27.0725904316243,-13.8983165657899));
#30877=CARTESIAN_POINT('Ctrl Pts',(6.37427268165564,-14.0406695266741,-32.0290848932163));
#30878=CARTESIAN_POINT('Ctrl Pts',(6.46448755772839,-14.2166050753401,-31.9528098065586));
#30879=CARTESIAN_POINT('Ctrl Pts',(6.55512327887566,-14.3915605358513,-31.8752581000468));
#30880=CARTESIAN_POINT('Ctrl Pts',(7.61410360785655,-16.4151695040825,-30.958672886913));
#30881=CARTESIAN_POINT('Ctrl Pts',(8.61142775869687,-18.1677152487792,-29.9361952854453));
#30882=CARTESIAN_POINT('Ctrl Pts',(10.6634825022472,-21.2183968262284,-27.8730682250753));
#30883=CARTESIAN_POINT('Ctrl Pts',(11.6607542873627,-22.5462154536683,-26.7761583709751));
#30884=CARTESIAN_POINT('Ctrl Pts',(13.7353039743977,-24.8383185913233,-24.6873364683673));
#30885=CARTESIAN_POINT('Ctrl Pts',(14.7402095633116,-25.8029859119439,-23.6392130729629));
#30886=CARTESIAN_POINT('Ctrl Pts',(16.8490881066137,-27.4503074906309,-21.733995182915));
#30887=CARTESIAN_POINT('Ctrl Pts',(17.8672038783314,-28.117536242687,-20.8239061433235));
#30888=CARTESIAN_POINT('Ctrl Pts',(19.2585933984996,-28.8404836901117,-19.811022849419));
#30889=CARTESIAN_POINT('Ctrl Pts',(19.7636418533907,-29.0884650342025,-19.4499572035579));
#30890=CARTESIAN_POINT('Ctrl Pts',(20.8231816497994,-29.5540603372583,-18.7357747989967));
#30891=CARTESIAN_POINT('Ctrl Pts',(21.6568670511734,-29.8562628482712,-18.2431916560479));
#30892=CARTESIAN_POINT('Ctrl Pts',(22.3720072062876,-30.079259337671,-17.8815051531587));
#30893=CARTESIAN_POINT('Ctrl Pts',(22.6326824787812,-30.1574913312726,-17.7523977438431));
#30894=CARTESIAN_POINT('Ctrl Pts',(23.1697036949936,-30.3071564102285,-17.4991937768335));
#30895=CARTESIAN_POINT('Ctrl Pts',(23.7174377716561,-30.4422233412818,-17.2625030946595));
#30896=CARTESIAN_POINT('Ctrl Pts',(24.2790946262572,-30.5634410393028,-17.0457855087881));
#30897=CARTESIAN_POINT('Ctrl Pts',(24.8485847331463,-30.6748008187178,-16.8449230908939));
#30898=CARTESIAN_POINT('Ctrl Pts',(25.2859632686136,-30.7471152582868,-16.7140007344129));
#30899=CARTESIAN_POINT('Ctrl Pts',(25.8659001690754,-30.8313513860032,-16.5640760155963));
#30900=CARTESIAN_POINT('Ctrl Pts',(27.0467877055031,-30.9672841404843,-16.3181083484214));
#30901=CARTESIAN_POINT('Ctrl Pts',(28.1301993946288,-30.9999203594232,-16.2470842981322));
#30902=CARTESIAN_POINT('Ctrl Pts',(29.0438132065911,-31.0370949113971,-16.1769735529555));
#30903=CARTESIAN_POINT('Ctrl Pts',(29.4285323170642,-31.0489002942268,-16.1549555741443));
#30904=CARTESIAN_POINT('Ctrl Pts',(30.1500796604944,-31.0587367393327,-16.1364761766635));
#30905=CARTESIAN_POINT('Ctrl Pts',(31.3898224001987,-31.0524272220083,-16.1483068856791));
#30906=CARTESIAN_POINT('Ctrl Pts',(32.3742147772172,-31.032701705164,-16.1855693458549));
#30907=CARTESIAN_POINT('Ctrl Pts',(33.1546196294425,-31.0327939306213,-16.1853991323254));
#30908=CARTESIAN_POINT('Ctrl Pts',(33.4899805045661,-31.0328008093451,-16.1853856345319));
#30909=CARTESIAN_POINT('Ctrl Pts',(34.1453728987308,-31.0328173216773,-16.1853546639145));
#30910=CARTESIAN_POINT('Ctrl Pts',(34.9713787068035,-31.0328663827335,-16.1852616946182));
#30911=CARTESIAN_POINT('Ctrl Pts',(35.9585696612046,-31.0328872804502,-16.1852222245756));
#30912=CARTESIAN_POINT('Ctrl Pts',(37.9347583211501,-31.0329153648958,-16.1851690519236));
#30913=CARTESIAN_POINT('Ctrl Pts',(39.5833333333333,-31.0330603026358,-16.1848949119358));
#30914=CARTESIAN_POINT('Ctrl Pts',(40.9,-31.0330603026358,-16.1848949119358));
#30915=CARTESIAN_POINT('',(40.9,-29.2992994660114,-15.1839076262003));
#30916=CARTESIAN_POINT('Ctrl Pts',(40.9,-29.2992994660114,-15.1839076262003));
#30917=CARTESIAN_POINT('Ctrl Pts',(40.9,-29.7327406817405,-15.4341550287793));
#30918=CARTESIAN_POINT('Ctrl Pts',(40.9,-30.1661818974696,-15.6844024313584));
#30919=CARTESIAN_POINT('Ctrl Pts',(40.9,-30.5996231131986,-15.9346498339374));
#30920=CARTESIAN_POINT('',(38.,-29.2992994660114,-15.1839076262003));
#30921=CARTESIAN_POINT('Ctrl Pts',(38.,-29.2992994660114,-15.1839076262003));
#30922=CARTESIAN_POINT('Ctrl Pts',(38.9666666666667,-29.2992994660114,-15.1839076262003));
#30923=CARTESIAN_POINT('Ctrl Pts',(39.9333333333333,-29.2992994660114,-15.1839076262003));
#30924=CARTESIAN_POINT('Ctrl Pts',(40.9,-29.2992994660114,-15.1839076262003));
#30925=CARTESIAN_POINT('Ctrl Pts',(37.4974382384971,-28.7790269720418,-14.8838038109906));
#30926=CARTESIAN_POINT('Ctrl Pts',(37.6645213547145,-28.9527098777879,-14.9840691120819));
#30927=CARTESIAN_POINT('Ctrl Pts',(37.8313739960415,-29.1261374112004,-15.084184715056));
#30928=CARTESIAN_POINT('Ctrl Pts',(37.9978889629902,-29.2992044501374,-15.1840905833949));
#30929=CARTESIAN_POINT('',(6.9,-12.9951291628659,-27.0393531365015));
#30930=CARTESIAN_POINT('Ctrl Pts',(6.9,-12.9951291628659,-27.0393531365015));
#30931=CARTESIAN_POINT('Ctrl Pts',(6.9,-11.9174419758914,-24.649274247254));
#30932=CARTESIAN_POINT('Ctrl Pts',(6.90000000000115,-10.8339866674746,-22.230729924082));
#30933=CARTESIAN_POINT('Ctrl Pts',(6.90000000000115,-8.41000082059024,-16.7584145047598));
#30934=CARTESIAN_POINT('Ctrl Pts',(6.9,-6.82522008706163,-13.1312177506378));
#30935=CARTESIAN_POINT('Ctrl Pts',(6.9,-5.36789542693312,-9.63452070648529));
#30936=CARTESIAN_POINT('',(22.9245129145126,-27.5141512254857,-15.8853026165582));
#30937=CARTESIAN_POINT('Ctrl Pts',(22.9245129145126,-27.5141512254857,-15.8853026165582));
#30938=CARTESIAN_POINT('Ctrl Pts',(22.7202811020963,-27.405303612937,-15.9355315703924));
#30939=CARTESIAN_POINT('Ctrl Pts',(22.5089075447093,-27.2924652433825,-15.9922246435191));
#30940=CARTESIAN_POINT('Ctrl Pts',(22.2913349439917,-27.1762359097413,-16.0558281873747));
#30941=CARTESIAN_POINT('Ctrl Pts',(21.4451770585291,-26.7242103933931,-16.3031876434795));
#30942=CARTESIAN_POINT('Ctrl Pts',(20.5220951556666,-26.2108400614941,-16.6965145338606));
#30943=CARTESIAN_POINT('Ctrl Pts',(19.7671428819536,-25.7770859372677,-17.0753616782145));
#30944=CARTESIAN_POINT('Ctrl Pts',(19.519477305839,-25.6347908958338,-17.1996442316061));
#30945=CARTESIAN_POINT('Ctrl Pts',(19.286571638609,-25.4994131575072,-17.3225345039427));
#30946=CARTESIAN_POINT('Ctrl Pts',(19.0728538401323,-25.3740784559106,-17.4387046858284));
#30947=CARTESIAN_POINT('Ctrl Pts',(18.7028555998035,-25.15709316328,-17.6398239336529));
#30948=CARTESIAN_POINT('Ctrl Pts',(18.4144703596235,-24.9815167506411,-17.8106758656205));
#30949=CARTESIAN_POINT('Ctrl Pts',(18.0642874871537,-24.7606238748751,-18.0298340093775));
#30950=CARTESIAN_POINT('Ctrl Pts',(17.442092711672,-24.3681478172274,-18.4192278454841));
#30951=CARTESIAN_POINT('Ctrl Pts',(16.7224564418218,-23.8866996305775,-18.9163953124275));
#30952=CARTESIAN_POINT('Ctrl Pts',(15.9202806616111,-23.2999769887242,-19.5075155171573));
#30953=CARTESIAN_POINT('Ctrl Pts',(15.4090529834512,-22.9260578785765,-19.8842371999013));
#30954=CARTESIAN_POINT('Ctrl Pts',(14.8739602945702,-22.5035099772286,-20.3065653819892));
#30955=CARTESIAN_POINT('Ctrl Pts',(14.3169794331135,-22.0244589523024,-20.7640450546201));
#30956=CARTESIAN_POINT('Ctrl Pts',(13.8864206762823,-21.6541417151688,-21.1176871503438));
#30957=CARTESIAN_POINT('Ctrl Pts',(13.3867890027795,-21.2019814327435,-21.5394320189433));
#30958=CARTESIAN_POINT('Ctrl Pts',(12.8146824059514,-20.6456427149589,-22.0238946695559));
#30959=CARTESIAN_POINT('Ctrl Pts',(12.2526665517595,-20.0991166279862,-22.499812430193));
#30960=CARTESIAN_POINT('Ctrl Pts',(11.6379478462803,-19.44703563439,-23.0419154065947));
#30961=CARTESIAN_POINT('Ctrl Pts',(10.9739250490308,-18.6689137476991,-23.626535453056));
#30962=CARTESIAN_POINT('Ctrl Pts',(10.5683455447963,-18.1936434853748,-23.9836164291783));
#30963=CARTESIAN_POINT('Ctrl Pts',(10.1437415406956,-17.6694303965612,-24.3558958755273));
#30964=CARTESIAN_POINT('Ctrl Pts',(9.74137929176525,-17.1528053766524,-24.6998029803349));
#30965=CARTESIAN_POINT('Ctrl Pts',(8.72285779294234,-15.8450442956717,-25.5703537856744));
#30966=CARTESIAN_POINT('Ctrl Pts',(7.81323138778195,-14.4751178145146,-26.3485431508901));
#30967=CARTESIAN_POINT('Ctrl Pts',(6.9,-12.9951291628659,-27.0393531365015));
#30968=CARTESIAN_POINT('Ctrl Pts',(30.5,-31.0562879796886,-16.1402285275843));
#30969=CARTESIAN_POINT('Ctrl Pts',(29.9560179420817,-30.8470467059701,-16.0158030554221));
#30970=CARTESIAN_POINT('Ctrl Pts',(29.4152668325132,-30.6299015220344,-15.9055856438303));
#30971=CARTESIAN_POINT('Ctrl Pts',(28.8740459957565,-30.3967092920472,-15.8236145009996));
#30972=CARTESIAN_POINT('Ctrl Pts',(28.353527792344,-30.1724370682909,-15.7447788961961));
#30973=CARTESIAN_POINT('Ctrl Pts',(27.8179515912467,-29.9423746730404,-15.6599939665101));
#30974=CARTESIAN_POINT('Ctrl Pts',(27.2695051149491,-29.6962958928787,-15.5981844167478));
#30975=CARTESIAN_POINT('Ctrl Pts',(26.9554553615883,-29.5553870101399,-15.5627912203338));
#30976=CARTESIAN_POINT('Ctrl Pts',(26.6378099296971,-29.4095747645068,-15.5350208970661));
#30977=CARTESIAN_POINT('Ctrl Pts',(26.3179304017917,-29.2578762499931,-15.520523503095));
#30978=CARTESIAN_POINT('Ctrl Pts',(26.1078196745982,-29.1582340959379,-15.5110009868852));
#30979=CARTESIAN_POINT('Ctrl Pts',(25.8967402232745,-29.0560612282453,-15.5072071790431));
#30980=CARTESIAN_POINT('Ctrl Pts',(25.6850706236774,-28.9510881944939,-15.5107635234098));
#30981=CARTESIAN_POINT('Ctrl Pts',(25.6562210027417,-28.9367808388889,-15.5112482372614));
#30982=CARTESIAN_POINT('Ctrl Pts',(25.6277737638215,-28.9226278510966,-15.5118582602787));
#30983=CARTESIAN_POINT('Ctrl Pts',(25.5983858063598,-28.9079571471847,-15.5126342200129));
#30984=CARTESIAN_POINT('Ctrl Pts',(25.1249357452756,-28.6716070819486,-15.5251351971226));
#30985=CARTESIAN_POINT('Ctrl Pts',(24.1510084067019,-28.1678256190434,-15.5836572228941));
#30986=CARTESIAN_POINT('Ctrl Pts',(22.9245129145126,-27.5141512254857,-15.8853026165582));
#30987=CARTESIAN_POINT('Origin',(40.65,0.,0.));
#30988=CARTESIAN_POINT('',(40.4,-16.1848830792292,-31.0330398077868));
#30989=CARTESIAN_POINT('',(40.9,-15.9346498339374,-30.5996231131986));
#30990=CARTESIAN_POINT('Ctrl Pts',(40.4,-16.1848830792292,-31.0330398077868));
#30991=CARTESIAN_POINT('Ctrl Pts',(40.5666590138495,-16.1014769396247,-30.8885761363286));
#30992=CARTESIAN_POINT('Ctrl Pts',(40.7333430451341,-16.0180571835863,-30.744088880515));
#30993=CARTESIAN_POINT('Ctrl Pts',(40.9,-15.9346498339374,-30.5996231131986));
#30994=CARTESIAN_POINT('',(40.9,-18.5327260452908,-29.0996231131986));
#30995=CARTESIAN_POINT('Origin',(40.9,0.,0.));
#30996=CARTESIAN_POINT('',(40.4,-18.7829592905825,-29.5330398077868));
#30997=CARTESIAN_POINT('Ctrl Pts',(40.9,-18.5327260452908,-29.0996231131986));
#30998=CARTESIAN_POINT('Ctrl Pts',(40.7333430447101,-18.6161333951518,-29.2440888808826));
#30999=CARTESIAN_POINT('Ctrl Pts',(40.5666590132533,-18.6995531512764,-29.3885761368453));
#31000=CARTESIAN_POINT('Ctrl Pts',(40.4,-18.7829592905825,-29.5330398077868));
#31001=CARTESIAN_POINT('Origin',(40.4,0.,0.));
#31002=CARTESIAN_POINT('Origin',(35.7,0.,0.));
#31003=CARTESIAN_POINT('',(30.5,-18.8254200738635,-29.5059919176187));
#31004=CARTESIAN_POINT('Ctrl Pts',(40.3998805977105,-18.782947901926,-29.5330468723878));
#31005=CARTESIAN_POINT('Ctrl Pts',(39.2493532038275,-18.7828975281295,-29.5330781201994));
#31006=CARTESIAN_POINT('Ctrl Pts',(38.0972325173599,-18.7826942098824,-29.5332042421555));
#31007=CARTESIAN_POINT('Ctrl Pts',(36.9466403234098,-18.782625610211,-29.5332467931397));
#31008=CARTESIAN_POINT('Ctrl Pts',(36.745394297411,-18.7826136116842,-29.5332542355824));
#31009=CARTESIAN_POINT('Ctrl Pts',(36.5441950314761,-18.7826057345052,-29.5332591213989));
#31010=CARTESIAN_POINT('Ctrl Pts',(36.3429831482489,-18.7825981392881,-29.5332638326403));
#31011=CARTESIAN_POINT('Ctrl Pts',(36.2103627229667,-18.7825931332173,-29.5332669378586));
#31012=CARTESIAN_POINT('Ctrl Pts',(36.0823539051257,-18.7825884046849,-29.5332699079689));
#31013=CARTESIAN_POINT('Ctrl Pts',(35.9587472612939,-18.7825830316391,-29.5332733040083));
#31014=CARTESIAN_POINT('Ctrl Pts',(35.7554552091584,-18.7825741947555,-29.5332788893701));
#31015=CARTESIAN_POINT('Ctrl Pts',(35.5640774639622,-18.7825638026986,-29.5332855100023));
#31016=CARTESIAN_POINT('Ctrl Pts',(35.3838244596856,-18.782553672802,-29.5332919882553));
#31017=CARTESIAN_POINT('Ctrl Pts',(35.2391029657229,-18.7825455397126,-29.5332971895137));
#31018=CARTESIAN_POINT('Ctrl Pts',(35.1015509582127,-18.7825375448577,-29.5333023181014));
#31019=CARTESIAN_POINT('Ctrl Pts',(34.9707359993668,-18.7825301857251,-29.53330703978));
#31020=CARTESIAN_POINT('Ctrl Pts',(34.8578981782314,-18.7825238379151,-29.5333111125858));
#31021=CARTESIAN_POINT('Ctrl Pts',(34.7500670454672,-18.7825179390022,-29.5333148977088));
#31022=CARTESIAN_POINT('Ctrl Pts',(34.6468496336297,-18.782512339199,-29.5333184739616));
#31023=CARTESIAN_POINT('Ctrl Pts',(34.5887227637969,-18.7825091856706,-29.5333204879278));
#31024=CARTESIAN_POINT('Ctrl Pts',(34.5320601650633,-18.7825061280823,-29.5333224349598));
#31025=CARTESIAN_POINT('Ctrl Pts',(34.4767987085459,-18.7825031467929,-29.5333243245742));
#31026=CARTESIAN_POINT('Ctrl Pts',(34.3959515551434,-18.7824987851858,-29.5333270890679));
#31027=CARTESIAN_POINT('Ctrl Pts',(34.3181086379454,-18.7824945796072,-29.533329735068));
#31028=CARTESIAN_POINT('Ctrl Pts',(34.2432236356786,-18.7824903289018,-29.5333323757534));
#31029=CARTESIAN_POINT('Ctrl Pts',(34.1622675304678,-18.7824857335818,-29.5333352305253));
#31030=CARTESIAN_POINT('Ctrl Pts',(34.0847679660331,-18.7824810863437,-29.5333380785848));
#31031=CARTESIAN_POINT('Ctrl Pts',(34.0106064145705,-18.7824762391415,-29.533340998409));
#31032=CARTESIAN_POINT('Ctrl Pts',(34.0011740964187,-18.7824756226448,-29.53334136977));
#31033=CARTESIAN_POINT('Ctrl Pts',(33.9917957065823,-18.7824750030335,-29.5333417422189));
#31034=CARTESIAN_POINT('Ctrl Pts',(33.9824709442606,-18.7824743801028,-29.5333421158564));
#31035=CARTESIAN_POINT('Ctrl Pts',(33.9223617768599,-18.7824703645751,-29.533344524394));
#31036=CARTESIAN_POINT('Ctrl Pts',(33.8644761964478,-18.7824662176988,-29.5333469783448));
#31037=CARTESIAN_POINT('Ctrl Pts',(33.8085662292047,-18.7824621301166,-29.5333493560321));
#31038=CARTESIAN_POINT('Ctrl Pts',(33.7474237016288,-18.7824576599816,-29.533351956245));
#31039=CARTESIAN_POINT('Ctrl Pts',(33.6886441629994,-18.782453260435,-29.5333544654464));
#31040=CARTESIAN_POINT('Ctrl Pts',(33.6319696815835,-18.7824490897764,-29.5333567795391));
#31041=CARTESIAN_POINT('Ctrl Pts',(33.5826925637836,-18.7824454634877,-29.5333587915877));
#31042=CARTESIAN_POINT('Ctrl Pts',(33.5350083429209,-18.7824420082021,-29.5333606573655));
#31043=CARTESIAN_POINT('Ctrl Pts',(33.4887791610839,-18.7824387840041,-29.5333623350385));
#31044=CARTESIAN_POINT('Ctrl Pts',(33.4518540160536,-18.7824362087048,-29.5333636750648));
#31045=CARTESIAN_POINT('Ctrl Pts',(33.4158630419527,-18.7824337707087,-29.5333649012377));
#31046=CARTESIAN_POINT('Ctrl Pts',(33.3809178974527,-18.7824311830501,-29.5333661853037));
#31047=CARTESIAN_POINT('Ctrl Pts',(33.3430135142412,-18.7824283762623,-29.5333675781075));
#31048=CARTESIAN_POINT('Ctrl Pts',(33.3063394414416,-18.7824253936822,-29.5333690388471));
#31049=CARTESIAN_POINT('Ctrl Pts',(33.2709744550635,-18.7824219844966,-29.5333707164935));
#31050=CARTESIAN_POINT('Ctrl Pts',(33.2337091834356,-18.7824183921235,-29.5333724842856));
#31051=CARTESIAN_POINT('Ctrl Pts',(33.1978968817727,-18.7824143271502,-29.5333744922618));
#31052=CARTESIAN_POINT('Ctrl Pts',(33.1635680440812,-18.7824096073364,-29.5333768470679));
#31053=CARTESIAN_POINT('Ctrl Pts',(33.125851795334,-18.7824044217933,-29.5333794342353));
#31054=CARTESIAN_POINT('Ctrl Pts',(33.0899258347182,-18.7823984465448,-29.5333824396031));
#31055=CARTESIAN_POINT('Ctrl Pts',(33.0557653925381,-18.7823915567442,-29.5333859335397));
#31056=CARTESIAN_POINT('Ctrl Pts',(33.0368719877466,-18.7823877461438,-29.5333878659608));
#31057=CARTESIAN_POINT('Ctrl Pts',(33.0185175727353,-18.7823836577058,-29.5333899466652));
#31058=CARTESIAN_POINT('Ctrl Pts',(33.0006913489163,-18.7823792820484,-29.5333921804186));
#31059=CARTESIAN_POINT('Ctrl Pts',(32.9433364918128,-18.7823652036207,-29.5333993673924));
#31060=CARTESIAN_POINT('Ctrl Pts',(32.889323201888,-18.78254762761,-29.5332829792212));
#31061=CARTESIAN_POINT('Ctrl Pts',(32.8382230276384,-18.7828441879673,-29.5330947066102));
#31062=CARTESIAN_POINT('Ctrl Pts',(32.7810653124613,-18.7831759033222,-29.5328841156987));
#31063=CARTESIAN_POINT('Ctrl Pts',(32.727552456734,-18.7836507315896,-29.5325833908465));
#31064=CARTESIAN_POINT('Ctrl Pts',(32.6770430180203,-18.7841988326963,-29.532236338609));
#31065=CARTESIAN_POINT('Ctrl Pts',(32.6227203152382,-18.7847883132819,-29.5318630852917));
#31066=CARTESIAN_POINT('Ctrl Pts',(32.5718714572479,-18.785463223046,-29.5314358211882));
#31067=CARTESIAN_POINT('Ctrl Pts',(32.5236533105896,-18.7861776883228,-29.5309832901274));
#31068=CARTESIAN_POINT('Ctrl Pts',(32.4718100172051,-18.7869458686765,-29.5304967367823));
#31069=CARTESIAN_POINT('Ctrl Pts',(32.4230076638009,-18.7877604440451,-29.5299805544879));
#31070=CARTESIAN_POINT('Ctrl Pts',(32.3761512173999,-18.7885990068259,-29.5294487410664));
#31071=CARTESIAN_POINT('Ctrl Pts',(32.3248096593241,-18.789517837062,-29.5288660223209));
#31072=CARTESIAN_POINT('Ctrl Pts',(32.2758043952268,-18.7904660501636,-29.5282641699575));
#31073=CARTESIAN_POINT('Ctrl Pts',(32.2276418902244,-18.7914438969209,-29.5276429421487));
#31074=CARTESIAN_POINT('Ctrl Pts',(32.1780484881789,-18.7924507952825,-29.5270032578033));
#31075=CARTESIAN_POINT('Ctrl Pts',(32.129348520974,-18.7934898292201,-29.5263425802702));
#31076=CARTESIAN_POINT('Ctrl Pts',(32.0798596724228,-18.7945806304077,-29.525648507911));
#31077=CARTESIAN_POINT('Ctrl Pts',(32.031031972984,-18.7956568589742,-29.5249637080513));
#31078=CARTESIAN_POINT('Ctrl Pts',(31.9814363681891,-18.7967841298918,-29.5242459916461));
#31079=CARTESIAN_POINT('Ctrl Pts',(31.9294088358078,-18.7979897030586,-29.5234781935338));
#31080=CARTESIAN_POINT('Ctrl Pts',(31.898016936455,-18.7987171108326,-29.523014926491));
#31081=CARTESIAN_POINT('Ctrl Pts',(31.8657387727398,-18.7994731540541,-29.5225333463335));
#31082=CARTESIAN_POINT('Ctrl Pts',(31.8321995512669,-18.8002637764333,-29.5220297160307));
#31083=CARTESIAN_POINT('Ctrl Pts',(31.7313430764712,-18.8026412730644,-29.5205152391074));
#31084=CARTESIAN_POINT('Ctrl Pts',(31.6280303047182,-18.8051208626313,-29.5189339807854));
#31085=CARTESIAN_POINT('Ctrl Pts',(31.5230436279567,-18.8075570028383,-29.5173797885034));
#31086=CARTESIAN_POINT('Ctrl Pts',(31.4165412786074,-18.8100283131358,-29.5158031586445));
#31087=CARTESIAN_POINT('Ctrl Pts',(31.308316172914,-18.8124535008248,-29.5142552682412));
#31088=CARTESIAN_POINT('Ctrl Pts',(31.1992361814705,-18.8146708543332,-29.512840201736));
#31089=CARTESIAN_POINT('Ctrl Pts',(31.1417800745714,-18.8158388091388,-29.5120948385276));
#31090=CARTESIAN_POINT('Ctrl Pts',(31.0840876480106,-18.8169490689289,-29.5113863465313));
#31091=CARTESIAN_POINT('Ctrl Pts',(31.0262914639723,-18.8179790482416,-29.5107292749179));
#31092=CARTESIAN_POINT('Ctrl Pts',(30.9238422544137,-18.8198047841132,-29.5095645532577));
#31093=CARTESIAN_POINT('Ctrl Pts',(30.8210652532058,-18.8213763539421,-29.5085625948816));
#31094=CARTESIAN_POINT('Ctrl Pts',(30.718765507456,-18.8225556950176,-29.507810834769));
#31095=CARTESIAN_POINT('Ctrl Pts',(30.6466529343875,-18.82338702963,-29.5072809081729));
#31096=CARTESIAN_POINT('Ctrl Pts',(30.5747782907563,-18.8240238717387,-29.5068750504575));
#31097=CARTESIAN_POINT('Ctrl Pts',(30.503432395139,-18.8244289981692,-29.5066169468345));
#31098=CARTESIAN_POINT('Ctrl Pts',(30.5006731185507,-18.8244446662867,-29.5066069647707));
#31099=CARTESIAN_POINT('Ctrl Pts',(30.497914633606,-18.8244599892394,-29.5065972028237));
#31100=CARTESIAN_POINT('Ctrl Pts',(30.4951569527683,-18.8244749650172,-29.5065876622664));
#31101=CARTESIAN_POINT('',(30.5,-16.229443021655,-31.0097594187194));
#31102=CARTESIAN_POINT('Origin',(30.5,0.,0.));
#31103=CARTESIAN_POINT('Ctrl Pts',(30.5049076308141,-16.2304573503026,-31.0091238687319));
#31104=CARTESIAN_POINT('Ctrl Pts',(30.5973062294345,-16.2298682766552,-31.0094328533548));
#31105=CARTESIAN_POINT('Ctrl Pts',(30.689059158586,-16.2288427503286,-31.0099692677028));
#31106=CARTESIAN_POINT('Ctrl Pts',(30.7806364364919,-16.2274919709621,-31.0106763092384));
#31107=CARTESIAN_POINT('Ctrl Pts',(30.8441456090292,-16.2265552005994,-31.0111666450936));
#31108=CARTESIAN_POINT('Ctrl Pts',(30.9075713010184,-16.2254611740684,-31.0117394593184));
#31109=CARTESIAN_POINT('Ctrl Pts',(30.9710816356704,-16.2242390174924,-31.0123798375508));
#31110=CARTESIAN_POINT('Ctrl Pts',(31.0734991469995,-16.2222681534488,-31.0134125190071));
#31111=CARTESIAN_POINT('Ctrl Pts',(31.1761345288068,-16.2199648111636,-31.0146205155167));
#31112=CARTESIAN_POINT('Ctrl Pts',(31.279810056847,-16.2174702047238,-31.0159286966544));
#31113=CARTESIAN_POINT('Ctrl Pts',(31.3828326297126,-16.2149913094766,-31.0172286387828));
#31114=CARTESIAN_POINT('Ctrl Pts',(31.4868822244325,-16.2123218973815,-31.0186283615542));
#31115=CARTESIAN_POINT('Ctrl Pts',(31.5928140565585,-16.2095937955791,-31.020057669606));
#31116=CARTESIAN_POINT('Ctrl Pts',(31.6516194621098,-16.208079358137,-31.0208511142011));
#31117=CARTESIAN_POINT('Ctrl Pts',(31.7110057676085,-16.2065468518028,-31.0216536678951));
#31118=CARTESIAN_POINT('Ctrl Pts',(31.7711259776529,-16.2050208141949,-31.0224523036437));
#31119=CARTESIAN_POINT('Ctrl Pts',(31.8409078613427,-16.2032495333099,-31.0233792848848));
#31120=CARTESIAN_POINT('Ctrl Pts',(31.9056298453964,-16.2016434584277,-31.0242198767433));
#31121=CARTESIAN_POINT('Ctrl Pts',(31.9658749467865,-16.2002018139142,-31.0249744961546));
#31122=CARTESIAN_POINT('Ctrl Pts',(32.0341046687228,-16.1985691001829,-31.0258291295008));
#31123=CARTESIAN_POINT('Ctrl Pts',(32.0965918298941,-16.1971462744691,-31.026574015819));
#31124=CARTESIAN_POINT('Ctrl Pts',(32.1542461945013,-16.1959042389539,-31.0272242625029));
#31125=CARTESIAN_POINT('Ctrl Pts',(32.215166595352,-16.1945918439258,-31.0279113447196));
#31126=CARTESIAN_POINT('Ctrl Pts',(32.2706916712563,-16.1934801514051,-31.0284933558527));
#31127=CARTESIAN_POINT('Ctrl Pts',(32.3219582775162,-16.1925241206212,-31.0289937114781));
#31128=CARTESIAN_POINT('Ctrl Pts',(32.3761916324778,-16.1915127652646,-31.0295230221975));
#31129=CARTESIAN_POINT('Ctrl Pts',(32.425659986223,-16.1906748064835,-31.0299613681536));
#31130=CARTESIAN_POINT('Ctrl Pts',(32.4717693483789,-16.1899610544418,-31.0303343957023));
#31131=CARTESIAN_POINT('Ctrl Pts',(32.521533200307,-16.1891907325537,-31.0307369882959));
#31132=CARTESIAN_POINT('Ctrl Pts',(32.5673849287952,-16.1885644631731,-31.0310638203075));
#31133=CARTESIAN_POINT('Ctrl Pts',(32.6111519417719,-16.1880367365758,-31.0313387615313));
#31134=CARTESIAN_POINT('Ctrl Pts',(32.6551741210746,-16.1875059332764,-31.0316153056916));
#31135=CARTESIAN_POINT('Ctrl Pts',(32.697087871783,-16.1870745377529,-31.0318395012595));
#31136=CARTESIAN_POINT('Ctrl Pts',(32.7388013470514,-16.1867185738399,-31.0320241553172));
#31137=CARTESIAN_POINT('Ctrl Pts',(32.7801521457873,-16.1863657048443,-31.0322072039058));
#31138=CARTESIAN_POINT('Ctrl Pts',(32.8213062770012,-16.1860865454659,-31.0323516104906));
#31139=CARTESIAN_POINT('Ctrl Pts',(32.8641640035292,-16.1858844594634,-31.0324560971769));
#31140=CARTESIAN_POINT('Ctrl Pts',(32.9038200784524,-16.1856974701314,-31.0325527782703));
#31141=CARTESIAN_POINT('Ctrl Pts',(32.944934777289,-16.1855761117061,-31.0326154655019));
#31142=CARTESIAN_POINT('Ctrl Pts',(32.9890474705801,-16.1855509840873,-31.0326287580452));
#31143=CARTESIAN_POINT('Ctrl Pts',(32.9926089293361,-16.1855489553974,-31.0326298312248));
#31144=CARTESIAN_POINT('Ctrl Pts',(32.9961899495402,-16.1855475722577,-31.0326305730127));
#31145=CARTESIAN_POINT('Ctrl Pts',(32.9997913521114,-16.1855468609619,-31.0326309700537));
#31146=CARTESIAN_POINT('Ctrl Pts',(33.0362292496771,-16.1855396642873,-31.0326349871946));
#31147=CARTESIAN_POINT('Ctrl Pts',(33.0740922921119,-16.1855331333215,-31.0326386992184));
#31148=CARTESIAN_POINT('Ctrl Pts',(33.114143918563,-16.1855273500631,-31.0326422490868));
#31149=CARTESIAN_POINT('Ctrl Pts',(33.2461674547434,-16.1855082865122,-31.0326539506383));
#31150=CARTESIAN_POINT('Ctrl Pts',(33.3721931286568,-16.1855003220479,-31.0326588963952));
#31151=CARTESIAN_POINT('Ctrl Pts',(33.4993879207448,-16.1854928138549,-31.0326635427516));
#31152=CARTESIAN_POINT('Ctrl Pts',(33.6627849160625,-16.1854831686789,-31.0326695115547));
#31153=CARTESIAN_POINT('Ctrl Pts',(33.8281112474539,-16.1854742764644,-31.0326749862722));
#31154=CARTESIAN_POINT('Ctrl Pts',(33.9929845306743,-16.1854606405093,-31.0326833946004));
#31155=CARTESIAN_POINT('Ctrl Pts',(34.3227310971151,-16.1854333685992,-31.0327002112569));
#31156=CARTESIAN_POINT('Ctrl Pts',(34.6506654708718,-16.1853871217269,-31.032728762356));
#31157=CARTESIAN_POINT('Ctrl Pts',(34.979269363621,-16.1853559472169,-31.032748004237));
#31158=CARTESIAN_POINT('Ctrl Pts',(35.3078732563701,-16.1853247727068,-31.032767246118));
#31159=CARTESIAN_POINT('Ctrl Pts',(35.6371466681116,-16.185308670559,-31.032777178781));
#31160=CARTESIAN_POINT('Ctrl Pts',(35.9662682695208,-16.1852951338216,-31.0327855310262));
#31161=CARTESIAN_POINT('Ctrl Pts',(36.29538987093,-16.1852815970843,-31.0327938832713));
#31162=CARTESIAN_POINT('Ctrl Pts',(36.6243596620069,-16.1852706257574,-31.0328006550988));
#31163=CARTESIAN_POINT('Ctrl Pts',(36.9532592751492,-16.185248102247,-31.0328145551759));
#31164=CARTESIAN_POINT('Ctrl Pts',(38.102326278026,-16.1851694125146,-31.0328631174705));
#31165=CARTESIAN_POINT('Ctrl Pts',(39.2505367075414,-16.184949719878,-31.0329986853002));
#31166=CARTESIAN_POINT('Ctrl Pts',(40.4000986012038,-16.1848953623403,-31.0330322281526));
#31167=CARTESIAN_POINT('Ctrl Pts',(6.89999999997365,0.168526548676475,-11.0276873985587));
#31168=CARTESIAN_POINT('Ctrl Pts',(6.99168932310453,0.107121039164007,-11.0290491215116));
#31169=CARTESIAN_POINT('Ctrl Pts',(7.08383940291242,0.0458098125994604,
-11.0299018391088));
#31170=CARTESIAN_POINT('Ctrl Pts',(8.15761824498006,-0.664186592400577,
-11.0337651740187));
#31171=CARTESIAN_POINT('Ctrl Pts',(9.16607857437499,-1.30870352701556,-10.9699676285446));
#31172=CARTESIAN_POINT('Ctrl Pts',(11.2535171643192,-2.47376106241928,-10.77603305676));
#31173=CARTESIAN_POINT('Ctrl Pts',(12.2576790632369,-3.00237606292525,-10.6330057282434));
#31174=CARTESIAN_POINT('Ctrl Pts',(14.3563663857894,-3.944470058834,-10.3307260661656));
#31175=CARTESIAN_POINT('Ctrl Pts',(15.3658129161116,-4.36032593857961,-10.1540434041659));
#31176=CARTESIAN_POINT('Ctrl Pts',(17.4727193021212,-5.08193366885832,-9.82334300624283));
#31177=CARTESIAN_POINT('Ctrl Pts',(18.4888802671462,-5.39169279079136,-9.6488422591121));
#31178=CARTESIAN_POINT('Ctrl Pts',(19.8473882183426,-5.72385817850078,-9.45778984314827));
#31179=CARTESIAN_POINT('Ctrl Pts',(20.3451395577184,-5.84063156394592,-9.38741838105894));
#31180=CARTESIAN_POINT('Ctrl Pts',(21.119864121141,-6.00690103675049,-9.28201599203951));
#31181=CARTESIAN_POINT('Ctrl Pts',(21.9116430735678,-6.15921075032182,-9.18172875488037));
#31182=CARTESIAN_POINT('Ctrl Pts',(22.4533884343746,-6.25063668203688,-9.12054551137776));
#31183=CARTESIAN_POINT('Ctrl Pts',(22.8546099577479,-6.31320896750581,-9.07881438233611));
#31184=CARTESIAN_POINT('Ctrl Pts',(23.1058218650381,-6.35118260107244,-9.05298395410355));
#31185=CARTESIAN_POINT('Ctrl Pts',(23.6175153199788,-6.42382403760963,-9.00245668094437));
#31186=CARTESIAN_POINT('Ctrl Pts',(24.1364702886545,-6.49007583237977,-8.95485371029554));
#31187=CARTESIAN_POINT('Ctrl Pts',(24.6629181373246,-6.54944423929279,-8.91145225308144));
#31188=CARTESIAN_POINT('Ctrl Pts',(25.0606678571037,-6.59024788291775,-8.88140293076164));
#31189=CARTESIAN_POINT('Ctrl Pts',(25.3945416155882,-6.62099228309709,-8.85873533710263));
#31190=CARTESIAN_POINT('Ctrl Pts',(25.6627586119464,-6.64352323130153,-8.84221409068032));
#31191=CARTESIAN_POINT('Ctrl Pts',(25.7972076165425,-6.65408072739386,-8.83452216013014));
#31192=CARTESIAN_POINT('Ctrl Pts',(26.3824137782946,-6.69837697633853,-8.80240169886323));
#31193=CARTESIAN_POINT('Ctrl Pts',(27.4369717967155,-6.74704662082202,-8.76563881905853));
#31194=CARTESIAN_POINT('Ctrl Pts',(28.4593635146677,-6.76713562537254,-8.74917816753949));
#31195=CARTESIAN_POINT('Ctrl Pts',(29.0427481469891,-6.77974505298722,-8.73952198264543));
#31196=CARTESIAN_POINT('Ctrl Pts',(29.2174939164952,-6.78306424239322,-8.73701514175017));
#31197=CARTESIAN_POINT('Ctrl Pts',(29.5607048332279,-6.78786835107261,-8.73336568489192));
#31198=CARTESIAN_POINT('Ctrl Pts',(29.9899637006214,-6.79106253935676,-8.73093988338427));
#31199=CARTESIAN_POINT('Ctrl Pts',(30.5003627545718,-6.79139754852948,-8.73068255391871));
#31200=CARTESIAN_POINT('Ctrl Pts',(31.5152290141054,-6.78728755019409,-8.73381293113858));
#31201=CARTESIAN_POINT('Ctrl Pts',(32.346385618228,-6.77838967797265,-8.74063107149334));
#31202=CARTESIAN_POINT('Ctrl Pts',(33.1616392309915,-6.77840182636605,-8.74062146997073));
#31203=CARTESIAN_POINT('Ctrl Pts',(33.4928689770884,-6.77840284181041,-8.74062052628883));
#31204=CARTESIAN_POINT('Ctrl Pts',(33.9856875201801,-6.77840526161275,-8.74061852020512));
#31205=CARTESIAN_POINT('Ctrl Pts',(34.4799569296089,-6.7784068708528,-8.74061713883255));
#31206=CARTESIAN_POINT('Ctrl Pts',(35.1382080085716,-6.778409075901,-8.74061527897128));
#31207=CARTESIAN_POINT('Ctrl Pts',(35.9613703496106,-6.7784121544085,-8.74061266742264));
#31208=CARTESIAN_POINT('Ctrl Pts',(37.9364530322258,-6.77841531264166,-8.74060999527037));
#31209=CARTESIAN_POINT('Ctrl Pts',(39.5833333333333,-6.7784348060232,-8.74059347982545));
#31210=CARTESIAN_POINT('Ctrl Pts',(40.9,-6.7784348060232,-8.74059347982545));
#31211=CARTESIAN_POINT('Ctrl Pts',(6.71972576838711,0.727849695365748,-14.4135489955738));
#31212=CARTESIAN_POINT('Ctrl Pts',(6.81144220747046,0.647520064289719,-14.4181051875223));
#31213=CARTESIAN_POINT('Ctrl Pts',(6.90362846895807,0.56728056977469,-14.4219897194692));
#31214=CARTESIAN_POINT('Ctrl Pts',(7.97787094717212,-0.361837668282348,
-14.4591555519285));
#31215=CARTESIAN_POINT('Ctrl Pts',(8.98682261267022,-1.20743712855003,-14.4048184698324));
#31216=CARTESIAN_POINT('Ctrl Pts',(11.0806424583842,-2.74422300498291,-14.2022941804566));
#31217=CARTESIAN_POINT('Ctrl Pts',(12.0862214600973,-3.44223257454471,-14.038891127913));
#31218=CARTESIAN_POINT('Ctrl Pts',(14.1975721203649,-4.69396502652543,-13.6830024292515));
#31219=CARTESIAN_POINT('Ctrl Pts',(15.2099789251839,-5.24642829788655,-13.4699449244818));
#31220=CARTESIAN_POINT('Ctrl Pts',(17.3362999248755,-6.21145869787377,-13.0656161985035));
#31221=CARTESIAN_POINT('Ctrl Pts',(18.357013455463,-6.62511541331198,-12.850252612086));
#31222=CARTESIAN_POINT('Ctrl Pts',(19.7328409259837,-7.07198752003369,-12.6121436508471));
#31223=CARTESIAN_POINT('Ctrl Pts',(20.2337632876373,-7.22841114520151,-12.5247332071257));
#31224=CARTESIAN_POINT('Ctrl Pts',(21.0166345413949,-7.45203181169807,-12.3929576501156));
#31225=CARTESIAN_POINT('Ctrl Pts',(21.8175391230323,-7.65714338227215,-12.2672157657621));
#31226=CARTESIAN_POINT('Ctrl Pts',(22.3668263920487,-7.78054947414231,-12.190248920123));
#31227=CARTESIAN_POINT('Ctrl Pts',(22.7739396967848,-7.86506298164211,-12.1377120270328));
#31228=CARTESIAN_POINT('Ctrl Pts',(23.0274297041713,-7.916156632735,-12.1053188608807));
#31229=CARTESIAN_POINT('Ctrl Pts',(23.5449351393661,-8.01409846114017,-12.0417665186343));
#31230=CARTESIAN_POINT('Ctrl Pts',(24.0699575659665,-8.1034816713378,-11.9817953425795));
#31231=CARTESIAN_POINT('Ctrl Pts',(24.6032835407751,-8.18369268569514,-11.9270075754273));
#31232=CARTESIAN_POINT('Ctrl Pts',(25.0064847905103,-8.23885952183869,-11.8890391550575));
#31233=CARTESIAN_POINT('Ctrl Pts',(25.3452465270805,-8.28045801654025,-11.8603696837558));
#31234=CARTESIAN_POINT('Ctrl Pts',(25.6175460563752,-8.31095886138244,-11.8394640015962));
#31235=CARTESIAN_POINT('Ctrl Pts',(25.75409426488,-8.32525512288968,-11.8297282412419));
#31236=CARTESIAN_POINT('Ctrl Pts',(26.34877806292,-8.38525559473467,-11.7890598714193));
#31237=CARTESIAN_POINT('Ctrl Pts',(27.420647343066,-8.4511591136706,-11.7424863739248));
#31238=CARTESIAN_POINT('Ctrl Pts',(28.4470245212717,-8.47809267828295,-11.7218144944205));
#31239=CARTESIAN_POINT('Ctrl Pts',(29.0301431861018,-8.49498332574136,-11.7097207064843));
#31240=CARTESIAN_POINT('Ctrl Pts',(29.2075511609936,-8.49948124637056,-11.7065424548688));
#31241=CARTESIAN_POINT('Ctrl Pts',(29.5540559241346,-8.50596054299459,-11.7019389390664));
#31242=CARTESIAN_POINT('Ctrl Pts',(29.9873899374288,-8.51027178683721,-11.6988759349841));
#31243=CARTESIAN_POINT('Ctrl Pts',(30.501058587611,-8.51072031244606,-11.6985535595641));
#31244=CARTESIAN_POINT('Ctrl Pts',(31.520398261889,-8.50519297418975,-11.7024891534661));
#31245=CARTESIAN_POINT('Ctrl Pts',(32.3504760849347,-8.49329404471495,-11.7110091605269));
#31246=CARTESIAN_POINT('Ctrl Pts',(33.1607219786944,-8.49331406281709,-11.7109930603161));
#31247=CARTESIAN_POINT('Ctrl Pts',(33.4925972550183,-8.49331574772297,-11.7109914601493));
#31248=CARTESIAN_POINT('Ctrl Pts',(33.9851239882619,-8.49331974280042,-11.7109880844892));
#31249=CARTESIAN_POINT('Ctrl Pts',(34.4795557496198,-8.49332240354984,-11.7109857543654));
#31250=CARTESIAN_POINT('Ctrl Pts',(35.1377808103951,-8.49332604669792,-11.7109826209376));
#31251=CARTESIAN_POINT('Ctrl Pts',(35.9610196518539,-8.49333113419868,-11.7109782193289));
#31252=CARTESIAN_POINT('Ctrl Pts',(37.9361278153251,-8.49333635287233,-11.7109737164007));
#31253=CARTESIAN_POINT('Ctrl Pts',(39.5833333333333,-8.49336856563262,-11.7109458830841));
#31254=CARTESIAN_POINT('Ctrl Pts',(40.9,-8.49336856563262,-11.7109458830841));
#31255=CARTESIAN_POINT('Ctrl Pts',(6.48175880232276,2.0223358101383,-22.3152648782349));
#31256=CARTESIAN_POINT('Ctrl Pts',(6.5727030402579,1.89877066361228,-22.3270401223923));
#31257=CARTESIAN_POINT('Ctrl Pts',(6.66410021308729,1.77531589258794,-22.3377778183098));
#31258=CARTESIAN_POINT('Ctrl Pts',(7.73046719612232,0.343647388924397,-22.4505948584363));
#31259=CARTESIAN_POINT('Ctrl Pts',(8.73293490974102,-0.965853752252137,
-22.4183684385317));
#31260=CARTESIAN_POINT('Ctrl Pts',(10.8102891123217,-3.35126151217317,-22.1981640385547));
#31261=CARTESIAN_POINT('Ctrl Pts',(11.8125652928685,-4.44249581664877,-21.9890905805956));
#31262=CARTESIAN_POINT('Ctrl Pts',(13.9177091187558,-6.40690464277105,-21.5128074248294));
#31263=CARTESIAN_POINT('Ctrl Pts',(14.9295907318602,-7.27826244175744,-21.2167997396941));
#31264=CARTESIAN_POINT('Ctrl Pts',(17.0679705254901,-8.81262608188777,-20.6429560449296));
#31265=CARTESIAN_POINT('Ctrl Pts',(18.0930327325161,-9.47115000177604,-20.3328482957165));
#31266=CARTESIAN_POINT('Ctrl Pts',(19.4931651654931,-10.1918150595348,-19.9834260609175));
#31267=CARTESIAN_POINT('Ctrl Pts',(19.9989304172552,-10.4420751188792,-19.8560672526628));
#31268=CARTESIAN_POINT('Ctrl Pts',(20.794811594708,-10.8025573386247,-19.6618467626018));
#31269=CARTESIAN_POINT('Ctrl Pts',(21.6117660259797,-11.1342859263411,-19.4754657432766));
#31270=CARTESIAN_POINT('Ctrl Pts',(22.1753497026275,-11.3349591405942,-19.3605546952356));
#31271=CARTESIAN_POINT('Ctrl Pts',(22.5940479063322,-11.47260657239,-19.2819382297017));
#31272=CARTESIAN_POINT('Ctrl Pts',(22.8520812047022,-11.5550617085391,-19.2339198113556));
#31273=CARTESIAN_POINT('Ctrl Pts',(23.3813360719091,-11.7138435277865,-19.1391573021403));
#31274=CARTESIAN_POINT('Ctrl Pts',(23.9190563543678,-11.8589452906513,-19.0494991042743));
#31275=CARTESIAN_POINT('Ctrl Pts',(24.4671051082233,-11.989559546254,-18.9672572385016));
#31276=CARTESIAN_POINT('Ctrl Pts',(24.8821466483761,-12.0795190000423,-18.9101500634532));
#31277=CARTESIAN_POINT('Ctrl Pts',(25.2317043848841,-12.1474851335067,-18.8669280179621));
#31278=CARTESIAN_POINT('Ctrl Pts',(25.5130950900239,-12.1973721681455,-18.8353673631031));
#31279=CARTESIAN_POINT('Ctrl Pts',(25.6543465475614,-12.2207724172661,-18.8206563371687));
#31280=CARTESIAN_POINT('Ctrl Pts',(26.2703768283174,-12.3190725812828,-18.7591443923488));
#31281=CARTESIAN_POINT('Ctrl Pts',(27.3823409200252,-12.4269409232394,-18.6887004197342));
#31282=CARTESIAN_POINT('Ctrl Pts',(28.4180912195453,-12.4698946357076,-18.6581821178487));
#31283=CARTESIAN_POINT('Ctrl Pts',(29.0006188348746,-12.4967855079752,-18.6404003655932));
#31284=CARTESIAN_POINT('Ctrl Pts',(29.1842244806991,-12.5041566301777,-18.6355848623939));
#31285=CARTESIAN_POINT('Ctrl Pts',(29.5384110471465,-12.5146498740616,-18.6286952117012));
#31286=CARTESIAN_POINT('Ctrl Pts',(29.9812601150293,-12.5216494975055,-18.6240999155071));
#31287=CARTESIAN_POINT('Ctrl Pts',(30.5025631839301,-12.5223645690813,-18.6236255844566));
#31288=CARTESIAN_POINT('Ctrl Pts',(31.5323495650756,-12.5134871029148,-18.6294670720537));
#31289=CARTESIAN_POINT('Ctrl Pts',(32.3599484134842,-12.4946603930139,-18.6419219593216));
#31290=CARTESIAN_POINT('Ctrl Pts',(33.1585258504257,-12.4947174829697,-18.6418830267369));
#31291=CARTESIAN_POINT('Ctrl Pts',(33.4919095878066,-12.4947228565319,-18.6418790995137));
#31292=CARTESIAN_POINT('Ctrl Pts',(33.9837592380106,-12.4947346270607,-18.6418708983646));
#31293=CARTESIAN_POINT('Ctrl Pts',(34.4785726427749,-12.4947426563109,-18.6418652189506));
#31294=CARTESIAN_POINT('Ctrl Pts',(35.1367406589071,-12.4947535178469,-18.6418575939256));
#31295=CARTESIAN_POINT('Ctrl Pts',(35.9601632093981,-12.4947687456191,-18.641846877137));
#31296=CARTESIAN_POINT('Ctrl Pts',(37.9353361278946,-12.4947843377882,-18.6418359163297));
#31297=CARTESIAN_POINT('Ctrl Pts',(39.5833333333333,-12.4948806713879,-18.6417681573542));
#31298=CARTESIAN_POINT('Ctrl Pts',(40.9,-12.4948806713879,-18.6417681573542));
#31299=CARTESIAN_POINT('Ctrl Pts',(6.40644620858991,3.20016516784475,-30.2320800787095));
#31300=CARTESIAN_POINT('Ctrl Pts',(6.49686818484384,3.03404698664167,-30.2503623618083));
#31301=CARTESIAN_POINT('Ctrl Pts',(6.58771890650216,2.86810360702043,-30.2672526113879));
#31302=CARTESIAN_POINT('Ctrl Pts',(7.64885862899863,0.940991822615538,-30.4476905739236));
#31303=CARTESIAN_POINT('Ctrl Pts',(8.64788707329236,-0.826287776604476,
-30.430792173042));
#31304=CARTESIAN_POINT('Ctrl Pts',(10.707154859542,-4.031357203037,-30.1856445659011));
#31305=CARTESIAN_POINT('Ctrl Pts',(11.7059935225822,-5.50908116677459,-29.9282222211751));
#31306=CARTESIAN_POINT('Ctrl Pts',(13.7894394913649,-8.15261547988191,-29.3339211293757));
#31307=CARTESIAN_POINT('Ctrl Pts',(14.7965025532944,-9.33507154947816,-28.9559671306032));
#31308=CARTESIAN_POINT('Ctrl Pts',(16.9150296648082,-11.4103698853377,-28.2210428396417));
#31309=CARTESIAN_POINT('Ctrl Pts',(17.9356459667173,-12.3080290796725,-27.8189128366825));
#31310=CARTESIAN_POINT('Ctrl Pts',(19.3316976380886,-13.2937048286054,-27.3625462801585));
#31311=CARTESIAN_POINT('Ctrl Pts',(19.8372125803626,-13.6366910969767,-27.1960046691455));
#31312=CARTESIAN_POINT('Ctrl Pts',(20.6335801906183,-14.1320040365234,-26.9406914971977));
#31313=CARTESIAN_POINT('Ctrl Pts',(21.4537597225929,-14.5899345529251,-26.6943052661747));
#31314=CARTESIAN_POINT('Ctrl Pts',(22.0223258890083,-14.8686659459061,-26.5413031957662));
#31315=CARTESIAN_POINT('Ctrl Pts',(22.4461030502075,-15.0605640384028,-26.436200781156));
#31316=CARTESIAN_POINT('Ctrl Pts',(22.7062608359972,-15.1748824403433,-26.3723989822776));
#31317=CARTESIAN_POINT('Ctrl Pts',(23.2414929286472,-15.3959532265256,-26.2458547955408));
#31318=CARTESIAN_POINT('Ctrl Pts',(23.7867279834486,-15.5986167246948,-26.1256827576297));
#31319=CARTESIAN_POINT('Ctrl Pts',(24.3445890668936,-15.7819085569279,-26.0148742888258));
#31320=CARTESIAN_POINT('Ctrl Pts',(24.7681394700222,-15.9085256074861,-25.9376795444545));
#31321=CARTESIAN_POINT('Ctrl Pts',(25.1260106169383,-16.0045350828092,-25.8790242908718));
#31322=CARTESIAN_POINT('Ctrl Pts',(25.4147345926424,-16.0751760807979,-25.8360764159907));
#31323=CARTESIAN_POINT('Ctrl Pts',(25.5598889289846,-16.1083660281041,-25.816019030982));
#31324=CARTESIAN_POINT('Ctrl Pts',(26.193933911503,-16.2480157393789,-25.7320023110876));
#31325=CARTESIAN_POINT('Ctrl Pts',(27.3441597812047,-16.4017510524694,-25.6354753903564));
#31326=CARTESIAN_POINT('Ctrl Pts',(28.3894038584673,-16.4608066876634,-25.5950614103761));
#31327=CARTESIAN_POINT('Ctrl Pts',(28.9713246547182,-16.4977059168027,-25.5715886293348));
#31328=CARTESIAN_POINT('Ctrl Pts',(29.1610585442185,-16.5082319208974,-25.5649734110425));
#31329=CARTESIAN_POINT('Ctrl Pts',(29.5228882487203,-16.5229807852931,-25.5556580156131));
#31330=CARTESIAN_POINT('Ctrl Pts',(29.9752283100297,-16.5328527231063,-25.5494240137562));
#31331=CARTESIAN_POINT('Ctrl Pts',(30.5041683224499,-16.5338357099673,-25.5487969550272));
#31332=CARTESIAN_POINT('Ctrl Pts',(31.5443819697417,-16.5215002939531,-25.5566068476798));
#31333=CARTESIAN_POINT('Ctrl Pts',(32.3694794643941,-16.4958953935747,-25.5729102090687));
#31334=CARTESIAN_POINT('Ctrl Pts',(33.1563754893963,-16.4960222658506,-25.5728296448089));
#31335=CARTESIAN_POINT('Ctrl Pts',(33.4912658278754,-16.4960347835491,-25.572821407314));
#31336=CARTESIAN_POINT('Ctrl Pts',(33.9824352992262,-16.4960613233721,-25.5728043629855));
#31337=CARTESIAN_POINT('Ctrl Pts',(34.4776280283123,-16.4960796138348,-25.5727925244551));
#31338=CARTESIAN_POINT('Ctrl Pts',(35.1357360035507,-16.4961042295225,-25.5727766538608));
#31339=CARTESIAN_POINT('Ctrl Pts',(35.9593379975622,-16.4961387987434,-25.5727543372373));
#31340=CARTESIAN_POINT('Ctrl Pts',(37.9345713338105,-16.4961741679457,-25.5727315175493));
#31341=CARTESIAN_POINT('Ctrl Pts',(39.5833333333333,-16.4963927771432,-25.5725904316243));
#31342=CARTESIAN_POINT('Ctrl Pts',(40.9,-16.4963927771432,-25.5725904316243));
#31343=CARTESIAN_POINT('Ctrl Pts',(6.37427268165564,3.85496595036637,-34.7583359408307));
#31344=CARTESIAN_POINT('Ctrl Pts',(6.46448755772838,3.66446375246399,-34.7802475524424));
#31345=CARTESIAN_POINT('Ctrl Pts',(6.55512331969025,3.47417181608893,-34.8005635888992));
#31346=CARTESIAN_POINT('Ctrl Pts',(7.61410548625795,1.26339052014804,-35.0185788676572));
#31347=CARTESIAN_POINT('Ctrl Pts',(8.61145388480624,-0.76560245720769,-35.0093532870147));
#31348=CARTESIAN_POINT('Ctrl Pts',(10.6635149436019,-4.43910992978125,-34.747974440135));
#31349=CARTESIAN_POINT('Ctrl Pts',(11.6608017032625,-6.13747453196185,-34.4619345886989));
#31350=CARTESIAN_POINT('Ctrl Pts',(13.7353542747945,-9.16685810272324,-33.7990269238398));
#31351=CARTESIAN_POINT('Ctrl Pts',(14.7402715202386,-10.526297955279,-33.3736740493576));
#31352=CARTESIAN_POINT('Ctrl Pts',(16.8491677832147,-12.9054531131771,-32.5473921410153));
#31353=CARTESIAN_POINT('Ctrl Pts',(17.8672809631136,-13.9382203331611,-32.092886041556));
#31354=CARTESIAN_POINT('Ctrl Pts',(19.2587625104673,-15.0707179501981,-31.577179869867));
#31355=CARTESIAN_POINT('Ctrl Pts',(19.7635899403542,-15.4658689812884,-31.3885503410944));
#31356=CARTESIAN_POINT('Ctrl Pts',(20.5586991602297,-16.0362969262867,-31.0991569516509));
#31357=CARTESIAN_POINT('Ctrl Pts',(21.3785272493018,-16.564533786793,-30.819343278526));
#31358=CARTESIAN_POINT('Ctrl Pts',(21.9479176287994,-16.8867906552356,-30.6451300260617));
#31359=CARTESIAN_POINT('Ctrl Pts',(22.3729695502115,-17.1090467735268,-30.525234440013));
#31360=CARTESIAN_POINT('Ctrl Pts',(22.6337096028248,-17.2413581349254,-30.45253373981));
#31361=CARTESIAN_POINT('Ctrl Pts',(23.1707519864209,-17.4975676797996,-30.3080867629256));
#31362=CARTESIAN_POINT('Ctrl Pts',(23.7186485394885,-17.7328951431605,-30.170626807131));
#31363=CARTESIAN_POINT('Ctrl Pts',(24.2804077704385,-17.946249160495,-30.0435395405948));
#31364=CARTESIAN_POINT('Ctrl Pts',(24.7075732751058,-18.0938968083019,-29.9548357769835));
#31365=CARTESIAN_POINT('Ctrl Pts',(25.0692008252975,-18.2061112471098,-29.8872739715487));
#31366=CARTESIAN_POINT('Ctrl Pts',(25.3613771492325,-18.28880476277,-29.8377189043884));
#31367=CARTESIAN_POINT('Ctrl Pts',(25.5084154817281,-18.3277015544066,-29.8145466170753));
#31368=CARTESIAN_POINT('Ctrl Pts',(26.1512870025444,-18.4915385207408,-29.7173716879777));
#31369=CARTESIAN_POINT('Ctrl Pts',(27.3223884400173,-18.6726738474942,-29.6052740416531));
#31370=CARTESIAN_POINT('Ctrl Pts',(28.3731396048321,-18.7409825767551,-29.559177524821));
#31371=CARTESIAN_POINT('Ctrl Pts',(28.9547046473315,-18.7836137746098,-29.5324480977279));
#31372=CARTESIAN_POINT('Ctrl Pts',(29.1479037067738,-18.7960320303041,-29.5247529606444));
#31373=CARTESIAN_POINT('Ctrl Pts',(29.5140802367921,-18.8132921881813,-29.51400582112));
#31374=CARTESIAN_POINT('Ctrl Pts',(29.9718311305158,-18.8248686377542,-29.5067996680497));
#31375=CARTESIAN_POINT('Ctrl Pts',(30.5051365276119,-18.8260067178222,-29.5060845192011));
#31376=CARTESIAN_POINT('Ctrl Pts',(31.551298475448,-18.8116639693829,-29.5150383037988));
#31377=CARTESIAN_POINT('Ctrl Pts',(32.3749555043413,-18.7822473977007,-29.5335081969199));
#31378=CARTESIAN_POINT('Ctrl Pts',(33.1551698865007,-18.7824304492383,-29.5333957726549));
#31379=CARTESIAN_POINT('Ctrl Pts',(33.4909201969602,-18.782448957068,-29.5333841560219));
#31380=CARTESIAN_POINT('Ctrl Pts',(33.981699427726,-18.7824875453788,-29.5333602907362));
#31381=CARTESIAN_POINT('Ctrl Pts',(34.4771077390558,-18.7825142819534,-29.533343676228));
#31382=CARTESIAN_POINT('Ctrl Pts',(35.1351798881798,-18.7825501686284,-29.5333214285967));
#31383=CARTESIAN_POINT('Ctrl Pts',(35.958882261465,-18.7826006107083,-29.5332901329543));
#31384=CARTESIAN_POINT('Ctrl Pts',(37.9341479260215,-18.7826521993715,-29.5332581373787));
#31385=CARTESIAN_POINT('Ctrl Pts',(39.5833333333333,-18.7829711232891,-29.5330603026358));
#31386=CARTESIAN_POINT('Ctrl Pts',(40.9,-18.7829711232891,-29.5330603026358));
#31387=CARTESIAN_POINT('',(40.9,-17.7819838375536,-27.7992994660114));
#31388=CARTESIAN_POINT('Ctrl Pts',(40.9,-17.7819838375536,-27.7992994660114));
#31389=CARTESIAN_POINT('Ctrl Pts',(40.9,-18.0322312401327,-28.2327406817405));
#31390=CARTESIAN_POINT('Ctrl Pts',(40.9,-18.2824786427117,-28.6661818974695));
#31391=CARTESIAN_POINT('Ctrl Pts',(40.9,-18.5327260452908,-29.0996231131986));
#31392=CARTESIAN_POINT('',(38.,-17.7819838375536,-27.7992994660114));
#31393=CARTESIAN_POINT('Ctrl Pts',(38.,-17.7819838375536,-27.7992994660114));
#31394=CARTESIAN_POINT('Ctrl Pts',(38.9666666666667,-17.7819838375536,-27.7992994660114));
#31395=CARTESIAN_POINT('Ctrl Pts',(39.9333333333333,-17.7819838375536,-27.7992994660114));
#31396=CARTESIAN_POINT('Ctrl Pts',(40.9,-17.7819838375536,-27.7992994660114));
#31397=CARTESIAN_POINT('Ctrl Pts',(37.4972421947179,-17.4814252073799,-27.2792895089189));
#31398=CARTESIAN_POINT('Ctrl Pts',(37.6643036200225,-17.5817077438358,-27.4529624980705));
#31399=CARTESIAN_POINT('Ctrl Pts',(37.8311445342373,-17.6818443698597,-27.6263779214721));
#31400=CARTESIAN_POINT('Ctrl Pts',(37.9976555467136,-17.7817739539416,-27.7994312893194));
#31401=CARTESIAN_POINT('',(6.9,2.26556458774883,-29.9143312995417));
#31402=CARTESIAN_POINT('Ctrl Pts',(6.9,2.26556458774883,-29.9143312995417));
#31403=CARTESIAN_POINT('Ctrl Pts',(6.9,2.00382962437802,-27.3056186709172));
#31404=CARTESIAN_POINT('Ctrl Pts',(6.90000000000115,1.73285728374608,-24.6693701926632));
#31405=CARTESIAN_POINT('Ctrl Pts',(6.90000000000115,1.09593289590079,-18.7182130985667));
#31406=CARTESIAN_POINT('Ctrl Pts',(6.9,0.654794893503688,-14.7845781982083));
#31407=CARTESIAN_POINT('Ctrl Pts',(6.9,0.168526548660244,-11.02768739857));
#31408=CARTESIAN_POINT('',(22.9245129145126,-15.8853026165582,-27.5141512254856));
#31409=CARTESIAN_POINT('Ctrl Pts',(22.9245129145126,-15.8853026165582,-27.5141512254856));
#31410=CARTESIAN_POINT('Ctrl Pts',(22.7202811020963,-15.7659233420327,-27.5032269692373));
#31411=CARTESIAN_POINT('Ctrl Pts',(22.5089075447093,-15.6398559109135,-27.4959054260063));
#31412=CARTESIAN_POINT('Ctrl Pts',(22.2913349439917,-15.5073965833875,-27.4928730439354));
#31413=CARTESIAN_POINT('Ctrl Pts',(21.445177058529,-14.9922512750188,-27.4810798586143));
#31414=CARTESIAN_POINT('Ctrl Pts',(20.5220951556664,-14.3509960808543,-27.5650257717265));
#31415=CARTESIAN_POINT('Ctrl Pts',(19.7671428819534,-13.785930418101,-27.676239960775));
#31416=CARTESIAN_POINT('Ctrl Pts',(19.5194773058388,-13.600558020691,-27.7127242885423));
#31417=CARTESIAN_POINT('Ctrl Pts',(19.2865716386089,-13.421872324025,-27.7514615171005));
#31418=CARTESIAN_POINT('Ctrl Pts',(19.0728538401323,-13.2552441975238,-27.7894004949774));
#31419=CARTESIAN_POINT('Ctrl Pts',(18.7028555998035,-12.9667697979459,-27.8550822264681));
#31420=CARTESIAN_POINT('Ctrl Pts',(18.4144703596236,-12.7292901983115,-27.9152561335183));
#31421=CARTESIAN_POINT('Ctrl Pts',(18.0642874871538,-12.4284122845047,-27.9946062155751));
#31422=CARTESIAN_POINT('Ctrl Pts',(17.4420927116721,-11.8938211301513,-28.1355931408966));
#31423=CARTESIAN_POINT('Ctrl Pts',(16.7224564418218,-11.2282910364348,-28.3254287038798));
#31424=CARTESIAN_POINT('Ctrl Pts',(15.9202806616111,-10.4246142212493,-28.5439924969395));
#31425=CARTESIAN_POINT('Ctrl Pts',(15.4090529834518,-9.91242993152957,-28.6832834892781));
#31426=CARTESIAN_POINT('Ctrl Pts',(14.8739602945714,-9.33532862360331,-28.8377564730262));
#31427=CARTESIAN_POINT('Ctrl Pts',(14.3169794331154,-8.6917184299937,-28.9944199787763));
#31428=CARTESIAN_POINT('Ctrl Pts',(13.8864206762836,-8.19419324731423,-29.1155243989539));
#31429=CARTESIAN_POINT('Ctrl Pts',(13.3867890027804,-7.59173852185132,-29.2546860278644));
#31430=CARTESIAN_POINT('Ctrl Pts',(12.8146824059514,-6.86770373383358,-29.3960736315876));
#31431=CARTESIAN_POINT('Ctrl Pts',(12.2526665517595,-6.15643937836578,-29.5349674589251));
#31432=CARTESIAN_POINT('Ctrl Pts',(11.6379478462803,-5.32066918438559,-29.678401911158));
#31433=CARTESIAN_POINT('Ctrl Pts',(10.9739250490308,-4.35448584003993,-29.7956367796097));
#31434=CARTESIAN_POINT('Ctrl Pts',(10.5683455447963,-3.76434923114268,-29.8672428449776));
#31435=CARTESIAN_POINT('Ctrl Pts',(10.1437415406956,-3.12422765605932,-29.9275397584159));
#31436=CARTESIAN_POINT('Ctrl Pts',(9.74137929176525,-2.50486371218385,-29.9670595377668));
#31437=CARTESIAN_POINT('Ctrl Pts',(8.72285779294234,-0.93703399130421,-30.0670981099855));
#31438=CARTESIAN_POINT('Ctrl Pts',(7.81323138778195,0.638451825302681,-30.0560666286387));
#31439=CARTESIAN_POINT('Ctrl Pts',(6.9,2.26556458774884,-29.9143312995417));
#31440=CARTESIAN_POINT('Ctrl Pts',(30.5,-18.8254200738635,-29.5059919176187));
#31441=CARTESIAN_POINT('Ctrl Pts',(29.9560179420816,-18.7064245513841,-29.293615660989));
#31442=CARTESIAN_POINT('Ctrl Pts',(29.4152668325132,-18.5734800115823,-29.0895919906434));
#31443=CARTESIAN_POINT('Ctrl Pts',(28.8740459957565,-18.4125151878636,-28.9020067835811));
#31444=CARTESIAN_POINT('Ctrl Pts',(28.353527792344,-18.2577075471291,-28.7215970352204));
#31445=CARTESIAN_POINT('Ctrl Pts',(27.8179515912466,-18.1008601332298,-28.533139934629));
#31446=CARTESIAN_POINT('Ctrl Pts',(27.2695051149491,-17.9186544331585,-28.3565719042575));
#31447=CARTESIAN_POINT('Ctrl Pts',(26.9554553615883,-17.8143203592948,-28.2554660556724));
#31448=CARTESIAN_POINT('Ctrl Pts',(26.6378099296971,-17.7019284120276,-28.1585101274348));
#31449=CARTESIAN_POINT('Ctrl Pts',(26.3179304017917,-17.5778023417279,-28.0701057587103));
#31450=CARTESIAN_POINT('Ctrl Pts',(26.1078196745982,-17.4962709631331,-28.012037940737));
#31451=CARTESIAN_POINT('Ctrl Pts',(25.8967402232745,-17.409683568055,-27.9576659729224));
#31452=CARTESIAN_POINT('Ctrl Pts',(25.6850706236774,-17.3169960819306,-27.9082593406129));
#31453=CARTESIAN_POINT('Ctrl Pts',(25.6562210027417,-17.3043631915899,-27.9015254373195));
#31454=CARTESIAN_POINT('Ctrl Pts',(25.6277737638215,-17.2918013331136,-27.8949772388532));
#31455=CARTESIAN_POINT('Ctrl Pts',(25.5983858063598,-17.2787081509674,-27.8883138877393));
#31456=CARTESIAN_POINT('Ctrl Pts',(25.1249357452756,-17.067772501732,-27.7809650188704));
#31457=CARTESIAN_POINT('Ctrl Pts',(24.1510084067019,-16.6022239440147,-27.5797558484168));
#31458=CARTESIAN_POINT('Ctrl Pts',(22.9245129145126,-15.8853026165582,-27.5141512254856));
#31459=CARTESIAN_POINT('Origin',(40.65,0.,0.));
#31460=CARTESIAN_POINT('',(40.4,1.49999999999999,-34.9678423698117));
#31461=CARTESIAN_POINT('',(40.9,1.49999999999999,-34.4673758792282));
#31462=CARTESIAN_POINT('Ctrl Pts',(40.4,1.49999999999999,-34.9678423698117));
#31463=CARTESIAN_POINT('Ctrl Pts',(40.5666590142087,1.49999999999999,-34.8010300902431));
#31464=CARTESIAN_POINT('Ctrl Pts',(40.733343045307,1.49999999999999,-34.6341905783528));
#31465=CARTESIAN_POINT('Ctrl Pts',(40.9,1.49999999999999,-34.4673758792282));
#31466=CARTESIAN_POINT('',(40.9,-1.50000000000002,-34.4673758792282));
#31467=CARTESIAN_POINT('Origin',(40.9,0.,0.));
#31468=CARTESIAN_POINT('',(40.4,-1.50000000000001,-34.9678423698117));
#31469=CARTESIAN_POINT('Ctrl Pts',(40.9,-1.50000000000001,-34.4673758792282));
#31470=CARTESIAN_POINT('Ctrl Pts',(40.7333430449637,-1.50000000000001,-34.6341905786964));
#31471=CARTESIAN_POINT('Ctrl Pts',(40.5666590137783,-1.50000000000001,-34.8010300906738));
#31472=CARTESIAN_POINT('Ctrl Pts',(40.4,-1.50000000000001,-34.9678423698117));
#31473=CARTESIAN_POINT('Origin',(40.4,0.,0.));
#31474=CARTESIAN_POINT('Origin',(35.7,0.,0.));
#31475=CARTESIAN_POINT('',(30.5,-1.55029606206997,-34.9656486014478));
#31476=CARTESIAN_POINT('Ctrl Pts',(40.3999915729117,-1.49999518538963,-34.9678423422331));
#31477=CARTESIAN_POINT('Ctrl Pts',(39.2499539542075,-1.49997392326491,-34.9678422204405));
#31478=CARTESIAN_POINT('Ctrl Pts',(38.0997984110589,-1.49988846741895,-34.9678417309291));
#31479=CARTESIAN_POINT('Ctrl Pts',(36.9496886126402,-1.49986523425637,-34.9678415977222));
#31480=CARTESIAN_POINT('Ctrl Pts',(36.7850895654027,-1.49986190922042,-34.9678415786582));
#31481=CARTESIAN_POINT('Ctrl Pts',(36.6204914551167,-1.49985985864023,-34.967841566892));
#31482=CARTESIAN_POINT('Ctrl Pts',(36.4559074066593,-1.49985712176039,-34.9678415512222));
#31483=CARTESIAN_POINT('Ctrl Pts',(36.4193481336993,-1.49985651381364,-34.9678415477415));
#31484=CARTESIAN_POINT('Ctrl Pts',(36.3827895545826,-1.49985587200327,-34.9678415440681));
#31485=CARTESIAN_POINT('Ctrl Pts',(36.3462314281453,-1.49985520449066,-34.9678415402484));
#31486=CARTESIAN_POINT('Ctrl Pts',(36.0893715793236,-1.49985051450228,-34.967841513411));
#31487=CARTESIAN_POINT('Ctrl Pts',(35.8498573424242,-1.49984503951475,-34.9678415998896));
#31488=CARTESIAN_POINT('Ctrl Pts',(35.6261955219287,-1.49984104357288,-34.967841744545));
#31489=CARTESIAN_POINT('Ctrl Pts',(35.5726950208743,-1.49984008773299,-34.9678417791469));
#31490=CARTESIAN_POINT('Ctrl Pts',(35.5201018010634,-1.49983920821971,-34.9678418170305));
#31491=CARTESIAN_POINT('Ctrl Pts',(35.4683958334514,-1.49983842183596,-34.9678418573607));
#31492=CARTESIAN_POINT('Ctrl Pts',(35.3126687160222,-1.4998360534193,-34.9678419788262));
#31493=CARTESIAN_POINT('Ctrl Pts',(35.1649944183664,-1.49983427390521,-34.9678421210274));
#31494=CARTESIAN_POINT('Ctrl Pts',(35.0249177028203,-1.49982884904642,-34.9678422344455));
#31495=CARTESIAN_POINT('Ctrl Pts',(35.0080273577823,-1.49982819492103,-34.9678422481214));
#31496=CARTESIAN_POINT('Ctrl Pts',(34.9912474154116,-1.49982749115044,-34.9678422613979));
#31497=CARTESIAN_POINT('Ctrl Pts',(34.9745770299108,-1.49982673292213,-34.967842274203));
#31498=CARTESIAN_POINT('Ctrl Pts',(34.8398252803349,-1.49982060393425,-34.9678423777109));
#31499=CARTESIAN_POINT('Ctrl Pts',(34.7122270228894,-1.49981110422879,-34.9678424514863));
#31500=CARTESIAN_POINT('Ctrl Pts',(34.5911971286586,-1.49980195022803,-34.9678424931048));
#31501=CARTESIAN_POINT('Ctrl Pts',(34.4536573923533,-1.49979154751836,-34.9678425404006));
#31502=CARTESIAN_POINT('Ctrl Pts',(34.324600768997,-1.49978157387808,-34.9678425460693));
#31503=CARTESIAN_POINT('Ctrl Pts',(34.2032402166286,-1.49977474411704,-34.9678424909992));
#31504=CARTESIAN_POINT('Ctrl Pts',(34.1282158883669,-1.49977052200182,-34.9678424569553));
#31505=CARTESIAN_POINT('Ctrl Pts',(34.0561340587984,-1.49976744984812,-34.9678423994066));
#31506=CARTESIAN_POINT('Ctrl Pts',(33.9868183126576,-1.49976579826338,-34.9678423117327));
#31507=CARTESIAN_POINT('Ctrl Pts',(33.9445485903809,-1.49976479110364,-34.967842258268));
#31508=CARTESIAN_POINT('Ctrl Pts',(33.9033113298609,-1.49976427568321,-34.9678421933981));
#31509=CARTESIAN_POINT('Ctrl Pts',(33.8632060391111,-1.49976308937533,-34.9678421088662));
#31510=CARTESIAN_POINT('Ctrl Pts',(33.8167294892623,-1.49976171460666,-34.9678420109052));
#31511=CARTESIAN_POINT('Ctrl Pts',(33.7717637484314,-1.49975949629186,-34.9678418868506));
#31512=CARTESIAN_POINT('Ctrl Pts',(33.7280832525525,-1.49975712824878,-34.9678417374965));
#31513=CARTESIAN_POINT('Ctrl Pts',(33.6812412750936,-1.49975458881285,-34.9678415773325));
#31514=CARTESIAN_POINT('Ctrl Pts',(33.6358775556469,-1.49975187629478,-34.9678413880696));
#31515=CARTESIAN_POINT('Ctrl Pts',(33.5917762634972,-1.49974959276977,-34.967841169348));
#31516=CARTESIAN_POINT('Ctrl Pts',(33.5583149104291,-1.49974786017117,-34.9678410033954));
#31517=CARTESIAN_POINT('Ctrl Pts',(33.5255817104614,-1.49974636887339,-34.967840820454));
#31518=CARTESIAN_POINT('Ctrl Pts',(33.4935021420768,-1.49974530120961,-34.9678406199406));
#31519=CARTESIAN_POINT('Ctrl Pts',(33.4573943589309,-1.49974409947985,-34.9678403942487));
#31520=CARTESIAN_POINT('Ctrl Pts',(33.4221208193067,-1.49974341134213,-34.9678401461735));
#31521=CARTESIAN_POINT('Ctrl Pts',(33.3878054439024,-1.49974262313064,-34.9678398702965));
#31522=CARTESIAN_POINT('Ctrl Pts',(33.3506623489709,-1.49974176996748,-34.9678395716863));
#31523=CARTESIAN_POINT('Ctrl Pts',(33.3146417056247,-1.49974080006053,-34.9678392405062));
#31524=CARTESIAN_POINT('Ctrl Pts',(33.2798370373775,-1.49973916665773,-34.9678388710955));
#31525=CARTESIAN_POINT('Ctrl Pts',(33.2432420311725,-1.49973744923335,-34.9678384826825));
#31526=CARTESIAN_POINT('Ctrl Pts',(33.2079907612227,-1.4997350003436,-34.9678380520153));
#31527=CARTESIAN_POINT('Ctrl Pts',(33.1741302661583,-1.49973140839958,-34.9678375736847));
#31528=CARTESIAN_POINT('Ctrl Pts',(33.1370268066149,-1.49972747243971,-34.9678370495424));
#31529=CARTESIAN_POINT('Ctrl Pts',(33.1015929393419,-1.49972216527192,-34.9678364681763));
#31530=CARTESIAN_POINT('Ctrl Pts',(33.067825091431,-1.49971518245857,-34.9678358237089));
#31531=CARTESIAN_POINT('Ctrl Pts',(33.0456190541537,-1.49971059049838,-34.9678353999014));
#31532=CARTESIAN_POINT('Ctrl Pts',(33.0241321462894,-1.49970527875611,-34.9678349488311));
#31533=CARTESIAN_POINT('Ctrl Pts',(33.00335138524,-1.49969920384722,-34.9678344690522));
#31534=CARTESIAN_POINT('Ctrl Pts',(32.9442304423539,-1.49968192082565,-34.9678331040887));
#31535=CARTESIAN_POINT('Ctrl Pts',(32.8886870683166,-1.49990565391071,-34.9678225550375));
#31536=CARTESIAN_POINT('Ctrl Pts',(32.8362378081004,-1.50026775301229,-34.9678066545694));
#31537=CARTESIAN_POINT('Ctrl Pts',(32.7772899725208,-1.50067471696594,-34.9677887839993));
#31538=CARTESIAN_POINT('Ctrl Pts',(32.722250704254,-1.50125685144361,-34.9677641385155));
#31539=CARTESIAN_POINT('Ctrl Pts',(32.6703984222899,-1.50192703269666,-34.9677359437545));
#31540=CARTESIAN_POINT('Ctrl Pts',(32.6144142271636,-1.50265061817099,-34.9677055022591));
#31541=CARTESIAN_POINT('Ctrl Pts',(32.5621451030132,-1.50347772465866,-34.9676708895142));
#31542=CARTESIAN_POINT('Ctrl Pts',(32.512643139679,-1.50435187710663,-34.9676341616883));
#31543=CARTESIAN_POINT('Ctrl Pts',(32.4592340800666,-1.5052950247529,-34.9675945350046));
#31544=CARTESIAN_POINT('Ctrl Pts',(32.4090461376418,-1.50629382208342,-34.9675524123823));
#31545=CARTESIAN_POINT('Ctrl Pts',(32.3608457191396,-1.50732223503495,-34.9675086930052));
#31546=CARTESIAN_POINT('Ctrl Pts',(32.3080489575157,-1.50844871640463,-34.9674608045926));
#31547=CARTESIAN_POINT('Ctrl Pts',(32.2576369811114,-1.50961152287641,-34.9674109699093));
#31548=CARTESIAN_POINT('Ctrl Pts',(32.2079387024057,-1.510814387538,-34.9673589596438));
#31549=CARTESIAN_POINT('Ctrl Pts',(32.1569651256412,-1.51204811868044,-34.9673056147528));
#31550=CARTESIAN_POINT('Ctrl Pts',(32.1067423359644,-1.51332494201266,-34.9672499447226));
#31551=CARTESIAN_POINT('Ctrl Pts',(32.0554173210335,-1.51467266340921,-34.9671908342291));
#31552=CARTESIAN_POINT('Ctrl Pts',(32.0053517019588,-1.515987314874,-34.9671331741689));
#31553=CARTESIAN_POINT('Ctrl Pts',(31.9542374237157,-1.51737028688898,-34.9670722073686));
#31554=CARTESIAN_POINT('Ctrl Pts',(31.9003072570603,-1.51885640484753,-34.9670065941482));
#31555=CARTESIAN_POINT('Ctrl Pts',(31.8778006425156,-1.51947660474927,-34.9669792118583));
#31556=CARTESIAN_POINT('Ctrl Pts',(31.8548030119451,-1.52011480778718,-34.9669510193556));
#31557=CARTESIAN_POINT('Ctrl Pts',(31.8311831714798,-1.52077345952528,-34.966921924937));
#31558=CARTESIAN_POINT('Ctrl Pts',(31.7273359798822,-1.52366929336221,-34.9667940081687));
#31559=CARTESIAN_POINT('Ctrl Pts',(31.6209566880911,-1.52669736830073,-34.9666588995974));
#31560=CARTESIAN_POINT('Ctrl Pts',(31.5128850686401,-1.52967035112202,-34.966525984972));
#31561=CARTESIAN_POINT('Ctrl Pts',(31.4048094944667,-1.53264344273527,-34.9663930654827));
#31562=CARTESIAN_POINT('Ctrl Pts',(31.2950411944129,-1.5355595885407,-34.9662624112288));
#31563=CARTESIAN_POINT('Ctrl Pts',(31.1844688435936,-1.53821966510477,-34.9661438178107));
#31564=CARTESIAN_POINT('Ctrl Pts',(31.1320862054071,-1.53947985200658,-34.9660876352654));
#31565=CARTESIAN_POINT('Ctrl Pts',(31.0795238479782,-1.54068257273422,-34.9660341587666));
#31566=CARTESIAN_POINT('Ctrl Pts',(31.0268803009881,-1.5418076100978,-34.9659843897334));
#31567=CARTESIAN_POINT('Ctrl Pts',(30.9324572739831,-1.54382551047565,-34.9658951225195));
#31568=CARTESIAN_POINT('Ctrl Pts',(30.837770831616,-1.54559180591447,-34.9658178374821));
#31569=CARTESIAN_POINT('Ctrl Pts',(30.7433264837577,-1.54696313276377,-34.9657578054117));
#31570=CARTESIAN_POINT('Ctrl Pts',(30.6607858411442,-1.5481616184534,-34.9657053397451));
#31571=CARTESIAN_POINT('Ctrl Pts',(30.5784303320586,-1.54905826480272,-34.965666053989));
#31572=CARTESIAN_POINT('Ctrl Pts',(30.4966228217932,-1.54957830485528,-34.965642796755));
#31573=CARTESIAN_POINT('',(30.5,1.44976976333441,-34.9699609326822));
#31574=CARTESIAN_POINT('Origin',(30.5,0.,0.));
#31575=CARTESIAN_POINT('Ctrl Pts',(30.5051992612603,1.44903843638966,-34.9699071381489));
#31576=CARTESIAN_POINT('Ctrl Pts',(30.6030952980657,1.44976082626916,-34.9698787568566));
#31577=CARTESIAN_POINT('Ctrl Pts',(30.7001121880333,1.45104998650339,-34.9698264221104));
#31578=CARTESIAN_POINT('Ctrl Pts',(30.7969947619801,1.45274237549662,-34.9697577270266));
#31579=CARTESIAN_POINT('Ctrl Pts',(30.8545454823775,1.45374769773142,-34.9697169203944));
#31580=CARTESIAN_POINT('Ctrl Pts',(30.9120492097055,1.45489634227782,-34.9696702850816));
#31581=CARTESIAN_POINT('Ctrl Pts',(30.9696671110348,1.45616096255286,-34.9696190483589));
#31582=CARTESIAN_POINT('Ctrl Pts',(31.0687356284601,1.45833535719175,-34.969530951673));
#31583=CARTESIAN_POINT('Ctrl Pts',(31.1681385828748,1.46085179879274,-34.9694292858245));
#31584=CARTESIAN_POINT('Ctrl Pts',(31.2685908593294,1.46356721252908,-34.9693191238307));
#31585=CARTESIAN_POINT('Ctrl Pts',(31.3711796386319,1.46634037995092,-34.9692066188196));
#31586=CARTESIAN_POINT('Ctrl Pts',(31.4748629185106,1.46932276608705,-34.9690851710714));
#31587=CARTESIAN_POINT('Ctrl Pts',(31.5804543970555,1.4723695155306,-34.9689598486836));
#31588=CARTESIAN_POINT('Ctrl Pts',(31.6427002532174,1.47416556508155,-34.9688859715162));
#31589=CARTESIAN_POINT('Ctrl Pts',(31.7056101943812,1.47598400420447,-34.9688107472906));
#31590=CARTESIAN_POINT('Ctrl Pts',(31.7693590594471,1.4777925610394,-34.9687353433411));
#31591=CARTESIAN_POINT('Ctrl Pts',(31.8369567664635,1.47971030961302,-34.968655386873));
#31592=CARTESIAN_POINT('Ctrl Pts',(31.8998289473023,1.48145356148269,-34.9685826953725));
#31593=CARTESIAN_POINT('Ctrl Pts',(31.9584912820088,1.48302365833457,-34.9685172658125));
#31594=CARTESIAN_POINT('Ctrl Pts',(32.0219681801223,1.484722616932,-34.9684464662861));
#31595=CARTESIAN_POINT('Ctrl Pts',(32.0805160965733,1.48621979971339,-34.9683841232145));
#31596=CARTESIAN_POINT('Ctrl Pts',(32.1348442130202,1.48754049944246,-34.9683291276834));
#31597=CARTESIAN_POINT('Ctrl Pts',(32.1955320114797,1.48901580107678,-34.9682676943422));
#31598=CARTESIAN_POINT('Ctrl Pts',(32.2509543450015,1.49027186778442,-34.9682153821449));
#31599=CARTESIAN_POINT('Ctrl Pts',(32.3021641802418,1.49135570584798,-34.968170114115));
#31600=CARTESIAN_POINT('Ctrl Pts',(32.3568725417847,1.49251358898424,-34.9681217534879));
#31601=CARTESIAN_POINT('Ctrl Pts',(32.4067738547306,1.49347579219526,-34.9680813901956));
#31602=CARTESIAN_POINT('Ctrl Pts',(32.453214342574,1.4942964704374,-34.9680466762592));
#31603=CARTESIAN_POINT('Ctrl Pts',(32.5024778890101,1.49516703667321,-34.9680098521065));
#31604=CARTESIAN_POINT('Ctrl Pts',(32.5478477692433,1.49587895592537,-34.9679793561973));
#31605=CARTESIAN_POINT('Ctrl Pts',(32.5909873019015,1.49648137333635,-34.9679531603256));
#31606=CARTESIAN_POINT('Ctrl Pts',(32.6362425762323,1.49711333579668,-34.9679256796997));
#31607=CARTESIAN_POINT('Ctrl Pts',(32.6790438910161,1.49762527612468,-34.9679029082457));
#31608=CARTESIAN_POINT('Ctrl Pts',(32.7213614276283,1.49804900699202,-34.9678837287556));
#31609=CARTESIAN_POINT('Ctrl Pts',(32.7633326545664,1.49846927021662,-34.9678647062226));
#31610=CARTESIAN_POINT('Ctrl Pts',(32.8048283340736,1.49880319667879,-34.9678491963778));
#31611=CARTESIAN_POINT('Ctrl Pts',(32.8478112859666,1.49905168880696,-34.9678375791942));
#31612=CARTESIAN_POINT('Ctrl Pts',(32.8880595868492,1.49928437142881,-34.9678267011162));
#31613=CARTESIAN_POINT('Ctrl Pts',(32.9296120625659,1.49944259954574,-34.9678192143482));
#31614=CARTESIAN_POINT('Ctrl Pts',(32.9741124736877,1.49949475964765,-34.9678170031323));
#31615=CARTESIAN_POINT('Ctrl Pts',(32.9824658917628,1.49950455090861,-34.9678165880527));
#31616=CARTESIAN_POINT('Ctrl Pts',(32.9909232824633,1.49951049395371,-34.9678163642396));
#31617=CARTESIAN_POINT('Ctrl Pts',(32.9994956564547,1.4995122138931,-34.9678163521983));
#31618=CARTESIAN_POINT('Ctrl Pts',(33.035916707601,1.49951952132052,-34.9678163010392));
#31619=CARTESIAN_POINT('Ctrl Pts',(33.0737648470631,1.49952600456097,-34.9678163144541));
#31620=CARTESIAN_POINT('Ctrl Pts',(33.1138039348094,1.49953164904712,-34.9678165569182));
#31621=CARTESIAN_POINT('Ctrl Pts',(33.2457861392315,1.49955025515845,-34.9678173561608));
#31622=CARTESIAN_POINT('Ctrl Pts',(33.3718058092168,1.49955552940342,-34.9678177616075));
#31623=CARTESIAN_POINT('Ctrl Pts',(33.4990121011459,1.49956083536767,-34.9678181023247));
#31624=CARTESIAN_POINT('Ctrl Pts',(33.6624238693915,1.49956765151637,-34.9678185400169));
#31625=CARTESIAN_POINT('Ctrl Pts',(33.8277938592881,1.49957452000976,-34.9678188708891));
#31626=CARTESIAN_POINT('Ctrl Pts',(33.9926457806311,1.49958605843696,-34.9678194856962));
#31627=CARTESIAN_POINT('Ctrl Pts',(34.322349623317,1.49960913529134,-34.9678207153104));
#31628=CARTESIAN_POINT('Ctrl Pts',(34.649981191788,1.49965089188093,-34.9678230806641));
#31629=CARTESIAN_POINT('Ctrl Pts',(34.978743760729,1.499668413021,-34.9678240597269));
#31630=CARTESIAN_POINT('Ctrl Pts',(35.1431250451995,1.49967717359104,-34.9678245492582));
#31631=CARTESIAN_POINT('Ctrl Pts',(35.3077890797876,1.49967987529869,-34.9678246922169));
#31632=CARTESIAN_POINT('Ctrl Pts',(35.4723919953983,1.49968390458378,-34.9678249110675));
#31633=CARTESIAN_POINT('Ctrl Pts',(35.9662007422305,1.49969599243904,-34.9678255676192));
#31634=CARTESIAN_POINT('Ctrl Pts',(36.4594594182669,1.49972002849122,-34.9678269071982));
#31635=CARTESIAN_POINT('Ctrl Pts',(36.9527108273738,1.49975356610212,-34.9678287658476));
#31636=CARTESIAN_POINT('Ctrl Pts',(38.1015495523822,1.49983167901863,-34.9678330948538));
#31637=CARTESIAN_POINT('Ctrl Pts',(39.2503488559568,1.49996133572171,-34.9678402396984));
#31638=CARTESIAN_POINT('Ctrl Pts',(40.4000634893725,1.49999290859452,-34.9678419791559));
#31639=CARTESIAN_POINT('Ctrl Pts',(6.89999999997365,5.65979197164529,-9.46599415780712));
#31640=CARTESIAN_POINT('Ctrl Pts',(6.99168932310453,5.60729410195164,-9.49787619923353));
#31641=CARTESIAN_POINT('Ctrl Pts',(7.08406757664724,5.55450348934908,-9.52934743218563));
#31642=CARTESIAN_POINT('Ctrl Pts',(8.15335547176687,4.94393526084759,-9.88612718871467));
#31643=CARTESIAN_POINT('Ctrl Pts',(9.17064157978095,4.34950511965197,-10.155373368134));
#31644=CARTESIAN_POINT('Ctrl Pts',(11.2497073679685,3.24768323904103,-10.5680733268196));
#31645=CARTESIAN_POINT('Ctrl Pts',(12.2613257965134,2.71507134816794,-10.7096965195797));
#31646=CARTESIAN_POINT('Ctrl Pts',(14.3530385707896,1.75090834575261,-10.9182697262449));
#31647=CARTESIAN_POINT('Ctrl Pts',(15.3683954027039,1.30024059461546,-10.9736607960856));
#31648=CARTESIAN_POINT('Ctrl Pts',(17.4699663744738,0.511601148556842,-11.0479352514981));
#31649=CARTESIAN_POINT('Ctrl Pts',(18.4899687408706,0.154958649018866,-11.051850654124));
#31650=CARTESIAN_POINT('Ctrl Pts',(19.8459543561021,-0.227742125737042,
-11.0525070343707));
#31651=CARTESIAN_POINT('Ctrl Pts',(20.3436217075759,-0.364015941931448,
-11.0499451453311));
#31652=CARTESIAN_POINT('Ctrl Pts',(21.3765896493641,-0.626368709758944,
-11.0391193472025));
#31653=CARTESIAN_POINT('Ctrl Pts',(22.1786672894955,-0.801485129181549,
-11.0271785661492));
#31654=CARTESIAN_POINT('Ctrl Pts',(22.8524865110786,-0.927592368920619,
-11.0190187727781));
#31655=CARTESIAN_POINT('Ctrl Pts',(23.1034925219802,-0.973363366151912,
-11.0156366139706));
#31656=CARTESIAN_POINT('Ctrl Pts',(23.6153640104269,-1.06158199416384,-11.0082049867405));
#31657=CARTESIAN_POINT('Ctrl Pts',(24.2641052830132,-1.16309769090629,-10.9980910304789));
#31658=CARTESIAN_POINT('Ctrl Pts',(24.925223802488,-1.25113068226714,-10.9882977299783));
#31659=CARTESIAN_POINT('Ctrl Pts',(25.39243267008,-1.30426326836546,-10.9823394091471));
#31660=CARTESIAN_POINT('Ctrl Pts',(25.6607214646257,-1.33204812136028,-10.9792978116211));
#31661=CARTESIAN_POINT('Ctrl Pts',(25.7950851290472,-1.3450283872937,-10.9779152492989));
#31662=CARTESIAN_POINT('Ctrl Pts',(26.2512983640655,-1.38748632823361,-10.973504884093));
#31663=CARTESIAN_POINT('Ctrl Pts',(27.3073255991507,-1.45732001035815,-10.9653766251364));
#31664=CARTESIAN_POINT('Ctrl Pts',(28.3319095891359,-1.48237652410472,-10.9609947927216));
#31665=CARTESIAN_POINT('Ctrl Pts',(29.1279971548665,-1.50394615286608,-10.9582093263721));
#31666=CARTESIAN_POINT('Ctrl Pts',(29.4779663121082,-1.51103862156505,-10.9573325432847));
#31667=CARTESIAN_POINT('Ctrl Pts',(29.9466432965585,-1.51533372194798,-10.9567800734979));
#31668=CARTESIAN_POINT('Ctrl Pts',(30.4585813758454,-1.5163264007104,-10.9566567573898));
#31669=CARTESIAN_POINT('Ctrl Pts',(31.4732365826137,-1.51158267548692,-10.9572595410787));
#31670=CARTESIAN_POINT('Ctrl Pts',(32.3455737970013,-1.49995034482797,-10.9587933809202));
#31671=CARTESIAN_POINT('Ctrl Pts',(33.1628435364506,-1.49997381799307,-10.9587933913798));
#31672=CARTESIAN_POINT('Ctrl Pts',(33.4532364756742,-1.49997294893161,-10.9587933907408));
#31673=CARTESIAN_POINT('Ctrl Pts',(33.7813770806023,-1.49997567748037,-10.9587933918753));
#31674=CARTESIAN_POINT('Ctrl Pts',(34.275530783599,-1.49997630771875,-10.9587933920503));
#31675=CARTESIAN_POINT('Ctrl Pts',(34.810224248481,-1.49998265426638,-10.9587933943926));
#31676=CARTESIAN_POINT('Ctrl Pts',(35.6332393788981,-1.49998352671605,-10.9587933946975));
#31677=CARTESIAN_POINT('Ctrl Pts',(36.2915395642402,-1.49998521165682,-10.9587933953165));
#31678=CARTESIAN_POINT('Ctrl Pts',(38.1020088507064,-1.4999875244666,-10.9587933961529));
#31679=CARTESIAN_POINT('Ctrl Pts',(39.5833333333333,-1.5,-10.9587934006931));
#31680=CARTESIAN_POINT('Ctrl Pts',(40.9,-1.5,-10.9587934006931));
#31681=CARTESIAN_POINT('Ctrl Pts',(6.71972576838711,7.83711082411041,-12.1185747411757));
#31682=CARTESIAN_POINT('Ctrl Pts',(6.81144220747046,7.76982141889617,-12.1626853346856));
#31683=CARTESIAN_POINT('Ctrl Pts',(6.90386756592035,7.70211146561914,-12.206272355858));
#31684=CARTESIAN_POINT('Ctrl Pts',(7.97356860844392,6.9193341478531,-12.7007961961294));
#31685=CARTESIAN_POINT('Ctrl Pts',(8.99209675135677,6.15357612800253,-13.0797453577275));
#31686=CARTESIAN_POINT('Ctrl Pts',(11.0768095250715,4.72738288403858,-13.6699841865111));
#31687=CARTESIAN_POINT('Ctrl Pts',(12.0908998487774,4.03629416338865,-13.8792353432569));
#31688=CARTESIAN_POINT('Ctrl Pts',(14.1940249697802,2.77872196480346,-14.1957933847446));
#31689=CARTESIAN_POINT('Ctrl Pts',(15.2135111428103,2.19039552953479,-14.2882641966348));
#31690=CARTESIAN_POINT('Ctrl Pts',(17.3331413243803,1.15511424931918,-14.4203884130587));
#31691=CARTESIAN_POINT('Ctrl Pts',(18.3586247182578,0.687383264604317,-14.4409834784055));
#31692=CARTESIAN_POINT('Ctrl Pts',(19.7310977064191,0.182163287151178,-14.4582431367918));
#31693=CARTESIAN_POINT('Ctrl Pts',(20.2319281700692,0.00304050314957347,
-14.4607525000525));
#31694=CARTESIAN_POINT('Ctrl Pts',(21.2757193631683,-0.34316184167988,-14.4577287725711));
#31695=CARTESIAN_POINT('Ctrl Pts',(22.0878459668371,-0.574768167050975,
-14.4494235361695));
#31696=CARTESIAN_POINT('Ctrl Pts',(22.7712255558999,-0.741838037544796,
-14.4439791152719));
#31697=CARTESIAN_POINT('Ctrl Pts',(23.0244518575534,-0.802235623376846,
-14.4414745946824));
#31698=CARTESIAN_POINT('Ctrl Pts',(23.5421782294103,-0.918904682189656,
-14.4354166159132));
#31699=CARTESIAN_POINT('Ctrl Pts',(24.1985076923264,-1.05321891221311,-14.4263782772875));
#31700=CARTESIAN_POINT('Ctrl Pts',(24.8685349201902,-1.16990126309174,-14.4171649757332));
#31701=CARTESIAN_POINT('Ctrl Pts',(25.3425219397605,-1.24038895116693,-14.4115304423973));
#31702=CARTESIAN_POINT('Ctrl Pts',(25.6149132395532,-1.2772755062893,-14.4086772259669));
#31703=CARTESIAN_POINT('Ctrl Pts',(25.751350411375,-1.29451009974022,-14.4073941370215));
#31704=CARTESIAN_POINT('Ctrl Pts',(26.2150797233484,-1.35093461898509,-14.4033369558708));
#31705=CARTESIAN_POINT('Ctrl Pts',(27.290210767141,-1.44377946037276,-14.3955032503722));
#31706=CARTESIAN_POINT('Ctrl Pts',(28.3189127523345,-1.47663174833176,-14.3908275896983));
#31707=CARTESIAN_POINT('Ctrl Pts',(29.1160761436634,-1.50501177720119,-14.3880866255979));
#31708=CARTESIAN_POINT('Ctrl Pts',(29.4714822396865,-1.51444018285273,-14.3872233428149));
#31709=CARTESIAN_POINT('Ctrl Pts',(29.9435445757052,-1.5200984593836,-14.3866793881694));
#31710=CARTESIAN_POINT('Ctrl Pts',(30.4592512763238,-1.52141685888082,-14.3865579372846));
#31711=CARTESIAN_POINT('Ctrl Pts',(31.4783289771153,-1.51514975878901,-14.3871513993674));
#31712=CARTESIAN_POINT('Ctrl Pts',(32.3494109418822,-1.49991854815768,-14.3886610620144));
#31713=CARTESIAN_POINT('Ctrl Pts',(33.1623024290964,-1.49995704732011,-14.3886610002152));
#31714=CARTESIAN_POINT('Ctrl Pts',(33.4534378485101,-1.49995562308142,-14.3886610012865));
#31715=CARTESIAN_POINT('Ctrl Pts',(33.7812569880683,-1.49996009863815,-14.3886609937099));
#31716=CARTESIAN_POINT('Ctrl Pts',(34.2755369516761,-1.49996113279295,-14.3886609915395));
#31717=CARTESIAN_POINT('Ctrl Pts',(34.8101662657421,-1.49997154418691,-14.3886609724833));
#31718=CARTESIAN_POINT('Ctrl Pts',(35.6332120986579,-1.49997297550203,-14.3886609697809));
#31719=CARTESIAN_POINT('Ctrl Pts',(36.2915016928915,-1.49997573962884,-14.3886609647081));
#31720=CARTESIAN_POINT('Ctrl Pts',(38.1019871489809,-1.49997953382812,-14.3886609576808));
#31721=CARTESIAN_POINT('Ctrl Pts',(39.5833333333333,-1.5,-14.3886609199119));
#31722=CARTESIAN_POINT('Ctrl Pts',(40.9,-1.5,-14.3886609199119));
#31723=CARTESIAN_POINT('Ctrl Pts',(6.48179127333656,12.909089854674,-18.3143700731402));
#31724=CARTESIAN_POINT('Ctrl Pts',(6.5727355112717,12.8079669208388,-18.3863503069792));
#31725=CARTESIAN_POINT('Ctrl Pts',(6.66430583051619,12.7062136474361,-18.4575107126117));
#31726=CARTESIAN_POINT('Ctrl Pts',(7.72728755127275,11.526813643454,-19.2683717061286));
#31727=CARTESIAN_POINT('Ctrl Pts',(8.73767093241514,10.3681062987579,-19.8994793964433));
#31728=CARTESIAN_POINT('Ctrl Pts',(10.8072764746652,8.20052377414071,-20.8976754072823));
#31729=CARTESIAN_POINT('Ctrl Pts',(11.8176293289991,7.14335535654034,-21.2648595585571));
#31730=CARTESIAN_POINT('Ctrl Pts',(13.9143877357634,5.21126000157089,-21.8327192432693));
#31731=CARTESIAN_POINT('Ctrl Pts',(14.9340995606326,4.30265046255494,-22.0133279182349));
#31732=CARTESIAN_POINT('Ctrl Pts',(17.0643846051769,2.69212316987972,-22.28293018524));
#31733=CARTESIAN_POINT('Ctrl Pts',(18.0954552433595,1.9632331485467,-22.3440950085561));
#31734=CARTESIAN_POINT('Ctrl Pts',(19.4909197138958,1.16629947063494,-22.4018170797765));
#31735=CARTESIAN_POINT('Ctrl Pts',(19.9966086695085,0.886002865969556,-22.4166274395865));
#31736=CARTESIAN_POINT('Ctrl Pts',(21.057536308733,0.34008676046798,-22.4327717472399));
#31737=CARTESIAN_POINT('Ctrl Pts',(21.8881436826395,-0.0273249680472169,
-22.4335301553629));
#31738=CARTESIAN_POINT('Ctrl Pts',(22.5903109281612,-0.293403230880334,
-22.4347813300338));
#31739=CARTESIAN_POINT('Ctrl Pts',(22.8479490471753,-0.388703666414858,
-22.4344227430831));
#31740=CARTESIAN_POINT('Ctrl Pts',(23.3775020106794,-0.573741554000536,
-22.4317625870076));
#31741=CARTESIAN_POINT('Ctrl Pts',(24.0496637775493,-0.786975429601204,
-22.4254188817567));
#31742=CARTESIAN_POINT('Ctrl Pts',(24.7388948303246,-0.97298069201505,-22.4176871558595));
#31743=CARTESIAN_POINT('Ctrl Pts',(25.2278255076836,-1.08558489693713,-22.4128668811674));
#31744=CARTESIAN_POINT('Ctrl Pts',(25.5093513414538,-1.14461019857633,-22.4104803100082));
#31745=CARTESIAN_POINT('Ctrl Pts',(25.65043215624,-1.17219731393412,-22.4094403330887));
#31746=CARTESIAN_POINT('Ctrl Pts',(26.1310661693221,-1.26270961274929,-22.4062434753127));
#31747=CARTESIAN_POINT('Ctrl Pts',(27.2501415560404,-1.41179466704418,-22.3991278521003));
#31748=CARTESIAN_POINT('Ctrl Pts',(28.2886032423041,-1.46273606147739,-22.3937640305132));
#31749=CARTESIAN_POINT('Ctrl Pts',(29.0882604747173,-1.50713395382423,-22.3911301380753));
#31750=CARTESIAN_POINT('Ctrl Pts',(29.4563322715989,-1.52226638583168,-22.3902983022162));
#31751=CARTESIAN_POINT('Ctrl Pts',(29.9362980190428,-1.53114557872188,-22.3897746111047));
#31752=CARTESIAN_POINT('Ctrl Pts',(30.4607981263299,-1.53325643249715,-22.3896576468515));
#31753=CARTESIAN_POINT('Ctrl Pts',(31.4901962393228,-1.52335038033792,-22.3902297218138));
#31754=CARTESIAN_POINT('Ctrl Pts',(32.3583565740134,-1.49981123516845,-22.3916842973338));
#31755=CARTESIAN_POINT('Ctrl Pts',(33.1610357599842,-1.49990048269241,-22.3916846791414));
#31756=CARTESIAN_POINT('Ctrl Pts',(33.4539035041348,-1.49989717526718,-22.3916846678314));
#31757=CARTESIAN_POINT('Ctrl Pts',(33.7809729803152,-1.49990754848558,-22.3916847131259));
#31758=CARTESIAN_POINT('Ctrl Pts',(34.2755476513316,-1.49990994339324,-22.3916847245643));
#31759=CARTESIAN_POINT('Ctrl Pts',(34.8100282687525,-1.49993406756257,-22.3916848332468));
#31760=CARTESIAN_POINT('Ctrl Pts',(35.6331458770731,-1.49993738365807,-22.3916848483796));
#31761=CARTESIAN_POINT('Ctrl Pts',(36.2914110212366,-1.49994378833294,-22.391684877265));
#31762=CARTESIAN_POINT('Ctrl Pts',(38.1019345670508,-1.49995257945083,-22.3916849170636));
#31763=CARTESIAN_POINT('Ctrl Pts',(39.5833333333333,-1.5,-22.3916851314225));
#31764=CARTESIAN_POINT('Ctrl Pts',(40.9,-1.5,-22.3916851314225));
#31765=CARTESIAN_POINT('Ctrl Pts',(6.40644620858992,17.8874643710144,-24.5816667734855));
#31766=CARTESIAN_POINT('Ctrl Pts',(6.49686818484384,17.7527429476115,-24.6805587856898));
#31767=CARTESIAN_POINT('Ctrl Pts',(6.58784510136317,17.6172881830822,-24.7782796712625));
#31768=CARTESIAN_POINT('Ctrl Pts',(7.64659115698292,16.0421679652612,-25.8957117993605));
#31769=CARTESIAN_POINT('Ctrl Pts',(8.6514045236879,14.4950741541975,-26.7687295114656));
#31770=CARTESIAN_POINT('Ctrl Pts',(10.7050090174743,11.6047165303877,-28.1553288871656));
#31771=CARTESIAN_POINT('Ctrl Pts',(11.7100667319376,10.1884238311836,-28.6739187260774));
#31772=CARTESIAN_POINT('Ctrl Pts',(13.7869442940535,7.60965076371051,-29.4789383477456));
#31773=CARTESIAN_POINT('Ctrl Pts',(14.800547377598,6.38969931376494,-29.7443143884371));
#31774=CARTESIAN_POINT('Ctrl Pts',(16.9119018452747,4.23153286849663,-30.1445946231782));
#31775=CARTESIAN_POINT('Ctrl Pts',(17.9381035625226,3.24834169632011,-30.2457831733189));
#31776=CARTESIAN_POINT('Ctrl Pts',(19.3293046497141,2.1696711131215,-30.3432573890378));
#31777=CARTESIAN_POINT('Ctrl Pts',(19.834780983011,1.78946315727512,-30.3704921110681));
#31778=CARTESIAN_POINT('Ctrl Pts',(20.8961305093701,1.0472327615649,-30.4059869321106));
#31779=CARTESIAN_POINT('Ctrl Pts',(21.7315172578668,0.543887046860907,-30.4162256374442));
#31780=CARTESIAN_POINT('Ctrl Pts',(22.4417821405951,0.177022257580511,-30.4244987232164));
#31781=CARTESIAN_POINT('Ctrl Pts',(22.7014733500986,0.0463161543317088,
-30.4263999272521));
#31782=CARTESIAN_POINT('Ctrl Pts',(23.2370081907225,-0.208619908910742,
-30.4273647052435));
#31783=CARTESIAN_POINT('Ctrl Pts',(23.9184639528738,-0.503259137524155,
-30.4239702414859));
#31784=CARTESIAN_POINT('Ctrl Pts',(24.6208764942963,-0.761940486000404,
-30.4179198546273));
#31785=CARTESIAN_POINT('Ctrl Pts',(25.1213019205202,-0.91928494098934,-30.4140183351927));
#31786=CARTESIAN_POINT('Ctrl Pts',(25.4101854930952,-1.00200491165304,-30.4121479536513));
#31787=CARTESIAN_POINT('Ctrl Pts',(25.5551212201431,-1.04071255367786,-30.4113724623503));
#31788=CARTESIAN_POINT('Ctrl Pts',(26.0499700309764,-1.16807884822144,-30.4091032350971));
#31789=CARTESIAN_POINT('Ctrl Pts',(27.2099838300809,-1.37887073252529,-30.4027650251877));
#31790=CARTESIAN_POINT('Ctrl Pts',(28.2587071867247,-1.44776855241709,-30.3967001628547));
#31791=CARTESIAN_POINT('Ctrl Pts',(29.0606747532772,-1.50844446424265,-30.3941758184157));
#31792=CARTESIAN_POINT('Ctrl Pts',(29.4413133039643,-1.52986784607282,-30.3933750220959));
#31793=CARTESIAN_POINT('Ctrl Pts',(29.9291749316176,-1.54205805667022,-30.3928713041225));
#31794=CARTESIAN_POINT('Ctrl Pts',(30.4624577144424,-1.54503525729536,-30.3927586652121));
#31795=CARTESIAN_POINT('Ctrl Pts',(31.5021663454747,-1.53129124555949,-30.3933094956308));
#31796=CARTESIAN_POINT('Ctrl Pts',(32.3673500494201,-1.4996392507279,-30.3947081079589));
#31797=CARTESIAN_POINT('Ctrl Pts',(33.1597959712394,-1.49981015578451,-30.394708675703));
#31798=CARTESIAN_POINT('Ctrl Pts',(33.4543964419649,-1.49980374442732,-30.3947086583173));
#31799=CARTESIAN_POINT('Ctrl Pts',(33.780713697117,-1.49982358355628,-30.3947087254864));
#31800=CARTESIAN_POINT('Ctrl Pts',(34.2755823554681,-1.49982813702183,-30.3947087422566));
#31801=CARTESIAN_POINT('Ctrl Pts',(34.809907886371,-1.49987418368373,-30.3947089027709));
#31802=CARTESIAN_POINT('Ctrl Pts',(35.6330963662039,-1.49988050793533,-30.3947089250841));
#31803=CARTESIAN_POINT('Ctrl Pts',(36.2913353597009,-1.49989273190318,-30.3947089677392));
#31804=CARTESIAN_POINT('Ctrl Pts',(38.1018946411375,-1.49990950652165,-30.3947090264815));
#31805=CARTESIAN_POINT('Ctrl Pts',(39.5833333333333,-1.50000000000001,-30.3947093429332));
#31806=CARTESIAN_POINT('Ctrl Pts',(40.9,-1.50000000000001,-30.3947093429332));
#31807=CARTESIAN_POINT('Ctrl Pts',(6.37427268165564,20.7176664141567,-28.1741189428499));
#31808=CARTESIAN_POINT('Ctrl Pts',(6.46448755772839,20.5636424771022,-28.2883460540946));
#31809=CARTESIAN_POINT('Ctrl Pts',(6.55522920065044,20.4088241438424,-28.4012016037216));
#31810=CARTESIAN_POINT('Ctrl Pts',(7.61218358683609,18.6066930771539,-29.6930901664144));
#31811=CARTESIAN_POINT('Ctrl Pts',(8.61458966533695,16.8369834746305,-30.7034878418583));
#31812=CARTESIAN_POINT('Ctrl Pts',(10.6617286949536,13.5326707735154,-32.3103185106199));
#31813=CARTESIAN_POINT('Ctrl Pts',(11.6645299641072,11.9110262048008,-32.9144286242224));
#31814=CARTESIAN_POINT('Ctrl Pts',(13.7331354874437,8.96388086964109,-33.8529305432337));
#31815=CARTESIAN_POINT('Ctrl Pts',(14.7439974349565,7.56674273992029,-34.1658034093158));
#31816=CARTESIAN_POINT('Ctrl Pts',(16.8461293839489,5.10010790554499,-34.6388295936079));
#31817=CARTESIAN_POINT('Ctrl Pts',(17.869539668257,3.97330758910436,-34.7622699672013));
#31818=CARTESIAN_POINT('Ctrl Pts',(19.2561499197764,2.73819527916447,-34.8817370116275));
#31819=CARTESIAN_POINT('Ctrl Pts',(19.7609682985244,2.30174976258002,-34.9159236099686));
#31820=CARTESIAN_POINT('Ctrl Pts',(20.8205490930365,1.45014125059819,-34.962142837607));
#31821=CARTESIAN_POINT('Ctrl Pts',(21.6560398772552,0.871063560332534,-34.9776921520547));
#31822=CARTESIAN_POINT('Ctrl Pts',(22.3683071131494,0.447764459080894,-34.9899406319134));
#31823=CARTESIAN_POINT('Ctrl Pts',(22.628558263498,0.297072507988388,-34.9931292198003));
#31824=CARTESIAN_POINT('Ctrl Pts',(23.1658987323054,0.00272021601686333,
-34.9961615195562));
#31825=CARTESIAN_POINT('Ctrl Pts',(23.8506336743687,-0.338080815637156,
-34.9944685164155));
#31826=CARTESIAN_POINT('Ctrl Pts',(24.5584297298735,-0.638330240963619,
-34.9894063813143));
#31827=CARTESIAN_POINT('Ctrl Pts',(25.0640452406954,-0.821508451465936,
-34.9860482895808));
#31828=CARTESIAN_POINT('Ctrl Pts',(25.3563918473524,-0.917987033927376,
-34.9844827679614));
#31829=CARTESIAN_POINT('Ctrl Pts',(25.5031889952515,-0.963173610848517,
-34.9838627756015));
#31830=CARTESIAN_POINT('Ctrl Pts',(26.004987441878,-1.11209942724697,-34.9821396575606));
#31831=CARTESIAN_POINT('Ctrl Pts',(27.1869158502136,-1.35964566982755,-34.9762669195668));
#31832=CARTESIAN_POINT('Ctrl Pts',(28.241775526507,-1.43886068581106,-34.9698005674756));
#31833=CARTESIAN_POINT('Ctrl Pts',(29.0449901822568,-1.50891651433762,-34.967341499596));
#31834=CARTESIAN_POINT('Ctrl Pts',(29.4327578078034,-1.53412418433924,-34.9665584285133));
#31835=CARTESIAN_POINT('Ctrl Pts',(29.9251326248081,-1.54823778132882,-34.9660664877723));
#31836=CARTESIAN_POINT('Ctrl Pts',(30.4634303371364,-1.55173467727118,-34.9659564517225));
#31837=CARTESIAN_POINT('Ctrl Pts',(31.5090284502475,-1.53573375297651,-34.9664954568879));
#31838=CARTESIAN_POINT('Ctrl Pts',(32.3724987732541,-1.49951478355662,-34.9678633280106));
#31839=CARTESIAN_POINT('Ctrl Pts',(33.1590931275331,-1.49974473197886,-34.9678645639232));
#31840=CARTESIAN_POINT('Ctrl Pts',(33.4546837514055,-1.49973608826798,-34.96786452809));
#31841=CARTESIAN_POINT('Ctrl Pts',(33.780570662352,-1.49976277569534,-34.9678646749597));
#31842=CARTESIAN_POINT('Ctrl Pts',(34.275607154309,-1.49976889496147,-34.9678647123124));
#31843=CARTESIAN_POINT('Ctrl Pts',(34.8098427469218,-1.4998308160265,-34.9678650656176));
#31844=CARTESIAN_POINT('Ctrl Pts',(35.6330715352155,-1.49983931935013,-34.9678651148618));
#31845=CARTESIAN_POINT('Ctrl Pts',(36.291295234337,-1.49985575728851,-34.9678652087707));
#31846=CARTESIAN_POINT('Ctrl Pts',(38.1018744475862,-1.49987831370054,-34.9678653381985));
#31847=CARTESIAN_POINT('Ctrl Pts',(39.5833333333333,-1.50000000000001,-34.9678660352249));
#31848=CARTESIAN_POINT('Ctrl Pts',(40.9,-1.50000000000001,-34.9678660352249));
#31849=CARTESIAN_POINT('',(40.9,-1.50000000000002,-32.9658914637539));
#31850=CARTESIAN_POINT('Ctrl Pts',(40.9,-1.50000000000002,-32.9658914637539));
#31851=CARTESIAN_POINT('Ctrl Pts',(40.9,-1.50000000000002,-33.466386268912));
#31852=CARTESIAN_POINT('Ctrl Pts',(40.9,-1.50000000000002,-33.9668810740701));
#31853=CARTESIAN_POINT('Ctrl Pts',(40.9,-1.50000000000002,-34.4673758792282));
#31854=CARTESIAN_POINT('',(38.,-1.5,-32.9658914637539));
#31855=CARTESIAN_POINT('Ctrl Pts',(38.,-1.50000000000001,-32.9658914637539));
#31856=CARTESIAN_POINT('Ctrl Pts',(38.9666666666667,-1.50000000000001,-32.9658914637539));
#31857=CARTESIAN_POINT('Ctrl Pts',(39.9333333333333,-1.50000000000001,-32.9658914637539));
#31858=CARTESIAN_POINT('Ctrl Pts',(40.9,-1.50000000000001,-32.9658914637539));
#31859=CARTESIAN_POINT('Ctrl Pts',(37.499759314198,-1.49989731090857,-32.3652586491488));
#31860=CARTESIAN_POINT('Ctrl Pts',(37.6667177862607,-1.49990104941725,-32.5658057373987));
#31861=CARTESIAN_POINT('Ctrl Pts',(37.8334339226403,-1.49990571638763,-32.7660568899056));
#31862=CARTESIAN_POINT('Ctrl Pts',(37.9998061672102,-1.49991103444899,-32.9658910126336));
#31863=CARTESIAN_POINT('',(6.9,16.9192021366758,-24.7737885487526));
#31864=CARTESIAN_POINT('Ctrl Pts',(6.9,16.9192021366758,-24.7737885487526));
#31865=CARTESIAN_POINT('Ctrl Pts',(6.9,15.3881766950258,-22.645444622876));
#31866=CARTESIAN_POINT('Ctrl Pts',(6.90000000000115,13.8353835251886,-20.4978726403359));
#31867=CARTESIAN_POINT('Ctrl Pts',(6.90000000000115,10.3082122779765,-15.662481608859));
#31868=CARTESIAN_POINT('Ctrl Pts',(6.9,7.95935811114668,-12.4764228571341));
#31869=CARTESIAN_POINT('Ctrl Pts',(6.9,5.6597919716369,-9.46599415782505));
#31870=CARTESIAN_POINT('',(22.9245129145126,-5.83616550085653E-15,-31.7706052331164));
#31871=CARTESIAN_POINT('Ctrl Pts',(22.9245129145126,-9.86197306871846E-15,
-31.7706052331164));
#31872=CARTESIAN_POINT('Ctrl Pts',(22.7202811020963,0.0979233563002592,
-31.7014549124251));
#31873=CARTESIAN_POINT('Ctrl Pts',(22.5089075447093,0.203440182623867,-31.6320805544326));
#31874=CARTESIAN_POINT('Ctrl Pts',(22.2913349439917,0.316637134194161,-31.5632247707622));
#31875=CARTESIAN_POINT('Ctrl Pts',(21.4451770585292,0.756869465221163,-31.2954389184984));
#31876=CARTESIAN_POINT('Ctrl Pts',(20.5220951556668,1.35418571023225,-31.0475106147151));
#31877=CARTESIAN_POINT('Ctrl Pts',(19.7671428819538,1.89915402350704,-30.8612920963158));
#31878=CARTESIAN_POINT('Ctrl Pts',(19.5194773058391,2.07793339270832,-30.8002022522972));
#31879=CARTESIAN_POINT('Ctrl Pts',(19.2865716386091,2.25204835959322,-30.7444068279678));
#31880=CARTESIAN_POINT('Ctrl Pts',(19.0728538401323,2.41532203906683,-30.6939488833522));
#31881=CARTESIAN_POINT('Ctrl Pts',(18.7028555998036,2.69798906318807,-30.6065937315988));
#31882=CARTESIAN_POINT('Ctrl Pts',(18.4144703596236,2.93373938287709,-30.539966063932));
#31883=CARTESIAN_POINT('Ctrl Pts',(18.0642874871539,3.23398234069978,-30.4582462938821));
#31884=CARTESIAN_POINT('Ctrl Pts',(17.4420927116722,3.76744532366909,-30.3130489756353));
#31885=CARTESIAN_POINT('Ctrl Pts',(16.7224564418219,4.43872907330225,-30.1446863488622));
#31886=CARTESIAN_POINT('Ctrl Pts',(15.9202806616111,5.24401550821528,-29.9321297384067));
#31887=CARTESIAN_POINT('Ctrl Pts',(15.4090529834523,5.75722561070076,-29.7966671314305));
#31888=CARTESIAN_POINT('Ctrl Pts',(14.8739602945724,6.33424649579561,-29.6418940055918));
#31889=CARTESIAN_POINT('Ctrl Pts',(14.3169794331169,6.96996102647052,-29.4557634846127));
#31890=CARTESIAN_POINT('Ctrl Pts',(13.8864206762846,7.46138268378274,-29.3118803976572));
#31891=CARTESIAN_POINT('Ctrl Pts',(13.386789002781,8.05270459511923,-29.1311705407941));
#31892=CARTESIAN_POINT('Ctrl Pts',(12.8146824059514,8.75043091662867,-28.8915984033895));
#31893=CARTESIAN_POINT('Ctrl Pts',(12.2526665517594,9.43585083093896,-28.6562518085588));
#31894=CARTESIAN_POINT('Ctrl Pts',(11.6379478462803,10.2313662767681,-28.3625845909802));
#31895=CARTESIAN_POINT('Ctrl Pts',(10.9739250490307,11.1267230319108,-27.9810212930959));
#31896=CARTESIAN_POINT('Ctrl Pts',(10.5683455447962,11.6735993596029,-27.7479656603209));
#31897=CARTESIAN_POINT('Ctrl Pts',(10.1437415406955,12.2581093618547,-27.4801235315866));
#31898=CARTESIAN_POINT('Ctrl Pts',(9.74137929176524,12.8142541611144,-27.2046666925187));
#31899=CARTESIAN_POINT('Ctrl Pts',(8.72285779294233,14.2220538143138,-26.5073877769786));
#31900=CARTESIAN_POINT('Ctrl Pts',(7.81323138778195,15.580948814124,-25.7100913255874));
#31901=CARTESIAN_POINT('Ctrl Pts',(6.9,16.9192021366758,-24.7737885487526));
#31902=CARTESIAN_POINT('Ctrl Pts',(30.5,-1.55029606206997,-34.9656486014478));
#31903=CARTESIAN_POINT('Ctrl Pts',(29.9560179420817,-1.55343104498103,-34.7222276068062));
#31904=CARTESIAN_POINT('Ctrl Pts',(29.4152668325132,-1.54030953139106,-34.4790656554127));
#31905=CARTESIAN_POINT('Ctrl Pts',(28.8740459957565,-1.49470250846617,-34.2361296888632));
#31906=CARTESIAN_POINT('Ctrl Pts',(28.3535277923439,-1.45084003307051,-34.0024864433252));
#31907=CARTESIAN_POINT('Ctrl Pts',(27.8179515912466,-1.40923473841146,-33.7608540997398));
#31908=CARTESIAN_POINT('Ctrl Pts',(27.2695051149491,-1.33972398862117,-33.5168388499063));
#31909=CARTESIAN_POINT('Ctrl Pts',(26.9554553615883,-1.29992095446743,-33.3771115796287));
#31910=CARTESIAN_POINT('Ctrl Pts',(26.6378099296971,-1.25106463707209,-33.2369493090937));
#31911=CARTESIAN_POINT('Ctrl Pts',(26.3179304017917,-1.18777049128279,-33.0983258448229));
#31912=CARTESIAN_POINT('Ctrl Pts',(26.1078196745982,-1.14619615520082,-33.0072719500184));
#31913=CARTESIAN_POINT('Ctrl Pts',(25.8967402232745,-1.09839525532295,-32.9168907470981));
#31914=CARTESIAN_POINT('Ctrl Pts',(25.6850706236774,-1.04282885388103,-32.8277596053404));
#31915=CARTESIAN_POINT('Ctrl Pts',(25.6562210027417,-1.03525540156945,-32.8156114288513));
#31916=CARTESIAN_POINT('Ctrl Pts',(25.6277737638215,-1.0276506122434,-32.8036595933923));
#31917=CARTESIAN_POINT('Ctrl Pts',(25.5983858063598,-1.01964325944537,-32.7913423709803));
#31918=CARTESIAN_POINT('Ctrl Pts',(25.1249357452756,-0.890642063078177,
-32.5929076988546));
#31919=CARTESIAN_POINT('Ctrl Pts',(24.1510084067019,-0.588069770626608,
-32.1858811669087));
#31920=CARTESIAN_POINT('Ctrl Pts',(22.9245129145126,-9.86197306871846E-15,
-31.7706052331164));
#31921=CARTESIAN_POINT('Origin',(40.65,0.,0.));
#31922=CARTESIAN_POINT('',(40.4,18.7829592905825,-29.5330398077868));
#31923=CARTESIAN_POINT('',(40.9,18.5327260452907,-29.0996231131986));
#31924=CARTESIAN_POINT('Ctrl Pts',(40.4,18.7829592905825,-29.5330398077868));
#31925=CARTESIAN_POINT('Ctrl Pts',(40.5666590140292,18.699553150888,-29.3885761361728));
#31926=CARTESIAN_POINT('Ctrl Pts',(40.7333430452231,18.616133394895,-29.2440888804379));
#31927=CARTESIAN_POINT('Ctrl Pts',(40.9,18.5327260452907,-29.0996231131986));
#31928=CARTESIAN_POINT('',(40.9,15.9346498339374,-30.5996231131986));
#31929=CARTESIAN_POINT('Origin',(40.9,0.,0.));
#31930=CARTESIAN_POINT('',(40.4,16.1848830792292,-31.0330398077868));
#31931=CARTESIAN_POINT('Ctrl Pts',(40.9,15.9346498339374,-30.5996231131986));
#31932=CARTESIAN_POINT('Ctrl Pts',(40.7333430442937,16.0180571840068,-30.7440888812435));
#31933=CARTESIAN_POINT('Ctrl Pts',(40.5666590123859,16.1014769403571,-30.8885761375972));
#31934=CARTESIAN_POINT('Ctrl Pts',(40.4,16.1848830792292,-31.0330398077868));
#31935=CARTESIAN_POINT('Origin',(40.4,0.,0.));
#31936=CARTESIAN_POINT('Origin',(35.7,0.,0.));
#31937=CARTESIAN_POINT('',(30.5,16.1402285275843,-31.0562879796886));
#31938=CARTESIAN_POINT('Ctrl Pts',(40.3999012894849,16.1848928782182,-31.0330346270951));
#31939=CARTESIAN_POINT('Ctrl Pts',(39.2494626810401,16.1849362443212,-31.0330116996609));
#31940=CARTESIAN_POINT('Ctrl Pts',(38.0976708836828,16.1851115327779,-31.0329190263647));
#31941=CARTESIAN_POINT('Ctrl Pts',(36.9467340384723,16.1851746119074,-31.0328856894588));
#31942=CARTESIAN_POINT('Ctrl Pts',(36.745427730736,16.1851856448556,-31.032879858618));
#31943=CARTESIAN_POINT('Ctrl Pts',(36.5441475779313,16.1851932450653,-31.0328758430125));
#31944=CARTESIAN_POINT('Ctrl Pts',(36.3429119519248,16.1852000001162,-31.0328722727086));
#31945=CARTESIAN_POINT('Ctrl Pts',(36.2102758775794,16.1852044524265,-31.0328699194916));
#31946=CARTESIAN_POINT('Ctrl Pts',(36.0822774296293,16.1852084224022,-31.0328678560427));
#31947=CARTESIAN_POINT('Ctrl Pts',(35.9587202262686,16.1852125810273,-31.0328657167445));
#31948=CARTESIAN_POINT('Ctrl Pts',(35.7925662245335,16.1852181733537,-31.0328628399153));
#31949=CARTESIAN_POINT('Ctrl Pts',(35.6344388155487,16.1852241162452,-31.0328598211429));
#31950=CARTESIAN_POINT('Ctrl Pts',(35.483771446345,16.1852312078525,-31.032856216152));
#31951=CARTESIAN_POINT('Ctrl Pts',(35.3175474553568,16.1852390316786,-31.0328522389407));
#31952=CARTESIAN_POINT('Ctrl Pts',(35.1604041224798,16.1852482463284,-31.0328475520712));
#31953=CARTESIAN_POINT('Ctrl Pts',(35.0116427948666,16.1852592402396,-31.0328419178902));
#31954=CARTESIAN_POINT('Ctrl Pts',(34.9979272091136,16.1852602538628,-31.0328413984267));
#31955=CARTESIAN_POINT('Ctrl Pts',(34.9842829110367,16.1852612822246,-31.0328408711132));
#31956=CARTESIAN_POINT('Ctrl Pts',(34.9707093736272,16.1852623254083,-31.0328403358797));
#31957=CARTESIAN_POINT('Ctrl Pts',(34.8522491799023,16.1852714295753,-31.0328356647415));
#31958=CARTESIAN_POINT('Ctrl Pts',(34.7391835006529,16.1852816068676,-31.0328304196803));
#31959=CARTESIAN_POINT('Ctrl Pts',(34.6312849042887,16.1852915612822,-31.0328252639047));
#31960=CARTESIAN_POINT('Ctrl Pts',(34.5096795260851,16.1853027802452,-31.0328194531708));
#31961=CARTESIAN_POINT('Ctrl Pts',(34.3946370581326,16.1853137193614,-31.0328137541413));
#31962=CARTESIAN_POINT('Ctrl Pts',(34.2857585821188,16.1853233495613,-31.0328086821746));
#31963=CARTESIAN_POINT('Ctrl Pts',(34.1786801908151,16.1853328205454,-31.0328036940625));
#31964=CARTESIAN_POINT('Ctrl Pts',(34.0775620514827,16.185341043166,-31.0327993031901));
#31965=CARTESIAN_POINT('Ctrl Pts',(33.9819758246427,16.1853475980775,-31.0327957057953));
#31966=CARTESIAN_POINT('Ctrl Pts',(33.9184449689727,16.1853519547631,-31.0327933148067));
#31967=CARTESIAN_POINT('Ctrl Pts',(33.8573517602305,16.1853555977386,-31.0327912624254));
#31968=CARTESIAN_POINT('Ctrl Pts',(33.7984399511826,16.1853587887284,-31.0327894081824));
#31969=CARTESIAN_POINT('Ctrl Pts',(33.7337970612213,16.1853622901452,-31.0327873735543));
#31970=CARTESIAN_POINT('Ctrl Pts',(33.6717809742681,16.1853652470741,-31.0327855776265));
#31971=CARTESIAN_POINT('Ctrl Pts',(33.6121191806454,16.1853678991827,-31.0327838881567));
#31972=CARTESIAN_POINT('Ctrl Pts',(33.5695978710648,16.1853697893561,-31.0327826840617));
#31973=CARTESIAN_POINT('Ctrl Pts',(33.5282738752657,16.1853715223629,-31.0327815352149));
#31974=CARTESIAN_POINT('Ctrl Pts',(33.4880643388298,16.1853731585247,-31.032780407062));
#31975=CARTESIAN_POINT('Ctrl Pts',(33.4508270573206,16.1853746737428,-31.0327793623013));
#31976=CARTESIAN_POINT('Ctrl Pts',(33.4145509216558,16.1853761126591,-31.0327783314862));
#31977=CARTESIAN_POINT('Ctrl Pts',(33.3793439789548,16.1853777420672,-31.0327771639657));
#31978=CARTESIAN_POINT('Ctrl Pts',(33.3411337035362,16.1853795104722,-31.0327758968498));
#31979=CARTESIAN_POINT('Ctrl Pts',(33.3041826660689,16.1853815029502,-31.0327744688781));
#31980=CARTESIAN_POINT('Ctrl Pts',(33.2685652776782,16.1853839484229,-31.0327727495066));
#31981=CARTESIAN_POINT('Ctrl Pts',(33.231009447455,16.1853865269881,-31.0327709365599));
#31982=CARTESIAN_POINT('Ctrl Pts',(33.1949357943681,16.185389608116,-31.0327688002292));
#31983=CARTESIAN_POINT('Ctrl Pts',(33.1603699172393,16.1853933524012,-31.0327662471215));
#31984=CARTESIAN_POINT('Ctrl Pts',(33.1223715679419,16.1853974685027,-31.0327634404841));
#31985=CARTESIAN_POINT('Ctrl Pts',(33.0861949166477,16.1854023852333,-31.0327601306123));
#31986=CARTESIAN_POINT('Ctrl Pts',(33.0518089354075,16.1854082033113,-31.0327562557942));
#31987=CARTESIAN_POINT('Ctrl Pts',(33.034103081306,16.1854111991264,-31.0327542605926));
#31988=CARTESIAN_POINT('Ctrl Pts',(33.0168710360022,16.1854144322605,-31.032752116523));
#31989=CARTESIAN_POINT('Ctrl Pts',(33.0001033802535,16.1854179076007,-31.0327498200704));
#31990=CARTESIAN_POINT('Ctrl Pts',(32.9420348133412,16.1854299431543,-31.0327418671573));
#31991=CARTESIAN_POINT('Ctrl Pts',(32.8874145324497,16.1852296143113,-31.0328461364757));
#31992=CARTESIAN_POINT('Ctrl Pts',(32.8357863520582,16.1849068811705,-31.0330149777623));
#31993=CARTESIAN_POINT('Ctrl Pts',(32.7779739682632,16.1845454899291,-31.0332040434467));
#31994=CARTESIAN_POINT('Ctrl Pts',(32.7239136589684,16.1840302574575,-31.0334742654593));
#31995=CARTESIAN_POINT('Ctrl Pts',(32.6729278684753,16.1834371021678,-31.033785409572));
#31996=CARTESIAN_POINT('Ctrl Pts',(32.6180801336262,16.1827990180322,-31.0341201214522));
#31997=CARTESIAN_POINT('Ctrl Pts',(32.5667902508433,16.1820699950121,-31.0345025939175));
#31998=CARTESIAN_POINT('Ctrl Pts',(32.5181731636799,16.1812992842338,-31.034906696383));
#31999=CARTESIAN_POINT('Ctrl Pts',(32.4659536029866,16.1804714646211,-31.0353407424038));
#32000=CARTESIAN_POINT('Ctrl Pts',(32.4168175136243,16.1795947944396,-31.0358001425894));
#32001=CARTESIAN_POINT('Ctrl Pts',(32.3696233879005,16.1786925325961,-31.0362725138779));
#32002=CARTESIAN_POINT('Ctrl Pts',(32.3182581618423,16.1777105272545,-31.0367866341767));
#32003=CARTESIAN_POINT('Ctrl Pts',(32.2691934412637,16.1766975364928,-31.0373164741889));
#32004=CARTESIAN_POINT('Ctrl Pts',(32.2209064724814,16.1756521425246,-31.0378627004434));
#32005=CARTESIAN_POINT('Ctrl Pts',(32.1715370438637,16.1745833137247,-31.0384211715746));
#32006=CARTESIAN_POINT('Ctrl Pts',(32.1229805798595,16.173479840102,-31.0389971805319));
#32007=CARTESIAN_POINT('Ctrl Pts',(32.0735591134775,16.1723205501866,-31.039601856364));
#32008=CARTESIAN_POINT('Ctrl Pts',(32.0254239419637,16.1711914331653,-31.0401907942693));
#32009=CARTESIAN_POINT('Ctrl Pts',(31.9764682879407,16.1700086968176,-31.0408072809901));
#32010=CARTESIAN_POINT('Ctrl Pts',(31.9250947921519,16.1687449477338,-31.041465759884));
#32011=CARTESIAN_POINT('Ctrl Pts',(31.895291910488,16.168011819419,-31.0418477578044));
#32012=CARTESIAN_POINT('Ctrl Pts',(31.8646744620479,16.1672513233695,-31.0422439429542));
#32013=CARTESIAN_POINT('Ctrl Pts',(31.8329224323944,16.1664582369103,-31.0426570718779));
#32014=CARTESIAN_POINT('Ctrl Pts',(31.7319354368357,16.163935833788,-31.0439710240642));
#32015=CARTESIAN_POINT('Ctrl Pts',(31.6284526822058,16.1613063818565,-31.0453389332579));
#32016=CARTESIAN_POINT('Ctrl Pts',(31.523233635432,16.1587277943726,-31.0466795487252));
#32017=CARTESIAN_POINT('Ctrl Pts',(31.4188807866252,16.156170434673,-31.0480091278028));
#32018=CARTESIAN_POINT('Ctrl Pts',(31.3128198672025,16.1536645426213,-31.0493111005243));
#32019=CARTESIAN_POINT('Ctrl Pts',(31.2058402970409,16.1513736799426,-31.0505011542277));
#32020=CARTESIAN_POINT('Ctrl Pts',(31.1464339374053,16.1501015509562,-31.0511619977718));
#32021=CARTESIAN_POINT('Ctrl Pts',(31.0867451889515,16.1488957763821,-31.051788304276));
#32022=CARTESIAN_POINT('Ctrl Pts',(31.0269161235859,16.1477831210733,-31.052366291213));
#32023=CARTESIAN_POINT('Ctrl Pts',(30.9223727403119,16.1458389029967,-31.0533762469848));
#32024=CARTESIAN_POINT('Ctrl Pts',(30.8173993541569,16.1441811147896,-31.0542375463396));
#32025=CARTESIAN_POINT('Ctrl Pts',(30.7129204018003,16.1429541726495,-31.0548748925162));
#32026=CARTESIAN_POINT('Ctrl Pts',(30.6397146645873,16.1420944855847,-31.0553214647269));
#32027=CARTESIAN_POINT('Ctrl Pts',(30.5667525557982,16.1414458510594,-31.0556583368409));
#32028=CARTESIAN_POINT('Ctrl Pts',(30.4943593393942,16.1410459118957,-31.0558660149161));
#32029=CARTESIAN_POINT('',(30.5,18.7405179110272,-29.559989655385));
#32030=CARTESIAN_POINT('Origin',(30.5,0.,0.));
#32031=CARTESIAN_POINT('Ctrl Pts',(30.5049791804999,18.7395177484755,-29.5605178050969));
#32032=CARTESIAN_POINT('Ctrl Pts',(30.597367682774,18.74007970098,-29.5601622646425));
#32033=CARTESIAN_POINT('Ctrl Pts',(30.6891105694842,18.741056756011,-29.5595425101545));
#32034=CARTESIAN_POINT('Ctrl Pts',(30.7806774793076,18.7423441244045,-29.5587264396731));
#32035=CARTESIAN_POINT('Ctrl Pts',(30.8441888930625,18.7432370516295,-29.5581604077944));
#32036=CARTESIAN_POINT('Ctrl Pts',(30.9076166453413,18.7442800408073,-29.5574994222388));
#32037=CARTESIAN_POINT('Ctrl Pts',(30.9711288096736,18.7454455999908,-29.5567612578197));
#32038=CARTESIAN_POINT('Ctrl Pts',(31.0735567068107,18.7473253308645,-29.5555707987951));
#32039=CARTESIAN_POINT('Ctrl Pts',(31.176201908291,18.7495231556638,-29.5541800414695));
#32040=CARTESIAN_POINT('Ctrl Pts',(31.2798872709465,18.7519033574719,-29.5526737444511));
#32041=CARTESIAN_POINT('Ctrl Pts',(31.3828989348227,18.7542680938468,-29.5511772346432));
#32042=CARTESIAN_POINT('Ctrl Pts',(31.4869372222045,18.7568144117906,-29.5495656759356));
#32043=CARTESIAN_POINT('Ctrl Pts',(31.5928574097326,18.7594156373079,-29.5479181178242));
#32044=CARTESIAN_POINT('Ctrl Pts',(31.6516459294224,18.7608593866168,-29.5470036792764));
#32045=CARTESIAN_POINT('Ctrl Pts',(31.7110150391174,18.7623200347848,-29.5460781618904));
#32046=CARTESIAN_POINT('Ctrl Pts',(31.771117672524,18.7637740491308,-29.5451562912552));
#32047=CARTESIAN_POINT('Ctrl Pts',(31.8409082760362,18.7654624366934,-29.5440858238838));
#32048=CARTESIAN_POINT('Ctrl Pts',(31.9056373311744,18.7669933631238,-29.5431152615712));
#32049=CARTESIAN_POINT('Ctrl Pts',(31.9658882086279,18.7683675834938,-29.5422441375116));
#32050=CARTESIAN_POINT('Ctrl Pts',(32.0341093482752,18.7699235920322,-29.5412577771691));
#32051=CARTESIAN_POINT('Ctrl Pts',(32.0965888127919,18.7712796560441,-29.5403982847663));
#32052=CARTESIAN_POINT('Ctrl Pts',(32.1542362617658,18.772463407492,-29.5396480149482));
#32053=CARTESIAN_POINT('Ctrl Pts',(32.2151538519833,18.7737143090828,-29.5388551849072));
#32054=CARTESIAN_POINT('Ctrl Pts',(32.2706761902197,18.7747738843963,-29.5381836213571));
#32055=CARTESIAN_POINT('Ctrl Pts',(32.3219402247771,18.7756849339007,-29.5376060245815));
#32056=CARTESIAN_POINT('Ctrl Pts',(32.3761674213252,18.7766486438578,-29.5369950415767));
#32057=CARTESIAN_POINT('Ctrl Pts',(32.4256304058838,18.7774469218489,-29.5364887148645));
#32058=CARTESIAN_POINT('Ctrl Pts',(32.471735031406,18.7781265619111,-29.5360572749795));
#32059=CARTESIAN_POINT('Ctrl Pts',(32.5214923281247,18.7788600469324,-29.5355916539678));
#32060=CARTESIAN_POINT('Ctrl Pts',(32.5673384642519,18.7794559410664,-29.535212877449));
#32061=CARTESIAN_POINT('Ctrl Pts',(32.6111004962922,18.7799576530149,-29.5348934788925));
#32062=CARTESIAN_POINT('Ctrl Pts',(32.6551147163173,18.7804622561848,-29.5345722397342));
#32063=CARTESIAN_POINT('Ctrl Pts',(32.6970214084867,18.7808718608787,-29.5343108907555));
#32064=CARTESIAN_POINT('Ctrl Pts',(32.7387279964578,18.7812095285093,-29.5340950825229));
#32065=CARTESIAN_POINT('Ctrl Pts',(32.7800761354878,18.7815442940419,-29.5338811290628));
#32066=CARTESIAN_POINT('Ctrl Pts',(32.821227734235,18.7818087481601,-29.5337116838821));
#32067=CARTESIAN_POINT('Ctrl Pts',(32.8640829337526,18.7820000955038,-29.5335890251801));
#32068=CARTESIAN_POINT('Ctrl Pts',(32.9037320332525,18.782177127695,-29.5334755428692));
#32069=CARTESIAN_POINT('Ctrl Pts',(32.9448394203908,18.7822919200909,-29.5334018918634));
#32070=CARTESIAN_POINT('Ctrl Pts',(32.9889438598235,18.7823158450365,-29.5333868654403));
#32071=CARTESIAN_POINT('Ctrl Pts',(32.9925102269245,18.7823177796522,-29.5333856503758));
#32072=CARTESIAN_POINT('Ctrl Pts',(32.9960962106233,18.7823191027631,-29.5333848297965));
#32073=CARTESIAN_POINT('Ctrl Pts',(32.9997026353886,18.7823197895504,-29.5333844198651));
#32074=CARTESIAN_POINT('Ctrl Pts',(33.0361388185044,18.7823267282527,-29.5333802782741));
#32075=CARTESIAN_POINT('Ctrl Pts',(33.0740002606602,18.7823330770043,-29.5333765562526));
#32076=CARTESIAN_POINT('Ctrl Pts',(33.1140504028665,18.7823389179973,-29.5333733966323));
#32077=CARTESIAN_POINT('Ctrl Pts',(33.2460690464805,18.7823581718609,-29.5333629814687));
#32078=CARTESIAN_POINT('Ctrl Pts',(33.3720922029404,18.7823661897827,-29.5333587011921));
#32079=CARTESIAN_POINT('Ctrl Pts',(33.4992849360723,18.7823737360728,-29.5333546566754));
#32080=CARTESIAN_POINT('Ctrl Pts',(33.6626792864135,18.7823834301892,-29.5333494610076));
#32081=CARTESIAN_POINT('Ctrl Pts',(33.8280037294634,18.7823923459957,-29.5333446544024));
#32082=CARTESIAN_POINT('Ctrl Pts',(33.9928746198632,18.7824059536075,-29.533337331307));
#32083=CARTESIAN_POINT('Ctrl Pts',(34.3226164006628,18.7824331688311,-29.5333226851163));
#32084=CARTESIAN_POINT('Ctrl Pts',(34.6505439708619,18.7824791512757,-29.533297972965));
#32085=CARTESIAN_POINT('Ctrl Pts',(34.9791449252859,18.7825099763788,-29.5332814027047));
#32086=CARTESIAN_POINT('Ctrl Pts',(35.3077458797098,18.7825408014818,-29.5332648324443));
#32087=CARTESIAN_POINT('Ctrl Pts',(35.6370202183587,18.7825564692434,-29.533256404075));
#32088=CARTESIAN_POINT('Ctrl Pts',(35.9661418060972,18.7825697306316,-29.5332492722833));
#32089=CARTESIAN_POINT('Ctrl Pts',(36.2952633938356,18.7825829920198,-29.5332421404916));
#32090=CARTESIAN_POINT('Ctrl Pts',(36.6242322306636,18.7825938470346,-29.5332363052775));
#32091=CARTESIAN_POINT('Ctrl Pts',(36.9531363303402,18.7826154119859,-29.5332247108409));
#32092=CARTESIAN_POINT('Ctrl Pts',(38.1022190076917,18.7826907528288,-29.5331842036953));
#32093=CARTESIAN_POINT('Ctrl Pts',(39.2505115204485,18.782896816333,-29.5330734009978));
#32094=CARTESIAN_POINT('Ctrl Pts',(40.400093943525,18.7829477771169,-29.533045998731));
#32095=CARTESIAN_POINT('Ctrl Pts',(6.89999999997365,9.63452070648359,-5.36789542691341));
#32096=CARTESIAN_POINT('Ctrl Pts',(6.99168932310453,9.60499723839753,-5.42175501956001));
#32097=CARTESIAN_POINT('Ctrl Pts',(7.08383915760478,9.57508016834563,-5.47527828673705));
#32098=CARTESIAN_POINT('Ctrl Pts',(8.15762752947026,9.22342495405909,-6.09209251732963));
#32099=CARTESIAN_POINT('Ctrl Pts',(9.16608342448599,8.84591675027098,-6.61836595106259));
#32100=CARTESIAN_POINT('Ctrl Pts',(11.2535425311854,8.09542754093136,-7.53037930120419));
#32101=CARTESIAN_POINT('Ctrl Pts',(12.2577133097064,7.7072500137176,-7.91666449612082));
#32102=CARTESIAN_POINT('Ctrl Pts',(14.356433377742,6.97440810645326,-8.58141250110814));
#32103=CARTESIAN_POINT('Ctrl Pts',(15.3659105035251,6.61345583116596,-8.85322312286061));
#32104=CARTESIAN_POINT('Ctrl Pts',(17.4728641219044,5.96623757129007,-9.31281879192962));
#32105=CARTESIAN_POINT('Ctrl Pts',(18.4890996814195,5.66020885204394,-9.49384943617778));
#32106=CARTESIAN_POINT('Ctrl Pts',(19.8476172011441,5.32865724601648,-9.68599953593308));
#32107=CARTESIAN_POINT('Ctrl Pts',(20.3454889307686,5.20930542916259,-9.75195458239819));
#32108=CARTESIAN_POINT('Ctrl Pts',(21.3782040612024,4.97678151322346,-9.87366876552719));
#32109=CARTESIAN_POINT('Ctrl Pts',(22.1792648896895,4.81935607344486,-9.95072592994715));
#32110=CARTESIAN_POINT('Ctrl Pts',(22.8542621828909,4.70591921690554,-10.0067883222624));
#32111=CARTESIAN_POINT('Ctrl Pts',(23.1054579010967,4.66456206383028,-10.0267605301623));
#32112=CARTESIAN_POINT('Ctrl Pts',(23.6171513959785,4.58448144656259,-10.0644076466806));
#32113=CARTESIAN_POINT('Ctrl Pts',(24.1360713221937,4.51012725444834,-10.0979855598765));
#32114=CARTESIAN_POINT('Ctrl Pts',(24.6624927871864,4.44285620865165,-10.1277002159266));
#32115=CARTESIAN_POINT('Ctrl Pts',(25.1928168818088,4.3809527171812,-10.154786256444));
#32116=CARTESIAN_POINT('Ctrl Pts',(25.5948982287615,4.34117176259643,-10.1721457030179));
#32117=CARTESIAN_POINT('Ctrl Pts',(26.1232031889651,4.29604941535506,-10.1922876384417));
#32118=CARTESIAN_POINT('Ctrl Pts',(27.1768897027567,4.2232612911204,-10.2241871753182));
#32119=CARTESIAN_POINT('Ctrl Pts',(28.2111297865347,4.19969555688313,-10.2325109692973));
#32120=CARTESIAN_POINT('Ctrl Pts',(29.1277555719713,4.17661492679514,-10.2421056253618));
#32121=CARTESIAN_POINT('Ctrl Pts',(29.4767605677587,4.1700561490002,-10.2448788784735));
#32122=CARTESIAN_POINT('Ctrl Pts',(30.1601418995912,4.16421367130871,-10.2473221772452));
#32123=CARTESIAN_POINT('Ctrl Pts',(31.3500242312262,4.16794387579264,-10.2457563290907));
#32124=CARTESIAN_POINT('Ctrl Pts',(32.3461596131128,4.18040640609126,-10.2405791191157));
#32125=CARTESIAN_POINT('Ctrl Pts',(33.1614718826738,4.18039330945984,-10.2405840900447));
#32126=CARTESIAN_POINT('Ctrl Pts',(33.4925794155279,4.18039253080268,-10.2405841444578));
#32127=CARTESIAN_POINT('Ctrl Pts',(34.1499904318886,4.18039030822714,-10.2405848392549));
#32128=CARTESIAN_POINT('Ctrl Pts',(34.9738731541179,4.18038393925505,-10.2405865289644));
#32129=CARTESIAN_POINT('Ctrl Pts',(35.9612754428242,4.18038119412748,-10.2405873001735));
#32130=CARTESIAN_POINT('Ctrl Pts',(37.936646788162,4.18037753677864,-10.2405882857915));
#32131=CARTESIAN_POINT('Ctrl Pts',(39.5833333333333,4.18035859466987,-10.2405934798255));
#32132=CARTESIAN_POINT('Ctrl Pts',(40.9,4.18035859466987,-10.2405934798255));
#32133=CARTESIAN_POINT('Ctrl Pts',(6.71972576838711,12.8464244365415,-6.57643817146341));
#32134=CARTESIAN_POINT('Ctrl Pts',(6.81144220747046,12.8102053989753,-6.64828376862611));
#32135=CARTESIAN_POINT('Ctrl Pts',(6.90362823998598,12.7734498343709,-6.7197152492286));
#32136=CARTESIAN_POINT('Ctrl Pts',(7.9778781148633,12.3410744046091,-7.54294881554196));
#32137=CARTESIAN_POINT('Ctrl Pts',(8.98681832185142,11.871220138602,-8.24809748747638));
#32138=CARTESIAN_POINT('Ctrl Pts',(11.0806583453373,10.9274240314556,-9.47774891389535));
#32139=CARTESIAN_POINT('Ctrl Pts',(12.0862475175457,10.4368998098017,-10.0005505115845));
#32140=CARTESIAN_POINT('Ctrl Pts',(14.197639322261,9.50280276487817,-10.906656993414));
#32141=CARTESIAN_POINT('Ctrl Pts',(15.2100862637122,9.04203633254719,-11.2785931828498));
#32142=CARTESIAN_POINT('Ctrl Pts',(17.3364698493954,8.20932952666152,-11.9121957711898));
#32143=CARTESIAN_POINT('Ctrl Pts',(18.357279581038,7.81594677169138,-12.1627870018009));
#32144=CARTESIAN_POINT('Ctrl Pts',(19.7331217809845,7.38628119283515,-12.4307568384137));
#32145=CARTESIAN_POINT('Ctrl Pts',(20.2341927100358,7.23233618870704,-12.5225360922774));
#32146=CARTESIAN_POINT('Ctrl Pts',(21.2777139275316,6.93114017240204,-12.6928916013278));
#32147=CARTESIAN_POINT('Ctrl Pts',(22.0885637816418,6.72673758680646,-12.8012350092453));
#32148=CARTESIAN_POINT('Ctrl Pts',(22.7734874647764,6.57909772915771,-12.8801738355232));
#32149=CARTESIAN_POINT('Ctrl Pts',(23.0269571312139,6.52549682636868,-12.9082278965574));
#32150=CARTESIAN_POINT('Ctrl Pts',(23.5444618566097,6.42148511325402,-12.9612738268023));
#32151=CARTESIAN_POINT('Ctrl Pts',(24.0694383156461,6.32485290039693,-13.0087020921734));
#32152=CARTESIAN_POINT('Ctrl Pts',(24.6027295908464,6.2373000813771,-13.0507741241225));
#32153=CARTESIAN_POINT('Ctrl Pts',(25.1403192523141,6.15667530541498,-13.0891677302172));
#32154=CARTESIAN_POINT('Ctrl Pts',(25.5484689870706,6.10479659087691,-13.1137995888261));
#32155=CARTESIAN_POINT('Ctrl Pts',(26.0852808149067,6.04589855121054,-13.1423647911197));
#32156=CARTESIAN_POINT('Ctrl Pts',(27.1586857291269,5.95074158602807,-13.1877077660314));
#32157=CARTESIAN_POINT('Ctrl Pts',(28.1995312980844,5.92039197700573,-13.1995114624862));
#32158=CARTESIAN_POINT('Ctrl Pts',(29.1157533315888,5.89061060808305,-13.2130297822556));
#32159=CARTESIAN_POINT('Ctrl Pts',(29.4698938670486,5.88204921070822,-13.2169740538762));
#32160=CARTESIAN_POINT('Ctrl Pts',(30.1587234046998,5.87447683559579,-13.220429005539));
#32161=CARTESIAN_POINT('Ctrl Pts',(31.355731195606,5.87931523414859,-13.2182120926509));
#32162=CARTESIAN_POINT('Ctrl Pts',(32.350180243561,5.89537176970751,-13.2109234983782));
#32163=CARTESIAN_POINT('Ctrl Pts',(33.1605031382466,5.89535013085608,-13.2109314016452));
#32164=CARTESIAN_POINT('Ctrl Pts',(33.4922179295252,5.89534881762644,-13.2109314596682));
#32165=CARTESIAN_POINT('Ctrl Pts',(34.1493400019899,5.89534512891167,-13.2109325467447));
#32166=CARTESIAN_POINT('Ctrl Pts',(34.9735241318652,5.89533452524069,-13.2109351472382));
#32167=CARTESIAN_POINT('Ctrl Pts',(35.9608954520827,5.89532995964261,-13.2109363413972));
#32168=CARTESIAN_POINT('Ctrl Pts',(37.9363824842976,5.89532387223529,-13.2109378608691));
#32169=CARTESIAN_POINT('Ctrl Pts',(39.5833333333333,5.89529235427928,-13.2109458830841));
#32170=CARTESIAN_POINT('Ctrl Pts',(40.9,5.89529235427928,-13.2109458830841));
#32171=CARTESIAN_POINT('Ctrl Pts',(6.48177011792014,20.336764848396,-9.40621265917916));
#32172=CARTESIAN_POINT('Ctrl Pts',(6.57271435585528,20.2851799357091,-9.51911083717173));
#32173=CARTESIAN_POINT('Ctrl Pts',(6.66411141569866,20.2327517601296,-9.63139437446866));
#32174=CARTESIAN_POINT('Ctrl Pts',(7.73048017258431,19.614616528956,-10.9276768808967));
#32175=CARTESIAN_POINT('Ctrl Pts',(8.73292722985418,18.9319609573801,-12.0456324995184));
#32176=CARTESIAN_POINT('Ctrl Pts',(10.8102906905198,17.5485371602851,-14.0013807284478));
#32177=CARTESIAN_POINT('Ctrl Pts',(11.8125687231201,16.8218444562665,-14.8418955382559));
#32178=CARTESIAN_POINT('Ctrl Pts',(13.9177445864075,15.4271303717406,-16.3050153868123));
#32179=CARTESIAN_POINT('Ctrl Pts',(14.9296562678442,14.7350649820735,-16.9116612373854));
#32180=CARTESIAN_POINT('Ctrl Pts',(17.0680844879216,13.4708635112562,-17.9535844659564));
#32181=CARTESIAN_POINT('Ctrl Pts',(18.0932339179161,12.8729609429,-18.3688941094638));
#32182=CARTESIAN_POINT('Ctrl Pts',(19.4933464326809,12.2099892645604,-18.8183285494774));
#32183=CARTESIAN_POINT('Ctrl Pts',(19.9993272808496,11.9744841299437,-18.971430097181));
#32184=CARTESIAN_POINT('Ctrl Pts',(21.0600020168761,11.5100300116438,-19.2581324129064));
#32185=CARTESIAN_POINT('Ctrl Pts',(21.8888875769482,11.1928649299996,-19.4420158954033));
#32186=CARTESIAN_POINT('Ctrl Pts',(22.5933490549503,10.962505511385,-19.5764520117208));
#32187=CARTESIAN_POINT('Ctrl Pts',(22.8513437851799,10.8796937171906,-19.6238525927722));
#32188=CARTESIAN_POINT('Ctrl Pts',(23.3805933886566,10.7182299385361,-19.7139851739534));
#32189=CARTESIAN_POINT('Ctrl Pts',(23.9182257576785,10.5680285062335,-19.7948254980796));
#32190=CARTESIAN_POINT('Ctrl Pts',(24.4662138806868,10.4315004891655,-19.8668205194741));
#32191=CARTESIAN_POINT('Ctrl Pts',(25.0195744741822,10.3055778221167,-19.9326328666884));
#32192=CARTESIAN_POINT('Ctrl Pts',(25.4412458088222,10.2242864909386,-19.9749776253082));
#32193=CARTESIAN_POINT('Ctrl Pts',(25.9971983460992,10.131797107587,-20.0240850656221));
#32194=CARTESIAN_POINT('Ctrl Pts',(27.1157050405652,9.9818233225046,-20.102368552767));
#32195=CARTESIAN_POINT('Ctrl Pts',(28.1723100127449,9.93573708068023,-20.1222437541335));
#32196=CARTESIAN_POINT('Ctrl Pts',(29.0876106506766,9.89029022572783,-20.1449463132817));
#32197=CARTESIAN_POINT('Ctrl Pts',(29.4537207931442,9.87684873205162,-20.1517438988729));
#32198=CARTESIAN_POINT('Ctrl Pts',(30.1552759232946,9.86516345924736,-20.1576060163182));
#32199=CARTESIAN_POINT('Ctrl Pts',(31.368924127636,9.87263514017792,-20.1538463873917));
#32200=CARTESIAN_POINT('Ctrl Pts',(32.3594787154311,9.89702302165623,-20.1416711708076));
#32201=CARTESIAN_POINT('Ctrl Pts',(33.1581760188914,9.89696607979066,-20.1416983285705));
#32202=CARTESIAN_POINT('Ctrl Pts',(33.4913102145729,9.89696201382194,-20.1416998058431));
#32203=CARTESIAN_POINT('Ctrl Pts',(34.1477617736107,9.89695193052412,-20.1417043298969));
#32204=CARTESIAN_POINT('Ctrl Pts',(34.9726616332633,9.89692218573782,-20.1417171222835));
#32205=CARTESIAN_POINT('Ctrl Pts',(35.9599657908142,9.89690948638391,-20.1417226604566));
#32206=CARTESIAN_POINT('Ctrl Pts',(37.9357298104643,9.89689244880615,-20.1417300151411));
#32207=CARTESIAN_POINT('Ctrl Pts',(39.5833333333333,9.89680446003459,-20.1417681573542));
#32208=CARTESIAN_POINT('Ctrl Pts',(40.9,9.89680446003459,-20.1417681573542));
#32209=CARTESIAN_POINT('Ctrl Pts',(6.40644620858992,27.7818319413302,-12.3446157076951));
#32210=CARTESIAN_POINT('Ctrl Pts',(6.49686818484384,27.7146057723314,-12.4976194141968));
#32211=CARTESIAN_POINT('Ctrl Pts',(6.58771883172007,27.6462615383487,-12.6497754970258));
#32212=CARTESIAN_POINT('Ctrl Pts',(7.64885870107048,26.838967465877,-14.4089312086777));
#32213=CARTESIAN_POINT('Ctrl Pts',(8.64786699401838,25.9406999974137,-15.9309901815184));
#32214=CARTESIAN_POINT('Ctrl Pts',(10.7071344443812,24.1258468463739,-18.5841088194585));
#32215=CARTESIAN_POINT('Ctrl Pts',(11.7059636153277,23.1640388241121,-19.7351568023896));
#32216=CARTESIAN_POINT('Ctrl Pts',(13.7894167134297,21.32755345859,-21.7274097031724));
#32217=CARTESIAN_POINT('Ctrl Pts',(14.7964804448639,20.4089660621499,-22.5625068415354));
#32218=CARTESIAN_POINT('Ctrl Pts',(16.9150096963282,18.7347867871849,-23.9923642448819));
#32219=CARTESIAN_POINT('Ctrl Pts',(17.9356563974909,17.9376031564435,-24.568778311437));
#32220=CARTESIAN_POINT('Ctrl Pts',(19.3316378726114,17.0495061236355,-25.1942531765859));
#32221=CARTESIAN_POINT('Ctrl Pts',(19.8373783148988,16.733671277521,-25.4080883980549));
#32222=CARTESIAN_POINT('Ctrl Pts',(20.8986146451321,16.1088561234904,-25.8097110946141));
#32223=CARTESIAN_POINT('Ctrl Pts',(21.7322089233615,15.6790344990822,-26.0695581056351));
#32224=CARTESIAN_POINT('Ctrl Pts',(22.4452152218927,15.3644450466694,-26.2607608176433));
#32225=CARTESIAN_POINT('Ctrl Pts',(22.7053175952387,15.2520352575854,-26.3278633535721));
#32226=CARTESIAN_POINT('Ctrl Pts',(23.2405350109148,15.0319031635371,-26.456049557717));
#32227=CARTESIAN_POINT('Ctrl Pts',(23.7856351879594,14.8265027181049,-26.5714803865859));
#32228=CARTESIAN_POINT('Ctrl Pts',(24.3434088150882,14.6389049166987,-26.6748081507042));
#32229=CARTESIAN_POINT('Ctrl Pts',(24.9080926446007,14.4653482504621,-26.7695587595053));
#32230=CARTESIAN_POINT('Ctrl Pts',(25.3404979553364,14.3526452692475,-26.8308622015488));
#32231=CARTESIAN_POINT('Ctrl Pts',(25.9125607075504,14.2239063651395,-26.9021372597287));
#32232=CARTESIAN_POINT('Ctrl Pts',(27.0720378258712,14.0136986134135,-27.0165941086124));
#32233=CARTESIAN_POINT('Ctrl Pts',(28.1454151442859,13.9518646781024,-27.0445191043407));
#32234=CARTESIAN_POINT('Ctrl Pts',(29.0596751952944,13.890725520751,-27.0764264216485));
#32235=CARTESIAN_POINT('Ctrl Pts',(29.4376599373188,13.8719255145712,-27.0863532011149));
#32236=CARTESIAN_POINT('Ctrl Pts',(30.1519376760718,13.855954576287,-27.0947220176404));
#32237=CARTESIAN_POINT('Ctrl Pts',(31.3821999577689,13.8661782937677,-27.0893514143297));
#32238=CARTESIAN_POINT('Ctrl Pts',(32.3688386893657,13.8987881217581,-27.0723527225427));
#32239=CARTESIAN_POINT('Ctrl Pts',(33.1558986739574,13.8986675947835,-27.0724155351932));
#32240=CARTESIAN_POINT('Ctrl Pts',(33.49045038666,13.8986584195583,-27.072419804706));
#32241=CARTESIAN_POINT('Ctrl Pts',(34.1462287076184,13.8986367255002,-27.0724307945236));
#32242=CARTESIAN_POINT('Ctrl Pts',(34.9718350023128,13.8985720488061,-27.0724629552156));
#32243=CARTESIAN_POINT('Ctrl Pts',(35.9590682028415,13.8985445297567,-27.0724767217601));
#32244=CARTESIAN_POINT('Ctrl Pts',(37.9351039480424,13.8985075170899,-27.072495155898));
#32245=CARTESIAN_POINT('Ctrl Pts',(39.5833333333333,13.8983165657899,-27.0725904316243));
#32246=CARTESIAN_POINT('Ctrl Pts',(40.9,13.8983165657899,-27.0725904316243));
#32247=CARTESIAN_POINT('Ctrl Pts',(6.37427268165564,32.0290848932163,-14.0406695266741));
#32248=CARTESIAN_POINT('Ctrl Pts',(6.46448755772838,31.9528098065586,-14.2166050753401));
#32249=CARTESIAN_POINT('Ctrl Pts',(6.55512327887565,31.8752581000468,-14.3915605358513));
#32250=CARTESIAN_POINT('Ctrl Pts',(7.61410360785656,30.958672886913,-16.4151695040826));
#32251=CARTESIAN_POINT('Ctrl Pts',(8.61142775869687,29.9361952854453,-18.1677152487792));
#32252=CARTESIAN_POINT('Ctrl Pts',(10.6634825022472,27.8730682250752,-21.2183968262284));
#32253=CARTESIAN_POINT('Ctrl Pts',(11.6607542873627,26.7761583709751,-22.5462154536683));
#32254=CARTESIAN_POINT('Ctrl Pts',(13.7353039743977,24.6873364683673,-24.8383185913233));
#32255=CARTESIAN_POINT('Ctrl Pts',(14.7402095633116,23.6392130729629,-25.802985911944));
#32256=CARTESIAN_POINT('Ctrl Pts',(16.8490881066137,21.733995182915,-27.450307490631));
#32257=CARTESIAN_POINT('Ctrl Pts',(17.8672038783315,20.8239061433235,-28.1175362426871));
#32258=CARTESIAN_POINT('Ctrl Pts',(19.2585933984997,19.811022849419,-28.8404836901117));
#32259=CARTESIAN_POINT('Ctrl Pts',(19.7636418533908,19.4499572035579,-29.0884650342026));
#32260=CARTESIAN_POINT('Ctrl Pts',(20.8231816497994,18.7357747989967,-29.5540603372584));
#32261=CARTESIAN_POINT('Ctrl Pts',(21.6568670511735,18.2431916560479,-29.8562628482713));
#32262=CARTESIAN_POINT('Ctrl Pts',(22.3720072062877,17.8815051531587,-30.0792593376712));
#32263=CARTESIAN_POINT('Ctrl Pts',(22.6326824787813,17.7523977438431,-30.1574913312728));
#32264=CARTESIAN_POINT('Ctrl Pts',(23.1697036949937,17.4991937768336,-30.3071564102286));
#32265=CARTESIAN_POINT('Ctrl Pts',(23.7174377716562,17.2625030946595,-30.4422233412819));
#32266=CARTESIAN_POINT('Ctrl Pts',(24.2790946262572,17.0457855087881,-30.5634410393029));
#32267=CARTESIAN_POINT('Ctrl Pts',(24.8485847331463,16.8449230908939,-30.6748008187179));
#32268=CARTESIAN_POINT('Ctrl Pts',(25.2859632686137,16.714000734413,-30.7471152582869));
#32269=CARTESIAN_POINT('Ctrl Pts',(25.8659001690755,16.5640760155963,-30.8313513860032));
#32270=CARTESIAN_POINT('Ctrl Pts',(27.0467877055032,16.3181083484214,-30.9672841404844));
#32271=CARTESIAN_POINT('Ctrl Pts',(28.1301993946288,16.2470842981322,-30.9999203594232));
#32272=CARTESIAN_POINT('Ctrl Pts',(29.0438132065911,16.1769735529556,-31.0370949113971));
#32273=CARTESIAN_POINT('Ctrl Pts',(29.4285323170642,16.1549555741443,-31.0489002942269));
#32274=CARTESIAN_POINT('Ctrl Pts',(30.1500796604944,16.1364761766636,-31.0587367393328));
#32275=CARTESIAN_POINT('Ctrl Pts',(31.3898224001987,16.1483068856791,-31.0524272220083));
#32276=CARTESIAN_POINT('Ctrl Pts',(32.3742147772173,16.1855693458549,-31.0327017051641));
#32277=CARTESIAN_POINT('Ctrl Pts',(33.1546196294426,16.1853991323255,-31.0327939306214));
#32278=CARTESIAN_POINT('Ctrl Pts',(33.4899805045662,16.1853856345319,-31.0328008093452));
#32279=CARTESIAN_POINT('Ctrl Pts',(34.1453728987309,16.1853546639145,-31.0328173216774));
#32280=CARTESIAN_POINT('Ctrl Pts',(34.9713787068036,16.1852616946182,-31.0328663827335));
#32281=CARTESIAN_POINT('Ctrl Pts',(35.9585696612047,16.1852222245757,-31.0328872804502));
#32282=CARTESIAN_POINT('Ctrl Pts',(37.9347583211501,16.1851690519236,-31.0329153648958));
#32283=CARTESIAN_POINT('Ctrl Pts',(39.5833333333333,16.1848949119358,-31.0330603026358));
#32284=CARTESIAN_POINT('Ctrl Pts',(40.9,16.1848949119358,-31.0330603026358));
#32285=CARTESIAN_POINT('',(40.9,15.1839076262002,-29.2992994660114));
#32286=CARTESIAN_POINT('Ctrl Pts',(40.9,15.1839076262002,-29.2992994660114));
#32287=CARTESIAN_POINT('Ctrl Pts',(40.9,15.4341550287793,-29.7327406817405));
#32288=CARTESIAN_POINT('Ctrl Pts',(40.9,15.6844024313583,-30.1661818974696));
#32289=CARTESIAN_POINT('Ctrl Pts',(40.9,15.9346498339374,-30.5996231131986));
#32290=CARTESIAN_POINT('',(38.,15.1839076262003,-29.2992994660114));
#32291=CARTESIAN_POINT('Ctrl Pts',(38.,15.1839076262003,-29.2992994660114));
#32292=CARTESIAN_POINT('Ctrl Pts',(38.9666666666667,15.1839076262003,-29.2992994660114));
#32293=CARTESIAN_POINT('Ctrl Pts',(39.9333333333333,15.1839076262003,-29.2992994660114));
#32294=CARTESIAN_POINT('Ctrl Pts',(40.9,15.1839076262003,-29.2992994660114));
#32295=CARTESIAN_POINT('Ctrl Pts',(37.4974382384971,14.8838038109906,-28.7790269720419));
#32296=CARTESIAN_POINT('Ctrl Pts',(37.6645213547145,14.9840691120819,-28.9527098777878));
#32297=CARTESIAN_POINT('Ctrl Pts',(37.8313739960415,15.0841847150559,-29.1261374112003));
#32298=CARTESIAN_POINT('Ctrl Pts',(37.9978889629903,15.1840905833949,-29.2992044501375));
#32299=CARTESIAN_POINT('',(6.9,27.0393531365015,-12.9951291628659));
#32300=CARTESIAN_POINT('Ctrl Pts',(6.9,27.0393531365015,-12.9951291628659));
#32301=CARTESIAN_POINT('Ctrl Pts',(6.9,24.649274247254,-11.9174419758914));
#32302=CARTESIAN_POINT('Ctrl Pts',(6.90000000000115,22.230729924082,-10.8339866674746));
#32303=CARTESIAN_POINT('Ctrl Pts',(6.90000000000115,16.7584145047598,-8.41000082059025));
#32304=CARTESIAN_POINT('Ctrl Pts',(6.9,13.1312177506378,-6.82522008706164));
#32305=CARTESIAN_POINT('Ctrl Pts',(6.9,9.63452070648529,-5.36789542693313));
#32306=CARTESIAN_POINT('',(22.9245129145126,15.8853026165582,-27.5141512254857));
#32307=CARTESIAN_POINT('Ctrl Pts',(22.9245129145126,15.8853026165582,-27.5141512254857));
#32308=CARTESIAN_POINT('Ctrl Pts',(22.7202811020963,15.9355315703924,-27.405303612937));
#32309=CARTESIAN_POINT('Ctrl Pts',(22.5089075447093,15.9922246435191,-27.2924652433825));
#32310=CARTESIAN_POINT('Ctrl Pts',(22.2913349439917,16.0558281873747,-27.1762359097413));
#32311=CARTESIAN_POINT('Ctrl Pts',(21.4451770585294,16.3031876434794,-26.7242103933933));
#32312=CARTESIAN_POINT('Ctrl Pts',(20.5220951556672,16.6965145338604,-26.2108400614944));
#32313=CARTESIAN_POINT('Ctrl Pts',(19.7671428819544,17.0753616782141,-25.7770859372682));
#32314=CARTESIAN_POINT('Ctrl Pts',(19.5194773058395,17.1996442316058,-25.6347908958341));
#32315=CARTESIAN_POINT('Ctrl Pts',(19.2865716386092,17.3225345039426,-25.4994131575073));
#32316=CARTESIAN_POINT('Ctrl Pts',(19.0728538401323,17.4387046858284,-25.3740784559106));
#32317=CARTESIAN_POINT('Ctrl Pts',(18.7028555998036,17.6398239336528,-25.1570931632801));
#32318=CARTESIAN_POINT('Ctrl Pts',(18.4144703596236,17.8106758656204,-24.9815167506412));
#32319=CARTESIAN_POINT('Ctrl Pts',(18.0642874871539,18.0298340093773,-24.7606238748753));
#32320=CARTESIAN_POINT('Ctrl Pts',(17.4420927116722,18.419227845484,-24.3681478172275));
#32321=CARTESIAN_POINT('Ctrl Pts',(16.7224564418219,18.9163953124274,-23.8866996305776));
#32322=CARTESIAN_POINT('Ctrl Pts',(15.9202806616111,19.5075155171573,-23.2999769887242));
#32323=CARTESIAN_POINT('Ctrl Pts',(15.409052983452,19.8842371999007,-22.926057878577));
#32324=CARTESIAN_POINT('Ctrl Pts',(14.8739602945718,20.3065653819879,-22.5035099772299));
#32325=CARTESIAN_POINT('Ctrl Pts',(14.316979433116,20.764045054618,-22.0244589523046));
#32326=CARTESIAN_POINT('Ctrl Pts',(13.886420676284,21.1176871503423,-21.6541417151704));
#32327=CARTESIAN_POINT('Ctrl Pts',(13.3867890027807,21.5394320189423,-21.2019814327446));
#32328=CARTESIAN_POINT('Ctrl Pts',(12.8146824059514,22.0238946695559,-20.6456427149589));
#32329=CARTESIAN_POINT('Ctrl Pts',(12.2526665517594,22.499812430193,-20.0991166279862));
#32330=CARTESIAN_POINT('Ctrl Pts',(11.6379478462803,23.0419154065947,-19.4470356343899));
#32331=CARTESIAN_POINT('Ctrl Pts',(10.9739250490307,23.6265354530561,-18.668913747699));
#32332=CARTESIAN_POINT('Ctrl Pts',(10.5683455447962,23.9836164291783,-18.1936434853747));
#32333=CARTESIAN_POINT('Ctrl Pts',(10.1437415406955,24.3558958755273,-17.6694303965612));
#32334=CARTESIAN_POINT('Ctrl Pts',(9.74137929176525,24.6998029803349,-17.1528053766524));
#32335=CARTESIAN_POINT('Ctrl Pts',(8.72285779294233,25.5703537856744,-15.8450442956717));
#32336=CARTESIAN_POINT('Ctrl Pts',(7.81323138778195,26.3485431508901,-14.4751178145147));
#32337=CARTESIAN_POINT('Ctrl Pts',(6.9,27.0393531365015,-12.9951291628659));
#32338=CARTESIAN_POINT('Ctrl Pts',(30.5,16.1402285275843,-31.0562879796886));
#32339=CARTESIAN_POINT('Ctrl Pts',(29.9560179420817,16.0158030554221,-30.8470467059701));
#32340=CARTESIAN_POINT('Ctrl Pts',(29.4152668325132,15.9055856438303,-30.6299015220344));
#32341=CARTESIAN_POINT('Ctrl Pts',(28.8740459957565,15.8236145009995,-30.3967092920472));
#32342=CARTESIAN_POINT('Ctrl Pts',(28.353527792344,15.7447788961961,-30.1724370682909));
#32343=CARTESIAN_POINT('Ctrl Pts',(27.8179515912467,15.65999396651,-29.9423746730404));
#32344=CARTESIAN_POINT('Ctrl Pts',(27.2695051149491,15.5981844167478,-29.6962958928787));
#32345=CARTESIAN_POINT('Ctrl Pts',(26.9554553615883,15.5627912203338,-29.5553870101399));
#32346=CARTESIAN_POINT('Ctrl Pts',(26.6378099296971,15.535020897066,-29.4095747645068));
#32347=CARTESIAN_POINT('Ctrl Pts',(26.3179304017917,15.520523503095,-29.2578762499931));
#32348=CARTESIAN_POINT('Ctrl Pts',(26.1078196745982,15.5110009868852,-29.1582340959378));
#32349=CARTESIAN_POINT('Ctrl Pts',(25.8967402232745,15.507207179043,-29.0560612282453));
#32350=CARTESIAN_POINT('Ctrl Pts',(25.6850706236774,15.5107635234098,-28.9510881944939));
#32351=CARTESIAN_POINT('Ctrl Pts',(25.6562210027417,15.5112482372614,-28.9367808388889));
#32352=CARTESIAN_POINT('Ctrl Pts',(25.6277737638215,15.5118582602787,-28.9226278510966));
#32353=CARTESIAN_POINT('Ctrl Pts',(25.5983858063598,15.5126342200129,-28.9079571471847));
#32354=CARTESIAN_POINT('Ctrl Pts',(25.1249357452756,15.5251351971226,-28.6716070819486));
#32355=CARTESIAN_POINT('Ctrl Pts',(24.1510084067019,15.583657222894,-28.1678256190434));
#32356=CARTESIAN_POINT('Ctrl Pts',(22.9245129145126,15.8853026165582,-27.5141512254857));
#32357=CARTESIAN_POINT('Origin',(40.65,0.,0.));
#32358=CARTESIAN_POINT('',(40.4,31.0330398077868,-16.1848830792292));
#32359=CARTESIAN_POINT('',(40.9,30.5996231131986,-15.9346498339374));
#32360=CARTESIAN_POINT('Ctrl Pts',(40.4,31.0330398077868,-16.1848830792292));
#32361=CARTESIAN_POINT('Ctrl Pts',(40.5666590138513,30.888576136327,-16.1014769396238));
#32362=CARTESIAN_POINT('Ctrl Pts',(40.7333430451333,30.7440888805157,-16.0180571835867));
#32363=CARTESIAN_POINT('Ctrl Pts',(40.9,30.5996231131986,-15.9346498339374));
#32364=CARTESIAN_POINT('',(40.9,29.0996231131986,-18.5327260452908));
#32365=CARTESIAN_POINT('Origin',(40.9,0.,0.));
#32366=CARTESIAN_POINT('',(40.4,29.5330398077868,-18.7829592905825));
#32367=CARTESIAN_POINT('Ctrl Pts',(40.9,29.0996231131986,-18.5327260452908));
#32368=CARTESIAN_POINT('Ctrl Pts',(40.7333430447098,29.2440888808829,-18.616133395152));
#32369=CARTESIAN_POINT('Ctrl Pts',(40.566659013253,29.3885761368456,-18.6995531512765));
#32370=CARTESIAN_POINT('Ctrl Pts',(40.4,29.5330398077868,-18.7829592905825));
#32371=CARTESIAN_POINT('Origin',(40.4,0.,0.));
#32372=CARTESIAN_POINT('Origin',(35.7,0.,0.));
#32373=CARTESIAN_POINT('',(30.5,29.5059919176187,-18.8254200738635));
#32374=CARTESIAN_POINT('Ctrl Pts',(40.3998805977094,29.5330468723882,-18.7829479019245));
#32375=CARTESIAN_POINT('Ctrl Pts',(39.2493532038211,29.5330781202017,-18.7828975281219));
#32376=CARTESIAN_POINT('Ctrl Pts',(38.0972325173324,29.5332042421652,-18.7826942098493));
#32377=CARTESIAN_POINT('Ctrl Pts',(36.9466403233752,29.5332467931519,-18.7826256101695));
#32378=CARTESIAN_POINT('Ctrl Pts',(36.7453942973752,29.533254235595,-18.7826136116412));
#32379=CARTESIAN_POINT('Ctrl Pts',(36.5441950314395,29.5332591214118,-18.7826057344612));
#32380=CARTESIAN_POINT('Ctrl Pts',(36.3429831482115,29.5332638326534,-18.7825981392431));
#32381=CARTESIAN_POINT('Ctrl Pts',(36.2103627229287,29.533266937872,-18.7825931331717));
#32382=CARTESIAN_POINT('Ctrl Pts',(36.0823539050873,29.5332699079824,-18.7825884046388));
#32383=CARTESIAN_POINT('Ctrl Pts',(35.9587472612551,29.533273304022,-18.7825830315924));
#32384=CARTESIAN_POINT('Ctrl Pts',(35.7554552092513,29.5332788893841,-18.7825741947079));
#32385=CARTESIAN_POINT('Ctrl Pts',(35.5640774641711,29.5332855100166,-18.78256380265));
#32386=CARTESIAN_POINT('Ctrl Pts',(35.3838244599967,29.5332919882698,-18.7825536727525));
#32387=CARTESIAN_POINT('Ctrl Pts',(35.2391029659044,29.5332971895284,-18.7825455396624));
#32388=CARTESIAN_POINT('Ctrl Pts',(35.1015509582766,29.5333023181163,-18.7825375448068));
#32389=CARTESIAN_POINT('Ctrl Pts',(34.9707359993239,29.5333070397951,-18.7825301856736));
#32390=CARTESIAN_POINT('Ctrl Pts',(34.857898178191,29.533311112601,-18.7825238378632));
#32391=CARTESIAN_POINT('Ctrl Pts',(34.7500670454289,29.5333148977242,-18.7825179389498));
#32392=CARTESIAN_POINT('Ctrl Pts',(34.6468496335934,29.5333184739771,-18.7825123391461));
#32393=CARTESIAN_POINT('Ctrl Pts',(34.5887227637577,29.5333204879433,-18.7825091856174));
#32394=CARTESIAN_POINT('Ctrl Pts',(34.5320601650214,29.5333224349754,-18.7825061280289));
#32395=CARTESIAN_POINT('Ctrl Pts',(34.4767987085013,29.5333243245899,-18.7825031467392));
#32396=CARTESIAN_POINT('Ctrl Pts',(34.3959515550964,29.5333270890838,-18.7824987851317));
#32397=CARTESIAN_POINT('Ctrl Pts',(34.3181086378962,29.533329735084,-18.7824945795527));
#32398=CARTESIAN_POINT('Ctrl Pts',(34.2432236356273,29.5333323757695,-18.7824903288468));
#32399=CARTESIAN_POINT('Ctrl Pts',(34.162267530415,29.5333352305416,-18.7824857335262));
#32400=CARTESIAN_POINT('Ctrl Pts',(34.0847679659788,29.5333380786013,-18.7824810862876));
#32401=CARTESIAN_POINT('Ctrl Pts',(34.0106064145146,29.5333409984257,-18.7824762390846));
#32402=CARTESIAN_POINT('Ctrl Pts',(34.0011740963656,29.5333413697867,-18.7824756225878));
#32403=CARTESIAN_POINT('Ctrl Pts',(33.9917957065319,29.5333417422356,-18.7824750029764));
#32404=CARTESIAN_POINT('Ctrl Pts',(33.982470944213,29.5333421158732,-18.7824743800456));
#32405=CARTESIAN_POINT('Ctrl Pts',(33.9223617768104,29.533344524411,-18.7824703645173));
#32406=CARTESIAN_POINT('Ctrl Pts',(33.8644761963965,29.5333469783619,-18.7824662176402));
#32407=CARTESIAN_POINT('Ctrl Pts',(33.8085662291515,29.5333493560495,-18.7824621300573));
#32408=CARTESIAN_POINT('Ctrl Pts',(33.7474237015737,29.5333519562626,-18.7824576599214));
#32409=CARTESIAN_POINT('Ctrl Pts',(33.6886441629424,29.5333544654644,-18.7824532603738));
#32410=CARTESIAN_POINT('Ctrl Pts',(33.6319696815246,29.5333567795573,-18.7824490897141));
#32411=CARTESIAN_POINT('Ctrl Pts',(33.5826925637263,29.5333587916063,-18.7824454634244));
#32412=CARTESIAN_POINT('Ctrl Pts',(33.5350083428651,29.5333606573844,-18.7824420081377));
#32413=CARTESIAN_POINT('Ctrl Pts',(33.4887791610293,29.5333623350577,-18.7824387839385));
#32414=CARTESIAN_POINT('Ctrl Pts',(33.4518540159975,29.5333636750843,-18.7824362086382));
#32415=CARTESIAN_POINT('Ctrl Pts',(33.415863041895,29.5333649012575,-18.7824337706412));
#32416=CARTESIAN_POINT('Ctrl Pts',(33.3809178973935,29.5333661853238,-18.7824311829815));
#32417=CARTESIAN_POINT('Ctrl Pts',(33.3430135141806,29.533367578128,-18.7824283761925));
#32418=CARTESIAN_POINT('Ctrl Pts',(33.3063394413794,29.533369038868,-18.782425393611));
#32419=CARTESIAN_POINT('Ctrl Pts',(33.2709744549996,29.5333707165148,-18.782421984424));
#32420=CARTESIAN_POINT('Ctrl Pts',(33.2337091833701,29.5333724843074,-18.7824183920493));
#32421=CARTESIAN_POINT('Ctrl Pts',(33.1978968817055,29.5333744922841,-18.7824143270743));
#32422=CARTESIAN_POINT('Ctrl Pts',(33.1635680440121,29.5333768470907,-18.7824096072585));
#32423=CARTESIAN_POINT('Ctrl Pts',(33.1258517952633,29.5333794342587,-18.7824044217132));
#32424=CARTESIAN_POINT('Ctrl Pts',(33.0899258346456,29.5333824396273,-18.7823984464624));
#32425=CARTESIAN_POINT('Ctrl Pts',(33.0557653924634,29.5333859335647,-18.7823915566589));
#32426=CARTESIAN_POINT('Ctrl Pts',(33.0368719876719,29.5333878659862,-18.7823877460571));
#32427=CARTESIAN_POINT('Ctrl Pts',(33.0185175726606,29.5333899466911,-18.7823836576174));
#32428=CARTESIAN_POINT('Ctrl Pts',(33.0006913488414,29.533392180445,-18.7823792819583));
#32429=CARTESIAN_POINT('Ctrl Pts',(32.9433364917301,29.5333993674205,-18.782365203525));
#32430=CARTESIAN_POINT('Ctrl Pts',(32.8893232017973,29.5332829792511,-18.7825476275078));
#32431=CARTESIAN_POINT('Ctrl Pts',(32.8382230275391,29.5330947066423,-18.7828441878577));
#32432=CARTESIAN_POINT('Ctrl Pts',(32.7810653123534,29.5328841157333,-18.7831759032042));
#32433=CARTESIAN_POINT('Ctrl Pts',(32.7275524566167,29.5325833908839,-18.783650731462));
#32434=CARTESIAN_POINT('Ctrl Pts',(32.6770430178925,29.5322363386496,-18.7841988325575));
#32435=CARTESIAN_POINT('Ctrl Pts',(32.6227203150995,29.5318630853359,-18.7847883131311));
#32436=CARTESIAN_POINT('Ctrl Pts',(32.5718714570969,29.5314358212364,-18.7854632228815));
#32437=CARTESIAN_POINT('Ctrl Pts',(32.5236533104246,29.5309832901802,-18.7861776881423));
#32438=CARTESIAN_POINT('Ctrl Pts',(32.4718100170281,29.5304967368401,-18.7869458684789));
#32439=CARTESIAN_POINT('Ctrl Pts',(32.4230076636094,29.5299805545515,-18.787760443828));
#32440=CARTESIAN_POINT('Ctrl Pts',(32.3761512171914,29.5294487411366,-18.7885990065863));
#32441=CARTESIAN_POINT('Ctrl Pts',(32.3248096591116,29.5288660223985,-18.7895178367975));
#32442=CARTESIAN_POINT('Ctrl Pts',(32.2758043950059,29.5282641700435,-18.7904660498706));
#32443=CARTESIAN_POINT('Ctrl Pts',(32.2276418899913,29.5276429422444,-18.7914438965952));
#32444=CARTESIAN_POINT('Ctrl Pts',(32.1780484879523,29.5270032579093,-18.7924507949227));
#32445=CARTESIAN_POINT('Ctrl Pts',(32.1293485207493,29.5263425803878,-18.7934898288216));
#32446=CARTESIAN_POINT('Ctrl Pts',(32.0798596721981,29.5256485080419,-18.7945806299647));
#32447=CARTESIAN_POINT('Ctrl Pts',(32.0310319727761,29.5249637081956,-18.795656858487));
#32448=CARTESIAN_POINT('Ctrl Pts',(31.9814363679965,29.5242459918055,-18.7967841293548));
#32449=CARTESIAN_POINT('Ctrl Pts',(31.9294088356335,29.5234781937103,-18.7979897024647));
#32450=CARTESIAN_POINT('Ctrl Pts',(31.8980169361542,29.5230149266759,-18.7987171102076));
#32451=CARTESIAN_POINT('Ctrl Pts',(31.8657387723059,29.5225333465274,-18.7994731533957));
#32452=CARTESIAN_POINT('Ctrl Pts',(31.832199550689,29.5220297162343,-18.8002637757389));
#32453=CARTESIAN_POINT('Ctrl Pts',(31.7313430769547,29.5205152393625,-18.8026412722264));
#32454=CARTESIAN_POINT('Ctrl Pts',(31.6280303063014,29.5189339810999,-18.8051208616254));
#32455=CARTESIAN_POINT('Ctrl Pts',(31.5230436306591,29.5173797888791,-18.8075570016555));
#32456=CARTESIAN_POINT('Ctrl Pts',(31.4165412834615,29.5158031590972,-18.8100283117502));
#32457=CARTESIAN_POINT('Ctrl Pts',(31.308316179973,29.514255268772,-18.8124534992281));
#32458=CARTESIAN_POINT('Ctrl Pts',(31.1992361907457,29.5128402023346,-18.8146708525442));
#32459=CARTESIAN_POINT('Ctrl Pts',(31.1417800802777,29.5120948391005,-18.815838807345));
#32460=CARTESIAN_POINT('Ctrl Pts',(31.0840876501121,29.5113863470817,-18.8169490671259));
#32461=CARTESIAN_POINT('Ctrl Pts',(31.0262914624598,29.5107292754507,-18.8179790464239));
#32462=CARTESIAN_POINT('Ctrl Pts',(30.9238422517516,29.5095645538192,-18.819804782176));
#32463=CARTESIAN_POINT('Ctrl Pts',(30.8210652493991,29.508562595471,-18.8213763518942));
#32464=CARTESIAN_POINT('Ctrl Pts',(30.7187655025437,29.5078108353848,-18.822555692875));
#32465=CARTESIAN_POINT('Ctrl Pts',(30.6466529304573,29.5072809088202,-18.8233870274004));
#32466=CARTESIAN_POINT('Ctrl Pts',(30.574778287816,29.5068750511295,-18.8240238694395));
#32467=CARTESIAN_POINT('Ctrl Pts',(30.5034323931867,29.5066169475222,-18.8244289958229));
#32468=CARTESIAN_POINT('Ctrl Pts',(30.500673116597,29.5066069654589,-18.8244446639388));
#32469=CARTESIAN_POINT('Ctrl Pts',(30.497914631651,29.5065972035123,-18.8244599868899));
#32470=CARTESIAN_POINT('Ctrl Pts',(30.4951569508121,29.5065876629555,-18.8244749626662));
#32471=CARTESIAN_POINT('',(30.5,31.0097594187194,-16.229443021655));
#32472=CARTESIAN_POINT('Origin',(30.5,0.,0.));
#32473=CARTESIAN_POINT('Ctrl Pts',(30.504907630814,31.0091238687318,-16.2304573503026));
#32474=CARTESIAN_POINT('Ctrl Pts',(30.5973062294344,31.0094328533547,-16.2298682766552));
#32475=CARTESIAN_POINT('Ctrl Pts',(30.689059158586,31.0099692677028,-16.2288427503286));
#32476=CARTESIAN_POINT('Ctrl Pts',(30.7806364364919,31.0106763092383,-16.2274919709621));
#32477=CARTESIAN_POINT('Ctrl Pts',(30.8441456090292,31.0111666450935,-16.2265552005993));
#32478=CARTESIAN_POINT('Ctrl Pts',(30.9075713010183,31.0117394593183,-16.2254611740684));
#32479=CARTESIAN_POINT('Ctrl Pts',(30.9710816356703,31.0123798375508,-16.2242390174924));
#32480=CARTESIAN_POINT('Ctrl Pts',(31.0734991469994,31.013412519007,-16.2222681534487));
#32481=CARTESIAN_POINT('Ctrl Pts',(31.1761345288067,31.0146205155167,-16.2199648111636));
#32482=CARTESIAN_POINT('Ctrl Pts',(31.2798100568469,31.0159286966544,-16.2174702047238));
#32483=CARTESIAN_POINT('Ctrl Pts',(31.3828326297147,31.0172286387828,-16.2149913094765));
#32484=CARTESIAN_POINT('Ctrl Pts',(31.4868822244369,31.0186283615542,-16.2123218973813));
#32485=CARTESIAN_POINT('Ctrl Pts',(31.5928140565652,31.020057669606,-16.2095937955789));
#32486=CARTESIAN_POINT('Ctrl Pts',(31.6516194621143,31.0208511142011,-16.2080793581369));
#32487=CARTESIAN_POINT('Ctrl Pts',(31.7110057676108,31.0216536678951,-16.2065468518027));
#32488=CARTESIAN_POINT('Ctrl Pts',(31.7711259776529,31.0224523036437,-16.2050208141949));
#32489=CARTESIAN_POINT('Ctrl Pts',(31.8409078613426,31.0233792848848,-16.2032495333099));
#32490=CARTESIAN_POINT('Ctrl Pts',(31.9056298453963,31.0242198767433,-16.2016434584277));
#32491=CARTESIAN_POINT('Ctrl Pts',(31.9658749467864,31.0249744961546,-16.2002018139142));
#32492=CARTESIAN_POINT('Ctrl Pts',(32.0341046687228,31.0258291295008,-16.1985691001829));
#32493=CARTESIAN_POINT('Ctrl Pts',(32.096591829894,31.026574015819,-16.1971462744691));
#32494=CARTESIAN_POINT('Ctrl Pts',(32.1542461945013,31.0272242625029,-16.1959042389539));
#32495=CARTESIAN_POINT('Ctrl Pts',(32.215166595352,31.0279113447196,-16.1945918439258));
#32496=CARTESIAN_POINT('Ctrl Pts',(32.2706916712563,31.0284933558527,-16.1934801514051));
#32497=CARTESIAN_POINT('Ctrl Pts',(32.3219582775163,31.0289937114781,-16.1925241206212));
#32498=CARTESIAN_POINT('Ctrl Pts',(32.3761916324787,31.0295230221975,-16.1915127652646));
#32499=CARTESIAN_POINT('Ctrl Pts',(32.4256599862246,31.0299613681536,-16.1906748064835));
#32500=CARTESIAN_POINT('Ctrl Pts',(32.4717693483811,31.0303343957023,-16.1899610544418));
#32501=CARTESIAN_POINT('Ctrl Pts',(32.5215332003089,31.0307369882959,-16.1891907325537));
#32502=CARTESIAN_POINT('Ctrl Pts',(32.5673849287969,31.0310638203075,-16.1885644631731));
#32503=CARTESIAN_POINT('Ctrl Pts',(32.6111519417734,31.0313387615313,-16.1880367365758));
#32504=CARTESIAN_POINT('Ctrl Pts',(32.6551741210766,31.0316153056916,-16.1875059332764));
#32505=CARTESIAN_POINT('Ctrl Pts',(32.6970878717853,31.0318395012596,-16.1870745377529));
#32506=CARTESIAN_POINT('Ctrl Pts',(32.7388013470543,31.0320241553173,-16.1867185738399));
#32507=CARTESIAN_POINT('Ctrl Pts',(32.7801521457897,31.0322072039059,-16.1863657048443));
#32508=CARTESIAN_POINT('Ctrl Pts',(32.8213062770032,31.0323516104907,-16.1860865454659));
#32509=CARTESIAN_POINT('Ctrl Pts',(32.8641640035307,31.0324560971769,-16.1858844594634));
#32510=CARTESIAN_POINT('Ctrl Pts',(32.9038200784545,31.0325527782703,-16.1856974701314));
#32511=CARTESIAN_POINT('Ctrl Pts',(32.9449347772916,31.032615465502,-16.1855761117061));
#32512=CARTESIAN_POINT('Ctrl Pts',(32.9890474705834,31.0326287580452,-16.1855509840874));
#32513=CARTESIAN_POINT('Ctrl Pts',(32.9926089293383,31.0326298312249,-16.1855489553974));
#32514=CARTESIAN_POINT('Ctrl Pts',(32.9961899495414,31.0326305730127,-16.1855475722577));
#32515=CARTESIAN_POINT('Ctrl Pts',(32.9997913521115,31.0326309700538,-16.1855468609619));
#32516=CARTESIAN_POINT('Ctrl Pts',(33.0362292496772,31.0326349871946,-16.1855396642873));
#32517=CARTESIAN_POINT('Ctrl Pts',(33.074092292112,31.0326386992185,-16.1855331333215));
#32518=CARTESIAN_POINT('Ctrl Pts',(33.1141439185631,31.0326422490868,-16.1855273500631));
#32519=CARTESIAN_POINT('Ctrl Pts',(33.2461674547434,31.0326539506383,-16.1855082865123));
#32520=CARTESIAN_POINT('Ctrl Pts',(33.3721931286569,31.0326588963953,-16.1855003220479));
#32521=CARTESIAN_POINT('Ctrl Pts',(33.4993879207449,31.0326635427516,-16.185492813855));
#32522=CARTESIAN_POINT('Ctrl Pts',(33.6627849160625,31.0326695115547,-16.1854831686789));
#32523=CARTESIAN_POINT('Ctrl Pts',(33.828111247454,31.0326749862723,-16.1854742764644));
#32524=CARTESIAN_POINT('Ctrl Pts',(33.9929845306744,31.0326833946005,-16.1854606405094));
#32525=CARTESIAN_POINT('Ctrl Pts',(34.3227310971152,31.0327002112569,-16.1854333685993));
#32526=CARTESIAN_POINT('Ctrl Pts',(34.6506654708719,31.032728762356,-16.185387121727));
#32527=CARTESIAN_POINT('Ctrl Pts',(34.979269363621,31.032748004237,-16.1853559472169));
#32528=CARTESIAN_POINT('Ctrl Pts',(35.3078732563701,31.0327672461181,-16.1853247727068));
#32529=CARTESIAN_POINT('Ctrl Pts',(35.6371466681116,31.032777178781,-16.185308670559));
#32530=CARTESIAN_POINT('Ctrl Pts',(35.9662682695208,31.0327855310262,-16.1852951338217));
#32531=CARTESIAN_POINT('Ctrl Pts',(36.29538987093,31.0327938832714,-16.1852815970843));
#32532=CARTESIAN_POINT('Ctrl Pts',(36.6243596620069,31.0328006550988,-16.1852706257574));
#32533=CARTESIAN_POINT('Ctrl Pts',(36.9532592751492,31.0328145551759,-16.185248102247));
#32534=CARTESIAN_POINT('Ctrl Pts',(38.102326278026,31.0328631174705,-16.1851694125146));
#32535=CARTESIAN_POINT('Ctrl Pts',(39.2505367075415,31.0329986853002,-16.184949719878));
#32536=CARTESIAN_POINT('Ctrl Pts',(40.4000986012038,31.0330322281526,-16.1848953623403));
#32537=CARTESIAN_POINT('Ctrl Pts',(6.89999999997365,11.0276873985587,0.168526548676475));
#32538=CARTESIAN_POINT('Ctrl Pts',(6.99168932310453,11.0290491215116,0.107121039164007));
#32539=CARTESIAN_POINT('Ctrl Pts',(7.08383940291242,11.0299018391088,0.0458098125994608));
#32540=CARTESIAN_POINT('Ctrl Pts',(8.15761824498006,11.0337651740187,-0.664186592400576));
#32541=CARTESIAN_POINT('Ctrl Pts',(9.16607857437499,10.9699676285446,-1.30870352701556));
#32542=CARTESIAN_POINT('Ctrl Pts',(11.2535171643192,10.77603305676,-2.47376106241928));
#32543=CARTESIAN_POINT('Ctrl Pts',(12.2576790632369,10.6330057282435,-3.00237606292525));
#32544=CARTESIAN_POINT('Ctrl Pts',(14.3563663857894,10.3307260661656,-3.944470058834));
#32545=CARTESIAN_POINT('Ctrl Pts',(15.3658129161116,10.1540434041659,-4.36032593857962));
#32546=CARTESIAN_POINT('Ctrl Pts',(17.4727193021212,9.82334300624284,-5.08193366885832));
#32547=CARTESIAN_POINT('Ctrl Pts',(18.4888802671462,9.6488422591121,-5.39169279079136));
#32548=CARTESIAN_POINT('Ctrl Pts',(19.8473882183426,9.45778984314828,-5.72385817850078));
#32549=CARTESIAN_POINT('Ctrl Pts',(20.3451395577184,9.38741838105895,-5.84063156394592));
#32550=CARTESIAN_POINT('Ctrl Pts',(21.119864121141,9.28201599203951,-6.00690103675049));
#32551=CARTESIAN_POINT('Ctrl Pts',(21.9116430735678,9.18172875488038,-6.15921075032183));
#32552=CARTESIAN_POINT('Ctrl Pts',(22.4533884343746,9.12054551137776,-6.25063668203688));
#32553=CARTESIAN_POINT('Ctrl Pts',(22.8546099577479,9.07881438233612,-6.31320896750581));
#32554=CARTESIAN_POINT('Ctrl Pts',(23.1058218650381,9.05298395410356,-6.35118260107245));
#32555=CARTESIAN_POINT('Ctrl Pts',(23.6175153199788,9.00245668094437,-6.42382403760964));
#32556=CARTESIAN_POINT('Ctrl Pts',(24.1364702886545,8.95485371029555,-6.49007583237978));
#32557=CARTESIAN_POINT('Ctrl Pts',(24.6629181373246,8.91145225308144,-6.54944423929279));
#32558=CARTESIAN_POINT('Ctrl Pts',(25.0606678571037,8.88140293076164,-6.59024788291775));
#32559=CARTESIAN_POINT('Ctrl Pts',(25.3945416155882,8.85873533710264,-6.6209922830971));
#32560=CARTESIAN_POINT('Ctrl Pts',(25.6627586119464,8.84221409068033,-6.64352323130153));
#32561=CARTESIAN_POINT('Ctrl Pts',(25.7972076165425,8.83452216013014,-6.65408072739387));
#32562=CARTESIAN_POINT('Ctrl Pts',(26.3824137782946,8.80240169886323,-6.69837697633853));
#32563=CARTESIAN_POINT('Ctrl Pts',(27.4369717967155,8.76563881905854,-6.74704662082203));
#32564=CARTESIAN_POINT('Ctrl Pts',(28.4593635146677,8.74917816753949,-6.76713562537254));
#32565=CARTESIAN_POINT('Ctrl Pts',(29.0427481469891,8.73952198264544,-6.77974505298723));
#32566=CARTESIAN_POINT('Ctrl Pts',(29.2174939164952,8.73701514175018,-6.78306424239323));
#32567=CARTESIAN_POINT('Ctrl Pts',(29.5607048332279,8.73336568489193,-6.78786835107262));
#32568=CARTESIAN_POINT('Ctrl Pts',(29.9899637006214,8.73093988338428,-6.79106253935677));
#32569=CARTESIAN_POINT('Ctrl Pts',(30.5003627545718,8.73068255391872,-6.79139754852948));
#32570=CARTESIAN_POINT('Ctrl Pts',(31.5152290141054,8.73381293113859,-6.7872875501941));
#32571=CARTESIAN_POINT('Ctrl Pts',(32.346385618228,8.74063107149335,-6.77838967797266));
#32572=CARTESIAN_POINT('Ctrl Pts',(33.1616392309915,8.74062146997074,-6.77840182636606));
#32573=CARTESIAN_POINT('Ctrl Pts',(33.4928689770884,8.74062052628883,-6.77840284181041));
#32574=CARTESIAN_POINT('Ctrl Pts',(33.9856875201801,8.74061852020513,-6.77840526161275));
#32575=CARTESIAN_POINT('Ctrl Pts',(34.4799569296089,8.74061713883255,-6.7784068708528));
#32576=CARTESIAN_POINT('Ctrl Pts',(35.1382080085716,8.74061527897129,-6.778409075901));
#32577=CARTESIAN_POINT('Ctrl Pts',(35.9613703496106,8.74061266742265,-6.7784121544085));
#32578=CARTESIAN_POINT('Ctrl Pts',(37.9364530322258,8.74060999527038,-6.77841531264167));
#32579=CARTESIAN_POINT('Ctrl Pts',(39.5833333333333,8.74059347982546,-6.7784348060232));
#32580=CARTESIAN_POINT('Ctrl Pts',(40.9,8.74059347982546,-6.7784348060232));
#32581=CARTESIAN_POINT('Ctrl Pts',(6.65963435785827,15.5421695279122,0.914290744262172));
#32582=CARTESIAN_POINT('Ctrl Pts',(6.7513219377677,15.5478000748543,0.82766409749893));
#32583=CARTESIAN_POINT('Ctrl Pts',(6.84347928233528,15.552705535984,0.741125593738214));
#32584=CARTESIAN_POINT('Ctrl Pts',(7.91768245328712,15.6010379387116,-0.26091214146805));
#32585=CARTESIAN_POINT('Ctrl Pts',(8.92716941433652,15.5498192559038,-1.17337698529147));
#32586=CARTESIAN_POINT('Ctrl Pts',(11.0226592374973,15.3445243615387,-2.83406080960164));
#32587=CARTESIAN_POINT('Ctrl Pts',(12.028922251309,15.174357849642,-3.58841078209879));
#32588=CARTESIAN_POINT('Ctrl Pts',(14.1441326723881,14.8006104561251,-4.94359337154892));
#32589=CARTESIAN_POINT('Ctrl Pts',(15.1576282381579,14.5754503759515,-5.54148857510366));
#32590=CARTESIAN_POINT('Ctrl Pts',(17.2903455772588,14.1464770374584,-6.58799131832697));
#32591=CARTESIAN_POINT('Ctrl Pts',(18.3126565164254,13.9174993841978,-7.03615941125111));
#32592=CARTESIAN_POINT('Ctrl Pts',(19.6943886098338,13.6636269320846,-7.52140607073201));
#32593=CARTESIAN_POINT('Ctrl Pts',(20.1963997689949,13.5705283753709,-7.69105316997363));
#32594=CARTESIAN_POINT('Ctrl Pts',(20.9820476354982,13.4299327266448,-7.93384577456641));
#32595=CARTESIAN_POINT('Ctrl Pts',(21.7860719497258,13.2956844767357,-8.15658902665418));
#32596=CARTESIAN_POINT('Ctrl Pts',(22.337913112583,13.2134517389134,-8.29065006793576));
#32597=CARTESIAN_POINT('Ctrl Pts',(22.7470242103181,13.1573095336481,-8.38247788994951));
#32598=CARTESIAN_POINT('Ctrl Pts',(23.0012838485784,13.1227286630507,-8.43794163853499));
#32599=CARTESIAN_POINT('Ctrl Pts',(23.5207560883432,13.0548326909721,-8.54431696039332));
#32600=CARTESIAN_POINT('Ctrl Pts',(24.0478165510037,12.9907421048666,-8.64139629793569));
#32601=CARTESIAN_POINT('Ctrl Pts',(24.5834508086858,12.9321620155411,-8.72854413973125));
#32602=CARTESIAN_POINT('Ctrl Pts',(24.9884814516724,12.8915554305395,-8.78849484453724));
#32603=CARTESIAN_POINT('Ctrl Pts',(25.328876176695,12.8608881947636,-8.83370307828861));
#32604=CARTESIAN_POINT('Ctrl Pts',(25.6025411192576,12.8385223247211,-8.86685769924429));
#32605=CARTESIAN_POINT('Ctrl Pts',(25.7397909478799,12.8281059147068,-8.88239886754126));
#32606=CARTESIAN_POINT('Ctrl Pts',(26.337634174326,12.7845927902169,-8.94762125696996));
#32607=CARTESIAN_POINT('Ctrl Pts',(27.4152541470276,12.7347557261564,-9.01924678134852));
#32608=CARTESIAN_POINT('Ctrl Pts',(28.4429499146132,12.7126826807293,-9.04845162691344));
#32609=CARTESIAN_POINT('Ctrl Pts',(29.025973512459,12.6997781188675,-9.06676270853365));
#32610=CARTESIAN_POINT('Ctrl Pts',(29.2042686472713,12.6963761571783,-9.07165323227904));
#32611=CARTESIAN_POINT('Ctrl Pts',(29.5518704410185,12.6914548812215,-9.07868995890013));
#32612=CARTESIAN_POINT('Ctrl Pts',(29.9865605489543,12.6881801081656,-9.0833711721763));
#32613=CARTESIAN_POINT('Ctrl Pts',(30.5013181269546,12.687836307306,-9.08385656546478));
#32614=CARTESIAN_POINT('Ctrl Pts',(31.5221463919967,12.692041007367,-9.07785413361794));
#32615=CARTESIAN_POINT('Ctrl Pts',(32.3518561954418,12.7011306199595,-9.06494609970921));
#32616=CARTESIAN_POINT('Ctrl Pts',(33.1604291208177,12.7011133788387,-9.06496486760966));
#32617=CARTESIAN_POINT('Ctrl Pts',(33.492519059067,12.7011117013819,-9.06496624091916));
#32618=CARTESIAN_POINT('Ctrl Pts',(33.9849476449336,12.7011081104537,-9.06496984963707));
#32619=CARTESIAN_POINT('Ctrl Pts',(34.4794328720439,12.7011056432242,-9.06497218408094));
#32620=CARTESIAN_POINT('Ctrl Pts',(35.1376484147356,12.7011023177079,-9.06497542847038));
#32621=CARTESIAN_POINT('Ctrl Pts',(35.9609115545804,12.7010976498373,-9.06497993729913));
#32622=CARTESIAN_POINT('Ctrl Pts',(37.9360269889122,12.7010928728514,-9.06498457262958));
#32623=CARTESIAN_POINT('Ctrl Pts',(39.5833333333333,12.701063350837,-9.06501315216909));
#32624=CARTESIAN_POINT('Ctrl Pts',(40.9,12.701063350837,-9.06501315216909));
#32625=CARTESIAN_POINT('Ctrl Pts',(6.47499700785697,23.4452408248497,2.19830497971403));
#32626=CARTESIAN_POINT('Ctrl Pts',(6.56578730943226,23.4579749263878,2.06870104448402));
#32627=CARTESIAN_POINT('Ctrl Pts',(6.65702462351448,23.4696212195475,1.93921681262018));
#32628=CARTESIAN_POINT('Ctrl Pts',(7.72175305647137,23.5924911125725,0.437116228582368));
#32629=CARTESIAN_POINT('Ctrl Pts',(8.72281885180382,23.562968194923,-0.937680140908612));
#32630=CARTESIAN_POINT('Ctrl Pts',(10.7949492361907,23.3400040819285,-3.44026704375966));
#32631=CARTESIAN_POINT('Ctrl Pts',(11.7960921547002,23.1244337632637,-4.58695803318564));
#32632=CARTESIAN_POINT('Ctrl Pts',(13.8958332645754,22.6316660291752,-6.64967501166335));
#32633=CARTESIAN_POINT('Ctrl Pts',(14.90655296446,22.3241101177864,-7.56603922905965));
#32634=CARTESIAN_POINT('Ctrl Pts',(17.0410718223018,21.7268962408645,-9.17994203101702));
#32635=CARTESIAN_POINT('Ctrl Pts',(18.0654584152639,21.4035033181339,-9.87337110606603));
#32636=CARTESIAN_POINT('Ctrl Pts',(19.4655915747002,21.0382396447148,-10.6334003056859));
#32637=CARTESIAN_POINT('Ctrl Pts',(19.9714665789849,20.9051898734593,-10.8971713557552));
#32638=CARTESIAN_POINT('Ctrl Pts',(20.7678306953019,20.7020007981629,-11.2774874271219));
#32639=CARTESIAN_POINT('Ctrl Pts',(21.5858101282049,20.5068169170513,-11.6277425327431));
#32640=CARTESIAN_POINT('Ctrl Pts',(22.1506096305012,20.3863209191721,-11.8398576536859));
#32641=CARTESIAN_POINT('Ctrl Pts',(22.5704199924792,20.3038374401207,-11.9854171937934));
#32642=CARTESIAN_POINT('Ctrl Pts',(22.8289065956907,20.2535349220293,-12.0724797867542));
#32643=CARTESIAN_POINT('Ctrl Pts',(23.3593853239227,20.1541718428526,-12.2402701514191));
#32644=CARTESIAN_POINT('Ctrl Pts',(23.8985486588058,20.0601195256968,-12.3936552183108));
#32645=CARTESIAN_POINT('Ctrl Pts',(24.4483714419233,19.9737860075934,-12.5318087211867));
#32646=CARTESIAN_POINT('Ctrl Pts',(24.8648919059683,19.9138158121695,-12.6269879069122));
#32647=CARTESIAN_POINT('Ctrl Pts',(25.2158455690755,19.8684065291874,-12.6989260386038));
#32648=CARTESIAN_POINT('Ctrl Pts',(25.4984343217206,19.835239602927,-12.7517388774023));
#32649=CARTESIAN_POINT('Ctrl Pts',(25.6403132052063,19.819776905443,-12.7765150372188));
#32650=CARTESIAN_POINT('Ctrl Pts',(26.259216041408,19.7551088720196,-12.880614699098));
#32651=CARTESIAN_POINT('Ctrl Pts',(27.3768446537004,19.681063586732,-12.994818613011));
#32652=CARTESIAN_POINT('Ctrl Pts',(28.4139434096804,19.6491350216628,-13.040069216748));
#32653=CARTESIAN_POINT('Ctrl Pts',(28.9963902080607,19.6305403234116,-13.068390840642));
#32654=CARTESIAN_POINT('Ctrl Pts',(29.1808784030088,19.62547738919,-13.0761959447011));
#32655=CARTESIAN_POINT('Ctrl Pts',(29.5361613355605,19.6182496508376,-13.0872826938044));
#32656=CARTESIAN_POINT('Ctrl Pts',(29.9803701492973,19.6134266676609,-13.0946820190498));
#32657=CARTESIAN_POINT('Ctrl Pts',(30.502764565205,19.6129305494836,-13.0954354949455));
#32658=CARTESIAN_POINT('Ctrl Pts',(31.5340441540657,19.6190493314859,-13.0860712826797));
#32659=CARTESIAN_POINT('Ctrl Pts',(32.3612933570749,19.6320590316267,-13.0662692307128));
#32660=CARTESIAN_POINT('Ctrl Pts',(33.1582057305722,19.6320151866218,-13.0663352315321));
#32661=CARTESIAN_POINT('Ctrl Pts',(33.4918052160808,19.6320107493385,-13.0663415440457));
#32662=CARTESIAN_POINT('Ctrl Pts',(33.9835585756086,19.6320015037507,-13.0663552182345));
#32663=CARTESIAN_POINT('Ctrl Pts',(34.4784268233885,19.6319950964453,-13.0663645784941));
#32664=CARTESIAN_POINT('Ctrl Pts',(35.1365871092732,19.6319864972548,-13.0663772185058));
#32665=CARTESIAN_POINT('Ctrl Pts',(35.9600364992905,19.631974409872,-13.0663949498221));
#32666=CARTESIAN_POINT('Ctrl Pts',(37.935219274406,19.6319620479287,-13.0664131007023));
#32667=CARTESIAN_POINT('Ctrl Pts',(39.5833333333333,19.6318856251071,-13.0665252579244));
#32668=CARTESIAN_POINT('Ctrl Pts',(40.9,19.6318856251071,-13.0665252579244));
#32669=CARTESIAN_POINT('Ctrl Pts',(6.39840282685635,31.3636440442398,3.36386536347515));
#32670=CARTESIAN_POINT('Ctrl Pts',(6.48879582230594,31.3828291635015,3.19164073503352));
#32671=CARTESIAN_POINT('Ctrl Pts',(6.57961766269115,31.4005708453189,3.01959979440375));
#32672=CARTESIAN_POINT('Ctrl Pts',(7.64032554406628,31.5903744166847,1.0214771742003));
#32673=CARTESIAN_POINT('Ctrl Pts',(8.63867106160223,31.5754173772483,-0.811297807542591));
#32674=CARTESIAN_POINT('Ctrl Pts',(10.6964316380006,31.3261515036618,-4.13353910931636));
#32675=CARTESIAN_POINT('Ctrl Pts',(11.6947290441859,31.0615534966588,-5.66648609020815));
#32676=CARTESIAN_POINT('Ctrl Pts',(13.7762263687762,30.4500782098735,-8.40637303045945));
#32677=CARTESIAN_POINT('Ctrl Pts',(14.7826773906134,30.0602543273649,-9.63313444048393));
#32678=CARTESIAN_POINT('Ctrl Pts',(16.8988982405362,29.3025485110513,-11.7841821047735));
#32679=CARTESIAN_POINT('Ctrl Pts',(17.9188263508252,28.8873179990429,-12.7156877051221));
#32680=CARTESIAN_POINT('Ctrl Pts',(19.3136620513073,28.4161739072999,-13.7379571249216));
#32681=CARTESIAN_POINT('Ctrl Pts',(19.8189838754923,28.2441169214324,-14.0939758439964));
#32682=CARTESIAN_POINT('Ctrl Pts',(20.6150001505384,27.9803060047161,-14.6080226620617));
#32683=CARTESIAN_POINT('Ctrl Pts',(21.4350390683301,27.7255808745093,-15.0835002485374));
#32684=CARTESIAN_POINT('Ctrl Pts',(22.0037815933943,27.5672808319297,-15.3731124530265));
#32685=CARTESIAN_POINT('Ctrl Pts',(22.4278524797961,27.4584837184542,-15.5725968076267));
#32686=CARTESIAN_POINT('Ctrl Pts',(22.688147887321,27.3924576319504,-15.6914147925572));
#32687=CARTESIAN_POINT('Ctrl Pts',(23.223810634427,27.2614400973337,-15.921268075794));
#32688=CARTESIAN_POINT('Ctrl Pts',(23.7696978745004,27.1369441741205,-16.1321064141347));
#32689=CARTESIAN_POINT('Ctrl Pts',(24.3285206801332,27.0220641661339,-16.3229204338608));
#32690=CARTESIAN_POINT('Ctrl Pts',(24.7529653140503,26.9419913350361,-16.4547973514758));
#32691=CARTESIAN_POINT('Ctrl Pts',(25.1117719491783,26.8811074137508,-16.5548637960119));
#32692=CARTESIAN_POINT('Ctrl Pts',(25.4013553254923,26.8365068705618,-16.6285198436921));
#32693=CARTESIAN_POINT('Ctrl Pts',(25.5469791293169,26.8156703264604,-16.6631374284085));
#32694=CARTESIAN_POINT('Ctrl Pts',(26.1832292898986,26.7283606594224,-16.8088431266916));
#32695=CARTESIAN_POINT('Ctrl Pts',(27.3386864567866,26.6279357083784,-16.9694451045117));
#32696=CARTESIAN_POINT('Ctrl Pts',(28.3853135289693,26.586099013527,-17.0308214554547));
#32697=CARTESIAN_POINT('Ctrl Pts',(28.9671494424547,26.5618106446085,-17.0691585340133));
#32698=CARTESIAN_POINT('Ctrl Pts',(29.1577497745604,26.5549253720647,-17.0801578267591));
#32699=CARTESIAN_POINT('Ctrl Pts',(29.5206667656999,26.5452518307314,-17.095535221436));
#32700=CARTESIAN_POINT('Ctrl Pts',(29.9743609805095,26.5387742795116,-17.1058350294712));
#32701=CARTESIAN_POINT('Ctrl Pts',(30.5043929318941,26.5381249904398,-17.1068574997827));
#32702=CARTESIAN_POINT('Ctrl Pts',(31.5460952643804,26.5462202887399,-17.0940221862974));
#32703=CARTESIAN_POINT('Ctrl Pts',(32.3708379684223,26.5630634070366,-17.0674707682792));
#32704=CARTESIAN_POINT('Ctrl Pts',(33.1560659395073,26.5629740474711,-17.0676145179389));
#32705=CARTESIAN_POINT('Ctrl Pts',(33.4911715963805,26.5629648505726,-17.0676289242213));
#32706=CARTESIAN_POINT('Ctrl Pts',(33.9822440621775,26.5629459056337,-17.0676591426917));
#32707=CARTESIAN_POINT('Ctrl Pts',(34.4774910986523,26.5629327280363,-17.0676800396183));
#32708=CARTESIAN_POINT('Ctrl Pts',(35.1355906516825,26.5629150749568,-17.0677081152075));
#32709=CARTESIAN_POINT('Ctrl Pts',(35.9592185001008,26.5628902459987,-17.0677475655254));
#32710=CARTESIAN_POINT('Ctrl Pts',(37.9344606912907,26.5628648600815,-17.067787918432));
#32711=CARTESIAN_POINT('Ctrl Pts',(39.5833333333333,26.5627078993772,-17.0680373636797));
#32712=CARTESIAN_POINT('Ctrl Pts',(40.9,26.5627078993772,-17.0680373636797));
#32713=CARTESIAN_POINT('Ctrl Pts',(6.37427268165564,34.7583359408307,3.85496595036636));
#32714=CARTESIAN_POINT('Ctrl Pts',(6.46448755772839,34.7802475524424,3.66446375246399));
#32715=CARTESIAN_POINT('Ctrl Pts',(6.55512331969025,34.8005635888992,3.47417181608893));
#32716=CARTESIAN_POINT('Ctrl Pts',(7.61410548625795,35.0185788676571,1.26339052014804));
#32717=CARTESIAN_POINT('Ctrl Pts',(8.61145388480624,35.0093532870147,-0.76560245720769));
#32718=CARTESIAN_POINT('Ctrl Pts',(10.6635149436019,34.747974440135,-4.43910992978125));
#32719=CARTESIAN_POINT('Ctrl Pts',(11.6608017032625,34.4619345886989,-6.13747453196185));
#32720=CARTESIAN_POINT('Ctrl Pts',(13.7353542747945,33.7990269238398,-9.16685810272324));
#32721=CARTESIAN_POINT('Ctrl Pts',(14.7402715202386,33.3736740493576,-10.526297955279));
#32722=CARTESIAN_POINT('Ctrl Pts',(16.8491677832147,32.5473921410153,-12.9054531131771));
#32723=CARTESIAN_POINT('Ctrl Pts',(17.8672809631136,32.092886041556,-13.9382203331611));
#32724=CARTESIAN_POINT('Ctrl Pts',(19.2587625104673,31.577179869867,-15.0707179501981));
#32725=CARTESIAN_POINT('Ctrl Pts',(19.7635899403542,31.3885503410944,-15.4658689812884));
#32726=CARTESIAN_POINT('Ctrl Pts',(20.5586991602297,31.0991569516509,-16.0362969262867));
#32727=CARTESIAN_POINT('Ctrl Pts',(21.3785272493018,30.819343278526,-16.564533786793));
#32728=CARTESIAN_POINT('Ctrl Pts',(21.9479176287994,30.6451300260617,-16.8867906552356));
#32729=CARTESIAN_POINT('Ctrl Pts',(22.3729695502115,30.525234440013,-17.1090467735268));
#32730=CARTESIAN_POINT('Ctrl Pts',(22.6337096028248,30.45253373981,-17.2413581349254));
#32731=CARTESIAN_POINT('Ctrl Pts',(23.1707519864209,30.3080867629256,-17.4975676797996));
#32732=CARTESIAN_POINT('Ctrl Pts',(23.7186485394885,30.170626807131,-17.7328951431605));
#32733=CARTESIAN_POINT('Ctrl Pts',(24.2804077704385,30.0435395405948,-17.946249160495));
#32734=CARTESIAN_POINT('Ctrl Pts',(24.7075732751058,29.9548357769835,-18.0938968083019));
#32735=CARTESIAN_POINT('Ctrl Pts',(25.0692008252975,29.8872739715487,-18.2061112471098));
#32736=CARTESIAN_POINT('Ctrl Pts',(25.3613771492325,29.8377189043884,-18.28880476277));
#32737=CARTESIAN_POINT('Ctrl Pts',(25.5084154817281,29.8145466170753,-18.3277015544066));
#32738=CARTESIAN_POINT('Ctrl Pts',(26.1512870025444,29.7173716879777,-18.4915385207408));
#32739=CARTESIAN_POINT('Ctrl Pts',(27.3223884400173,29.6052740416531,-18.6726738474942));
#32740=CARTESIAN_POINT('Ctrl Pts',(28.3731396048321,29.559177524821,-18.7409825767551));
#32741=CARTESIAN_POINT('Ctrl Pts',(28.9547046473315,29.5324480977279,-18.7836137746098));
#32742=CARTESIAN_POINT('Ctrl Pts',(29.1479037067738,29.5247529606444,-18.7960320303041));
#32743=CARTESIAN_POINT('Ctrl Pts',(29.5140802367921,29.51400582112,-18.8132921881813));
#32744=CARTESIAN_POINT('Ctrl Pts',(29.9718311305158,29.5067996680497,-18.8248686377542));
#32745=CARTESIAN_POINT('Ctrl Pts',(30.5051365276119,29.5060845192011,-18.8260067178222));
#32746=CARTESIAN_POINT('Ctrl Pts',(31.551298475448,29.5150383037988,-18.8116639693829));
#32747=CARTESIAN_POINT('Ctrl Pts',(32.3749555043413,29.5335081969199,-18.7822473977007));
#32748=CARTESIAN_POINT('Ctrl Pts',(33.1551698865007,29.5333957726549,-18.7824304492383));
#32749=CARTESIAN_POINT('Ctrl Pts',(33.4909201969602,29.5333841560219,-18.782448957068));
#32750=CARTESIAN_POINT('Ctrl Pts',(33.981699427726,29.5333602907362,-18.7824875453788));
#32751=CARTESIAN_POINT('Ctrl Pts',(34.4771077390558,29.533343676228,-18.7825142819534));
#32752=CARTESIAN_POINT('Ctrl Pts',(35.1351798881798,29.5333214285967,-18.7825501686284));
#32753=CARTESIAN_POINT('Ctrl Pts',(35.958882261465,29.5332901329543,-18.7826006107083));
#32754=CARTESIAN_POINT('Ctrl Pts',(37.9341479260215,29.5332581373787,-18.7826521993715));
#32755=CARTESIAN_POINT('Ctrl Pts',(39.5833333333333,29.5330603026358,-18.7829711232891));
#32756=CARTESIAN_POINT('Ctrl Pts',(40.9,29.5330603026358,-18.7829711232891));
#32757=CARTESIAN_POINT('',(40.9,27.7992994660114,-17.7819838375536));
#32758=CARTESIAN_POINT('Ctrl Pts',(40.9,27.7992994660114,-17.7819838375536));
#32759=CARTESIAN_POINT('Ctrl Pts',(40.9,28.2327406817405,-18.0322312401327));
#32760=CARTESIAN_POINT('Ctrl Pts',(40.9,28.6661818974695,-18.2824786427117));
#32761=CARTESIAN_POINT('Ctrl Pts',(40.9,29.0996231131986,-18.5327260452908));
#32762=CARTESIAN_POINT('',(38.,27.7992994660114,-17.7819838375536));
#32763=CARTESIAN_POINT('Ctrl Pts',(38.,27.7992994660114,-17.7819838375536));
#32764=CARTESIAN_POINT('Ctrl Pts',(38.9666666666667,27.7992994660114,-17.7819838375536));
#32765=CARTESIAN_POINT('Ctrl Pts',(39.9333333333333,27.7992994660114,-17.7819838375536));
#32766=CARTESIAN_POINT('Ctrl Pts',(40.9,27.7992994660114,-17.7819838375536));
#32767=CARTESIAN_POINT('Ctrl Pts',(37.4972396727241,27.2792903521173,-17.4814222894395));
#32768=CARTESIAN_POINT('Ctrl Pts',(37.6643013627084,27.4529632561668,-17.5817051235871));
#32769=CARTESIAN_POINT('Ctrl Pts',(37.8311425499706,27.6263785906016,-17.6818420596932));
#32770=CARTESIAN_POINT('Ctrl Pts',(37.9976538234737,27.7994318724651,-17.7817719425585));
#32771=CARTESIAN_POINT('',(6.9,29.9143312995417,2.26556458774883));
#32772=CARTESIAN_POINT('Ctrl Pts',(6.9,29.9143312995417,2.26556458774883));
#32773=CARTESIAN_POINT('Ctrl Pts',(6.9,27.3056186709172,2.00382962437802));
#32774=CARTESIAN_POINT('Ctrl Pts',(6.90000000000115,24.6693701926632,1.73285728374608));
#32775=CARTESIAN_POINT('Ctrl Pts',(6.90000000000115,18.7182130985667,1.09593289590079));
#32776=CARTESIAN_POINT('Ctrl Pts',(6.9,14.7845781982083,0.654794893503689));
#32777=CARTESIAN_POINT('Ctrl Pts',(6.9,11.02768739857,0.168526548660245));
#32778=CARTESIAN_POINT('',(22.9245129145126,27.5141512254856,-15.8853026165582));
#32779=CARTESIAN_POINT('Ctrl Pts',(22.9245129145126,27.5141512254856,-15.8853026165582));
#32780=CARTESIAN_POINT('Ctrl Pts',(22.7202811020963,27.5032269692373,-15.7659233420327));
#32781=CARTESIAN_POINT('Ctrl Pts',(22.5089075447093,27.4959054260063,-15.6398559109135));
#32782=CARTESIAN_POINT('Ctrl Pts',(22.2913349439917,27.4928730439354,-15.5073965833875));
#32783=CARTESIAN_POINT('Ctrl Pts',(21.4451770585291,27.4810798586143,-14.9922512750188));
#32784=CARTESIAN_POINT('Ctrl Pts',(20.5220951556665,27.5650257717264,-14.3509960808544));
#32785=CARTESIAN_POINT('Ctrl Pts',(19.7671428819535,27.6762399607749,-13.7859304181011));
#32786=CARTESIAN_POINT('Ctrl Pts',(19.5194773058389,27.7127242885422,-13.600558020691));
#32787=CARTESIAN_POINT('Ctrl Pts',(19.286571638609,27.7514615171004,-13.421872324025));
#32788=CARTESIAN_POINT('Ctrl Pts',(19.0728538401323,27.7894004949774,-13.2552441975238));
#32789=CARTESIAN_POINT('Ctrl Pts',(18.7028555998036,27.8550822264681,-12.966769797946));
#32790=CARTESIAN_POINT('Ctrl Pts',(18.4144703596237,27.9152561335183,-12.7292901983116));
#32791=CARTESIAN_POINT('Ctrl Pts',(18.064287487154,27.994606215575,-12.4284122845048));
#32792=CARTESIAN_POINT('Ctrl Pts',(17.4420927116723,28.1355931408966,-11.8938211301514));
#32793=CARTESIAN_POINT('Ctrl Pts',(16.7224564418219,28.3254287038798,-11.2282910364348));
#32794=CARTESIAN_POINT('Ctrl Pts',(15.9202806616111,28.5439924969395,-10.4246142212493));
#32795=CARTESIAN_POINT('Ctrl Pts',(15.4090529834518,28.6832834892781,-9.91242993152956));
#32796=CARTESIAN_POINT('Ctrl Pts',(14.8739602945714,28.8377564730262,-9.33532862360329));
#32797=CARTESIAN_POINT('Ctrl Pts',(14.3169794331154,28.9944199787763,-8.69171842999367));
#32798=CARTESIAN_POINT('Ctrl Pts',(13.8864206762836,29.1155243989539,-8.19419324731421));
#32799=CARTESIAN_POINT('Ctrl Pts',(13.3867890027804,29.2546860278643,-7.5917385218513));
#32800=CARTESIAN_POINT('Ctrl Pts',(12.8146824059514,29.3960736315876,-6.86770373383358));
#32801=CARTESIAN_POINT('Ctrl Pts',(12.2526665517595,29.5349674589251,-6.15643937836581));
#32802=CARTESIAN_POINT('Ctrl Pts',(11.6379478462803,29.678401911158,-5.32066918438564));
#32803=CARTESIAN_POINT('Ctrl Pts',(10.9739250490308,29.7956367796097,-4.35448584004002));
#32804=CARTESIAN_POINT('Ctrl Pts',(10.5683455447963,29.8672428449776,-3.76434923114274));
#32805=CARTESIAN_POINT('Ctrl Pts',(10.1437415406956,29.9275397584159,-3.12422765605936));
#32806=CARTESIAN_POINT('Ctrl Pts',(9.74137929176525,29.9670595377668,-2.50486371218385));
#32807=CARTESIAN_POINT('Ctrl Pts',(8.72285779294234,30.0670981099855,-0.93703399130421));
#32808=CARTESIAN_POINT('Ctrl Pts',(7.81323138778195,30.0560666286387,0.638451825302682));
#32809=CARTESIAN_POINT('Ctrl Pts',(6.9,29.9143312995417,2.26556458774884));
#32810=CARTESIAN_POINT('Ctrl Pts',(30.5,29.5059919176187,-18.8254200738635));
#32811=CARTESIAN_POINT('Ctrl Pts',(29.9560179420816,29.293615660989,-18.7064245513841));
#32812=CARTESIAN_POINT('Ctrl Pts',(29.4152668325132,29.0895919906434,-18.5734800115823));
#32813=CARTESIAN_POINT('Ctrl Pts',(28.8740459957565,28.9020067835811,-18.4125151878636));
#32814=CARTESIAN_POINT('Ctrl Pts',(28.353527792344,28.7215970352204,-18.2577075471291));
#32815=CARTESIAN_POINT('Ctrl Pts',(27.8179515912466,28.533139934629,-18.1008601332298));
#32816=CARTESIAN_POINT('Ctrl Pts',(27.2695051149491,28.3565719042575,-17.9186544331585));
#32817=CARTESIAN_POINT('Ctrl Pts',(26.9554553615883,28.2554660556724,-17.8143203592948));
#32818=CARTESIAN_POINT('Ctrl Pts',(26.6378099296971,28.1585101274348,-17.7019284120276));
#32819=CARTESIAN_POINT('Ctrl Pts',(26.3179304017917,28.0701057587103,-17.5778023417279));
#32820=CARTESIAN_POINT('Ctrl Pts',(26.1078196745982,28.012037940737,-17.4962709631331));
#32821=CARTESIAN_POINT('Ctrl Pts',(25.8967402232745,27.9576659729224,-17.409683568055));
#32822=CARTESIAN_POINT('Ctrl Pts',(25.6850706236774,27.9082593406129,-17.3169960819306));
#32823=CARTESIAN_POINT('Ctrl Pts',(25.6562210027417,27.9015254373195,-17.3043631915899));
#32824=CARTESIAN_POINT('Ctrl Pts',(25.6277737638215,27.8949772388532,-17.2918013331136));
#32825=CARTESIAN_POINT('Ctrl Pts',(25.5983858063598,27.8883138877393,-17.2787081509674));
#32826=CARTESIAN_POINT('Ctrl Pts',(25.1249357452756,27.7809650188704,-17.067772501732));
#32827=CARTESIAN_POINT('Ctrl Pts',(24.1510084067019,27.5797558484168,-16.6022239440147));
#32828=CARTESIAN_POINT('Ctrl Pts',(22.9245129145126,27.5141512254856,-15.8853026165582));
#32829=CARTESIAN_POINT('Origin',(49.9,0.,0.));
#32830=CARTESIAN_POINT('',(50.15,-9.2,1.12667505521557E-15));
#32831=CARTESIAN_POINT('Origin',(50.15,0.,0.));
#32832=CARTESIAN_POINT('',(49.65,-8.7,-1.0654427152582E-15));
#32833=CARTESIAN_POINT('',(49.9,-8.95,-1.09605888523688E-15));
#32834=CARTESIAN_POINT('Origin',(49.65,0.,0.));
#32835=CARTESIAN_POINT('Origin',(49.65,7.7,0.));
#32836=CARTESIAN_POINT('',(49.65,-7.7,-9.42978035343462E-16));
#32837=CARTESIAN_POINT('Origin',(49.65,0.,0.));
#32838=CARTESIAN_POINT('Origin',(49.75,0.,0.));
#32839=CARTESIAN_POINT('',(51.6,-9.2,1.12667505521557E-15));
#32840=CARTESIAN_POINT('Origin',(51.6,0.,0.));
#32841=CARTESIAN_POINT('',(49.75,-9.2,-1.12667505521557E-15));
#32842=CARTESIAN_POINT('Origin',(47.75,0.,0.));
#32843=CARTESIAN_POINT('',(47.5,-9.2,-1.12667505521557E-15));
#32844=CARTESIAN_POINT('Origin',(47.5,0.,0.));
#32845=CARTESIAN_POINT('',(48.,-8.7,1.0654427152582E-15));
#32846=CARTESIAN_POINT('',(47.75,-8.95,1.09605888523688E-15));
#32847=CARTESIAN_POINT('Origin',(48.,0.,0.));
#32848=CARTESIAN_POINT('Origin',(48.,9.7,0.));
#32849=CARTESIAN_POINT('',(48.,-7.7,-9.42978035343462E-16));
#32850=CARTESIAN_POINT('Origin',(48.,0.,0.));
#32851=CARTESIAN_POINT('Origin',(49.75,0.,0.));
#32852=CARTESIAN_POINT('',(44.4,-9.2,-1.12667505521557E-15));
#32853=CARTESIAN_POINT('',(49.75,-9.2,-1.12667505521557E-15));
#32854=CARTESIAN_POINT('Origin',(44.4,0.,0.));
#32855=CARTESIAN_POINT('Origin',(39.5,29.8970448036199,13.5172791635421));
#32856=CARTESIAN_POINT('',(37.6890795305109,29.8980142324913,13.062275865462));
#32857=CARTESIAN_POINT('',(38.,29.8960753747485,13.9722824616222));
#32858=CARTESIAN_POINT('Ctrl Pts',(37.6890795305109,29.8980142324913,13.062275865462));
#32859=CARTESIAN_POINT('Ctrl Pts',(37.8392820392456,29.8970503150544,13.5146923611995));
#32860=CARTESIAN_POINT('Ctrl Pts',(38.,29.8960753747485,13.9722824616222));
#32861=CARTESIAN_POINT('',(41.,29.8960753747485,13.9722824616222));
#32862=CARTESIAN_POINT('',(39.5,29.8960753747485,13.9722824616222));
#32863=CARTESIAN_POINT('',(41.1878146323178,29.897037739141,13.520600663113));
#32864=CARTESIAN_POINT('Ctrl Pts',(41.,29.8960753747485,13.9722824616222));
#32865=CARTESIAN_POINT('Ctrl Pts',(41.0954573034532,29.8965579362819,13.7457970542549));
#32866=CARTESIAN_POINT('Ctrl Pts',(41.1878146323178,29.897037739141,13.520600663113));
#32867=CARTESIAN_POINT('',(41.,29.8980142324913,13.062275865462));
#32868=CARTESIAN_POINT('Ctrl Pts',(41.1878146323178,29.897037739141,13.520600663113));
#32869=CARTESIAN_POINT('Ctrl Pts',(41.0874190143433,29.8975316564897,13.2887794747321));
#32870=CARTESIAN_POINT('Ctrl Pts',(41.,29.8980142324913,13.062275865462));
#32871=CARTESIAN_POINT('',(39.5,29.8980142324913,13.062275865462));
#32872=CARTESIAN_POINT('Origin',(41.25,37.284736894758,9.9904151409573));
#32873=CARTESIAN_POINT('',(41.5,29.553277056526,13.5223450340618));
#32874=CARTESIAN_POINT('Ctrl Pts',(41.1878146323178,29.8970377514405,13.5206006631392));
#32875=CARTESIAN_POINT('Ctrl Pts',(41.2916267029318,29.7825583314293,13.5218058342594));
#32876=CARTESIAN_POINT('Ctrl Pts',(41.3956918967678,29.6679697026706,13.5223797770881));
#32877=CARTESIAN_POINT('Ctrl Pts',(41.5,29.553277056526,13.5223450340618));
#32878=CARTESIAN_POINT('',(41.5,32.3550612130622,3.06594421002715));
#32879=CARTESIAN_POINT('Origin',(41.5,37.284736894758,9.9904151409573));
#32880=CARTESIAN_POINT('',(41.1878146546253,32.6518945010449,3.23933521449283));
#32881=CARTESIAN_POINT('Ctrl Pts',(41.5,32.3550612130622,3.06594421002716));
#32882=CARTESIAN_POINT('Ctrl Pts',(41.39570853676,32.4543894816631,3.12325130125064));
#32883=CARTESIAN_POINT('Ctrl Pts',(41.2916432763383,32.5533392901647,3.18104250345541));
#32884=CARTESIAN_POINT('Ctrl Pts',(41.1878146546253,32.6518945010449,3.23933521449283));
#32885=CARTESIAN_POINT('',(41.,32.4235777807772,3.63674438551515));
#32886=CARTESIAN_POINT('Ctrl Pts',(41.1878146546253,32.6518945010449,3.23933521449283));
#32887=CARTESIAN_POINT('Ctrl Pts',(41.0874190341598,32.5364116500246,3.44034521515088));
#32888=CARTESIAN_POINT('Ctrl Pts',(41.,32.4235777807772,3.63674438551515));
#32889=CARTESIAN_POINT('Origin',(41.,37.284736894758,9.9904151409573));
#32890=CARTESIAN_POINT('Origin',(41.25,0.,0.));
#32891=CARTESIAN_POINT('',(41.,27.0483892479909,18.9046195171755));
#32892=CARTESIAN_POINT('Origin',(41.,0.,0.));
#32893=CARTESIAN_POINT('',(41.1878146339918,26.6577025178081,19.1312938476316));
#32894=CARTESIAN_POINT('Ctrl Pts',(41.1878146339918,26.6577025178081,19.1312938476316));
#32895=CARTESIAN_POINT('Ctrl Pts',(41.0954573053938,26.8524884122049,19.0182801301661));
#32896=CARTESIAN_POINT('Ctrl Pts',(41.,27.0483892479909,18.9046195171755));
#32897=CARTESIAN_POINT('',(41.5,26.4873328464988,18.8327161790004));
#32898=CARTESIAN_POINT('Ctrl Pts',(41.5,26.4873328464988,18.8327161790004));
#32899=CARTESIAN_POINT('Ctrl Pts',(41.3957085361513,26.5447001051442,18.9320097106969));
#32900=CARTESIAN_POINT('Ctrl Pts',(41.2916417549508,26.6014983751947,19.0315347253102));
#32901=CARTESIAN_POINT('Ctrl Pts',(41.1878146339918,26.6577025235174,19.1312938574719));
#32902=CARTESIAN_POINT('Origin',(41.5,0.,0.));
#32903=CARTESIAN_POINT('Origin',(39.5,0.,0.));
#32904=CARTESIAN_POINT('Origin',(38.,0.,0.));
#32905=CARTESIAN_POINT('',(40.9,27.7992994660114,17.7819838375536));
#32906=CARTESIAN_POINT('Origin',(40.9,0.,0.));
#32907=CARTESIAN_POINT('',(38.,27.7992994660114,17.7819838375536));
#32908=CARTESIAN_POINT('Ctrl Pts',(40.9,27.7992994660114,17.7819838375536));
#32909=CARTESIAN_POINT('Ctrl Pts',(39.9333333333333,27.7992994660114,17.7819838375536));
#32910=CARTESIAN_POINT('Ctrl Pts',(38.9666666666667,27.7992994660114,17.7819838375536));
#32911=CARTESIAN_POINT('Ctrl Pts',(38.,27.7992994660114,17.7819838375536));
#32912=CARTESIAN_POINT('',(38.,27.0483892479909,18.9046195171755));
#32913=CARTESIAN_POINT('Origin',(38.,0.,0.));
#32914=CARTESIAN_POINT('',(39.5,27.0483892479909,18.9046195171755));
#32915=CARTESIAN_POINT('Origin',(39.5,26.6548295474835,19.1329607162453));
#32916=CARTESIAN_POINT('',(37.6890795305109,26.2612698469761,19.3613019153151));
#32917=CARTESIAN_POINT('Ctrl Pts',(38.,27.0483892479909,18.9046195171755));
#32918=CARTESIAN_POINT('Ctrl Pts',(37.8392820392454,26.6525920666572,19.1342588904591));
#32919=CARTESIAN_POINT('Ctrl Pts',(37.6890795305109,26.2612698469761,19.3613019153151));
#32920=CARTESIAN_POINT('',(41.,26.2612698469761,19.3613019153151));
#32921=CARTESIAN_POINT('',(39.5,26.2612698469761,19.3613019153151));
#32922=CARTESIAN_POINT('Ctrl Pts',(41.,26.2612698469761,19.3613019153151));
#32923=CARTESIAN_POINT('Ctrl Pts',(41.0874190154267,26.4571864382329,19.2476321871109));
#32924=CARTESIAN_POINT('Ctrl Pts',(41.1878146339918,26.6577025178081,19.1312938476316));
#32925=CARTESIAN_POINT('Origin',(41.25,27.2943217538007,27.2943217538007));
#32926=CARTESIAN_POINT('',(41.,19.3613019153151,26.2612698469761));
#32927=CARTESIAN_POINT('Origin',(41.,27.2943217538007,27.2943217538007));
#32928=CARTESIAN_POINT('',(41.1878146323178,19.1312938484417,26.6577025182511));
#32929=CARTESIAN_POINT('Ctrl Pts',(41.1878146323178,19.1312938484417,26.6577025182511));
#32930=CARTESIAN_POINT('Ctrl Pts',(41.0874190143433,19.2476321876035,26.457186438652));
#32931=CARTESIAN_POINT('Ctrl Pts',(41.,19.3613019153151,26.2612698469761));
#32932=CARTESIAN_POINT('',(41.5,18.8327161790004,26.4873328464988));
#32933=CARTESIAN_POINT('Ctrl Pts',(41.1878146323178,19.1312938590803,26.6577025244235));
#32934=CARTESIAN_POINT('Ctrl Pts',(41.2916267029318,19.0315491875799,26.601506523224));
#32935=CARTESIAN_POINT('Ctrl Pts',(41.3956918967678,18.9320255526757,26.5447092579146));
#32936=CARTESIAN_POINT('Ctrl Pts',(41.5,18.8327161790004,26.4873328464988));
#32937=CARTESIAN_POINT('Origin',(41.5,27.2943217538007,27.2943217538007));
#32938=CARTESIAN_POINT('Origin',(39.5,19.1329607162453,26.6548295474835));
#32939=CARTESIAN_POINT('',(37.6890795305109,19.3613019153151,26.2612698469761));
#32940=CARTESIAN_POINT('',(38.,18.9046195171755,27.0483892479908));
#32941=CARTESIAN_POINT('Ctrl Pts',(37.6890795305109,19.3613019153151,26.2612698469761));
#32942=CARTESIAN_POINT('Ctrl Pts',(37.8392820392454,19.1342588904592,26.652592066657));
#32943=CARTESIAN_POINT('Ctrl Pts',(38.,18.9046195171755,27.0483892479908));
#32944=CARTESIAN_POINT('',(41.,18.9046195171755,27.0483892479908));
#32945=CARTESIAN_POINT('',(39.5,18.9046195171755,27.0483892479908));
#32946=CARTESIAN_POINT('Ctrl Pts',(41.,18.9046195171755,27.0483892479908));
#32947=CARTESIAN_POINT('Ctrl Pts',(41.0954573034533,19.0182801314061,26.8524884123908));
#32948=CARTESIAN_POINT('Ctrl Pts',(41.1878146323178,19.1312938484417,26.6577025182511));
#32949=CARTESIAN_POINT('',(39.5,19.3613019153151,26.2612698469761));
#32950=CARTESIAN_POINT('Origin',(41.25,0.,0.));
#32951=CARTESIAN_POINT('',(41.,13.9722824616222,29.8960753747485));
#32952=CARTESIAN_POINT('Origin',(41.,0.,0.));
#32953=CARTESIAN_POINT('',(41.1878146339917,13.5206006631344,29.8970377382179));
#32954=CARTESIAN_POINT('Ctrl Pts',(41.1878146339917,13.5206006631344,29.8970377382179));
#32955=CARTESIAN_POINT('Ctrl Pts',(41.0954573053939,13.7457970547134,29.8965579351151));
#32956=CARTESIAN_POINT('Ctrl Pts',(41.,13.9722824616222,29.8960753747485));
#32957=CARTESIAN_POINT('',(41.5,13.5223450340618,29.553277056526));
#32958=CARTESIAN_POINT('Ctrl Pts',(41.5,13.5223450340618,29.553277056526));
#32959=CARTESIAN_POINT('Ctrl Pts',(41.3957085361513,13.5223797715459,29.6679514067293));
#32960=CARTESIAN_POINT('Ctrl Pts',(41.2916417549508,13.521806008994,29.7825417327217));
#32961=CARTESIAN_POINT('Ctrl Pts',(41.1878146339918,13.5206006631586,29.8970377495945));
#32962=CARTESIAN_POINT('Origin',(41.5,0.,0.));
#32963=CARTESIAN_POINT('Origin',(39.5,0.,0.));
#32964=CARTESIAN_POINT('Origin',(38.,0.,0.));
#32965=CARTESIAN_POINT('',(40.9,15.1839076262003,29.2992994660114));
#32966=CARTESIAN_POINT('Origin',(40.9,0.,0.));
#32967=CARTESIAN_POINT('',(38.,15.1839076262003,29.2992994660114));
#32968=CARTESIAN_POINT('Ctrl Pts',(40.9,15.1839076262003,29.2992994660114));
#32969=CARTESIAN_POINT('Ctrl Pts',(39.9333333333333,15.1839076262003,29.2992994660114));
#32970=CARTESIAN_POINT('Ctrl Pts',(38.9666666666667,15.1839076262003,29.2992994660114));
#32971=CARTESIAN_POINT('Ctrl Pts',(38.,15.1839076262003,29.2992994660114));
#32972=CARTESIAN_POINT('',(38.,13.9722824616222,29.8960753747485));
#32973=CARTESIAN_POINT('Origin',(38.,0.,0.));
#32974=CARTESIAN_POINT('',(39.5,13.9722824616222,29.8960753747485));
#32975=CARTESIAN_POINT('Origin',(39.5,13.5172791635421,29.8970448036199));
#32976=CARTESIAN_POINT('',(37.6890795305109,13.062275865462,29.8980142324913));
#32977=CARTESIAN_POINT('Ctrl Pts',(38.,13.9722824616222,29.8960753747485));
#32978=CARTESIAN_POINT('Ctrl Pts',(37.8392820392454,13.5146923611992,29.8970503150544));
#32979=CARTESIAN_POINT('Ctrl Pts',(37.6890795305109,13.062275865462,29.8980142324913));
#32980=CARTESIAN_POINT('',(41.,13.062275865462,29.8980142324913));
#32981=CARTESIAN_POINT('',(39.5,13.062275865462,29.8980142324913));
#32982=CARTESIAN_POINT('Ctrl Pts',(41.,13.062275865462,29.8980142324913));
#32983=CARTESIAN_POINT('Ctrl Pts',(41.0874190154267,13.2887794746153,29.8975316558535));
#32984=CARTESIAN_POINT('Ctrl Pts',(41.1878146339917,13.5206006631344,29.8970377382179));
#32985=CARTESIAN_POINT('Origin',(41.25,9.99041514095731,37.284736894758));
#32986=CARTESIAN_POINT('',(41.,3.63674438551516,32.4235777807772));
#32987=CARTESIAN_POINT('Origin',(41.,9.99041514095731,37.284736894758));
#32988=CARTESIAN_POINT('',(41.1878146323178,3.23933522088993,32.6518945115547));
#32989=CARTESIAN_POINT('Ctrl Pts',(41.1878146323178,3.23933522088992,32.6518945115547));
#32990=CARTESIAN_POINT('Ctrl Pts',(41.0874190143434,3.44034521783764,32.5364116623356));
#32991=CARTESIAN_POINT('Ctrl Pts',(41.,3.63674438551516,32.4235777807772));
#32992=CARTESIAN_POINT('',(41.5,3.06594421002715,32.3550612130622));
#32993=CARTESIAN_POINT('Ctrl Pts',(41.1878146323177,3.23933522701702,32.6518945222195));
#32994=CARTESIAN_POINT('Ctrl Pts',(41.2916267029318,3.18105180820533,32.5533550218394));
#32995=CARTESIAN_POINT('Ctrl Pts',(41.3956918967678,3.12326044475599,32.4544053297638));
#32996=CARTESIAN_POINT('Ctrl Pts',(41.5,3.06594421002716,32.3550612130622));
#32997=CARTESIAN_POINT('Origin',(41.5,9.99041514095731,37.284736894758));
#32998=CARTESIAN_POINT('Origin',(39.5,3.24221525613641,32.6502398797874));
#32999=CARTESIAN_POINT('',(37.6890795305109,3.63674438551516,32.4235777807772));
#33000=CARTESIAN_POINT('',(38.,2.84768612675767,32.8769019787977));
#33001=CARTESIAN_POINT('Ctrl Pts',(37.6890795305109,3.63674438551516,32.4235777807772));
#33002=CARTESIAN_POINT('Ctrl Pts',(37.8392820392455,3.24445824839702,32.6489512516584));
#33003=CARTESIAN_POINT('Ctrl Pts',(38.,2.84768612675767,32.8769019787977));
#33004=CARTESIAN_POINT('',(41.,2.84768612675767,32.8769019787977));
#33005=CARTESIAN_POINT('',(39.5,2.84768612675767,32.8769019787977));
#33006=CARTESIAN_POINT('Ctrl Pts',(41.,2.84768612675767,32.8769019787977));
#33007=CARTESIAN_POINT('Ctrl Pts',(41.0954573034532,3.04406952389089,32.7640771856609));
#33008=CARTESIAN_POINT('Ctrl Pts',(41.1878146323178,3.23933522088993,32.6518945115547));
#33009=CARTESIAN_POINT('',(39.5,3.63674438551516,32.4235777807772));
#33010=CARTESIAN_POINT('Origin',(41.25,0.,0.));
#33011=CARTESIAN_POINT('',(41.,-2.84768612675766,32.8769019787977));
#33012=CARTESIAN_POINT('Origin',(41.,0.,0.));
#33013=CARTESIAN_POINT('',(41.1878146339918,-3.23933522040986,32.651894510766));
#33014=CARTESIAN_POINT('Ctrl Pts',(41.1878146339918,-3.23933522040986,32.651894510766));
#33015=CARTESIAN_POINT('Ctrl Pts',(41.095457305394,-3.04406952291064,32.7640771848795));
#33016=CARTESIAN_POINT('Ctrl Pts',(41.,-2.84768612675766,32.8769019787977));
#33017=CARTESIAN_POINT('',(41.5,-3.06594421002714,32.3550612130622));
#33018=CARTESIAN_POINT('Ctrl Pts',(41.5,-3.06594421002715,32.3550612130622));
#33019=CARTESIAN_POINT('Ctrl Pts',(41.3957085361513,-3.1232513015851,32.4543894822428));
#33020=CARTESIAN_POINT('Ctrl Pts',(41.2916417549508,-3.181043357527,32.5533407343041));
#33021=CARTESIAN_POINT('Ctrl Pts',(41.1878146339918,-3.23933522607716,32.6518945206305));
#33022=CARTESIAN_POINT('Origin',(41.5,0.,0.));
#33023=CARTESIAN_POINT('Origin',(39.5,0.,0.));
#33024=CARTESIAN_POINT('Origin',(38.,0.,0.));
#33025=CARTESIAN_POINT('',(40.9,-1.5,32.9658914637539));
#33026=CARTESIAN_POINT('Origin',(40.9,0.,0.));
#33027=CARTESIAN_POINT('',(38.,-1.5,32.9658914637539));
#33028=CARTESIAN_POINT('Ctrl Pts',(40.9,-1.5,32.9658914637539));
#33029=CARTESIAN_POINT('Ctrl Pts',(39.9333333333333,-1.5,32.9658914637539));
#33030=CARTESIAN_POINT('Ctrl Pts',(38.9666666666667,-1.5,32.9658914637539));
#33031=CARTESIAN_POINT('Ctrl Pts',(38.,-1.5,32.9658914637539));
#33032=CARTESIAN_POINT('',(38.,-2.84768612675766,32.8769019787977));
#33033=CARTESIAN_POINT('Origin',(38.,0.,0.));
#33034=CARTESIAN_POINT('',(39.5,-2.84768612675766,32.8769019787977));
#33035=CARTESIAN_POINT('Origin',(39.5,-3.2422152561364,32.6502398797874));
#33036=CARTESIAN_POINT('',(37.6890795305109,-3.63674438551515,32.4235777807772));
#33037=CARTESIAN_POINT('Ctrl Pts',(38.,-2.84768612675766,32.8769019787977));
#33038=CARTESIAN_POINT('Ctrl Pts',(37.8392820392455,-3.244458248397,32.6489512516584));
#33039=CARTESIAN_POINT('Ctrl Pts',(37.6890795305109,-3.63674438551515,32.4235777807772));
#33040=CARTESIAN_POINT('',(41.,-3.63674438551515,32.4235777807772));
#33041=CARTESIAN_POINT('',(39.5,-3.63674438551515,32.4235777807772));
#33042=CARTESIAN_POINT('Ctrl Pts',(41.,-3.63674438551515,32.4235777807772));
#33043=CARTESIAN_POINT('Ctrl Pts',(41.0874190154267,-3.44034521762067,32.5364116617262));
#33044=CARTESIAN_POINT('Ctrl Pts',(41.1878146339918,-3.23933522040986,32.651894510766));
#33045=CARTESIAN_POINT('Origin',(41.25,-9.9904151409573,37.284736894758));
#33046=CARTESIAN_POINT('',(41.,-13.062275865462,29.8980142324913));
#33047=CARTESIAN_POINT('Origin',(41.,-9.9904151409573,37.284736894758));
#33048=CARTESIAN_POINT('',(41.1878146323178,-13.520600663113,29.897037739141));
#33049=CARTESIAN_POINT('Ctrl Pts',(41.1878146323178,-13.520600663113,29.897037739141));
#33050=CARTESIAN_POINT('Ctrl Pts',(41.0874190143433,-13.2887794747321,29.8975316564897));
#33051=CARTESIAN_POINT('Ctrl Pts',(41.,-13.062275865462,29.8980142324913));
#33052=CARTESIAN_POINT('',(41.5,-13.5223450340618,29.553277056526));
#33053=CARTESIAN_POINT('Ctrl Pts',(41.1878146323178,-13.5206006631392,29.8970377514405));
#33054=CARTESIAN_POINT('Ctrl Pts',(41.2916267029318,-13.5218058342594,29.7825583314293));
#33055=CARTESIAN_POINT('Ctrl Pts',(41.3956918967678,-13.5223797770881,29.6679697026706));
#33056=CARTESIAN_POINT('Ctrl Pts',(41.5,-13.5223450340618,29.553277056526));
#33057=CARTESIAN_POINT('Origin',(41.5,-9.9904151409573,37.284736894758));
#33058=CARTESIAN_POINT('Origin',(39.5,-13.5172791635421,29.8970448036199));
#33059=CARTESIAN_POINT('',(37.6890795305109,-13.062275865462,29.8980142324913));
#33060=CARTESIAN_POINT('',(38.,-13.9722824616222,29.8960753747485));
#33061=CARTESIAN_POINT('Ctrl Pts',(37.6890795305109,-13.062275865462,29.8980142324913));
#33062=CARTESIAN_POINT('Ctrl Pts',(37.8392820392455,-13.5146923611994,29.8970503150544));
#33063=CARTESIAN_POINT('Ctrl Pts',(38.,-13.9722824616222,29.8960753747485));
#33064=CARTESIAN_POINT('',(41.,-13.9722824616222,29.8960753747485));
#33065=CARTESIAN_POINT('',(39.5,-13.9722824616222,29.8960753747485));
#33066=CARTESIAN_POINT('Ctrl Pts',(41.,-13.9722824616222,29.8960753747485));
#33067=CARTESIAN_POINT('Ctrl Pts',(41.0954573034533,-13.7457970542547,29.8965579362819));
#33068=CARTESIAN_POINT('Ctrl Pts',(41.1878146323178,-13.520600663113,29.897037739141));
#33069=CARTESIAN_POINT('',(39.5,-13.062275865462,29.8980142324913));
#33070=CARTESIAN_POINT('Origin',(41.25,0.,0.));
#33071=CARTESIAN_POINT('',(41.,-18.9046195171755,27.0483892479909));
#33072=CARTESIAN_POINT('Origin',(41.,0.,0.));
#33073=CARTESIAN_POINT('',(41.1878146339917,-19.1312938476316,26.6577025178081));
#33074=CARTESIAN_POINT('Ctrl Pts',(41.1878146339917,-19.1312938476316,26.6577025178081));
#33075=CARTESIAN_POINT('Ctrl Pts',(41.0954573053939,-19.0182801301662,26.8524884122047));
#33076=CARTESIAN_POINT('Ctrl Pts',(41.,-18.9046195171755,27.0483892479909));
#33077=CARTESIAN_POINT('',(41.5,-18.8327161790004,26.4873328464988));
#33078=CARTESIAN_POINT('Ctrl Pts',(41.5,-18.8327161790004,26.4873328464988));
#33079=CARTESIAN_POINT('Ctrl Pts',(41.3957085361513,-18.9320097106969,26.5447001051442));
#33080=CARTESIAN_POINT('Ctrl Pts',(41.2916417549508,-19.0315347253102,26.6014983751947));
#33081=CARTESIAN_POINT('Ctrl Pts',(41.1878146339918,-19.1312938574719,26.6577025235174));
#33082=CARTESIAN_POINT('Origin',(41.5,0.,0.));
#33083=CARTESIAN_POINT('Origin',(39.5,0.,0.));
#33084=CARTESIAN_POINT('Origin',(38.,0.,0.));
#33085=CARTESIAN_POINT('',(40.9,-17.7819838375536,27.7992994660114));
#33086=CARTESIAN_POINT('Origin',(40.9,0.,0.));
#33087=CARTESIAN_POINT('',(38.,-17.7819838375536,27.7992994660114));
#33088=CARTESIAN_POINT('Ctrl Pts',(40.9,-17.7819838375536,27.7992994660114));
#33089=CARTESIAN_POINT('Ctrl Pts',(39.9333333333333,-17.7819838375536,27.7992994660114));
#33090=CARTESIAN_POINT('Ctrl Pts',(38.9666666666667,-17.7819838375536,27.7992994660114));
#33091=CARTESIAN_POINT('Ctrl Pts',(38.,-17.7819838375536,27.7992994660114));
#33092=CARTESIAN_POINT('',(38.,-18.9046195171755,27.0483892479909));
#33093=CARTESIAN_POINT('Origin',(38.,0.,0.));
#33094=CARTESIAN_POINT('',(39.5,-18.9046195171755,27.0483892479909));
#33095=CARTESIAN_POINT('Origin',(39.5,-19.1329607162453,26.6548295474835));
#33096=CARTESIAN_POINT('',(37.6890795305109,-19.3613019153151,26.2612698469761));
#33097=CARTESIAN_POINT('Ctrl Pts',(38.,-18.9046195171755,27.0483892479909));
#33098=CARTESIAN_POINT('Ctrl Pts',(37.8392820392454,-19.1342588904591,26.6525920666571));
#33099=CARTESIAN_POINT('Ctrl Pts',(37.6890795305109,-19.3613019153151,26.2612698469761));
#33100=CARTESIAN_POINT('',(41.,-19.3613019153151,26.2612698469761));
#33101=CARTESIAN_POINT('',(39.5,-19.3613019153151,26.2612698469761));
#33102=CARTESIAN_POINT('Ctrl Pts',(41.,-19.3613019153151,26.2612698469761));
#33103=CARTESIAN_POINT('Ctrl Pts',(41.0874190154267,-19.2476321871109,26.4571864382329));
#33104=CARTESIAN_POINT('Ctrl Pts',(41.1878146339917,-19.1312938476316,26.6577025178081));
#33105=CARTESIAN_POINT('Origin',(41.25,-27.2943217538007,27.2943217538008));
#33106=CARTESIAN_POINT('',(41.,-26.2612698469761,19.3613019153151));
#33107=CARTESIAN_POINT('Origin',(41.,-27.2943217538007,27.2943217538008));
#33108=CARTESIAN_POINT('',(41.1878146323178,-26.657702518251,19.1312938484417));
#33109=CARTESIAN_POINT('Ctrl Pts',(41.1878146323178,-26.657702518251,19.1312938484417));
#33110=CARTESIAN_POINT('Ctrl Pts',(41.0874190143433,-26.457186438652,19.2476321876035));
#33111=CARTESIAN_POINT('Ctrl Pts',(41.,-26.2612698469761,19.3613019153152));
#33112=CARTESIAN_POINT('',(41.5,-26.4873328464988,18.8327161790004));
#33113=CARTESIAN_POINT('Ctrl Pts',(41.1878146323178,-26.6577025244235,19.1312938590803));
#33114=CARTESIAN_POINT('Ctrl Pts',(41.2916267029318,-26.6015065232239,19.0315491875799));
#33115=CARTESIAN_POINT('Ctrl Pts',(41.3956918967678,-26.5447092579146,18.9320255526757));
#33116=CARTESIAN_POINT('Ctrl Pts',(41.5,-26.4873328464988,18.8327161790004));
#33117=CARTESIAN_POINT('Origin',(41.5,-27.2943217538007,27.2943217538008));
#33118=CARTESIAN_POINT('Origin',(39.5,-26.6548295474835,19.1329607162453));
#33119=CARTESIAN_POINT('',(37.6890795305109,-26.2612698469761,19.3613019153151));
#33120=CARTESIAN_POINT('',(38.,-27.0483892479908,18.9046195171755));
#33121=CARTESIAN_POINT('Ctrl Pts',(37.6890795305109,-26.2612698469761,19.3613019153151));
#33122=CARTESIAN_POINT('Ctrl Pts',(37.8392820392455,-26.6525920666574,19.134258890459));
#33123=CARTESIAN_POINT('Ctrl Pts',(38.,-27.0483892479908,18.9046195171755));
#33124=CARTESIAN_POINT('',(41.,-27.0483892479908,18.9046195171755));
#33125=CARTESIAN_POINT('',(39.5,-27.0483892479908,18.9046195171755));
#33126=CARTESIAN_POINT('Ctrl Pts',(41.,-27.0483892479908,18.9046195171755));
#33127=CARTESIAN_POINT('Ctrl Pts',(41.0954573034532,-26.8524884123911,19.0182801314059));
#33128=CARTESIAN_POINT('Ctrl Pts',(41.1878146323178,-26.6577025182511,19.1312938484417));
#33129=CARTESIAN_POINT('',(39.5,-26.2612698469761,19.3613019153151));
#33130=CARTESIAN_POINT('Origin',(41.25,0.,0.));
#33131=CARTESIAN_POINT('',(41.,-29.8960753747485,13.9722824616222));
#33132=CARTESIAN_POINT('Origin',(41.,0.,0.));
#33133=CARTESIAN_POINT('',(41.1878146339917,-29.8970377382179,13.5206006631344));
#33134=CARTESIAN_POINT('Ctrl Pts',(41.1878146339917,-29.8970377382179,13.5206006631344));
#33135=CARTESIAN_POINT('Ctrl Pts',(41.0954573053939,-29.8965579351151,13.7457970547134));
#33136=CARTESIAN_POINT('Ctrl Pts',(41.,-29.8960753747485,13.9722824616222));
#33137=CARTESIAN_POINT('',(41.5,-29.553277056526,13.5223450340618));
#33138=CARTESIAN_POINT('Ctrl Pts',(41.5,-29.553277056526,13.5223450340618));
#33139=CARTESIAN_POINT('Ctrl Pts',(41.3957085361513,-29.6679514067293,13.5223797715459));
#33140=CARTESIAN_POINT('Ctrl Pts',(41.2916417549508,-29.7825417327216,13.521806008994));
#33141=CARTESIAN_POINT('Ctrl Pts',(41.1878146339918,-29.8970377495945,13.5206006631586));
#33142=CARTESIAN_POINT('Origin',(41.5,0.,0.));
#33143=CARTESIAN_POINT('Origin',(39.5,0.,0.));
#33144=CARTESIAN_POINT('Origin',(38.,0.,0.));
#33145=CARTESIAN_POINT('',(40.9,-29.2992994660114,15.1839076262003));
#33146=CARTESIAN_POINT('Origin',(40.9,0.,0.));
#33147=CARTESIAN_POINT('',(38.,-29.2992994660114,15.1839076262003));
#33148=CARTESIAN_POINT('Ctrl Pts',(40.9,-29.2992994660114,15.1839076262003));
#33149=CARTESIAN_POINT('Ctrl Pts',(39.9333333333333,-29.2992994660114,15.1839076262003));
#33150=CARTESIAN_POINT('Ctrl Pts',(38.9666666666667,-29.2992994660114,15.1839076262003));
#33151=CARTESIAN_POINT('Ctrl Pts',(38.,-29.2992994660114,15.1839076262003));
#33152=CARTESIAN_POINT('',(38.,-29.8960753747485,13.9722824616222));
#33153=CARTESIAN_POINT('Origin',(38.,0.,0.));
#33154=CARTESIAN_POINT('',(39.5,-29.8960753747485,13.9722824616222));
#33155=CARTESIAN_POINT('Origin',(39.5,-29.8970448036199,13.5172791635421));
#33156=CARTESIAN_POINT('',(37.6890795305109,-29.8980142324913,13.0622758654621));
#33157=CARTESIAN_POINT('Ctrl Pts',(38.,-29.8960753747485,13.9722824616222));
#33158=CARTESIAN_POINT('Ctrl Pts',(37.8392820392455,-29.8970503150544,13.5146923611995));
#33159=CARTESIAN_POINT('Ctrl Pts',(37.6890795305109,-29.8980142324913,13.0622758654621));
#33160=CARTESIAN_POINT('',(41.,-29.8980142324913,13.0622758654621));
#33161=CARTESIAN_POINT('',(39.5,-29.8980142324913,13.0622758654621));
#33162=CARTESIAN_POINT('Ctrl Pts',(41.,-29.8980142324913,13.0622758654621));
#33163=CARTESIAN_POINT('Ctrl Pts',(41.0874190154267,-29.8975316558535,13.2887794746154));
#33164=CARTESIAN_POINT('Ctrl Pts',(41.1878146339917,-29.8970377382179,13.5206006631344));
#33165=CARTESIAN_POINT('Origin',(41.25,-37.284736894758,9.99041514095732));
#33166=CARTESIAN_POINT('',(41.,-32.4235777807772,3.63674438551517));
#33167=CARTESIAN_POINT('Origin',(41.,-37.284736894758,9.99041514095732));
#33168=CARTESIAN_POINT('',(41.1878146546253,-32.6518945010449,3.23933521449285));
#33169=CARTESIAN_POINT('Ctrl Pts',(41.,-32.4235777807772,3.63674438551517));
#33170=CARTESIAN_POINT('Ctrl Pts',(41.0874190341598,-32.5364116500246,3.44034521515094));
#33171=CARTESIAN_POINT('Ctrl Pts',(41.1878146546253,-32.6518945010449,3.23933521449285));
#33172=CARTESIAN_POINT('',(41.5,-32.3550612130622,3.06594421002716));
#33173=CARTESIAN_POINT('Ctrl Pts',(41.1878146546253,-32.6518945010449,3.23933521449284));
#33174=CARTESIAN_POINT('Ctrl Pts',(41.2916290694684,-32.5533527754738,3.18105047964687));
#33175=CARTESIAN_POINT('Ctrl Pts',(41.3956920266496,-32.454405206063,3.12326037338726));
#33176=CARTESIAN_POINT('Ctrl Pts',(41.5,-32.3550612130622,3.06594421002717));
#33177=CARTESIAN_POINT('Origin',(41.5,-37.284736894758,9.99041514095732));
#33178=CARTESIAN_POINT('Origin',(41.5,14.,0.));
#33179=CARTESIAN_POINT('',(41.5,-32.3550612130622,-3.06594421002714));
#33180=CARTESIAN_POINT('Origin',(41.5,0.,0.));
#33181=CARTESIAN_POINT('',(41.5,-29.553277056526,-13.5223450340618));
#33182=CARTESIAN_POINT('Origin',(41.5,-37.284736894758,-9.9904151409573));
#33183=CARTESIAN_POINT('',(41.5,-26.4873328464988,-18.8327161790004));
#33184=CARTESIAN_POINT('Origin',(41.5,0.,0.));
#33185=CARTESIAN_POINT('',(41.5,-18.8327161790004,-26.4873328464988));
#33186=CARTESIAN_POINT('Origin',(41.5,-27.2943217538008,-27.2943217538007));
#33187=CARTESIAN_POINT('',(41.5,-13.5223450340618,-29.553277056526));
#33188=CARTESIAN_POINT('Origin',(41.5,0.,0.));
#33189=CARTESIAN_POINT('',(41.5,-3.06594421002716,-32.3550612130622));
#33190=CARTESIAN_POINT('Origin',(41.5,-9.99041514095732,-37.284736894758));
#33191=CARTESIAN_POINT('',(41.5,3.06594421002714,-32.3550612130622));
#33192=CARTESIAN_POINT('Origin',(41.5,0.,0.));
#33193=CARTESIAN_POINT('',(41.5,13.5223450340618,-29.553277056526));
#33194=CARTESIAN_POINT('Origin',(41.5,9.99041514095729,-37.284736894758));
#33195=CARTESIAN_POINT('',(41.5,18.8327161790004,-26.4873328464989));
#33196=CARTESIAN_POINT('Origin',(41.5,0.,0.));
#33197=CARTESIAN_POINT('',(41.5,26.4873328464988,-18.8327161790004));
#33198=CARTESIAN_POINT('Origin',(41.5,27.2943217538007,-27.2943217538008));
#33199=CARTESIAN_POINT('',(41.5,29.553277056526,-13.5223450340618));
#33200=CARTESIAN_POINT('Origin',(41.5,0.,0.));
#33201=CARTESIAN_POINT('',(41.5,32.3550612130622,-3.06594421002716));
#33202=CARTESIAN_POINT('Origin',(41.5,37.284736894758,-9.99041514095732));
#33203=CARTESIAN_POINT('Origin',(41.5,0.,0.));
#33204=CARTESIAN_POINT('',(41.5,-14.,-1.71450551880629E-15));
#33205=CARTESIAN_POINT('Origin',(41.5,0.,0.));
#33206=CARTESIAN_POINT('Origin',(41.25,0.,0.));
#33207=CARTESIAN_POINT('',(41.,-32.8769019787977,2.84768612675768));
#33208=CARTESIAN_POINT('Ctrl Pts',(41.,-32.8769019787977,2.84768612675768));
#33209=CARTESIAN_POINT('Ctrl Pts',(41.0954573242615,-32.7640771770247,3.04406951423267));
#33210=CARTESIAN_POINT('Ctrl Pts',(41.1878146546253,-32.6518945010449,3.23933521449286));
#33211=CARTESIAN_POINT('',(41.,-32.8769019787977,-2.84768612675766));
#33212=CARTESIAN_POINT('Origin',(41.,0.,0.));
#33213=CARTESIAN_POINT('',(41.1878146339919,-32.6518945107659,-3.23933522040983));
#33214=CARTESIAN_POINT('Ctrl Pts',(41.1878146339919,-32.6518945107659,-3.23933522040983));
#33215=CARTESIAN_POINT('Ctrl Pts',(41.0954573053598,-32.7640771848917,-3.0440695229333));
#33216=CARTESIAN_POINT('Ctrl Pts',(41.,-32.8769019787977,-2.84768612675766));
#33217=CARTESIAN_POINT('Ctrl Pts',(41.5,-32.3550612130622,-3.06594421002715));
#33218=CARTESIAN_POINT('Ctrl Pts',(41.3957085374147,-32.4543894810395,-3.12325130089087));
#33219=CARTESIAN_POINT('Ctrl Pts',(41.2916417560968,-32.5533407332163,-3.18104335688356));
#33220=CARTESIAN_POINT('Ctrl Pts',(41.1878146339919,-32.6518945206304,-3.23933522607709));
#33221=CARTESIAN_POINT('Origin',(39.5,-32.6502398797874,3.24221525613642));
#33222=CARTESIAN_POINT('',(37.6890795305109,-32.4235777807772,3.63674438551517));
#33223=CARTESIAN_POINT('',(39.5,-32.4235777807772,3.63674438551517));
#33224=CARTESIAN_POINT('',(38.,-32.8769019787977,2.84768612675768));
#33225=CARTESIAN_POINT('Ctrl Pts',(37.6890795305109,-32.4235777807772,3.63674438551517));
#33226=CARTESIAN_POINT('Ctrl Pts',(37.8392820392454,-32.6489512516583,3.2444582483972));
#33227=CARTESIAN_POINT('Ctrl Pts',(38.,-32.8769019787977,2.84768612675768));
#33228=CARTESIAN_POINT('',(39.5,-32.8769019787977,2.84768612675768));
#33229=CARTESIAN_POINT('Origin',(36.8,27.2943217538007,27.2943217538007));
#33230=CARTESIAN_POINT('Ctrl Pts',(37.5,25.9430157904516,19.4092743732572));
#33231=CARTESIAN_POINT('Ctrl Pts',(37.5185015343068,25.9748214246282,19.4038236586252));
#33232=CARTESIAN_POINT('Ctrl Pts',(37.537045458494,26.0064935487318,19.3985939360341));
#33233=CARTESIAN_POINT('Ctrl Pts',(37.599346002575,26.1122358651254,19.3817798286965));
#33234=CARTESIAN_POINT('Ctrl Pts',(37.6438438231274,26.18666663184,19.3710168782449));
#33235=CARTESIAN_POINT('Ctrl Pts',(37.6890795305109,26.2612698469761,19.3613019153151));
#33236=CARTESIAN_POINT('Origin',(36.8,27.2943217538007,27.2943217538007));
#33237=CARTESIAN_POINT('Ctrl Pts',(37.6890795305109,19.3613019153151,26.2612698469761));
#33238=CARTESIAN_POINT('Ctrl Pts',(37.6438438231274,19.3710168782449,26.18666663184));
#33239=CARTESIAN_POINT('Ctrl Pts',(37.599346002575,19.3817798286965,26.1122358651254));
#33240=CARTESIAN_POINT('Ctrl Pts',(37.537045458494,19.3985939360341,26.0064935487318));
#33241=CARTESIAN_POINT('Ctrl Pts',(37.5185015343068,19.4038236586252,25.9748214246282));
#33242=CARTESIAN_POINT('Ctrl Pts',(37.5,19.4092743732572,25.9430157904516));
#33243=CARTESIAN_POINT('Origin',(36.8,37.284736894758,9.9904151409573));
#33244=CARTESIAN_POINT('',(37.6890795305109,32.4235777807772,3.63674438551515));
#33245=CARTESIAN_POINT('',(39.5,32.4235777807772,3.63674438551515));
#33246=CARTESIAN_POINT('Ctrl Pts',(37.5,32.1719479119405,3.83741678103717));
#33247=CARTESIAN_POINT('Ctrl Pts',(37.5185015343068,32.196767041805,3.8167935066088));
#33248=CARTESIAN_POINT('Ctrl Pts',(37.537045458494,32.2215810445749,3.79642837193837));
#33249=CARTESIAN_POINT('Ctrl Pts',(37.599346002575,32.304749523158,3.72899576964524));
#33250=CARTESIAN_POINT('Ctrl Pts',(37.6438438231274,32.3638269827301,3.6824593977772));
#33251=CARTESIAN_POINT('Ctrl Pts',(37.6890795305109,32.4235777807772,3.63674438551516));
#33252=CARTESIAN_POINT('Origin',(36.8,37.284736894758,9.9904151409573));
#33253=CARTESIAN_POINT('Ctrl Pts',(37.6890795305109,29.8980142324913,13.062275865462));
#33254=CARTESIAN_POINT('Ctrl Pts',(37.6438438231274,29.8691260296172,12.9928101044853));
#33255=CARTESIAN_POINT('Ctrl Pts',(37.599346002575,29.8412316347707,12.9229696944615));
#33256=CARTESIAN_POINT('Ctrl Pts',(37.537045458494,29.8029219206701,12.8229871085408));
#33257=CARTESIAN_POINT('Ctrl Pts',(37.5185015343068,29.791614931237,12.7929433831798));
#33258=CARTESIAN_POINT('Ctrl Pts',(37.5,29.7804325714888,12.7626735386834));
#33259=CARTESIAN_POINT('Origin',(39.5,32.6502398797874,3.24221525613641));
#33260=CARTESIAN_POINT('',(41.,32.8769019787977,2.84768612675766));
#33261=CARTESIAN_POINT('Ctrl Pts',(41.1878146546253,32.6518945010449,3.23933521449283));
#33262=CARTESIAN_POINT('Ctrl Pts',(41.0954573242617,32.7640771770245,3.04406951423305));
#33263=CARTESIAN_POINT('Ctrl Pts',(41.,32.8769019787977,2.84768612675766));
#33264=CARTESIAN_POINT('',(38.,32.8769019787977,2.84768612675766));
#33265=CARTESIAN_POINT('',(39.5,32.8769019787977,2.84768612675766));
#33266=CARTESIAN_POINT('Ctrl Pts',(38.,32.8769019787977,2.84768612675766));
#33267=CARTESIAN_POINT('Ctrl Pts',(37.8392820392456,32.6489512516586,3.24445824839666));
#33268=CARTESIAN_POINT('Ctrl Pts',(37.6890795305109,32.4235777807772,3.63674438551515));
#33269=CARTESIAN_POINT('Origin',(39.5,0.,0.));
#33270=CARTESIAN_POINT('Origin',(38.,0.,0.));
#33271=CARTESIAN_POINT('',(40.9,-32.9658914637539,-1.5));
#33272=CARTESIAN_POINT('Origin',(40.9,0.,0.));
#33273=CARTESIAN_POINT('',(38.,-32.9658914637539,-1.49999999999998));
#33274=CARTESIAN_POINT('Ctrl Pts',(40.9,-32.9658914637539,-1.5));
#33275=CARTESIAN_POINT('Ctrl Pts',(39.9333333333333,-32.9658914637539,-1.5));
#33276=CARTESIAN_POINT('Ctrl Pts',(38.9666666666667,-32.9658914637539,-1.5));
#33277=CARTESIAN_POINT('Ctrl Pts',(38.,-32.9658914637539,-1.5));
#33278=CARTESIAN_POINT('',(38.,-32.8769019787977,-2.84768612675766));
#33279=CARTESIAN_POINT('Origin',(38.,0.,0.));
#33280=CARTESIAN_POINT('',(39.5,-32.8769019787977,-2.84768612675766));
#33281=CARTESIAN_POINT('Origin',(39.5,-32.6502398797874,-3.2422152561364));
#33282=CARTESIAN_POINT('',(37.6890795305109,-32.4235777807772,-3.63674438551514));
#33283=CARTESIAN_POINT('Ctrl Pts',(38.,-32.8769019787977,-2.84768612675766));
#33284=CARTESIAN_POINT('Ctrl Pts',(37.8392820392454,-32.6489512516582,-3.24445824839731));
#33285=CARTESIAN_POINT('Ctrl Pts',(37.6890795305109,-32.4235777807772,-3.63674438551514));
#33286=CARTESIAN_POINT('',(41.,-32.4235777807772,-3.63674438551514));
#33287=CARTESIAN_POINT('',(39.5,-32.4235777807772,-3.63674438551514));
#33288=CARTESIAN_POINT('Ctrl Pts',(41.,-32.4235777807772,-3.63674438551515));
#33289=CARTESIAN_POINT('Ctrl Pts',(41.0874190154268,-32.5364116617262,-3.4403452176206));
#33290=CARTESIAN_POINT('Ctrl Pts',(41.1878146339919,-32.6518945107659,-3.23933522040983));
#33291=CARTESIAN_POINT('Origin',(41.25,-37.284736894758,-9.9904151409573));
#33292=CARTESIAN_POINT('',(41.,-29.8980142324913,-13.062275865462));
#33293=CARTESIAN_POINT('Origin',(41.,-37.284736894758,-9.9904151409573));
#33294=CARTESIAN_POINT('',(41.1878146546253,-29.8970377268407,-13.5206006633981));
#33295=CARTESIAN_POINT('Ctrl Pts',(41.,-29.8980142324913,-13.062275865462));
#33296=CARTESIAN_POINT('Ctrl Pts',(41.0874190341598,-29.8975316444848,-13.2887794709034));
#33297=CARTESIAN_POINT('Ctrl Pts',(41.1878146546253,-29.8970377268407,-13.5206006633981));
#33298=CARTESIAN_POINT('Ctrl Pts',(41.1878146546253,-29.8970377268407,-13.5206006633982));
#33299=CARTESIAN_POINT('Ctrl Pts',(41.2916290694684,-29.7825557217404,-13.5218058616421));
#33300=CARTESIAN_POINT('Ctrl Pts',(41.3956920266496,-29.6679695598581,-13.5223797770449));
#33301=CARTESIAN_POINT('Ctrl Pts',(41.5,-29.553277056526,-13.5223450340618));
#33302=CARTESIAN_POINT('Origin',(41.25,0.,0.));
#33303=CARTESIAN_POINT('',(41.,-29.8960753747485,-13.9722824616222));
#33304=CARTESIAN_POINT('Ctrl Pts',(41.,-29.8960753747485,-13.9722824616222));
#33305=CARTESIAN_POINT('Ctrl Pts',(41.0954573242615,-29.8965579239737,-13.7457970583011));
#33306=CARTESIAN_POINT('Ctrl Pts',(41.1878146546253,-29.8970377268408,-13.5206006633981));
#33307=CARTESIAN_POINT('',(41.,-27.0483892479909,-18.9046195171755));
#33308=CARTESIAN_POINT('Origin',(41.,0.,0.));
#33309=CARTESIAN_POINT('',(41.1878146339919,-26.657702517808,-19.1312938476315));
#33310=CARTESIAN_POINT('Ctrl Pts',(41.1878146339919,-26.657702517808,-19.1312938476315));
#33311=CARTESIAN_POINT('Ctrl Pts',(41.0954573053599,-26.8524884122035,-19.0182801301921));
#33312=CARTESIAN_POINT('Ctrl Pts',(41.,-27.0483892479909,-18.9046195171755));
#33313=CARTESIAN_POINT('Ctrl Pts',(41.5,-26.4873328464988,-18.8327161790004));
#33314=CARTESIAN_POINT('Ctrl Pts',(41.3957085374147,-26.5447001044493,-18.9320097094941));
#33315=CARTESIAN_POINT('Ctrl Pts',(41.2916417560968,-26.6014983745743,-19.031534724209));
#33316=CARTESIAN_POINT('Ctrl Pts',(41.1878146339919,-26.6577025235173,-19.1312938574718));
#33317=CARTESIAN_POINT('Origin',(39.5,-29.8970448036199,-13.5172791635421));
#33318=CARTESIAN_POINT('',(37.6890795305109,-29.8980142324913,-13.062275865462));
#33319=CARTESIAN_POINT('',(39.5,-29.8980142324913,-13.062275865462));
#33320=CARTESIAN_POINT('',(38.,-29.8960753747485,-13.9722824616222));
#33321=CARTESIAN_POINT('Ctrl Pts',(37.6890795305109,-29.8980142324913,-13.062275865462));
#33322=CARTESIAN_POINT('Ctrl Pts',(37.8392820392454,-29.8970503150544,-13.5146923611991));
#33323=CARTESIAN_POINT('Ctrl Pts',(38.,-29.8960753747485,-13.9722824616222));
#33324=CARTESIAN_POINT('',(39.5,-29.8960753747485,-13.9722824616222));
#33325=CARTESIAN_POINT('Origin',(39.5,0.,0.));
#33326=CARTESIAN_POINT('Origin',(38.,0.,0.));
#33327=CARTESIAN_POINT('',(40.9,-27.7992994660114,-17.7819838375536));
#33328=CARTESIAN_POINT('Origin',(40.9,0.,0.));
#33329=CARTESIAN_POINT('',(38.,-27.7992994660114,-17.7819838375536));
#33330=CARTESIAN_POINT('Ctrl Pts',(40.9,-27.7992994660114,-17.7819838375536));
#33331=CARTESIAN_POINT('Ctrl Pts',(39.9333333333333,-27.7992994660114,-17.7819838375536));
#33332=CARTESIAN_POINT('Ctrl Pts',(38.9666666666667,-27.7992994660114,-17.7819838375536));
#33333=CARTESIAN_POINT('Ctrl Pts',(38.,-27.7992994660114,-17.7819838375536));
#33334=CARTESIAN_POINT('',(38.,-27.0483892479909,-18.9046195171755));
#33335=CARTESIAN_POINT('Origin',(38.,0.,0.));
#33336=CARTESIAN_POINT('',(39.5,-27.0483892479909,-18.9046195171755));
#33337=CARTESIAN_POINT('Origin',(39.5,-26.6548295474835,-19.1329607162453));
#33338=CARTESIAN_POINT('',(37.6890795305109,-26.2612698469761,-19.3613019153151));
#33339=CARTESIAN_POINT('Ctrl Pts',(38.,-27.0483892479909,-18.9046195171755));
#33340=CARTESIAN_POINT('Ctrl Pts',(37.8392820392455,-26.6525920666573,-19.134258890459));
#33341=CARTESIAN_POINT('Ctrl Pts',(37.6890795305109,-26.2612698469761,-19.3613019153151));
#33342=CARTESIAN_POINT('',(41.,-26.2612698469761,-19.3613019153151));
#33343=CARTESIAN_POINT('',(39.5,-26.2612698469761,-19.3613019153151));
#33344=CARTESIAN_POINT('Ctrl Pts',(41.,-26.2612698469761,-19.3613019153151));
#33345=CARTESIAN_POINT('Ctrl Pts',(41.0874190154268,-26.4571864382328,-19.2476321871108));
#33346=CARTESIAN_POINT('Ctrl Pts',(41.1878146339919,-26.657702517808,-19.1312938476315));
#33347=CARTESIAN_POINT('Origin',(41.25,-27.2943217538008,-27.2943217538007));
#33348=CARTESIAN_POINT('',(41.,-19.3613019153151,-26.2612698469761));
#33349=CARTESIAN_POINT('Origin',(41.,-27.2943217538008,-27.2943217538007));
#33350=CARTESIAN_POINT('',(41.1878146546253,-19.1312938376468,-26.6577025123479));
#33351=CARTESIAN_POINT('Ctrl Pts',(41.,-19.3613019153151,-26.2612698469761));
#33352=CARTESIAN_POINT('Ctrl Pts',(41.0874190341598,-19.2476321791213,-26.4571864293338));
#33353=CARTESIAN_POINT('Ctrl Pts',(41.1878146546253,-19.1312938376468,-26.6577025123479));
#33354=CARTESIAN_POINT('Ctrl Pts',(41.1878146546253,-19.1312938376468,-26.6577025123479));
#33355=CARTESIAN_POINT('Ctrl Pts',(41.2916290694684,-19.0315469138318,-26.6015052420936));
#33356=CARTESIAN_POINT('Ctrl Pts',(41.3956920266496,-18.9320254290181,-26.5447091864709));
#33357=CARTESIAN_POINT('Ctrl Pts',(41.5,-18.8327161790004,-26.4873328464988));
#33358=CARTESIAN_POINT('Origin',(41.25,0.,0.));
#33359=CARTESIAN_POINT('',(41.,-18.9046195171755,-27.0483892479908));
#33360=CARTESIAN_POINT('Ctrl Pts',(41.,-18.9046195171755,-27.0483892479908));
#33361=CARTESIAN_POINT('Ctrl Pts',(41.0954573242616,-19.0182801187237,-26.8524884097409));
#33362=CARTESIAN_POINT('Ctrl Pts',(41.1878146546253,-19.1312938376468,-26.6577025123479));
#33363=CARTESIAN_POINT('',(41.,-13.9722824616222,-29.8960753747485));
#33364=CARTESIAN_POINT('Origin',(41.,0.,0.));
#33365=CARTESIAN_POINT('',(41.1878146339919,-13.5206006631344,-29.8970377382179));
#33366=CARTESIAN_POINT('Ctrl Pts',(41.1878146339919,-13.5206006631344,-29.8970377382179));
#33367=CARTESIAN_POINT('Ctrl Pts',(41.0954573053598,-13.7457970546997,-29.8965579351369));
#33368=CARTESIAN_POINT('Ctrl Pts',(41.,-13.9722824616222,-29.8960753747485));
#33369=CARTESIAN_POINT('Ctrl Pts',(41.5,-13.5223450340618,-29.553277056526));
#33370=CARTESIAN_POINT('Ctrl Pts',(41.3957085374147,-13.5223797715455,-29.6679514053401));
#33371=CARTESIAN_POINT('Ctrl Pts',(41.2916417560968,-13.5218060090073,-29.7825417314578));
#33372=CARTESIAN_POINT('Ctrl Pts',(41.1878146339919,-13.5206006631586,-29.8970377495944));
#33373=CARTESIAN_POINT('Origin',(39.5,-19.1329607162453,-26.6548295474835));
#33374=CARTESIAN_POINT('',(37.6890795305109,-19.3613019153152,-26.2612698469761));
#33375=CARTESIAN_POINT('',(39.5,-19.3613019153151,-26.2612698469761));
#33376=CARTESIAN_POINT('',(38.,-18.9046195171755,-27.0483892479908));
#33377=CARTESIAN_POINT('Ctrl Pts',(37.6890795305109,-19.3613019153152,-26.2612698469761));
#33378=CARTESIAN_POINT('Ctrl Pts',(37.8392820392454,-19.1342588904591,-26.6525920666571));
#33379=CARTESIAN_POINT('Ctrl Pts',(38.,-18.9046195171755,-27.0483892479908));
#33380=CARTESIAN_POINT('',(39.5,-18.9046195171755,-27.0483892479908));
#33381=CARTESIAN_POINT('Origin',(39.5,0.,0.));
#33382=CARTESIAN_POINT('Origin',(38.,0.,0.));
#33383=CARTESIAN_POINT('',(40.9,-15.1839076262003,-29.2992994660114));
#33384=CARTESIAN_POINT('Origin',(40.9,0.,0.));
#33385=CARTESIAN_POINT('',(38.,-15.1839076262003,-29.2992994660114));
#33386=CARTESIAN_POINT('Ctrl Pts',(40.9,-15.1839076262003,-29.2992994660114));
#33387=CARTESIAN_POINT('Ctrl Pts',(39.9333333333333,-15.1839076262003,-29.2992994660114));
#33388=CARTESIAN_POINT('Ctrl Pts',(38.9666666666667,-15.1839076262003,-29.2992994660114));
#33389=CARTESIAN_POINT('Ctrl Pts',(38.,-15.1839076262003,-29.2992994660114));
#33390=CARTESIAN_POINT('',(38.,-13.9722824616222,-29.8960753747485));
#33391=CARTESIAN_POINT('Origin',(38.,0.,0.));
#33392=CARTESIAN_POINT('',(39.5,-13.9722824616222,-29.8960753747485));
#33393=CARTESIAN_POINT('Origin',(39.5,-13.5172791635421,-29.8970448036199));
#33394=CARTESIAN_POINT('',(37.6890795305109,-13.0622758654621,-29.8980142324913));
#33395=CARTESIAN_POINT('Ctrl Pts',(38.,-13.9722824616222,-29.8960753747485));
#33396=CARTESIAN_POINT('Ctrl Pts',(37.8392820392453,-13.5146923611989,-29.8970503150544));
#33397=CARTESIAN_POINT('Ctrl Pts',(37.6890795305109,-13.0622758654621,-29.8980142324913));
#33398=CARTESIAN_POINT('',(41.,-13.0622758654621,-29.8980142324913));
#33399=CARTESIAN_POINT('',(39.5,-13.0622758654621,-29.8980142324913));
#33400=CARTESIAN_POINT('Ctrl Pts',(41.,-13.0622758654621,-29.8980142324913));
#33401=CARTESIAN_POINT('Ctrl Pts',(41.0874190154268,-13.2887794746153,-29.8975316558534));
#33402=CARTESIAN_POINT('Ctrl Pts',(41.1878146339919,-13.5206006631344,-29.8970377382179));
#33403=CARTESIAN_POINT('Origin',(41.25,-9.99041514095732,-37.284736894758));
#33404=CARTESIAN_POINT('',(41.,-3.63674438551517,-32.4235777807772));
#33405=CARTESIAN_POINT('Origin',(41.,-9.99041514095732,-37.284736894758));
#33406=CARTESIAN_POINT('',(41.1878146546253,-3.23933521449285,-32.6518945010449));
#33407=CARTESIAN_POINT('Ctrl Pts',(41.,-3.63674438551517,-32.4235777807772));
#33408=CARTESIAN_POINT('Ctrl Pts',(41.0874190341598,-3.44034521515094,-32.5364116500246));
#33409=CARTESIAN_POINT('Ctrl Pts',(41.1878146546253,-3.23933521449285,-32.6518945010449));
#33410=CARTESIAN_POINT('Ctrl Pts',(41.1878146546253,-3.23933521449285,-32.6518945010449));
#33411=CARTESIAN_POINT('Ctrl Pts',(41.2916290694684,-3.18105047964687,-32.5533527754738));
#33412=CARTESIAN_POINT('Ctrl Pts',(41.3956920266496,-3.12326037338726,-32.454405206063));
#33413=CARTESIAN_POINT('Ctrl Pts',(41.5,-3.06594421002717,-32.3550612130622));
#33414=CARTESIAN_POINT('Origin',(41.25,0.,0.));
#33415=CARTESIAN_POINT('',(41.,-2.84768612675768,-32.8769019787977));
#33416=CARTESIAN_POINT('Ctrl Pts',(41.,-2.84768612675768,-32.8769019787977));
#33417=CARTESIAN_POINT('Ctrl Pts',(41.0954573242614,-3.04406951423239,-32.7640771770249));
#33418=CARTESIAN_POINT('Ctrl Pts',(41.1878146546253,-3.23933521449284,-32.6518945010449));
#33419=CARTESIAN_POINT('',(41.,2.84768612675766,-32.8769019787977));
#33420=CARTESIAN_POINT('Origin',(41.,0.,0.));
#33421=CARTESIAN_POINT('',(41.1878146339919,3.23933522040982,-32.6518945107659));
#33422=CARTESIAN_POINT('Ctrl Pts',(41.1878146339919,3.23933522040982,-32.6518945107659));
#33423=CARTESIAN_POINT('Ctrl Pts',(41.0954573053598,3.04406952293321,-32.7640771848917));
#33424=CARTESIAN_POINT('Ctrl Pts',(41.,2.84768612675766,-32.8769019787977));
#33425=CARTESIAN_POINT('Ctrl Pts',(41.5,3.06594421002715,-32.3550612130622));
#33426=CARTESIAN_POINT('Ctrl Pts',(41.3957085374147,3.12325130089087,-32.4543894810395));
#33427=CARTESIAN_POINT('Ctrl Pts',(41.2916417560968,3.18104335688356,-32.5533407332163));
#33428=CARTESIAN_POINT('Ctrl Pts',(41.1878146339919,3.2393352260771,-32.6518945206304));
#33429=CARTESIAN_POINT('Origin',(39.5,-3.24221525613642,-32.6502398797874));
#33430=CARTESIAN_POINT('',(37.6890795305109,-3.63674438551517,-32.4235777807772));
#33431=CARTESIAN_POINT('',(39.5,-3.63674438551517,-32.4235777807772));
#33432=CARTESIAN_POINT('',(38.,-2.84768612675768,-32.8769019787977));
#33433=CARTESIAN_POINT('Ctrl Pts',(37.6890795305109,-3.63674438551517,-32.4235777807772));
#33434=CARTESIAN_POINT('Ctrl Pts',(37.8392820392455,-3.24445824839701,-32.6489512516584));
#33435=CARTESIAN_POINT('Ctrl Pts',(38.,-2.84768612675768,-32.8769019787977));
#33436=CARTESIAN_POINT('',(39.5,-2.84768612675768,-32.8769019787977));
#33437=CARTESIAN_POINT('Origin',(39.5,0.,0.));
#33438=CARTESIAN_POINT('Origin',(38.,0.,0.));
#33439=CARTESIAN_POINT('',(40.9,1.5,-32.9658914637539));
#33440=CARTESIAN_POINT('Origin',(40.9,0.,0.));
#33441=CARTESIAN_POINT('',(38.,1.49999999999998,-32.9658914637539));
#33442=CARTESIAN_POINT('Ctrl Pts',(40.9,1.49999999999999,-32.9658914637539));
#33443=CARTESIAN_POINT('Ctrl Pts',(39.9333333333333,1.49999999999999,-32.9658914637539));
#33444=CARTESIAN_POINT('Ctrl Pts',(38.9666666666667,1.49999999999999,-32.9658914637539));
#33445=CARTESIAN_POINT('Ctrl Pts',(38.,1.49999999999999,-32.9658914637539));
#33446=CARTESIAN_POINT('',(38.,2.84768612675766,-32.8769019787977));
#33447=CARTESIAN_POINT('Origin',(38.,0.,0.));
#33448=CARTESIAN_POINT('',(39.5,2.84768612675766,-32.8769019787977));
#33449=CARTESIAN_POINT('Origin',(39.5,3.2422152561364,-32.6502398797874));
#33450=CARTESIAN_POINT('',(37.6890795305109,3.63674438551514,-32.4235777807772));
#33451=CARTESIAN_POINT('Ctrl Pts',(38.,2.84768612675766,-32.8769019787977));
#33452=CARTESIAN_POINT('Ctrl Pts',(37.8392820392455,3.24445824839707,-32.6489512516583));
#33453=CARTESIAN_POINT('Ctrl Pts',(37.6890795305109,3.63674438551514,-32.4235777807772));
#33454=CARTESIAN_POINT('',(41.,3.63674438551514,-32.4235777807772));
#33455=CARTESIAN_POINT('',(39.5,3.63674438551514,-32.4235777807772));
#33456=CARTESIAN_POINT('Ctrl Pts',(41.,3.63674438551514,-32.4235777807772));
#33457=CARTESIAN_POINT('Ctrl Pts',(41.0874190154268,3.44034521762059,-32.5364116617262));
#33458=CARTESIAN_POINT('Ctrl Pts',(41.1878146339919,3.23933522040982,-32.6518945107659));
#33459=CARTESIAN_POINT('Origin',(41.25,9.99041514095729,-37.284736894758));
#33460=CARTESIAN_POINT('',(41.,13.0622758654621,-29.8980142324913));
#33461=CARTESIAN_POINT('Origin',(41.,9.99041514095729,-37.284736894758));
#33462=CARTESIAN_POINT('',(41.1878146546253,13.5206006633982,-29.8970377268407));
#33463=CARTESIAN_POINT('Ctrl Pts',(41.,13.0622758654621,-29.8980142324913));
#33464=CARTESIAN_POINT('Ctrl Pts',(41.0874190341598,13.2887794709034,-29.8975316444848));
#33465=CARTESIAN_POINT('Ctrl Pts',(41.1878146546253,13.5206006633982,-29.8970377268407));
#33466=CARTESIAN_POINT('Ctrl Pts',(41.1878146546253,13.5206006633982,-29.8970377268407));
#33467=CARTESIAN_POINT('Ctrl Pts',(41.2916290694684,13.5218058616421,-29.7825557217404));
#33468=CARTESIAN_POINT('Ctrl Pts',(41.3956920266496,13.5223797770449,-29.6679695598581));
#33469=CARTESIAN_POINT('Ctrl Pts',(41.5,13.5223450340618,-29.553277056526));
#33470=CARTESIAN_POINT('Origin',(41.25,0.,0.));
#33471=CARTESIAN_POINT('',(41.,13.9722824616222,-29.8960753747485));
#33472=CARTESIAN_POINT('Ctrl Pts',(41.,13.9722824616222,-29.8960753747485));
#33473=CARTESIAN_POINT('Ctrl Pts',(41.0954573242616,13.745797058301,-29.8965579239736));
#33474=CARTESIAN_POINT('Ctrl Pts',(41.1878146546253,13.5206006633982,-29.8970377268407));
#33475=CARTESIAN_POINT('',(41.,18.9046195171755,-27.0483892479909));
#33476=CARTESIAN_POINT('Origin',(41.,0.,0.));
#33477=CARTESIAN_POINT('',(41.1878146339919,19.1312938476315,-26.6577025178081));
#33478=CARTESIAN_POINT('Ctrl Pts',(41.1878146339919,19.1312938476315,-26.6577025178081));
#33479=CARTESIAN_POINT('Ctrl Pts',(41.09545730536,19.0182801301922,-26.8524884122034));
#33480=CARTESIAN_POINT('Ctrl Pts',(41.,18.9046195171755,-27.0483892479909));
#33481=CARTESIAN_POINT('Ctrl Pts',(41.5,18.8327161790004,-26.4873328464988));
#33482=CARTESIAN_POINT('Ctrl Pts',(41.3957085374147,18.932009709494,-26.5447001044493));
#33483=CARTESIAN_POINT('Ctrl Pts',(41.2916417560968,19.031534724209,-26.6014983745743));
#33484=CARTESIAN_POINT('Ctrl Pts',(41.1878146339919,19.1312938574718,-26.6577025235173));
#33485=CARTESIAN_POINT('Origin',(39.5,13.5172791635421,-29.8970448036199));
#33486=CARTESIAN_POINT('',(37.6890795305109,13.0622758654621,-29.8980142324913));
#33487=CARTESIAN_POINT('',(39.5,13.0622758654621,-29.8980142324913));
#33488=CARTESIAN_POINT('',(38.,13.9722824616222,-29.8960753747485));
#33489=CARTESIAN_POINT('Ctrl Pts',(37.6890795305109,13.0622758654621,-29.8980142324913));
#33490=CARTESIAN_POINT('Ctrl Pts',(37.8392820392456,13.5146923611998,-29.8970503150544));
#33491=CARTESIAN_POINT('Ctrl Pts',(38.,13.9722824616222,-29.8960753747485));
#33492=CARTESIAN_POINT('',(39.5,13.9722824616222,-29.8960753747485));
#33493=CARTESIAN_POINT('Origin',(39.5,0.,0.));
#33494=CARTESIAN_POINT('Origin',(38.,0.,0.));
#33495=CARTESIAN_POINT('',(40.9,17.7819838375536,-27.7992994660114));
#33496=CARTESIAN_POINT('Origin',(40.9,0.,0.));
#33497=CARTESIAN_POINT('',(38.,17.7819838375536,-27.7992994660114));
#33498=CARTESIAN_POINT('Ctrl Pts',(40.9,17.7819838375536,-27.7992994660114));
#33499=CARTESIAN_POINT('Ctrl Pts',(39.9333333333333,17.7819838375536,-27.7992994660114));
#33500=CARTESIAN_POINT('Ctrl Pts',(38.9666666666667,17.7819838375536,-27.7992994660114));
#33501=CARTESIAN_POINT('Ctrl Pts',(38.,17.7819838375536,-27.7992994660114));
#33502=CARTESIAN_POINT('',(38.,18.9046195171755,-27.0483892479909));
#33503=CARTESIAN_POINT('Origin',(38.,0.,0.));
#33504=CARTESIAN_POINT('',(39.5,18.9046195171755,-27.0483892479909));
#33505=CARTESIAN_POINT('Origin',(39.5,19.1329607162453,-26.6548295474835));
#33506=CARTESIAN_POINT('',(37.6890795305109,19.3613019153151,-26.2612698469762));
#33507=CARTESIAN_POINT('Ctrl Pts',(38.,18.9046195171755,-27.0483892479909));
#33508=CARTESIAN_POINT('Ctrl Pts',(37.8392820392454,19.1342588904591,-26.6525920666571));
#33509=CARTESIAN_POINT('Ctrl Pts',(37.6890795305109,19.3613019153151,-26.2612698469762));
#33510=CARTESIAN_POINT('',(41.,19.3613019153151,-26.2612698469762));
#33511=CARTESIAN_POINT('',(39.5,19.3613019153151,-26.2612698469762));
#33512=CARTESIAN_POINT('Ctrl Pts',(41.,19.3613019153151,-26.2612698469762));
#33513=CARTESIAN_POINT('Ctrl Pts',(41.0874190154268,19.2476321871109,-26.4571864382327));
#33514=CARTESIAN_POINT('Ctrl Pts',(41.1878146339919,19.1312938476315,-26.6577025178081));
#33515=CARTESIAN_POINT('Origin',(41.25,27.2943217538007,-27.2943217538008));
#33516=CARTESIAN_POINT('',(41.,26.2612698469761,-19.3613019153152));
#33517=CARTESIAN_POINT('Origin',(41.,27.2943217538007,-27.2943217538008));
#33518=CARTESIAN_POINT('',(41.1878146546253,26.6577025123479,-19.1312938376468));
#33519=CARTESIAN_POINT('Ctrl Pts',(41.,26.2612698469761,-19.3613019153152));
#33520=CARTESIAN_POINT('Ctrl Pts',(41.0874190341598,26.4571864293338,-19.2476321791213));
#33521=CARTESIAN_POINT('Ctrl Pts',(41.1878146546253,26.6577025123479,-19.1312938376468));
#33522=CARTESIAN_POINT('Ctrl Pts',(41.1878146546253,26.6577025123479,-19.1312938376468));
#33523=CARTESIAN_POINT('Ctrl Pts',(41.2916290694684,26.6015052420936,-19.0315469138318));
#33524=CARTESIAN_POINT('Ctrl Pts',(41.3956920266496,26.5447091864709,-18.9320254290182));
#33525=CARTESIAN_POINT('Ctrl Pts',(41.5,26.4873328464988,-18.8327161790004));
#33526=CARTESIAN_POINT('Origin',(41.25,0.,0.));
#33527=CARTESIAN_POINT('',(41.,27.0483892479908,-18.9046195171755));
#33528=CARTESIAN_POINT('Ctrl Pts',(41.,27.0483892479908,-18.9046195171755));
#33529=CARTESIAN_POINT('Ctrl Pts',(41.0954573242615,26.852488409741,-19.0182801187236));
#33530=CARTESIAN_POINT('Ctrl Pts',(41.1878146546253,26.6577025123479,-19.1312938376468));
#33531=CARTESIAN_POINT('',(41.,29.8960753747485,-13.9722824616222));
#33532=CARTESIAN_POINT('Origin',(41.,0.,0.));
#33533=CARTESIAN_POINT('',(41.1878146339919,29.8970377382179,-13.5206006631344));
#33534=CARTESIAN_POINT('Ctrl Pts',(41.1878146339919,29.8970377382179,-13.5206006631344));
#33535=CARTESIAN_POINT('Ctrl Pts',(41.0954573053599,29.8965579351369,-13.7457970546994));
#33536=CARTESIAN_POINT('Ctrl Pts',(41.,29.8960753747485,-13.9722824616222));
#33537=CARTESIAN_POINT('Ctrl Pts',(41.5,29.553277056526,-13.5223450340618));
#33538=CARTESIAN_POINT('Ctrl Pts',(41.3957085374147,29.6679514053401,-13.5223797715455));
#33539=CARTESIAN_POINT('Ctrl Pts',(41.2916417560968,29.7825417314578,-13.5218060090073));
#33540=CARTESIAN_POINT('Ctrl Pts',(41.1878146339919,29.8970377495944,-13.5206006631586));
#33541=CARTESIAN_POINT('Origin',(39.5,26.6548295474835,-19.1329607162453));
#33542=CARTESIAN_POINT('',(37.6890795305109,26.2612698469761,-19.3613019153152));
#33543=CARTESIAN_POINT('',(39.5,26.2612698469761,-19.3613019153152));
#33544=CARTESIAN_POINT('',(38.,27.0483892479908,-18.9046195171755));
#33545=CARTESIAN_POINT('Ctrl Pts',(37.6890795305109,26.2612698469761,-19.3613019153152));
#33546=CARTESIAN_POINT('Ctrl Pts',(37.8392820392455,26.6525920666573,-19.1342588904591));
#33547=CARTESIAN_POINT('Ctrl Pts',(38.,27.0483892479908,-18.9046195171755));
#33548=CARTESIAN_POINT('',(39.5,27.0483892479908,-18.9046195171755));
#33549=CARTESIAN_POINT('Origin',(39.5,0.,0.));
#33550=CARTESIAN_POINT('',(41.,32.8769019787977,-2.84768612675768));
#33551=CARTESIAN_POINT('Origin',(41.,0.,0.));
#33552=CARTESIAN_POINT('',(38.,32.8769019787977,-2.84768612675768));
#33553=CARTESIAN_POINT('',(39.5,32.8769019787977,-2.84768612675768));
#33554=CARTESIAN_POINT('Origin',(38.,0.,0.));
#33555=CARTESIAN_POINT('',(40.9,32.9658914637539,1.5));
#33556=CARTESIAN_POINT('Origin',(40.9,0.,0.));
#33557=CARTESIAN_POINT('',(38.,32.9658914637539,1.5));
#33558=CARTESIAN_POINT('Ctrl Pts',(40.9,32.9658914637539,1.5));
#33559=CARTESIAN_POINT('Ctrl Pts',(39.9333333333333,32.9658914637539,1.5));
#33560=CARTESIAN_POINT('Ctrl Pts',(38.9666666666667,32.9658914637539,1.5));
#33561=CARTESIAN_POINT('Ctrl Pts',(38.,32.9658914637539,1.5));
#33562=CARTESIAN_POINT('Origin',(38.,0.,0.));
#33563=CARTESIAN_POINT('Origin',(41.25,0.,0.));
#33564=CARTESIAN_POINT('',(41.1878146546253,32.6518945010449,-3.23933521449284));
#33565=CARTESIAN_POINT('Ctrl Pts',(41.1878146546253,32.6518945010449,-3.23933521449285));
#33566=CARTESIAN_POINT('Ctrl Pts',(41.2916290694684,32.5533527754738,-3.18105047964687));
#33567=CARTESIAN_POINT('Ctrl Pts',(41.3956920266496,32.454405206063,-3.12326037338726));
#33568=CARTESIAN_POINT('Ctrl Pts',(41.5,32.3550612130622,-3.06594421002717));
#33569=CARTESIAN_POINT('Ctrl Pts',(41.,32.8769019787977,-2.84768612675768));
#33570=CARTESIAN_POINT('Ctrl Pts',(41.0954573242615,32.7640771770247,-3.04406951423265));
#33571=CARTESIAN_POINT('Ctrl Pts',(41.1878146546253,32.6518945010449,-3.23933521449285));
#33572=CARTESIAN_POINT('Origin',(39.5,0.,0.));
#33573=CARTESIAN_POINT('Origin',(38.,0.,0.));
#33574=CARTESIAN_POINT('',(40.9,29.2992994660114,-15.1839076262003));
#33575=CARTESIAN_POINT('Origin',(40.9,0.,0.));
#33576=CARTESIAN_POINT('',(38.,29.2992994660114,-15.1839076262003));
#33577=CARTESIAN_POINT('Ctrl Pts',(40.9,29.2992994660114,-15.1839076262003));
#33578=CARTESIAN_POINT('Ctrl Pts',(39.9333333333333,29.2992994660114,-15.1839076262003));
#33579=CARTESIAN_POINT('Ctrl Pts',(38.9666666666667,29.2992994660114,-15.1839076262003));
#33580=CARTESIAN_POINT('Ctrl Pts',(38.,29.2992994660114,-15.1839076262003));
#33581=CARTESIAN_POINT('',(38.,29.8960753747485,-13.9722824616222));
#33582=CARTESIAN_POINT('Origin',(38.,0.,0.));
#33583=CARTESIAN_POINT('',(39.5,29.8960753747485,-13.9722824616222));
#33584=CARTESIAN_POINT('Origin',(39.5,29.8970448036199,-13.5172791635421));
#33585=CARTESIAN_POINT('',(37.6890795305109,29.8980142324913,-13.0622758654621));
#33586=CARTESIAN_POINT('Ctrl Pts',(38.,29.8960753747485,-13.9722824616222));
#33587=CARTESIAN_POINT('Ctrl Pts',(37.8392820392455,29.8970503150544,-13.5146923611996));
#33588=CARTESIAN_POINT('Ctrl Pts',(37.6890795305109,29.8980142324913,-13.0622758654621));
#33589=CARTESIAN_POINT('',(41.,29.8980142324913,-13.0622758654621));
#33590=CARTESIAN_POINT('',(39.5,29.8980142324913,-13.0622758654621));
#33591=CARTESIAN_POINT('Ctrl Pts',(41.,29.8980142324913,-13.0622758654621));
#33592=CARTESIAN_POINT('Ctrl Pts',(41.0874190154268,29.8975316558534,-13.2887794746153));
#33593=CARTESIAN_POINT('Ctrl Pts',(41.1878146339919,29.8970377382179,-13.5206006631344));
#33594=CARTESIAN_POINT('Origin',(41.25,37.284736894758,-9.99041514095732));
#33595=CARTESIAN_POINT('',(41.,32.4235777807772,-3.63674438551517));
#33596=CARTESIAN_POINT('Origin',(41.,37.284736894758,-9.99041514095732));
#33597=CARTESIAN_POINT('Ctrl Pts',(41.,32.4235777807772,-3.63674438551517));
#33598=CARTESIAN_POINT('Ctrl Pts',(41.0874190341598,32.5364116500246,-3.44034521515093));
#33599=CARTESIAN_POINT('Ctrl Pts',(41.1878146546253,32.6518945010449,-3.23933521449284));
#33600=CARTESIAN_POINT('Origin',(39.5,32.6502398797874,-3.24221525613642));
#33601=CARTESIAN_POINT('',(37.6890795305109,32.4235777807772,-3.63674438551517));
#33602=CARTESIAN_POINT('',(39.5,32.4235777807772,-3.63674438551517));
#33603=CARTESIAN_POINT('Ctrl Pts',(37.6890795305109,32.4235777807772,-3.63674438551517));
#33604=CARTESIAN_POINT('Ctrl Pts',(37.8392820392455,32.6489512516583,-3.24445824839707));
#33605=CARTESIAN_POINT('Ctrl Pts',(38.,32.8769019787977,-2.84768612675768));
#33606=CARTESIAN_POINT('Origin',(37.75,0.,0.));
#33607=CARTESIAN_POINT('',(37.5,32.1719479119405,-3.83741678103716));
#33608=CARTESIAN_POINT('Ctrl Pts',(37.6890795305109,32.4235777807772,-3.63674438551516));
#33609=CARTESIAN_POINT('Ctrl Pts',(37.6438438231274,32.3638269827301,-3.68245939777721));
#33610=CARTESIAN_POINT('Ctrl Pts',(37.599346002575,32.304749523158,-3.72899576964525));
#33611=CARTESIAN_POINT('Ctrl Pts',(37.537045458494,32.2215810445749,-3.79642837193839));
#33612=CARTESIAN_POINT('Ctrl Pts',(37.5185015343068,32.196767041805,-3.81679350660881));
#33613=CARTESIAN_POINT('Ctrl Pts',(37.5,32.1719479119405,-3.83741678103718));
#33614=CARTESIAN_POINT('Origin',(37.5,0.,0.));
#33615=CARTESIAN_POINT('Origin',(36.8,37.284736894758,-9.99041514095732));
#33616=CARTESIAN_POINT('',(37.5,29.7804325714888,-12.7626735386834));
#33617=CARTESIAN_POINT('Ctrl Pts',(37.5,29.7804325714888,-12.7626735386834));
#33618=CARTESIAN_POINT('Ctrl Pts',(37.5185015343068,29.791614931237,-12.7929433831798));
#33619=CARTESIAN_POINT('Ctrl Pts',(37.537045458494,29.8029219206701,-12.8229871085408));
#33620=CARTESIAN_POINT('Ctrl Pts',(37.599346002575,29.8412316347707,-12.9229696944615));
#33621=CARTESIAN_POINT('Ctrl Pts',(37.6438438231274,29.8691260296172,-12.9928101044853));
#33622=CARTESIAN_POINT('Ctrl Pts',(37.6890795305109,29.8980142324913,-13.0622758654621));
#33623=CARTESIAN_POINT('',(36.8,29.4900464626661,-11.7911930472673));
#33624=CARTESIAN_POINT('Ctrl Pts',(36.8,29.4900464626661,-11.7911930472673));
#33625=CARTESIAN_POINT('Ctrl Pts',(37.0122659037828,29.5692859507914,-12.1341821953296));
#33626=CARTESIAN_POINT('Ctrl Pts',(37.2470086540955,29.6681218786624,-12.458656561616));
#33627=CARTESIAN_POINT('Ctrl Pts',(37.5,29.7804325714888,-12.7626735386834));
#33628=CARTESIAN_POINT('',(36.8,31.4347259190859,-4.53355051147316));
#33629=CARTESIAN_POINT('Origin',(36.8,37.284736894758,-9.99041514095732));
#33630=CARTESIAN_POINT('Ctrl Pts',(37.5,32.1719479119405,-3.83741678103719));
#33631=CARTESIAN_POINT('Ctrl Pts',(37.2470086540956,31.9226755103027,-4.04454785994595));
#33632=CARTESIAN_POINT('Ctrl Pts',(37.0122659037829,31.6748439028165,-4.27613294009144));
#33633=CARTESIAN_POINT('Ctrl Pts',(36.8,31.4347259190859,-4.53355051147316));
#33634=CARTESIAN_POINT('Origin',(173.058,8.10351388986772E-16,-1.22178682300763E-16));
#33635=CARTESIAN_POINT('',(173.058,-0.317020535431457,3.42736954239177));
#33636=CARTESIAN_POINT('Ctrl Pts',(173.058,2.6445394957829,-1.13133757670322));
#33637=CARTESIAN_POINT('Ctrl Pts',(173.058,2.68388676478393,-1.06040744504102));
#33638=CARTESIAN_POINT('Ctrl Pts',(173.058,2.71996664284584,-0.987874460436406));
#33639=CARTESIAN_POINT('Ctrl Pts',(173.058,2.75260599077044,-0.913896544786152));
#33640=CARTESIAN_POINT('Ctrl Pts',(173.058,2.79080948766531,-0.827307343391491));
#33641=CARTESIAN_POINT('Ctrl Pts',(173.058,2.82430130285621,-0.738739077560077));
#33642=CARTESIAN_POINT('Ctrl Pts',(173.058,2.85320325444538,-0.6485602460535));
#33643=CARTESIAN_POINT('Ctrl Pts',(173.058,2.87052216452721,-0.594522404721965));
#33644=CARTESIAN_POINT('Ctrl Pts',(173.058,2.8861921276262,-0.539905615643428));
#33645=CARTESIAN_POINT('Ctrl Pts',(173.058,2.90023180440349,-0.484784713552764));
#33646=CARTESIAN_POINT('Ctrl Pts',(173.058,2.90495816775042,-0.466228630287898));
#33647=CARTESIAN_POINT('Ctrl Pts',(173.058,2.90949972520718,-0.447615393832835));
#33648=CARTESIAN_POINT('Ctrl Pts',(173.058,2.91385704339701,-0.428947796047142));
#33649=CARTESIAN_POINT('Ctrl Pts',(173.058,2.91798497003428,-0.41126295624517));
#33650=CARTESIAN_POINT('Ctrl Pts',(173.058,2.92194557683693,-0.39353765489647));
#33651=CARTESIAN_POINT('Ctrl Pts',(173.058,2.92573901615535,-0.375778161205653));
#33652=CARTESIAN_POINT('Ctrl Pts',(173.058,2.94706671207049,-0.275929699361356));
#33653=CARTESIAN_POINT('Ctrl Pts',(173.058,2.96312338895318,-0.17496588958598));
#33654=CARTESIAN_POINT('Ctrl Pts',(173.058,2.97405583198172,-0.0733312989060914));
#33655=CARTESIAN_POINT('Ctrl Pts',(173.058,2.98362171963169,0.0155989679388112));
#33656=CARTESIAN_POINT('Ctrl Pts',(173.058,2.98926355991625,0.105043810517558));
#33657=CARTESIAN_POINT('Ctrl Pts',(173.058,2.99104538503735,0.194721159461318));
#33658=CARTESIAN_POINT('Ctrl Pts',(173.058,2.9919477288971,0.240135158972413));
#33659=CARTESIAN_POINT('Ctrl Pts',(173.058,2.99185963655175,0.285608966682687));
#33660=CARTESIAN_POINT('Ctrl Pts',(173.058,2.99078627853696,0.331106705631171));
#33661=CARTESIAN_POINT('Ctrl Pts',(173.058,2.99039011742852,0.347899271061504));
#33662=CARTESIAN_POINT('Ctrl Pts',(173.058,2.98985962973635,0.364695414585539));
#33663=CARTESIAN_POINT('Ctrl Pts',(173.058,2.98919583576813,0.381478052754939));
#33664=CARTESIAN_POINT('Ctrl Pts',(173.058,2.98517361899542,0.483171367196758));
#33665=CARTESIAN_POINT('Ctrl Pts',(173.058,2.97625835266948,0.584503472695341));
#33666=CARTESIAN_POINT('Ctrl Pts',(173.058,2.96258323513638,0.685067958781066));
#33667=CARTESIAN_POINT('Ctrl Pts',(173.058,2.94869737691069,0.787182196040461));
#33668=CARTESIAN_POINT('Ctrl Pts',(173.058,2.92990395107091,0.88850588487361));
#33669=CARTESIAN_POINT('Ctrl Pts',(173.058,2.90629107171056,0.988628707087666));
#33670=CARTESIAN_POINT('Ctrl Pts',(173.058,2.88278756415779,1.08828777332012));
#33671=CARTESIAN_POINT('Ctrl Pts',(173.058,2.85450910237203,1.18675804608544));
#33672=CARTESIAN_POINT('Ctrl Pts',(173.058,2.82149181038043,1.28363554367967));
#33673=CARTESIAN_POINT('Ctrl Pts',(173.058,2.80072893032535,1.34455682889888));
#33674=CARTESIAN_POINT('Ctrl Pts',(173.058,2.77809106867539,1.40484821518742));
#33675=CARTESIAN_POINT('Ctrl Pts',(173.058,2.75357694953202,1.46440672670599));
#33676=CARTESIAN_POINT('Ctrl Pts',(173.058,2.74765579823695,1.47879251619931));
#33677=CARTESIAN_POINT('Ctrl Pts',(173.058,2.74162514642604,1.49313553453836));
#33678=CARTESIAN_POINT('Ctrl Pts',(173.058,2.73548490672827,1.50743430130681));
#33679=CARTESIAN_POINT('Ctrl Pts',(173.058,2.7297149744626,1.52087073372598));
#33680=CARTESIAN_POINT('Ctrl Pts',(173.058,2.72385220696792,1.53425892684204));
#33681=CARTESIAN_POINT('Ctrl Pts',(173.058,2.71789703616041,1.54759752544682));
#33682=CARTESIAN_POINT('Ctrl Pts',(173.058,2.67487005930043,1.64397084404051));
#33683=CARTESIAN_POINT('Ctrl Pts',(173.058,2.6270219018787,1.737759129436));
#33684=CARTESIAN_POINT('Ctrl Pts',(173.058,2.57444790271155,1.82854142353784));
#33685=CARTESIAN_POINT('Ctrl Pts',(173.058,2.54586514607472,1.87789677523928));
#33686=CARTESIAN_POINT('Ctrl Pts',(173.058,2.51588464763651,1.92636367759785));
#33687=CARTESIAN_POINT('Ctrl Pts',(173.058,2.48451528981652,1.97387379690175));
#33688=CARTESIAN_POINT('Ctrl Pts',(173.058,2.4286458194415,2.05849029489302));
#33689=CARTESIAN_POINT('Ctrl Pts',(173.058,2.36837369723511,2.14007342029795));
#33690=CARTESIAN_POINT('Ctrl Pts',(173.058,2.30406148503067,2.21852057948255));
#33691=CARTESIAN_POINT('Ctrl Pts',(173.058,2.23853237955843,2.29845208847597));
#33692=CARTESIAN_POINT('Ctrl Pts',(173.058,2.16880835636398,2.37512837214474));
#33693=CARTESIAN_POINT('Ctrl Pts',(173.058,2.09522678862175,2.4484128735308));
#33694=CARTESIAN_POINT('Ctrl Pts',(173.058,2.0767086217718,2.46685627812007));
#33695=CARTESIAN_POINT('Ctrl Pts',(173.058,2.05794592621631,2.48508469783389));
#33696=CARTESIAN_POINT('Ctrl Pts',(173.058,2.03894369044655,2.5030956193348));
#33697=CARTESIAN_POINT('Ctrl Pts',(173.058,2.02757992226549,2.5138665590886));
#33698=CARTESIAN_POINT('Ctrl Pts',(173.058,2.01613687709355,2.52455362818136));
#33699=CARTESIAN_POINT('Ctrl Pts',(173.058,2.00461862649846,2.53515407788848));
#33700=CARTESIAN_POINT('Ctrl Pts',(173.058,1.92673714454547,2.60682978295701));
#33701=CARTESIAN_POINT('Ctrl Pts',(173.058,1.84538286439517,2.67458398376605));
#33702=CARTESIAN_POINT('Ctrl Pts',(173.058,1.76097463544042,2.73832174508392));
#33703=CARTESIAN_POINT('Ctrl Pts',(173.058,1.67547637152312,2.80288260610582));
#33704=CARTESIAN_POINT('Ctrl Pts',(173.058,1.58684416396937,2.86332314304966));
#33705=CARTESIAN_POINT('Ctrl Pts',(173.058,1.49546564431326,2.91951596239309));
#33706=CARTESIAN_POINT('Ctrl Pts',(173.058,1.40339423056955,2.97613487391262));
#33707=CARTESIAN_POINT('Ctrl Pts',(173.058,1.30853399756601,3.02844194726936));
#33708=CARTESIAN_POINT('Ctrl Pts',(173.058,1.21124337720924,3.07626987325074));
#33709=CARTESIAN_POINT('Ctrl Pts',(173.058,1.15206303145065,3.10536284424954));
#33710=CARTESIAN_POINT('Ctrl Pts',(173.058,1.09198272382463,3.1327977355338));
#33711=CARTESIAN_POINT('Ctrl Pts',(173.058,1.03107802904275,3.15852895038418));
#33712=CARTESIAN_POINT('Ctrl Pts',(173.058,1.0114596465522,3.1668173888484));
#33713=CARTESIAN_POINT('Ctrl Pts',(173.058,0.991755702241084,3.17492900566073));
#33714=CARTESIAN_POINT('Ctrl Pts',(173.058,0.971968657952046,3.18286212972466));
#33715=CARTESIAN_POINT('Ctrl Pts',(173.058,0.956867573602449,3.18891653451071));
#33716=CARTESIAN_POINT('Ctrl Pts',(173.058,0.94172575171078,3.1948638770094));
#33717=CARTESIAN_POINT('Ctrl Pts',(173.058,0.926549215256223,3.20070193666412));
#33718=CARTESIAN_POINT('Ctrl Pts',(173.058,0.822753641283176,3.24062967344152));
#33719=CARTESIAN_POINT('Ctrl Pts',(173.058,0.717267605953907,3.27547679138173));
#33720=CARTESIAN_POINT('Ctrl Pts',(173.058,0.610497881757582,3.3051135063329));
#33721=CARTESIAN_POINT('Ctrl Pts',(173.058,0.503660205739328,3.33476908308026));
#33722=CARTESIAN_POINT('Ctrl Pts',(173.058,0.395536406906948,3.35920812012469));
#33723=CARTESIAN_POINT('Ctrl Pts',(173.058,0.286502176775991,3.37825926969399));
#33724=CARTESIAN_POINT('Ctrl Pts',(173.058,0.17972562081492,3.3969159441683));
#33725=CARTESIAN_POINT('Ctrl Pts',(173.058,0.072075126876207,3.41040586117002));
#33726=CARTESIAN_POINT('Ctrl Pts',(173.058,-0.0361149137713203,3.41852273121879));
#33727=CARTESIAN_POINT('Ctrl Pts',(173.058,-0.129418258192251,3.42552273895746));
#33728=CARTESIAN_POINT('Ctrl Pts',(173.058,-0.223123452753258,3.42852607773628));
#33729=CARTESIAN_POINT('Ctrl Pts',(173.058,-0.317020535431506,3.42736954239176));
#33730=CARTESIAN_POINT('',(173.058,-3.44200000000001,-4.2152342826652E-16));
#33731=CARTESIAN_POINT('Origin',(173.058,0.,0.));
#33732=CARTESIAN_POINT('',(173.058,-2.9035416885497,1.85819928779561));
#33733=CARTESIAN_POINT('Origin',(173.058,0.,0.));
#33734=CARTESIAN_POINT('Ctrl Pts',(173.058,-2.90354168854955,1.85819928779586));
#33735=CARTESIAN_POINT('Ctrl Pts',(173.058,-2.94927698134181,1.77348528868279));
#33736=CARTESIAN_POINT('Ctrl Pts',(173.058,-2.99114946863433,1.68689959241407));
#33737=CARTESIAN_POINT('Ctrl Pts',(173.058,-3.02892190972098,1.59857426255952));
#33738=CARTESIAN_POINT('Ctrl Pts',(173.058,-3.07225686000619,1.4972418183738));
#33739=CARTESIAN_POINT('Ctrl Pts',(173.058,-3.11019621799762,1.39361911367756));
#33740=CARTESIAN_POINT('Ctrl Pts',(173.058,-3.1427908688464,1.28813764211491));
#33741=CARTESIAN_POINT('Ctrl Pts',(173.058,-3.16081628017585,1.22980454563925));
#33742=CARTESIAN_POINT('Ctrl Pts',(173.058,-3.17720619857394,1.17090282854363));
#33743=CARTESIAN_POINT('Ctrl Pts',(173.058,-3.19196248863544,1.1115053227446));
#33744=CARTESIAN_POINT('Ctrl Pts',(173.058,-3.19769929159171,1.08841335413712));
#33745=CARTESIAN_POINT('Ctrl Pts',(173.058,-3.2031891341079,1.06524645577256));
#33746=CARTESIAN_POINT('Ctrl Pts',(173.058,-3.20843193488223,1.04200893503998));
#33747=CARTESIAN_POINT('Ctrl Pts',(173.058,-3.21256128773105,1.0237065187234));
#33748=CARTESIAN_POINT('Ctrl Pts',(173.058,-3.21653710764215,1.00536119930646));
#33749=CARTESIAN_POINT('Ctrl Pts',(173.058,-3.22035696748742,0.986987648751191));
#33750=CARTESIAN_POINT('Ctrl Pts',(173.058,-3.24273618152464,0.879343484526355));
#33751=CARTESIAN_POINT('Ctrl Pts',(173.058,-3.25979279126121,0.7706167253394));
#33752=CARTESIAN_POINT('Ctrl Pts',(173.058,-3.27158446109908,0.661236741394953));
#33753=CARTESIAN_POINT('Ctrl Pts',(173.058,-3.2818639471905,0.565883832171975));
#33754=CARTESIAN_POINT('Ctrl Pts',(173.058,-3.2881413770772,0.470033964546229));
#33755=CARTESIAN_POINT('Ctrl Pts',(173.058,-3.29042275668324,0.373974651407001));
#33756=CARTESIAN_POINT('Ctrl Pts',(173.058,-3.29142086026088,0.331948701908589));
#33757=CARTESIAN_POINT('Ctrl Pts',(173.058,-3.29165371669549,0.289882748038347));
#33758=CARTESIAN_POINT('Ctrl Pts',(173.058,-3.29112009188747,0.247801422509378));
#33759=CARTESIAN_POINT('Ctrl Pts',(173.058,-3.29076373357566,0.219699224300322));
#33760=CARTESIAN_POINT('Ctrl Pts',(173.058,-3.29006552909826,0.191590178903719));
#33761=CARTESIAN_POINT('Ctrl Pts',(173.058,-3.2890248546268,0.163481743603303));
#33762=CARTESIAN_POINT('Ctrl Pts',(173.058,-3.28844078257146,0.147706059632424));
#33763=CARTESIAN_POINT('Ctrl Pts',(173.058,-3.28774893091277,0.131934287123879));
#33764=CARTESIAN_POINT('Ctrl Pts',(173.058,-3.28694984088798,0.116175937424863));
#33765=CARTESIAN_POINT('Ctrl Pts',(173.058,-3.28147503817363,0.00821081080604001));
#33766=CARTESIAN_POINT('Ctrl Pts',(173.058,-3.27096658134644,-0.0992403578637111));
#33767=CARTESIAN_POINT('Ctrl Pts',(173.058,-3.25547394530537,-0.205775224611218));
#33768=CARTESIAN_POINT('Ctrl Pts',(173.058,-3.24008355632353,-0.311606991072829));
#33769=CARTESIAN_POINT('Ctrl Pts',(173.058,-3.21977431584416,-0.416535404155237));
#33770=CARTESIAN_POINT('Ctrl Pts',(173.058,-3.19454570367412,-0.520151630293488));
#33771=CARTESIAN_POINT('Ctrl Pts',(173.058,-3.17007291782756,-0.620663608337271));
#33772=CARTESIAN_POINT('Ctrl Pts',(173.058,-3.14097073517173,-0.719941511152529));
#33773=CARTESIAN_POINT('Ctrl Pts',(173.058,-3.1071971623692,-0.817587324307012));
#33774=CARTESIAN_POINT('Ctrl Pts',(173.058,-3.08548206143738,-0.880369805172085));
#33775=CARTESIAN_POINT('Ctrl Pts',(173.058,-3.06183499229822,-0.942477053141852));
#33776=CARTESIAN_POINT('Ctrl Pts',(173.058,-3.03623629418228,-1.00379570569807));
#33777=CARTESIAN_POINT('Ctrl Pts',(173.058,-3.02812773113467,-1.02321880909165));
#33778=CARTESIAN_POINT('Ctrl Pts',(173.058,-3.01982330277573,-1.04256273766869));
#33779=CARTESIAN_POINT('Ctrl Pts',(173.058,-3.01132224969803,-1.06182373964142));
#33780=CARTESIAN_POINT('Ctrl Pts',(173.058,-3.00479372173366,-1.076615552944));
#33781=CARTESIAN_POINT('Ctrl Pts',(173.058,-2.99815215727783,-1.0913517307087));
#33782=CARTESIAN_POINT('Ctrl Pts',(173.058,-2.99140048475794,-1.10602445977451));
#33783=CARTESIAN_POINT('Ctrl Pts',(173.058,-2.94870774535495,-1.19880428529069));
#33784=CARTESIAN_POINT('Ctrl Pts',(173.058,-2.90158057124625,-1.28912974556565));
#33785=CARTESIAN_POINT('Ctrl Pts',(173.058,-2.8500188206114,-1.37663588218576));
#33786=CARTESIAN_POINT('Ctrl Pts',(173.058,-2.81978995482352,-1.42793769461331));
#33787=CARTESIAN_POINT('Ctrl Pts',(173.058,-2.78803607036402,-1.47827002836663));
#33788=CARTESIAN_POINT('Ctrl Pts',(173.058,-2.75475040343885,-1.52755433789291));
#33789=CARTESIAN_POINT('Ctrl Pts',(173.058,-2.69695413048116,-1.61313019287923));
#33790=CARTESIAN_POINT('Ctrl Pts',(173.058,-2.63454105743263,-1.69554864285166));
#33791=CARTESIAN_POINT('Ctrl Pts',(173.058,-2.56786860476729,-1.77461959696379));
#33792=CARTESIAN_POINT('Ctrl Pts',(173.058,-2.50091177594761,-1.85402781021296));
#33793=CARTESIAN_POINT('Ctrl Pts',(173.058,-2.42965826721123,-1.93006033993478));
#33794=CARTESIAN_POINT('Ctrl Pts',(173.058,-2.35444524775537,-2.00247889412283));
#33795=CARTESIAN_POINT('Ctrl Pts',(173.058,-2.34043558406068,-2.01596804263422));
#33796=CARTESIAN_POINT('Ctrl Pts',(173.058,-2.32628849698641,-2.02933166582729));
#33797=CARTESIAN_POINT('Ctrl Pts',(173.058,-2.31200610941859,-2.04256803058097));
#33798=CARTESIAN_POINT('Ctrl Pts',(173.058,-2.30065881337112,-2.05308426596102));
#33799=CARTESIAN_POINT('Ctrl Pts',(173.058,-2.28923218286527,-2.06351451415364));
#33800=CARTESIAN_POINT('Ctrl Pts',(173.058,-2.27773101546705,-2.07385511502059));
#33801=CARTESIAN_POINT('Ctrl Pts',(173.058,-2.20204585166299,-2.14190299601807));
#33802=CARTESIAN_POINT('Ctrl Pts',(173.058,-2.12308768631656,-2.20611658225596));
#33803=CARTESIAN_POINT('Ctrl Pts',(173.058,-2.04121912336534,-2.26634216288826));
#33804=CARTESIAN_POINT('Ctrl Pts',(173.058,-1.95923481267905,-2.32665289188886));
#33805=CARTESIAN_POINT('Ctrl Pts',(173.058,-1.87433096669665,-2.38296469657146));
#33806=CARTESIAN_POINT('Ctrl Pts',(173.058,-1.7868466424218,-2.43507739372807));
#33807=CARTESIAN_POINT('Ctrl Pts',(173.058,-1.70047530653565,-2.48652710551765));
#33808=CARTESIAN_POINT('Ctrl Pts',(173.058,-1.61158786513365,-2.53388410814607));
#33809=CARTESIAN_POINT('Ctrl Pts',(173.058,-1.52049938149984,-2.57690684306378));
#33810=CARTESIAN_POINT('Ctrl Pts',(173.058,-1.46934261688622,-2.60106910634249));
#33811=CARTESIAN_POINT('Ctrl Pts',(173.058,-1.41749148596287,-2.62386338352615));
#33812=CARTESIAN_POINT('Ctrl Pts',(173.058,-1.36500174485935,-2.64523955756217));
#33813=CARTESIAN_POINT('Ctrl Pts',(173.058,-1.35022593925688,-2.65125692753658));
#33814=CARTESIAN_POINT('Ctrl Pts',(173.058,-1.33539953217638,-2.65716189129253));
#33815=CARTESIAN_POINT('Ctrl Pts',(173.058,-1.32052377671622,-2.66295325147544));
#33816=CARTESIAN_POINT('Ctrl Pts',(173.058,-1.30634201517583,-2.66847442916141));
#33817=CARTESIAN_POINT('Ctrl Pts',(173.058,-1.29212315263705,-2.67388931397687));
#33818=CARTESIAN_POINT('Ctrl Pts',(173.058,-1.27787268843006,-2.67919566395992));
#33819=CARTESIAN_POINT('Ctrl Pts',(173.058,-1.18535651693264,-2.71364529155983));
#33820=CARTESIAN_POINT('Ctrl Pts',(173.058,-1.09145092288641,-2.74354721992335));
#33821=CARTESIAN_POINT('Ctrl Pts',(173.058,-0.996467560098021,-2.76872192402909));
#33822=CARTESIAN_POINT('Ctrl Pts',(173.058,-0.902843142461929,-2.79353644882447));
#33823=CARTESIAN_POINT('Ctrl Pts',(173.058,-0.808170782502429,-2.81375820684046));
#33824=CARTESIAN_POINT('Ctrl Pts',(173.058,-0.71274438433838,-2.82916570405975));
#33825=CARTESIAN_POINT('Ctrl Pts',(173.058,-0.620307640495166,-2.84409049322842));
#33826=CARTESIAN_POINT('Ctrl Pts',(173.058,-0.527162731451988,-2.85449793884808));
#33827=CARTESIAN_POINT('Ctrl Pts',(173.058,-0.433582809923952,-2.86013906025488));
#33828=CARTESIAN_POINT('Ctrl Pts',(173.058,-0.358936314546988,-2.86463884969835));
#33829=CARTESIAN_POINT('Ctrl Pts',(173.058,-0.284013023602468,-2.86610502511712));
#33830=CARTESIAN_POINT('Ctrl Pts',(173.058,-0.208958374082637,-2.86438831129802));
#33831=CARTESIAN_POINT('Ctrl Pts',(156.641910346562,-1.26059492705642,2.58055893749389));
#33832=CARTESIAN_POINT('Ctrl Pts',(156.694526018528,-2.1137122723725,2.16381379671687));
#33833=CARTESIAN_POINT('Ctrl Pts',(156.79975736246,-3.35978581135109,0.42459068590928));
#33834=CARTESIAN_POINT('Ctrl Pts',(156.957604378359,-2.19296763671057,-2.58504463930359));
#33835=CARTESIAN_POINT('Ctrl Pts',(157.115451394257,0.963301600147334,-3.24751306779502));
#33836=CARTESIAN_POINT('Ctrl Pts',(157.273298410156,3.24548551852033,-0.972003967714269));
#33837=CARTESIAN_POINT('Ctrl Pts',(157.431145426054,2.58940221207372,2.18521955033239));
#33838=CARTESIAN_POINT('Ctrl Pts',(157.588992441952,-0.412068725742385,
3.36277947991426));
#33839=CARTESIAN_POINT('Ctrl Pts',(157.746839457851,-3.04016140279596,1.49535934622665));
#33840=CARTESIAN_POINT('Ctrl Pts',(157.904686473749,-2.91518172767359,-1.72643828285233));
#33841=CARTESIAN_POINT('Ctrl Pts',(158.062533489648,-0.150157556215628,
-3.38468261701631));
#33842=CARTESIAN_POINT('Ctrl Pts',(158.220380505546,2.7508243349508,-1.97779608453694));
#33843=CARTESIAN_POINT('Ctrl Pts',(158.378227521445,3.1606675065917,1.2202074592191));
#33844=CARTESIAN_POINT('Ctrl Pts',(158.536074537343,0.708198630334437,3.31317840661986));
#33845=CARTESIAN_POINT('Ctrl Pts',(158.693921553242,-2.38561307487835,2.40573461840344));
#33846=CARTESIAN_POINT('Ctrl Pts',(158.85176856914,-3.31901103198709,-0.68034914075078));
#33847=CARTESIAN_POINT('Ctrl Pts',(159.009615585039,-1.24670620219767,-3.15030627040552));
#33848=CARTESIAN_POINT('Ctrl Pts',(159.167462600937,1.95461751556788,-2.76734131891007));
#33849=CARTESIAN_POINT('Ctrl Pts',(159.325309616835,3.38583646824711,0.121732956096346));
#33850=CARTESIAN_POINT('Ctrl Pts',(159.483156632734,1.75083606284643,2.90056550260836));
#33851=CARTESIAN_POINT('Ctrl Pts',(159.641003648632,-1.46972441564107,3.05264107133596));
#33852=CARTESIAN_POINT('Ctrl Pts',(159.798850664531,-3.35929998446003,0.440239652832843));
#33853=CARTESIAN_POINT('Ctrl Pts',(159.956697680429,-2.20668775975965,-2.57084352550351));
#33854=CARTESIAN_POINT('Ctrl Pts',(160.114544696328,0.944304649918255,-3.25376644164669));
#33855=CARTESIAN_POINT('Ctrl Pts',(160.272391712226,3.24013316437363,-0.99007292658079));
#33856=CARTESIAN_POINT('Ctrl Pts',(160.430238728125,2.6016915700248,2.17023231333377));
#33857=CARTESIAN_POINT('Ctrl Pts',(160.588085744023,-0.392846336843677,
3.36517147828997));
#33858=CARTESIAN_POINT('Ctrl Pts',(160.745932759922,-3.03162193287603,1.51260562534786));
#33859=CARTESIAN_POINT('Ctrl Pts',(160.90377977582,-2.92495554734722,-1.70977845567023));
#33860=CARTESIAN_POINT('Ctrl Pts',(161.061626791718,-0.169444440750171,
-3.38378425779796));
#33861=CARTESIAN_POINT('Ctrl Pts',(161.219473807617,2.73951583977761,-1.99342927772498));
#33862=CARTESIAN_POINT('Ctrl Pts',(161.377320823515,3.16756591388022,1.2021786484908));
#33863=CARTESIAN_POINT('Ctrl Pts',(161.535167839414,0.727062906055984,3.30909154487233));
#33864=CARTESIAN_POINT('Ctrl Pts',(161.693014855312,-2.37186950675857,2.41928550704491));
#33865=CARTESIAN_POINT('Ctrl Pts',(161.850861871211,-3.32283285798019,-0.661429602917294));
#33866=CARTESIAN_POINT('Ctrl Pts',(162.008708887109,-1.26463311846787,-3.14315293890823));
#33867=CARTESIAN_POINT('Ctrl Pts',(162.166555903007,1.93882052518752,-2.77843162464046));
#33868=CARTESIAN_POINT('Ctrl Pts',(162.324402918906,3.38647500189316,0.102442097028211));
#33869=CARTESIAN_POINT('Ctrl Pts',(162.482249934804,1.76733195403479,2.89054408130007));
#33870=CARTESIAN_POINT('Ctrl Pts',(162.640096950703,-1.4523099189108,3.0609644266349));
#33871=CARTESIAN_POINT('Ctrl Pts',(162.797943966601,-3.3567374578584,0.459370178289061));
#33872=CARTESIAN_POINT('Ctrl Pts',(162.9557909825,-2.2212978427249,-2.55823048523718));
#33873=CARTESIAN_POINT('Ctrl Pts',(163.113637998398,0.925752878818704,-3.25909326792743));
#33874=CARTESIAN_POINT('Ctrl Pts',(163.271485014297,3.23444021792712,-1.00851564110162));
#33875=CARTESIAN_POINT('Ctrl Pts',(163.429332030195,2.61401299155246,2.15537546652226));
#33876=CARTESIAN_POINT('Ctrl Pts',(163.587179046093,-0.37366884830378,3.36735488380693));
#33877=CARTESIAN_POINT('Ctrl Pts',(163.745026061992,-3.02295554325443,1.52985198800354));
#33878=CARTESIAN_POINT('Ctrl Pts',(163.90287307789,-2.93464855399438,-1.69308747152348));
#33879=CARTESIAN_POINT('Ctrl Pts',(164.060720093789,-0.188718840271762,
-3.38276403566928));
#33880=CARTESIAN_POINT('Ctrl Pts',(164.218567109687,2.72811497634857,-2.00900373257834));
#33881=CARTESIAN_POINT('Ctrl Pts',(164.376414125585,3.17436322788575,1.18411376950773));
#33882=CARTESIAN_POINT('Ctrl Pts',(164.534261141484,0.74590273835584,3.30489582689142));
#33883=CARTESIAN_POINT('Ctrl Pts',(164.692108157382,-2.35804854035057,2.43275859941788));
#33884=CARTESIAN_POINT('Ctrl Pts',(164.849955173281,-3.32654704816499,-0.642488955575008));
#33885=CARTESIAN_POINT('Ctrl Pts',(165.007802189179,-1.28251888829241,-3.13589741905954));
#33886=CARTESIAN_POINT('Ctrl Pts',(165.165649205078,1.92296055931244,-2.78943184340823));
#33887=CARTESIAN_POINT('Ctrl Pts',(165.323496220976,3.38700365205358,0.0831479564798997));
#33888=CARTESIAN_POINT('Ctrl Pts',(165.481343236875,1.78377047374568,2.88042882548487));
#33889=CARTESIAN_POINT('Ctrl Pts',(165.639190252773,-1.43484828107338,3.06918844843256));
#33890=CARTESIAN_POINT('Ctrl Pts',(165.797037268672,-3.35406599083499,0.478485789564522));
#33891=CARTESIAN_POINT('Ctrl Pts',(165.95488428457,-2.23583583159796,-2.54553441458444));
#33892=CARTESIAN_POINT('Ctrl Pts',(166.112731300469,0.90717106151226,-3.26431432108579));
#33893=CARTESIAN_POINT('Ctrl Pts',(166.270578316367,3.22864229756116,-1.02692562344606));
#33894=CARTESIAN_POINT('Ctrl Pts',(166.428425332265,2.62624957467685,2.14044866633159));
#33895=CARTESIAN_POINT('Ctrl Pts',(166.586272348164,-0.354479232189763,
3.36942900142401));
#33896=CARTESIAN_POINT('Ctrl Pts',(166.744119364062,-3.01419104315912,1.54704869898476));
#33897=CARTESIAN_POINT('Ctrl Pts',(166.901966379961,-2.94424631611884,-1.67634153790678));
#33898=CARTESIAN_POINT('Ctrl Pts',(167.059813395859,-0.207987114903346,
-3.38163402539736));
#33899=CARTESIAN_POINT('Ctrl Pts',(167.217660411758,2.71662557150557,-2.02451298487645));
#33900=CARTESIAN_POINT('Ctrl Pts',(167.375507427656,3.18105751740887,1.16601045991334));
#33901=CARTESIAN_POINT('Ctrl Pts',(167.533354443555,0.764718362261322,3.3005928479761));
#33902=CARTESIAN_POINT('Ctrl Pts',(167.691201459453,-2.34415104309101,2.44615273621018));
#33903=CARTESIAN_POINT('Ctrl Pts',(167.849048475351,-3.33015327471841,-0.623527456148029));
#33904=CARTESIAN_POINT('Ctrl Pts',(168.00689549125,-1.30036303375706,-3.12854012314479));
#33905=CARTESIAN_POINT('Ctrl Pts',(168.164742507148,1.90703818343888,-2.80034153070911));
#33906=CARTESIAN_POINT('Ctrl Pts',(168.322589523047,3.38742237645021,0.0638511173542441));
#33907=CARTESIAN_POINT('Ctrl Pts',(168.480436538945,1.80015110090155,2.87022008487266));
#33908=CARTESIAN_POINT('Ctrl Pts',(168.638283554844,-1.41734007501666,3.07731285922868));
#33909=CARTESIAN_POINT('Ctrl Pts',(168.796130570742,-3.3512856670145,0.497585871478016));
#33910=CARTESIAN_POINT('Ctrl Pts',(168.953977586641,-2.25030125612222,-2.53275572813956));
#33911=CARTESIAN_POINT('Ctrl Pts',(169.111824602539,0.888559801961863,-3.26942943049782));
#33912=CARTESIAN_POINT('Ctrl Pts',(169.269671618437,3.2227395907929,-1.04530227652681));
#33913=CARTESIAN_POINT('Ctrl Pts',(169.427518634336,2.63840092301917,2.12545239707543));
#33914=CARTESIAN_POINT('Ctrl Pts',(169.585365650234,-0.335278112564125,
3.37139376458444));
#33915=CARTESIAN_POINT('Ctrl Pts',(169.743212666133,-3.00532871463423,1.564195198398));
#33916=CARTESIAN_POINT('Ctrl Pts',(169.901059682031,-2.95374852702394,-1.65954119461478));
#33917=CARTESIAN_POINT('Ctrl Pts',(170.05890669793,-0.227248629623084,-3.38039427118688));
#33918=CARTESIAN_POINT('Ctrl Pts',(170.216753713828,2.7050479786207,-2.03995651601825));
#33919=CARTESIAN_POINT('Ctrl Pts',(170.374600729726,3.18764860462061,1.14786927643015));
#33920=CARTESIAN_POINT('Ctrl Pts',(170.532447745625,0.783509087420058,3.2961828100762));
#33921=CARTESIAN_POINT('Ctrl Pts',(170.690294761523,-2.33017730499065,2.45946735681956));
#33922=CARTESIAN_POINT('Ctrl Pts',(170.848141777422,-3.33365174602366,-0.604545465623319));
#33923=CARTESIAN_POINT('Ctrl Pts',(171.00598879332,-1.31816431809934,-3.12108180407131));
#33924=CARTESIAN_POINT('Ctrl Pts',(171.163835809219,1.89105258537231,-2.81115929350443));
#33925=CARTESIAN_POINT('Ctrl Pts',(171.321682825117,3.38773384709925,0.04455010635921));
#33926=CARTESIAN_POINT('Ctrl Pts',(171.479529841016,1.81646787669691,2.85992243368512));
#33927=CARTESIAN_POINT('Ctrl Pts',(171.637376856914,-1.39977490155201,3.08532882114793));
#33928=CARTESIAN_POINT('Ctrl Pts',(171.795223872812,-3.34841873999253,0.516687131179943));
#33929=CARTESIAN_POINT('Ctrl Pts',(171.953070888711,-2.26464885829485,-2.51992985577406));
#33930=CARTESIAN_POINT('Ctrl Pts',(172.110917904609,0.869829193827587,-3.27436767007504));
#33931=CARTESIAN_POINT('Ctrl Pts',(172.268764920508,3.21691519730582,-1.0637880016197));
#33932=CARTESIAN_POINT('Ctrl Pts',(172.426611936406,2.65009699317679,2.11067616912988));
#33933=CARTESIAN_POINT('Ctrl Pts',(172.584458952305,-0.315318796737369,
3.37266439996185));
#33934=CARTESIAN_POINT('Ctrl Pts',(172.742305968203,-2.9978837177994,1.58248414128088));
#33935=CARTESIAN_POINT('Ctrl Pts',(172.900152984102,-2.96002690825633,-1.64519866615417));
#33936=CARTESIAN_POINT('Ctrl Pts',(173.005384328034,-1.15590801223433,-2.79530792301902));
#33937=CARTESIAN_POINT('Ctrl Pts',(173.058,-0.208958374082637,-2.86438831129802));
#33938=CARTESIAN_POINT('Ctrl Pts',(156.751606897708,-1.34399083100512,2.75127836581));
#33939=CARTESIAN_POINT('Ctrl Pts',(156.804222569674,-2.25354699791245,2.30696303814315));
#33940=CARTESIAN_POINT('Ctrl Pts',(156.909453913606,-3.58205576405188,0.452679902595504));
#33941=CARTESIAN_POINT('Ctrl Pts',(157.067300929505,-2.33804557925064,-2.75606082365862));
#33942=CARTESIAN_POINT('Ctrl Pts',(157.225147945403,1.02702977007349,-3.46235550612409));
#33943=CARTESIAN_POINT('Ctrl Pts',(157.382994961302,3.46019382232215,-1.03630785137227));
#33944=CARTESIAN_POINT('Ctrl Pts',(157.5408419772,2.76070667596441,2.32978491055631));
#33945=CARTESIAN_POINT('Ctrl Pts',(157.698688993099,-0.439329539771279,
3.58524748171918));
#33946=CARTESIAN_POINT('Ctrl Pts',(157.856536008997,-3.24128628668565,1.59428632247425));
#33947=CARTESIAN_POINT('Ctrl Pts',(158.014383024895,-3.10803845756845,-1.84065251465661));
#33948=CARTESIAN_POINT('Ctrl Pts',(158.172230040794,-0.160091377831587,
-3.6085996425153));
#33949=CARTESIAN_POINT('Ctrl Pts',(158.330077056692,2.93280783900394,-2.10863914026887));
#33950=CARTESIAN_POINT('Ctrl Pts',(158.487924072591,3.36976459094144,1.30093149029555));
#33951=CARTESIAN_POINT('Ctrl Pts',(158.645771088489,0.755050211032075,3.53236500037256));
#33952=CARTESIAN_POINT('Ctrl Pts',(158.803618104388,-2.54343566687934,2.56488837101372));
#33953=CARTESIAN_POINT('Ctrl Pts',(158.961465120286,-3.5385834888386,-0.725358310925775));
#33954=CARTESIAN_POINT('Ctrl Pts',(159.119312136185,-1.3291832838194,-3.35871789692955));
#33955=CARTESIAN_POINT('Ctrl Pts',(159.277159152083,2.0839271701493,-2.95041752037001));
#33956=CARTESIAN_POINT('Ctrl Pts',(159.435006167982,3.60982982791527,0.129786320183477));
#33957=CARTESIAN_POINT('Ctrl Pts',(159.59285318388,1.86666435391219,3.09245528168063));
#33958=CARTESIAN_POINT('Ctrl Pts',(159.750700199778,-1.56695548770644,3.25459156003856));
#33959=CARTESIAN_POINT('Ctrl Pts',(159.908547215677,-3.58153779680244,0.4693641424005));
#33960=CARTESIAN_POINT('Ctrl Pts',(160.066394231575,-2.35267337060728,-2.74092022113221));
#33961=CARTESIAN_POINT('Ctrl Pts',(160.224241247474,1.00677605781672,-3.46902257810661));
#33962=CARTESIAN_POINT('Ctrl Pts',(160.382088263372,3.45448737789416,-1.05557218008024));
#33963=CARTESIAN_POINT('Ctrl Pts',(160.539935279271,2.77380904854317,2.3138061780738));
#33964=CARTESIAN_POINT('Ctrl Pts',(160.697782295169,-0.418835474726765,
3.58779772511277));
#33965=CARTESIAN_POINT('Ctrl Pts',(160.855629311068,-3.23218187968885,1.61267354624485));
#33966=CARTESIAN_POINT('Ctrl Pts',(161.013476326966,-3.1184588739475,-1.82289054013307));
#33967=CARTESIAN_POINT('Ctrl Pts',(161.171323342865,-0.180654205284504,
-3.60764185145451));
#33968=CARTESIAN_POINT('Ctrl Pts',(161.329170358763,2.92075121915007,-2.12530656281126));
#33969=CARTESIAN_POINT('Ctrl Pts',(161.487017374661,3.37711936918567,1.28170996576558));
#33970=CARTESIAN_POINT('Ctrl Pts',(161.64486439056,0.77516247156807,3.5280077682448));
#33971=CARTESIAN_POINT('Ctrl Pts',(161.802711406458,-2.52878287942016,2.57933573209316));
#33972=CARTESIAN_POINT('Ctrl Pts',(161.960558422357,-3.54265815150952,-0.705187132358178));
#33973=CARTESIAN_POINT('Ctrl Pts',(162.118405438255,-1.34829617296264,-3.35109132971343));
#33974=CARTESIAN_POINT('Ctrl Pts',(162.276252454154,2.06708511424935,-2.96224151624273));
#33975=CARTESIAN_POINT('Ctrl Pts',(162.434099470052,3.61051060438609,0.109219255257768));
#33976=CARTESIAN_POINT('Ctrl Pts',(162.59194648595,1.88425154709422,3.08177088333593));
#33977=CARTESIAN_POINT('Ctrl Pts',(162.749793501849,-1.54838891772451,3.26346555513791));
#33978=CARTESIAN_POINT('Ctrl Pts',(162.907640517747,-3.57880574371951,0.489760266685644));
#33979=CARTESIAN_POINT('Ctrl Pts',(163.065487533646,-2.36824999805838,-2.72747275271455));
#33980=CARTESIAN_POINT('Ctrl Pts',(163.223334549544,0.986996975955014,-3.47470180584743));
#33981=CARTESIAN_POINT('Ctrl Pts',(163.381181565443,3.44841780894597,-1.07523499061742));
#33982=CARTESIAN_POINT('Ctrl Pts',(163.539028581341,2.78694560589613,2.29796646187016));
#33983=CARTESIAN_POINT('Ctrl Pts',(163.69687559724,-0.398389280468699,3.59012557598079));
#33984=CARTESIAN_POINT('Ctrl Pts',(163.854722613138,-3.222942156492,1.63106085907622));
#33985=CARTESIAN_POINT('Ctrl Pts',(164.012569629037,-3.12879313103441,-1.80509534742508));
#33986=CARTESIAN_POINT('Ctrl Pts',(164.170416644935,-0.201203721766088,
-3.60655413552205));
#33987=CARTESIAN_POINT('Ctrl Pts',(164.328263660833,2.90859612032705,-2.14191136112637));
#33988=CARTESIAN_POINT('Ctrl Pts',(164.486110676732,3.38436636622082,1.26244998684979));
#33989=CARTESIAN_POINT('Ctrl Pts',(164.64395769263,0.795248671603639,3.52353447839189));
#33990=CARTESIAN_POINT('Ctrl Pts',(164.801804708528,-2.51404757331246,2.59370015021503));
#33991=CARTESIAN_POINT('Ctrl Pts',(164.959651724427,-3.54661805761881,-0.68499344776135));
#33992=CARTESIAN_POINT('Ctrl Pts',(165.117498740325,-1.3673651935764,-3.34335581377447));
#33993=CARTESIAN_POINT('Ctrl Pts',(165.275345756224,2.05017591664855,-2.97396946536074));
#33994=CARTESIAN_POINT('Ctrl Pts',(165.433192772122,3.61107422792063,0.0886486917623198));
#33995=CARTESIAN_POINT('Ctrl Pts',(165.591039788021,1.90177757333195,3.07098644276972));
#33996=CARTESIAN_POINT('Ctrl Pts',(165.748886803919,-1.52977208796888,3.27223364522999));
#33997=CARTESIAN_POINT('Ctrl Pts',(165.906733819818,-3.57595754315345,0.510140490127658));
#33998=CARTESIAN_POINT('Ctrl Pts',(166.064580835716,-2.38374976196135,-2.71393676095317));
#33999=CARTESIAN_POINT('Ctrl Pts',(166.222427851615,0.967185860149888,-3.48026826294036));
#34000=CARTESIAN_POINT('Ctrl Pts',(166.380274867513,3.44223632142488,-1.09486290354871));
#34001=CARTESIAN_POINT('Ctrl Pts',(166.538121883411,2.79999171227736,2.2820521644524));
#34002=CARTESIAN_POINT('Ctrl Pts',(166.69596889931,-0.377930156324856,3.59233690889983));
#34003=CARTESIAN_POINT('Ctrl Pts',(166.853815915208,-3.21359783222604,1.64939523547751));
#34004=CARTESIAN_POINT('Ctrl Pts',(167.011662931107,-3.13902584260304,-1.78724157001062));
#34005=CARTESIAN_POINT('Ctrl Pts',(167.169509947005,-0.22174670815951,-3.60534936830317));
#34006=CARTESIAN_POINT('Ctrl Pts',(167.327356962904,2.89634662254527,-2.15844664334671));
#34007=CARTESIAN_POINT('Ctrl Pts',(167.485203978802,3.39150352308704,1.24314903490759));
#34008=CARTESIAN_POINT('Ctrl Pts',(167.643050994701,0.815309061714566,3.51894683165139));
#34009=CARTESIAN_POINT('Ctrl Pts',(167.800898010599,-2.49923067337904,2.60798038937174));
#34010=CARTESIAN_POINT('Ctrl Pts',(167.958745026497,-3.55046285765591,-0.664777531589554));
#34011=CARTESIAN_POINT('Ctrl Pts',(168.116592042396,-1.38638983612959,-3.33551178867316));
#34012=CARTESIAN_POINT('Ctrl Pts',(168.274439058294,2.03320018025411,-2.98560089381315));
#34013=CARTESIAN_POINT('Ctrl Pts',(168.432286074193,3.61152065344378,0.0680752511624752));
#34014=CARTESIAN_POINT('Ctrl Pts',(168.590133090091,1.91924187707542,3.06010233282732));
#34015=CARTESIAN_POINT('Ctrl Pts',(168.74798010599,-1.51110560922735,3.28089553445622));
#34016=CARTESIAN_POINT('Ctrl Pts',(168.905827121888,-3.57299328426128,0.530504156847406));
#34017=CARTESIAN_POINT('Ctrl Pts',(169.063674137786,-2.39917216094927,-2.70031268787022));
#34018=CARTESIAN_POINT('Ctrl Pts',(169.221521153685,0.947343354320042,-3.48572176747365));
#34019=CARTESIAN_POINT('Ctrl Pts',(169.379368169583,3.43594311525342,-1.11445528228592));
#34020=CARTESIAN_POINT('Ctrl Pts',(169.537215185482,2.81294694508522,2.26606380217442));
#34021=CARTESIAN_POINT('Ctrl Pts',(169.69506220138,-0.357458767643203,3.59443165291001));
#34022=CARTESIAN_POINT('Ctrl Pts',(169.852909217279,-3.204149207594,1.66767607851488));
#34023=CARTESIAN_POINT('Ctrl Pts',(170.010756233177,-3.1491566816669,-1.76932978339498));
#34024=CARTESIAN_POINT('Ctrl Pts',(170.168603249076,-0.242282487432436,
-3.60402759692696));
#34025=CARTESIAN_POINT('Ctrl Pts',(170.326450264974,2.8840031025545,-2.17491185656266));
#34026=CARTESIAN_POINT('Ctrl Pts',(170.484297280873,3.39853065019093,1.22380770349201));
#34027=CARTESIAN_POINT('Ctrl Pts',(170.642144296771,0.835342905877536,3.51424504333333));
#34028=CARTESIAN_POINT('Ctrl Pts',(170.79999131267,-2.48433248881662,2.62217585187379));
#34029=CARTESIAN_POINT('Ctrl Pts',(170.957838328568,-3.55419277378985,-0.644539768711187));
#34030=CARTESIAN_POINT('Ctrl Pts',(171.115685344466,-1.40536878204047,-3.32756005712616));
#34031=CARTESIAN_POINT('Ctrl Pts',(171.273532360365,2.01615703913996,-2.99713431640342));
#34032=CARTESIAN_POINT('Ctrl Pts',(171.431379376263,3.61185272974161,0.0474973626991037));
#34033=CARTESIAN_POINT('Ctrl Pts',(171.589226392162,1.93663810530849,3.04912343034255));
#34034=CARTESIAN_POINT('Ctrl Pts',(171.74707340806,-1.49237839434269,3.28944180026288));
#34035=CARTESIAN_POINT('Ctrl Pts',(171.904920423959,-3.56993669284718,0.550869079273346));
#34036=CARTESIAN_POINT('Ctrl Pts',(172.062767439857,-2.41446894293137,-2.68663830723542));
#34037=CARTESIAN_POINT('Ctrl Pts',(172.220614455756,0.927373604282732,-3.49098670117333));
#34038=CARTESIAN_POINT('Ctrl Pts',(172.378461471654,3.42973340325571,-1.13416394880208));
#34039=CARTESIAN_POINT('Ctrl Pts',(172.536308487552,2.82541678032987,2.25031003825753));
#34040=CARTESIAN_POINT('Ctrl Pts',(172.694155503451,-0.336179023541002,
3.59578634842729));
#34041=CARTESIAN_POINT('Ctrl Pts',(172.852002519349,-3.19621167963151,1.68717494449934));
#34042=CARTESIAN_POINT('Ctrl Pts',(173.009849535248,-3.15585041541815,-1.75403841078134));
#34043=CARTESIAN_POINT('Ctrl Pts',(173.11508087918,-1.23237824981253,-2.98023428282876));
#34044=CARTESIAN_POINT('Ctrl Pts',(173.167696551146,-0.222782221950241,
-3.05388475250506));
#34045=CARTESIAN_POINT('Ctrl Pts',(156.861303448854,-1.42738673495382,2.92199779412611));
#34046=CARTESIAN_POINT('Ctrl Pts',(156.91391912082,-2.3933817234524,2.45011227956942));
#34047=CARTESIAN_POINT('Ctrl Pts',(157.019150464752,-3.80432571675269,0.480769119281727));
#34048=CARTESIAN_POINT('Ctrl Pts',(157.176997480651,-2.4831235217907,-2.92707700801364));
#34049=CARTESIAN_POINT('Ctrl Pts',(157.334844496549,1.09075793999965,-3.67719794445316));
#34050=CARTESIAN_POINT('Ctrl Pts',(157.492691512448,3.67490212612398,-1.10061173503027));
#34051=CARTESIAN_POINT('Ctrl Pts',(157.650538528346,2.93201113985509,2.47435027078023));
#34052=CARTESIAN_POINT('Ctrl Pts',(157.808385544245,-0.466590353800172,
3.8077154835241));
#34053=CARTESIAN_POINT('Ctrl Pts',(157.966232560143,-3.44241117057535,1.69321329872186));
#34054=CARTESIAN_POINT('Ctrl Pts',(158.124079576041,-3.3008951874633,-1.95486674646089));
#34055=CARTESIAN_POINT('Ctrl Pts',(158.28192659194,-0.17002519944755,-3.83251666801428));
#34056=CARTESIAN_POINT('Ctrl Pts',(158.439773607838,3.11479134305708,-2.23948219600079));
#34057=CARTESIAN_POINT('Ctrl Pts',(158.597620623737,3.57886167529118,1.381655521372));
#34058=CARTESIAN_POINT('Ctrl Pts',(158.755467639635,0.801901791729711,3.75155159412526));
#34059=CARTESIAN_POINT('Ctrl Pts',(158.913314655534,-2.70125825888032,2.72404212362399));
#34060=CARTESIAN_POINT('Ctrl Pts',(159.071161671432,-3.75815594569012,-0.770367481100765));
#34061=CARTESIAN_POINT('Ctrl Pts',(159.229008687331,-1.41166036544114,-3.56712952345359));
#34062=CARTESIAN_POINT('Ctrl Pts',(159.386855703229,2.21323682473072,-3.13349372182995));
#34063=CARTESIAN_POINT('Ctrl Pts',(159.544702719128,3.83382318758342,0.137839684270605));
#34064=CARTESIAN_POINT('Ctrl Pts',(159.702549735026,1.98249264497796,3.2843450607529));
#34065=CARTESIAN_POINT('Ctrl Pts',(159.860396750924,-1.66418655977181,3.45654204874115));
#34066=CARTESIAN_POINT('Ctrl Pts',(160.018243766823,-3.80377560914485,0.498488631968156));
#34067=CARTESIAN_POINT('Ctrl Pts',(160.176090782721,-2.49865898145491,-2.9109969167609));
#34068=CARTESIAN_POINT('Ctrl Pts',(160.33393779862,1.06924746571519,-3.68427871456653));
#34069=CARTESIAN_POINT('Ctrl Pts',(160.491784814518,3.66884159141469,-1.12107143357969));
#34070=CARTESIAN_POINT('Ctrl Pts',(160.649631830417,2.94592652706154,2.45738004281382));
#34071=CARTESIAN_POINT('Ctrl Pts',(160.807478846315,-0.444824612609852,
3.81042397193558));
#34072=CARTESIAN_POINT('Ctrl Pts',(160.965325862214,-3.43274182650167,1.71274146714184));
#34073=CARTESIAN_POINT('Ctrl Pts',(161.123172878112,-3.31196220054779,-1.93600262459591));
#34074=CARTESIAN_POINT('Ctrl Pts',(161.28101989401,-0.191863969818835,-3.83149944511106));
#34075=CARTESIAN_POINT('Ctrl Pts',(161.438866909909,3.10198659852252,-2.25718384789754));
#34076=CARTESIAN_POINT('Ctrl Pts',(161.596713925807,3.58667282449113,1.36124128304037));
#34077=CARTESIAN_POINT('Ctrl Pts',(161.754560941706,0.823262037080152,3.74692399161727));
#34078=CARTESIAN_POINT('Ctrl Pts',(161.912407957604,-2.68569625208175,2.73938595714142));
#34079=CARTESIAN_POINT('Ctrl Pts',(162.070254973503,-3.76248344503886,-0.748944661799061));
#34080=CARTESIAN_POINT('Ctrl Pts',(162.228101989401,-1.4319592274574,-3.55902972051863));
#34081=CARTESIAN_POINT('Ctrl Pts',(162.385949005299,2.19534970331118,-3.146051407845));
#34082=CARTESIAN_POINT('Ctrl Pts',(162.543796021198,3.83454620687902,0.115996413487326));
#34083=CARTESIAN_POINT('Ctrl Pts',(162.701643037096,2.00117114015365,3.27299768537179));
#34084=CARTESIAN_POINT('Ctrl Pts',(162.859490052995,-1.64446791653823,3.46596668364093));
#34085=CARTESIAN_POINT('Ctrl Pts',(163.017337068893,-3.80087402958061,0.52015035508223));
#34086=CARTESIAN_POINT('Ctrl Pts',(163.175184084792,-2.51520215339187,-2.89671502019193));
#34087=CARTESIAN_POINT('Ctrl Pts',(163.33303110069,1.04824107309133,-3.69031034376743));
#34088=CARTESIAN_POINT('Ctrl Pts',(163.490878116589,3.66239539996482,-1.14195434013322));
#34089=CARTESIAN_POINT('Ctrl Pts',(163.648725132487,2.95987822023979,2.44055745721806));
#34090=CARTESIAN_POINT('Ctrl Pts',(163.806572148386,-0.423109712633618,
3.81289626815465));
#34091=CARTESIAN_POINT('Ctrl Pts',(163.964419164284,-3.42292876972957,1.7322697301489));
#34092=CARTESIAN_POINT('Ctrl Pts',(164.122266180182,-3.32293770807444,-1.91710322332668));
#34093=CARTESIAN_POINT('Ctrl Pts',(164.280113196081,-0.213688603260413,
-3.83034423537483));
#34094=CARTESIAN_POINT('Ctrl Pts',(164.437960211979,3.08907726430553,-2.2748189896744));
#34095=CARTESIAN_POINT('Ctrl Pts',(164.595807227878,3.59436950455589,1.34078620419185));
#34096=CARTESIAN_POINT('Ctrl Pts',(164.753654243776,0.844594604851437,3.74217312989237));
#34097=CARTESIAN_POINT('Ctrl Pts',(164.911501259674,-2.67004660627436,2.75464170101219));
#34098=CARTESIAN_POINT('Ctrl Pts',(165.069348275573,-3.76668906707262,-0.727497939947697));
#34099=CARTESIAN_POINT('Ctrl Pts',(165.227195291472,-1.45221149886039,-3.5508142084894));
#34100=CARTESIAN_POINT('Ctrl Pts',(165.38504230737,2.17739127398466,-3.15850708731325));
#34101=CARTESIAN_POINT('Ctrl Pts',(165.542889323269,3.83514480378769,0.0941494270447407));
#34102=CARTESIAN_POINT('Ctrl Pts',(165.700736339167,2.0197846729182,3.26154406005457));
#34103=CARTESIAN_POINT('Ctrl Pts',(165.858583355065,-1.62469589486439,3.47527884202741));
#34104=CARTESIAN_POINT('Ctrl Pts',(166.016430370963,-3.79784909547192,0.541795190690796));
#34105=CARTESIAN_POINT('Ctrl Pts',(166.174277386862,-2.53166369232474,-2.8823391073219));
#34106=CARTESIAN_POINT('Ctrl Pts',(166.33212440276,1.02720065878751,-3.69622220479493));
#34107=CARTESIAN_POINT('Ctrl Pts',(166.489971418659,3.6558303452886,-1.16280018365137));
#34108=CARTESIAN_POINT('Ctrl Pts',(166.647818434557,2.97373384987786,2.4236556625732));
#34109=CARTESIAN_POINT('Ctrl Pts',(166.805665450456,-0.401381080459946,
3.81524481637566));
#34110=CARTESIAN_POINT('Ctrl Pts',(166.963512466354,-3.41300462129297,1.75174177197025));
#34111=CARTESIAN_POINT('Ctrl Pts',(167.121359482253,-3.33380536908723,-1.89814160211446));
#34112=CARTESIAN_POINT('Ctrl Pts',(167.279206498151,-0.235506301415678,
-3.82906471120899));
#34113=CARTESIAN_POINT('Ctrl Pts',(167.43705351405,3.07606767358497,-2.29238030181696));
#34114=CARTESIAN_POINT('Ctrl Pts',(167.594900529948,3.60194952876521,1.32028760990183));
#34115=CARTESIAN_POINT('Ctrl Pts',(167.752747545847,0.865899761167811,3.73730081532669));
#34116=CARTESIAN_POINT('Ctrl Pts',(167.910594561745,-2.65431030366708,2.76980804253329));
#34117=CARTESIAN_POINT('Ctrl Pts',(168.068441577643,-3.77077244059341,-0.706027607031077));
#34118=CARTESIAN_POINT('Ctrl Pts',(168.226288593542,-1.47241663850212,-3.54248345420153));
#34119=CARTESIAN_POINT('Ctrl Pts',(168.38413560944,2.15936217706934,-3.17086025691717));
#34120=CARTESIAN_POINT('Ctrl Pts',(168.541982625339,3.83561893043735,0.0722993849707047));
#34121=CARTESIAN_POINT('Ctrl Pts',(168.699829641237,2.03833265324929,3.24998458078198));
#34122=CARTESIAN_POINT('Ctrl Pts',(168.857676657136,-1.60487114343804,3.48447820968375));
#34123=CARTESIAN_POINT('Ctrl Pts',(169.015523673034,-3.79470090150806,0.5634224422168));
#34124=CARTESIAN_POINT('Ctrl Pts',(169.173370688933,-2.54804306577631,-2.86786964760089));
#34125=CARTESIAN_POINT('Ctrl Pts',(169.331217704831,1.00612690667822,-3.70201410444949));
#34126=CARTESIAN_POINT('Ctrl Pts',(169.489064720729,3.64914663971395,-1.18360828804503));
#34127=CARTESIAN_POINT('Ctrl Pts',(169.646911736628,2.98749296715126,2.4066752072734));
#34128=CARTESIAN_POINT('Ctrl Pts',(169.804758752526,-0.379639422722282,
3.81746954123559));
#34129=CARTESIAN_POINT('Ctrl Pts',(169.962605768425,-3.40296970055378,1.77115695863176));
#34130=CARTESIAN_POINT('Ctrl Pts',(170.120452784323,-3.34456483630987,-1.87911837217519));
#34131=CARTESIAN_POINT('Ctrl Pts',(170.278299800222,-0.257316345241784,
-3.82766092266703));
#34132=CARTESIAN_POINT('Ctrl Pts',(170.43614681612,3.06295822648831,-2.30986719710706));
#34133=CARTESIAN_POINT('Ctrl Pts',(170.593993832019,3.60941269576124,1.29974613055387));
#34134=CARTESIAN_POINT('Ctrl Pts',(170.751840847917,0.887176724335015,3.73230727659045));
#34135=CARTESIAN_POINT('Ctrl Pts',(170.909687863816,-2.63848767264258,2.78488434692803));
#34136=CARTESIAN_POINT('Ctrl Pts',(171.067534879714,-3.77473380155604,-0.684534071799058));
#34137=CARTESIAN_POINT('Ctrl Pts',(171.225381895612,-1.49257324598161,-3.534038310181));
#34138=CARTESIAN_POINT('Ctrl Pts',(171.383228911511,2.1412614929076,-3.1831093393024));
#34139=CARTESIAN_POINT('Ctrl Pts',(171.541075927409,3.83597161238398,0.0504446190389995));
#34140=CARTESIAN_POINT('Ctrl Pts',(171.698922943308,2.05680833392007,3.23832442699998));
#34141=CARTESIAN_POINT('Ctrl Pts',(171.856769959206,-1.58498188713336,3.49355477937783));
#34142=CARTESIAN_POINT('Ctrl Pts',(172.014616975104,-3.79145464570184,0.585051027366752));
#34143=CARTESIAN_POINT('Ctrl Pts',(172.172463991003,-2.56428902756788,-2.85334675869678));
#34144=CARTESIAN_POINT('Ctrl Pts',(172.330311006901,0.984918014737876,-3.70760573227161));
#34145=CARTESIAN_POINT('Ctrl Pts',(172.4881580228,3.6425516092056,-1.20453989598447));
#34146=CARTESIAN_POINT('Ctrl Pts',(172.646005038698,3.00073656748295,2.38994390738518));
#34147=CARTESIAN_POINT('Ctrl Pts',(172.803852054597,-0.357039250344633,
3.81890829689274));
#34148=CARTESIAN_POINT('Ctrl Pts',(172.961699070495,-3.39453964146364,1.7918657477178));
#34149=CARTESIAN_POINT('Ctrl Pts',(173.119546086394,-3.35167392257996,-1.86287815540851));
#34150=CARTESIAN_POINT('Ctrl Pts',(173.224777430326,-1.30884848739072,-3.16516064263851));
#34151=CARTESIAN_POINT('Ctrl Pts',(173.277393102292,-0.236606069817846,
-3.2433811937121));
#34152=CARTESIAN_POINT('Ctrl Pts',(156.971,-1.51078263890252,3.09271722244222));
#34153=CARTESIAN_POINT('Ctrl Pts',(157.023615671966,-2.53321644899234,2.59326152099569));
#34154=CARTESIAN_POINT('Ctrl Pts',(157.128847015899,-4.02659566945348,0.50885833596795));
#34155=CARTESIAN_POINT('Ctrl Pts',(157.286694031797,-2.62820146433077,-3.09809319236867));
#34156=CARTESIAN_POINT('Ctrl Pts',(157.444541047695,1.15448610992581,-3.89204038278222));
#34157=CARTESIAN_POINT('Ctrl Pts',(157.602388063594,3.88961042992581,-1.16491561868827));
#34158=CARTESIAN_POINT('Ctrl Pts',(157.760235079492,3.10331560374578,2.61891563100415));
#34159=CARTESIAN_POINT('Ctrl Pts',(157.918082095391,-0.493851167829066,
4.03018348532901));
#34160=CARTESIAN_POINT('Ctrl Pts',(158.075929111289,-3.64353605446504,1.79214027496947));
#34161=CARTESIAN_POINT('Ctrl Pts',(158.233776127187,-3.49375191735815,-2.06908097826516));
#34162=CARTESIAN_POINT('Ctrl Pts',(158.391623143086,-0.179959021063511,
-4.05643369351328));
#34163=CARTESIAN_POINT('Ctrl Pts',(158.549470158984,3.29677484711022,-2.37032525173271));
#34164=CARTESIAN_POINT('Ctrl Pts',(158.707317174883,3.78795875964091,1.46237955244845));
#34165=CARTESIAN_POINT('Ctrl Pts',(158.865164190781,0.848753372427349,3.97073818787796));
#34166=CARTESIAN_POINT('Ctrl Pts',(159.02301120668,-2.85908085088131,2.88319587623426));
#34167=CARTESIAN_POINT('Ctrl Pts',(159.180858222578,-3.97772840254164,-0.815376651275756));
#34168=CARTESIAN_POINT('Ctrl Pts',(159.338705238477,-1.49413744706287,-3.77554114997762));
#34169=CARTESIAN_POINT('Ctrl Pts',(159.496552254375,2.34254647931214,-3.31656992328989));
#34170=CARTESIAN_POINT('Ctrl Pts',(159.654399270274,4.05781654725159,0.145893048357734));
#34171=CARTESIAN_POINT('Ctrl Pts',(159.812246286172,2.09832093604372,3.47623483982516));
#34172=CARTESIAN_POINT('Ctrl Pts',(159.970093302071,-1.76141763183718,3.65849253744375));
#34173=CARTESIAN_POINT('Ctrl Pts',(160.127940317969,-4.02601342148726,0.527613121535813));
#34174=CARTESIAN_POINT('Ctrl Pts',(160.285787333867,-2.64464459230254,-3.0810736123896));
#34175=CARTESIAN_POINT('Ctrl Pts',(160.443634349766,1.13171887361366,-3.89953485102645));
#34176=CARTESIAN_POINT('Ctrl Pts',(160.601481365664,3.88319580493523,-1.18657068707914));
#34177=CARTESIAN_POINT('Ctrl Pts',(160.759328381563,3.1180440055799,2.60095390755385));
#34178=CARTESIAN_POINT('Ctrl Pts',(160.917175397461,-0.470813750492941,
4.03305021875839));
#34179=CARTESIAN_POINT('Ctrl Pts',(161.07502241336,-3.63330177331448,1.81280938803883));
#34180=CARTESIAN_POINT('Ctrl Pts',(161.232869429258,-3.50546552714807,-2.04911470905875));
#34181=CARTESIAN_POINT('Ctrl Pts',(161.390716445157,-0.203073734353165,
-4.05535703876761));
#34182=CARTESIAN_POINT('Ctrl Pts',(161.548563461055,3.28322197789498,-2.38906113298382));
#34183=CARTESIAN_POINT('Ctrl Pts',(161.706410476954,3.79622627979659,1.44077260031516));
#34184=CARTESIAN_POINT('Ctrl Pts',(161.864257492852,0.871361602592233,3.96584021498973));
#34185=CARTESIAN_POINT('Ctrl Pts',(162.02210450875,-2.84260962474333,2.89943618218967));
#34186=CARTESIAN_POINT('Ctrl Pts',(162.179951524649,-3.9823087385682,-0.792702191239944));
#34187=CARTESIAN_POINT('Ctrl Pts',(162.337798540547,-1.51562228195216,-3.76696811132383));
#34188=CARTESIAN_POINT('Ctrl Pts',(162.495645556446,2.32361429237301,-3.32986129944727));
#34189=CARTESIAN_POINT('Ctrl Pts',(162.653492572344,4.05858180937195,0.122773571716884));
#34190=CARTESIAN_POINT('Ctrl Pts',(162.811339588243,2.11809073321307,3.46422448740764));
#34191=CARTESIAN_POINT('Ctrl Pts',(162.969186604141,-1.74054691535194,3.66846781214395));
#34192=CARTESIAN_POINT('Ctrl Pts',(163.127033620039,-4.02294231544172,0.550540443478812));
#34193=CARTESIAN_POINT('Ctrl Pts',(163.284880635938,-2.66215430872536,-3.0659572876693));
#34194=CARTESIAN_POINT('Ctrl Pts',(163.442727651836,1.10948517022764,-3.90591888168743));
#34195=CARTESIAN_POINT('Ctrl Pts',(163.600574667735,3.87637299098367,-1.20867368964902));
#34196=CARTESIAN_POINT('Ctrl Pts',(163.758421683633,3.13281083458346,2.58314845256596));
#34197=CARTESIAN_POINT('Ctrl Pts',(163.916268699532,-0.447830144798535,
4.03566696032851));
#34198=CARTESIAN_POINT('Ctrl Pts',(164.07411571543,-3.62291538296715,1.83347860122158));
#34199=CARTESIAN_POINT('Ctrl Pts',(164.231962731329,-3.51708228511447,-2.02911109922828));
#34200=CARTESIAN_POINT('Ctrl Pts',(164.389809747227,-0.226173484754741,
-4.0541343352276));
#34201=CARTESIAN_POINT('Ctrl Pts',(164.547656763125,3.26955840828401,-2.40772661822243));
#34202=CARTESIAN_POINT('Ctrl Pts',(164.705503779024,3.80437264289096,1.41912242153392));
#34203=CARTESIAN_POINT('Ctrl Pts',(164.863350794922,0.893940538099236,3.96081178139284));
#34204=CARTESIAN_POINT('Ctrl Pts',(165.021197810821,-2.82604563923625,2.91558325180936));
#34205=CARTESIAN_POINT('Ctrl Pts',(165.179044826719,-3.98676007652644,-0.770002432134042));
#34206=CARTESIAN_POINT('Ctrl Pts',(165.336891842617,-1.53705780414438,-3.75827260320434));
#34207=CARTESIAN_POINT('Ctrl Pts',(165.494738858516,2.30460663132077,-3.34304470926576));
#34208=CARTESIAN_POINT('Ctrl Pts',(165.652585874414,4.05921537965474,0.0996501623271599));
#34209=CARTESIAN_POINT('Ctrl Pts',(165.810432890313,2.13779177250447,3.45210167733942));
#34210=CARTESIAN_POINT('Ctrl Pts',(165.968279906211,-1.71961970175989,3.67832403882484));
#34211=CARTESIAN_POINT('Ctrl Pts',(166.12612692211,-4.01974064779039,0.573449891253934));
#34212=CARTESIAN_POINT('Ctrl Pts',(166.283973938008,-2.67957762268814,-3.05074145369063));
#34213=CARTESIAN_POINT('Ctrl Pts',(166.441820953907,1.08721545742514,-3.9121761466495));
#34214=CARTESIAN_POINT('Ctrl Pts',(166.599667969805,3.86942436915232,-1.23073746375402));
#34215=CARTESIAN_POINT('Ctrl Pts',(166.757514985703,3.14747598747837,2.565259160694));
#34216=CARTESIAN_POINT('Ctrl Pts',(166.915362001602,-0.424832004595041,
4.03815272385149));
#34217=CARTESIAN_POINT('Ctrl Pts',(167.0732090175,-3.61241141035989,1.854088308463));
#34218=CARTESIAN_POINT('Ctrl Pts',(167.231056033399,-3.52858489557144,-2.0090416342183));
#34219=CARTESIAN_POINT('Ctrl Pts',(167.388903049297,-0.24926589467184,-4.0527800541148));
#34220=CARTESIAN_POINT('Ctrl Pts',(167.546750065196,3.25578872462467,-2.42631396028723));
#34221=CARTESIAN_POINT('Ctrl Pts',(167.704597081094,3.81239553444338,1.39742618489607));
#34222=CARTESIAN_POINT('Ctrl Pts',(167.862444096993,0.916490460621058,3.95565479900198));
#34223=CARTESIAN_POINT('Ctrl Pts',(168.020291112891,-2.80938993395512,2.93163569569484));
#34224=CARTESIAN_POINT('Ctrl Pts',(168.178138128789,-3.99108202353092,-0.747277682472601));
#34225=CARTESIAN_POINT('Ctrl Pts',(168.335985144688,-1.55844344087465,-3.74945511972991));
#34226=CARTESIAN_POINT('Ctrl Pts',(168.493832160586,2.28552417388456,-3.3561196200212));
#34227=CARTESIAN_POINT('Ctrl Pts',(168.651679176485,4.05971720743093,0.0765235187789346));
#34228=CARTESIAN_POINT('Ctrl Pts',(168.809526192383,2.15742342942316,3.43986682873663));
#34229=CARTESIAN_POINT('Ctrl Pts',(168.967373208282,-1.69863667764873,3.68806088491128));
#34230=CARTESIAN_POINT('Ctrl Pts',(169.12522022418,-4.01640851875484,0.596340727586192));
#34231=CARTESIAN_POINT('Ctrl Pts',(169.283067240078,-2.69691397060336,-3.03542660733155));
#34232=CARTESIAN_POINT('Ctrl Pts',(169.440914255977,1.0649104590364,-3.91830644142532));
#34233=CARTESIAN_POINT('Ctrl Pts',(169.598761271875,3.86235016417448,-1.25276129380414));
#34234=CARTESIAN_POINT('Ctrl Pts',(169.756608287774,3.16203898921731,2.54728661237238));
#34235=CARTESIAN_POINT('Ctrl Pts',(169.914455303672,-0.401820077801361,
4.04050742956116));
#34236=CARTESIAN_POINT('Ctrl Pts',(170.072302319571,-3.60179019351355,1.87463783874864));
#34237=CARTESIAN_POINT('Ctrl Pts',(170.230149335469,-3.53997299095283,-1.98890696095539));
#34238=CARTESIAN_POINT('Ctrl Pts',(170.387996351368,-0.272350203051137,
-4.05129424840711));
#34239=CARTESIAN_POINT('Ctrl Pts',(170.545843367266,3.24191335042212,-2.44482253765146));
#34240=CARTESIAN_POINT('Ctrl Pts',(170.703690383165,3.82029474133155,1.37568455761573));
#34241=CARTESIAN_POINT('Ctrl Pts',(170.861537399063,0.939010542792494,3.95036950984758));
#34242=CARTESIAN_POINT('Ctrl Pts',(171.019384414962,-2.79264285646855,2.94759284198226));
#34243=CARTESIAN_POINT('Ctrl Pts',(171.17723143086,-3.99527482932224,-0.724528374886929));
#34244=CARTESIAN_POINT('Ctrl Pts',(171.335078446758,-1.57977770992274,-3.74051656323585));
#34245=CARTESIAN_POINT('Ctrl Pts',(171.492925462657,2.26636594667525,-3.36908436220139));
#34246=CARTESIAN_POINT('Ctrl Pts',(171.650772478555,4.06009049502634,0.0533918753788966));
#34247=CARTESIAN_POINT('Ctrl Pts',(171.808619494454,2.17697856253166,3.42752542365741));
#34248=CARTESIAN_POINT('Ctrl Pts',(171.966466510352,-1.67758537992403,3.69766775849278));
#34249=CARTESIAN_POINT('Ctrl Pts',(172.12431352625,-4.0129725985565,0.619232975460156));
#34250=CARTESIAN_POINT('Ctrl Pts',(172.282160542149,-2.7141091122044,-3.02005521015814));
#34251=CARTESIAN_POINT('Ctrl Pts',(172.440007558047,1.04246242519302,-3.9242247633699));
#34252=CARTESIAN_POINT('Ctrl Pts',(172.597854573946,3.85536981515549,-1.27491584316685));
#34253=CARTESIAN_POINT('Ctrl Pts',(172.755701589844,3.17605635463602,2.52957777651284));
#34254=CARTESIAN_POINT('Ctrl Pts',(172.913548605743,-0.377899477148265,
4.04203024535818));
#34255=CARTESIAN_POINT('Ctrl Pts',(173.071395621641,-3.59286760329576,1.89655655093627));
#34256=CARTESIAN_POINT('Ctrl Pts',(173.22924263754,-3.54749742974178,-1.97171790003568));
#34257=CARTESIAN_POINT('Ctrl Pts',(173.334473981472,-1.38531872496892,-3.35008700244825));
#34258=CARTESIAN_POINT('Ctrl Pts',(173.387089653438,-0.25042991768545,-3.43287763491915));
#34259=CARTESIAN_POINT('Ctrl Pts',(172.148679545343,-3.44468745739532,0.00260595186748766));
#34260=CARTESIAN_POINT('Ctrl Pts',(172.193173210945,-3.43659168049753,-0.9575193993669));
#34261=CARTESIAN_POINT('Ctrl Pts',(172.237666876547,-3.01700009266596,-1.92385078687646));
#34262=CARTESIAN_POINT('Ctrl Pts',(172.282160542149,-2.30449110369684,-2.56420210475706));
#34263=CARTESIAN_POINT('Ctrl Pts',(172.334776214115,-1.46191859973859,-3.32144506122872));
#34264=CARTESIAN_POINT('Ctrl Pts',(172.387391886081,-0.20972808727278,-3.62283491229931));
#34265=CARTESIAN_POINT('Ctrl Pts',(172.440007558047,0.885185067287182,-3.3319783511341));
#34266=CARTESIAN_POINT('Ctrl Pts',(172.492623230014,1.98009822184718,-3.04112178996889));
#34267=CARTESIAN_POINT('Ctrl Pts',(172.54523890198,2.91773401850134,-2.15801881656787));
#34268=CARTESIAN_POINT('Ctrl Pts',(172.597854573946,3.27333300674184,-1.08238505992073));
#34269=CARTESIAN_POINT('Ctrl Pts',(172.650470245912,3.62893199498233,-0.00675130327361259));
#34270=CARTESIAN_POINT('Ctrl Pts',(172.703085917878,3.40249417480918,1.2614132366196));
#34271=CARTESIAN_POINT('Ctrl Pts',(172.755701589844,2.69694929275856,2.14757091804043));
#34272=CARTESIAN_POINT('Ctrl Pts',(172.80831726181,1.99140441070795,3.03372859946126));
#34273=CARTESIAN_POINT('Ctrl Pts',(172.860932933777,0.80675246677985,3.53787942240972));
#34274=CARTESIAN_POINT('Ctrl Pts',(172.913548605743,-0.321401526208764,
3.43237588481364));
#34275=CARTESIAN_POINT('Ctrl Pts',(172.961699070495,-1.35381519774084,3.33582586124758));
#34276=CARTESIAN_POINT('Ctrl Pts',(173.009849535248,-2.33891337062945,2.72870687739777));
#34277=CARTESIAN_POINT('Ctrl Pts',(173.058,-2.9035416885497,1.85819928779561));
#34278=CARTESIAN_POINT('',(156.971,-1.66746714335626,-2.33836210323109));
#34279=CARTESIAN_POINT('Ctrl Pts',(156.971,-1.67108163325028,-2.34115360979857));
#34280=CARTESIAN_POINT('Ctrl Pts',(156.971,-1.74156582682502,-2.30101299952705));
#34281=CARTESIAN_POINT('Ctrl Pts',(156.971,-1.81009195136928,-2.25780466502739));
#34282=CARTESIAN_POINT('Ctrl Pts',(156.971,-1.87643000725441,-2.2115735151457));
#34283=CARTESIAN_POINT('Ctrl Pts',(156.971,-1.95407697057863,-2.15746116060946));
#34284=CARTESIAN_POINT('Ctrl Pts',(156.971,-2.0287275990739,-2.0992089256144));
#34285=CARTESIAN_POINT('Ctrl Pts',(156.971,-2.10029440757325,-2.03719493253877));
#34286=CARTESIAN_POINT('Ctrl Pts',(156.971,-2.14317936038372,-2.00003430986464));
#34287=CARTESIAN_POINT('Ctrl Pts',(156.971,-2.18495660149505,-1.96152195550082));
#34288=CARTESIAN_POINT('Ctrl Pts',(156.971,-2.22560317199605,-1.92173149895334));
#34289=CARTESIAN_POINT('Ctrl Pts',(156.971,-2.23928658627073,-1.90833629009791));
#34290=CARTESIAN_POINT('Ctrl Pts',(156.971,-2.25284183387164,-1.89479619102025));
#34291=CARTESIAN_POINT('Ctrl Pts',(156.971,-2.26626794759505,-1.88111388128463));
#34292=CARTESIAN_POINT('Ctrl Pts',(156.971,-2.27898720160856,-1.86815191949852));
#34293=CARTESIAN_POINT('Ctrl Pts',(156.971,-2.29158455101912,-1.85506841721476));
#34294=CARTESIAN_POINT('Ctrl Pts',(156.971,-2.30405686724598,-1.8418688091367));
#34295=CARTESIAN_POINT('Ctrl Pts',(156.971,-2.3741795820906,-1.7676570639818));
#34296=CARTESIAN_POINT('Ctrl Pts',(156.971,-2.44037916018597,-1.68975253852306));
#34297=CARTESIAN_POINT('Ctrl Pts',(156.971,-2.50254990372574,-1.60861131636701));
#34298=CARTESIAN_POINT('Ctrl Pts',(156.971,-2.55694930432303,-1.53761274698046));
#34299=CARTESIAN_POINT('Ctrl Pts',(156.971,-2.60826396461782,-1.46413480075326));
#34300=CARTESIAN_POINT('Ctrl Pts',(156.971,-2.65640196169989,-1.3884517272919));
#34301=CARTESIAN_POINT('Ctrl Pts',(156.971,-2.68077979569537,-1.35012463615922));
#34302=CARTESIAN_POINT('Ctrl Pts',(156.971,-2.70434261126781,-1.31123160616743));
#34303=CARTESIAN_POINT('Ctrl Pts',(156.971,-2.72707617605973,-1.27180597383338));
#34304=CARTESIAN_POINT('Ctrl Pts',(156.971,-2.73546680340987,-1.25725454769381));
#34305=CARTESIAN_POINT('Ctrl Pts',(156.971,-2.74374453865664,-1.24263023968055));
#34306=CARTESIAN_POINT('Ctrl Pts',(156.971,-2.75190137317708,-1.22794817412566));
#34307=CARTESIAN_POINT('Ctrl Pts',(156.971,-2.80132721807123,-1.13898308687001));
#34308=CARTESIAN_POINT('Ctrl Pts',(156.971,-2.84638527771199,-1.04778307946572));
#34309=CARTESIAN_POINT('Ctrl Pts',(156.971,-2.88697808172597,-0.95476457681926));
#34310=CARTESIAN_POINT('Ctrl Pts',(156.971,-2.92819643846301,-0.860312618686309));
#34311=CARTESIAN_POINT('Ctrl Pts',(156.971,-2.96481143066595,-0.763984967763502));
#34312=CARTESIAN_POINT('Ctrl Pts',(156.971,-2.9966850422333,-0.666177951518305));
#34313=CARTESIAN_POINT('Ctrl Pts',(156.971,-3.02841101938765,-0.568823964619975));
#34314=CARTESIAN_POINT('Ctrl Pts',(156.971,-3.05543990645514,-0.470003430106361));
#34315=CARTESIAN_POINT('Ctrl Pts',(156.971,-3.07759256720278,-0.37008023699904));
#34316=CARTESIAN_POINT('Ctrl Pts',(156.971,-3.09152323719072,-0.30724367559562));
#34317=CARTESIAN_POINT('Ctrl Pts',(156.971,-3.10352472126607,-0.243970573036485));
#34318=CARTESIAN_POINT('Ctrl Pts',(156.971,-3.11354240097713,-0.180348235662287));
#34319=CARTESIAN_POINT('Ctrl Pts',(156.971,-3.11596207334912,-0.164980883498373));
#34320=CARTESIAN_POINT('Ctrl Pts',(156.971,-3.11826596901285,-0.149593149423556));
#34321=CARTESIAN_POINT('Ctrl Pts',(156.971,-3.12045324378791,-0.134186252698088));
#34322=CARTESIAN_POINT('Ctrl Pts',(156.971,-3.1225086104187,-0.119708500851479));
#34323=CARTESIAN_POINT('Ctrl Pts',(156.971,-3.12445959438249,-0.105223701268543));
#34324=CARTESIAN_POINT('Ctrl Pts',(156.971,-3.12630586019491,-0.0907332361958907));
#34325=CARTESIAN_POINT('Ctrl Pts',(156.971,-3.13964539671036,0.0139624618244236));
#34326=CARTESIAN_POINT('Ctrl Pts',(156.971,-3.14752256490358,0.118955963700162));
#34327=CARTESIAN_POINT('Ctrl Pts',(156.971,-3.14979998981073,0.223838097043022));
#34328=CARTESIAN_POINT('Ctrl Pts',(156.971,-3.15103815096673,0.280859069745446));
#34329=CARTESIAN_POINT('Ctrl Pts',(156.971,-3.15062042229049,0.337847632866582));
#34330=CARTESIAN_POINT('Ctrl Pts',(156.971,-3.14851887087268,0.394740793443));
#34331=CARTESIAN_POINT('Ctrl Pts',(156.971,-3.14477596423555,0.496068691739228));
#34332=CARTESIAN_POINT('Ctrl Pts',(156.971,-3.13569517353071,0.597093830712654));
#34333=CARTESIAN_POINT('Ctrl Pts',(156.971,-3.1215328967269,0.697540099410437));
#34334=CARTESIAN_POINT('Ctrl Pts',(156.971,-3.10710264617045,0.799886978012563));
#34335=CARTESIAN_POINT('Ctrl Pts',(156.971,-3.08739665071869,0.90163358834031));
#34336=CARTESIAN_POINT('Ctrl Pts',(156.971,-3.06263213549149,1.00248789881405));
#34337=CARTESIAN_POINT('Ctrl Pts',(156.971,-3.05639992686936,1.02786877534427));
#34338=CARTESIAN_POINT('Ctrl Pts',(156.971,-3.04984709488345,1.05319311007923));
#34339=CARTESIAN_POINT('Ctrl Pts',(156.971,-3.04297659426579,1.07845616335264));
#34340=CARTESIAN_POINT('Ctrl Pts',(156.971,-3.03886751101771,1.09356539552918));
#34341=CARTESIAN_POINT('Ctrl Pts',(156.971,-3.03464709377404,1.10864418789391));
#34342=CARTESIAN_POINT('Ctrl Pts',(156.971,-3.0303173931493,1.12368807181908));
#34343=CARTESIAN_POINT('Ctrl Pts',(156.971,-3.00104329645236,1.22540321355577));
#34344=CARTESIAN_POINT('Ctrl Pts',(156.971,-2.96676399966351,1.32557352761962));
#34345=CARTESIAN_POINT('Ctrl Pts',(156.971,-2.92778796706529,1.42390018595887));
#34346=CARTESIAN_POINT('Ctrl Pts',(156.971,-2.88830860897673,1.52349660702726));
#34347=CARTESIAN_POINT('Ctrl Pts',(156.971,-2.84401017748247,1.62120220936028));
#34348=CARTESIAN_POINT('Ctrl Pts',(156.971,-2.79515759563137,1.7167066642448));
#34349=CARTESIAN_POINT('Ctrl Pts',(156.971,-2.74593458387645,1.81293529182803));
#34350=CARTESIAN_POINT('Ctrl Pts',(156.971,-2.69208777854597,1.90693009151836));
#34351=CARTESIAN_POINT('Ctrl Pts',(156.971,-2.63383640916819,1.99836181408463));
#34352=CARTESIAN_POINT('Ctrl Pts',(156.971,-2.59840301290045,2.05397829987267));
#34353=CARTESIAN_POINT('Ctrl Pts',(156.971,-2.56133889987228,2.10864614082127));
#34354=CARTESIAN_POINT('Ctrl Pts',(156.971,-2.52268492979926,2.16228709920977));
#34355=CARTESIAN_POINT('Ctrl Pts',(156.971,-2.51023398438858,2.17956554805759));
#34356=CARTESIAN_POINT('Ctrl Pts',(156.971,-2.49761803355936,2.19673742063913));
#34357=CARTESIAN_POINT('Ctrl Pts',(156.971,-2.48483831170471,2.2138000097301));
#34358=CARTESIAN_POINT('Ctrl Pts',(156.971,-2.475084819656,2.22682218884494));
#34359=CARTESIAN_POINT('Ctrl Pts',(156.971,-2.46524087000302,2.23977408134567));
#34360=CARTESIAN_POINT('Ctrl Pts',(156.971,-2.45531045458567,2.25265065830578));
#34361=CARTESIAN_POINT('Ctrl Pts',(156.971,-2.38739538388514,2.34071481251011));
#34362=CARTESIAN_POINT('Ctrl Pts',(156.971,-2.31539519512402,2.42531743730386));
#34363=CARTESIAN_POINT('Ctrl Pts',(156.971,-2.23958992023872,2.50613621189154));
#34364=CARTESIAN_POINT('Ctrl Pts',(156.971,-2.16373640953125,2.58700641245246));
#34365=CARTESIAN_POINT('Ctrl Pts',(156.971,-2.0840725443841,2.66408878647399));
#34366=CARTESIAN_POINT('Ctrl Pts',(156.971,-2.00083019937915,2.73704166286336));
#34367=CARTESIAN_POINT('Ctrl Pts',(156.971,-1.91931149938911,2.80848395156199));
#34368=CARTESIAN_POINT('Ctrl Pts',(156.971,-1.83436044394798,2.87596668131474));
#34369=CARTESIAN_POINT('Ctrl Pts',(156.971,-1.74615546237234,2.93913980004792));
#34370=CARTESIAN_POINT('Ctrl Pts',(156.971,-1.67008718098456,2.99362051628523));
#34371=CARTESIAN_POINT('Ctrl Pts',(156.971,-1.59159806355185,3.04489584580896));
#34372=CARTESIAN_POINT('Ctrl Pts',(156.971,-1.51078263890252,3.09271722244222));
#34373=CARTESIAN_POINT('Ctrl Pts',(156.971,-1.67108163325026,-2.34115360979858));
#34374=CARTESIAN_POINT('Ctrl Pts',(157.019150464752,-0.963356763333181,
-2.83982097002305));
#34375=CARTESIAN_POINT('Ctrl Pts',(157.119916601471,1.02786046454763,-3.18314302195819));
#34376=CARTESIAN_POINT('Ctrl Pts',(157.273298410156,3.24548551852033,-0.972003967714269));
#34377=CARTESIAN_POINT('Ctrl Pts',(157.431145426054,2.58940221207372,2.18521955033239));
#34378=CARTESIAN_POINT('Ctrl Pts',(157.588992441952,-0.412068725742385,
3.36277947991426));
#34379=CARTESIAN_POINT('Ctrl Pts',(157.71847393057,-2.56788618045525,1.83093969563411));
#34380=CARTESIAN_POINT('Ctrl Pts',(157.79533974722,-2.86840235184534,0.439819957054708));
#34381=CARTESIAN_POINT('Ctrl Pts',(157.819589891905,-2.86758689937222,0.000602879185874344));
#34382=CARTESIAN_POINT('Origin',(156.971,-8.10351388986772E-16,-1.22178682300763E-16));
#34383=CARTESIAN_POINT('',(156.971,-3.442,-4.21523428266519E-16));
#34384=CARTESIAN_POINT('Origin',(156.971,0.,0.));
#34385=CARTESIAN_POINT('Origin',(156.971,0.,0.));
#34386=CARTESIAN_POINT('',(156.971,1.66746714335746,-2.33836210323023));
#34387=CARTESIAN_POINT('Ctrl Pts',(156.971,1.51450577336034,3.09672906731566));
#34388=CARTESIAN_POINT('Ctrl Pts',(156.971,1.5976122133282,3.04813379956916));
#34389=CARTESIAN_POINT('Ctrl Pts',(156.971,1.67839168866948,2.99593162634641));
#34390=CARTESIAN_POINT('Ctrl Pts',(156.971,1.75657288137401,2.94011204420089));
#34391=CARTESIAN_POINT('Ctrl Pts',(156.971,1.84626732484938,2.87607226452533));
#34392=CARTESIAN_POINT('Ctrl Pts',(156.971,1.93254295618487,2.80727123920175));
#34393=CARTESIAN_POINT('Ctrl Pts',(156.971,2.0152189467617,2.73410403576512));
#34394=CARTESIAN_POINT('Ctrl Pts',(156.971,2.06094021411052,2.69364129384751));
#34395=CARTESIAN_POINT('Ctrl Pts',(156.971,2.10555989642535,2.65184263331913));
#34396=CARTESIAN_POINT('Ctrl Pts',(156.971,2.14904172716354,2.60877124230549));
#34397=CARTESIAN_POINT('Ctrl Pts',(156.971,2.16594615215952,2.59202638390138));
#34398=CARTESIAN_POINT('Ctrl Pts',(156.971,2.18267855444771,2.57508914036822));
#34399=CARTESIAN_POINT('Ctrl Pts',(156.971,2.19923662551325,2.55796314915767));
#34400=CARTESIAN_POINT('Ctrl Pts',(156.971,2.21227815538319,2.54447431189873));
#34401=CARTESIAN_POINT('Ctrl Pts',(156.971,2.22521082737741,2.53086901431116));
#34402=CARTESIAN_POINT('Ctrl Pts',(156.971,2.23802494129898,2.51715852867729));
#34403=CARTESIAN_POINT('Ctrl Pts',(156.971,2.3130983252954,2.43683361826452));
#34404=CARTESIAN_POINT('Ctrl Pts',(156.971,2.38418748200277,2.35281708657033));
#34405=CARTESIAN_POINT('Ctrl Pts',(156.971,2.45111847796041,2.26550571111247));
#34406=CARTESIAN_POINT('Ctrl Pts',(156.971,2.50946613003779,2.1893912937977));
#34407=CARTESIAN_POINT('Ctrl Pts',(156.971,2.56465324413205,2.11077199669919));
#34408=CARTESIAN_POINT('Ctrl Pts',(156.971,2.61653549626154,2.02989655843326));
#34409=CARTESIAN_POINT('Ctrl Pts',(156.971,2.6392339815682,1.99451355419192));
#34410=CARTESIAN_POINT('Ctrl Pts',(156.971,2.66129952851454,1.95869858631448));
#34411=CARTESIAN_POINT('Ctrl Pts',(156.971,2.68271827828137,1.92247205653849));
#34412=CARTESIAN_POINT('Ctrl Pts',(156.971,2.69702185774087,1.89827974593054));
#34413=CARTESIAN_POINT('Ctrl Pts',(156.971,2.71103696537232,1.87390388858616));
#34414=CARTESIAN_POINT('Ctrl Pts',(156.971,2.72475919182257,1.84935053082851));
#34415=CARTESIAN_POINT('Ctrl Pts',(156.971,2.73246069787352,1.83557012616698));
#34416=CARTESIAN_POINT('Ctrl Pts',(156.971,2.74006809732495,1.82173703740762));
#34417=CARTESIAN_POINT('Ctrl Pts',(156.971,2.7475769083573,1.80785967126201));
#34418=CARTESIAN_POINT('Ctrl Pts',(156.971,2.79902208258213,1.71278156687673));
#34419=CARTESIAN_POINT('Ctrl Pts',(156.971,2.84589995525172,1.61552594512813));
#34420=CARTESIAN_POINT('Ctrl Pts',(156.971,2.88804364556441,1.51646223851979));
#34421=CARTESIAN_POINT('Ctrl Pts',(156.971,2.92990919612424,1.41805233215221));
#34422=CARTESIAN_POINT('Ctrl Pts',(156.971,2.96710310392466,1.31785723800263));
#34423=CARTESIAN_POINT('Ctrl Pts',(156.971,2.99941240513831,1.21622594408559));
#34424=CARTESIAN_POINT('Ctrl Pts',(156.971,3.03075374377295,1.1176394479721));
#34425=CARTESIAN_POINT('Ctrl Pts',(156.971,3.05749880022788,1.01770075724612));
#34426=CARTESIAN_POINT('Ctrl Pts',(156.971,3.07940480525096,0.916728058706169));
#34427=CARTESIAN_POINT('Ctrl Pts',(156.971,3.09348952736189,0.851806481347487));
#34428=CARTESIAN_POINT('Ctrl Pts',(156.971,3.10557281263683,0.786457470967977));
#34429=CARTESIAN_POINT('Ctrl Pts',(156.971,3.1155789372591,0.720767651007633));
#34430=CARTESIAN_POINT('Ctrl Pts',(156.971,3.11874731606386,0.699967367070817));
#34431=CARTESIAN_POINT('Ctrl Pts',(156.971,3.12170736344965,0.679132930743779));
#34432=CARTESIAN_POINT('Ctrl Pts',(156.971,3.1244564832137,0.658267149344455));
#34433=CARTESIAN_POINT('Ctrl Pts',(156.971,3.12656936527807,0.6422304033816));
#34434=CARTESIAN_POINT('Ctrl Pts',(156.971,3.12855665844618,0.626182400243434));
#34435=CARTESIAN_POINT('Ctrl Pts',(156.971,3.1304167981429,0.610131368191127));
#34436=CARTESIAN_POINT('Ctrl Pts',(156.971,3.14217399496676,0.508679233495234));
#34437=CARTESIAN_POINT('Ctrl Pts',(156.971,3.14886713191197,0.407018714846757));
#34438=CARTESIAN_POINT('Ctrl Pts',(156.971,3.15030637585759,0.305461515249309));
#34439=CARTESIAN_POINT('Ctrl Pts',(156.971,3.15115016476314,0.245921338922451));
#34440=CARTESIAN_POINT('Ctrl Pts',(156.971,3.15018716918967,0.186416637507053));
#34441=CARTESIAN_POINT('Ctrl Pts',(156.971,3.14737077987805,0.127010997247052));
#34442=CARTESIAN_POINT('Ctrl Pts',(156.971,3.14248054125356,0.023861991776158));
#34443=CARTESIAN_POINT('Ctrl Pts',(156.971,3.13200499774187,-0.0789895992824285));
#34444=CARTESIAN_POINT('Ctrl Pts',(156.971,3.11615067386057,-0.181195593903271));
#34445=CARTESIAN_POINT('Ctrl Pts',(156.971,3.10022872402003,-0.283837543944141));
#34446=CARTESIAN_POINT('Ctrl Pts',(156.971,3.0788814745367,-0.385829206510234));
#34447=CARTESIAN_POINT('Ctrl Pts',(156.971,3.05227309403315,-0.486791749188485));
#34448=CARTESIAN_POINT('Ctrl Pts',(156.971,3.04731684429539,-0.505597688001841));
#34449=CARTESIAN_POINT('Ctrl Pts',(156.971,3.04217794647225,-0.524367828260039));
#34450=CARTESIAN_POINT('Ctrl Pts',(156.971,3.03685731319712,-0.543099585892552));
#34451=CARTESIAN_POINT('Ctrl Pts',(156.971,3.03263009161328,-0.557981891451461));
#34452=CARTESIAN_POINT('Ctrl Pts',(156.971,3.0282903986042,-0.572831979422245));
#34453=CARTESIAN_POINT('Ctrl Pts',(156.971,3.02384043003072,-0.587644229154542));
#34454=CARTESIAN_POINT('Ctrl Pts',(156.971,2.99455675703092,-0.685118418104316));
#34455=CARTESIAN_POINT('Ctrl Pts',(156.971,2.96048389838246,-0.781018415258394));
#34456=CARTESIAN_POINT('Ctrl Pts',(156.971,2.92185171768902,-0.875024422665997));
#34457=CARTESIAN_POINT('Ctrl Pts',(156.971,2.88316491075989,-0.969163355376433));
#34458=CARTESIAN_POINT('Ctrl Pts',(156.971,2.83990529823815,-1.06140371995399));
#34459=CARTESIAN_POINT('Ctrl Pts',(156.971,2.79225847108116,-1.15139825807016));
#34460=CARTESIAN_POINT('Ctrl Pts',(156.971,2.74521780506821,-1.24024788905535));
#34461=CARTESIAN_POINT('Ctrl Pts',(156.971,2.69390022278398,-1.32690912442467));
#34462=CARTESIAN_POINT('Ctrl Pts',(156.971,2.63844931031572,-1.41101183192941));
#34463=CARTESIAN_POINT('Ctrl Pts',(156.971,2.60730719276541,-1.45824525491251));
#34464=CARTESIAN_POINT('Ctrl Pts',(156.971,2.57486079116401,-1.50467098225265));
#34465=CARTESIAN_POINT('Ctrl Pts',(156.971,2.54113168514896,-1.55021721735793));
#34466=CARTESIAN_POINT('Ctrl Pts',(156.971,2.53163696619057,-1.56303844961189));
#34467=CARTESIAN_POINT('Ctrl Pts',(156.971,2.5220405886108,-1.57578995917095));
#34468=CARTESIAN_POINT('Ctrl Pts',(156.971,2.51234300050255,-1.58847007178006));
#34469=CARTESIAN_POINT('Ctrl Pts',(156.971,2.50309786488165,-1.60055857868));
#34470=CARTESIAN_POINT('Ctrl Pts',(156.971,2.49376578236826,-1.61257556802877));
#34471=CARTESIAN_POINT('Ctrl Pts',(156.971,2.48435028538722,-1.62451626608972));
#34472=CARTESIAN_POINT('Ctrl Pts',(156.971,2.42322328666443,-1.70203729727816));
#34473=CARTESIAN_POINT('Ctrl Pts',(156.971,2.35854536219489,-1.77639557833669));
#34474=CARTESIAN_POINT('Ctrl Pts',(156.971,2.29048943148814,-1.84727574318768));
#34475=CARTESIAN_POINT('Ctrl Pts',(156.971,2.22340718132701,-1.91714182099481));
#34476=CARTESIAN_POINT('Ctrl Pts',(156.971,2.15304229743094,-1.98362914136461));
#34477=CARTESIAN_POINT('Ctrl Pts',(156.971,2.07953071995107,-2.0463957114678));
#34478=CARTESIAN_POINT('Ctrl Pts',(156.971,2.00832220888232,-2.10719584874094));
#34479=CARTESIAN_POINT('Ctrl Pts',(156.971,1.93416053444636,-2.16450503885106));
#34480=CARTESIAN_POINT('Ctrl Pts',(156.971,1.85714962127244,-2.21796859445852));
#34481=CARTESIAN_POINT('Ctrl Pts',(156.971,1.79571995702034,-2.26061512512972));
#34482=CARTESIAN_POINT('Ctrl Pts',(156.971,1.73247691508609,-2.30081400188467));
#34483=CARTESIAN_POINT('Ctrl Pts',(156.971,1.66746714335763,-2.33836210323011));
#34484=CARTESIAN_POINT('Origin',(156.971,0.,0.));
#34485=CARTESIAN_POINT('Origin',(155.122410108095,0.,0.));
#34486=CARTESIAN_POINT('Ctrl Pts',(156.971,1.66746714335746,-2.33836210323023));
#34487=CARTESIAN_POINT('Ctrl Pts',(157.023615671966,2.44051566432356,-1.78710744205035));
#34488=CARTESIAN_POINT('Ctrl Pts',(157.128847015899,3.38388779517831,0.133215779263953));
#34489=CARTESIAN_POINT('Ctrl Pts',(157.286694031797,1.73842129201381,2.91023290985255));
#34490=CARTESIAN_POINT('Ctrl Pts',(157.444541047695,-1.48379950765357,3.04509876769309));
#34491=CARTESIAN_POINT('Ctrl Pts',(157.556446406461,-2.81469700920609,1.18796503211997));
#34492=CARTESIAN_POINT('Ctrl Pts',(157.615736093261,-2.87579990686974,0.122127760897206));
#34493=CARTESIAN_POINT('Ctrl Pts',(157.622410108095,-2.87487623080957,0.00203977944324927));
#34494=CARTESIAN_POINT('Ctrl Pts',(156.641910346562,1.99840595662821,-2.80245207497164));
#34495=CARTESIAN_POINT('Ctrl Pts',(156.694526018528,2.92487984561336,-2.14179102212308));
#34496=CARTESIAN_POINT('Ctrl Pts',(156.79975736246,4.0554811250013,0.159654844089943));
#34497=CARTESIAN_POINT('Ctrl Pts',(156.957604378359,2.08344223088848,3.48782091772715));
#34498=CARTESIAN_POINT('Ctrl Pts',(157.115451394257,-1.77828617874074,3.64945332813361));
#34499=CARTESIAN_POINT('Ctrl Pts',(157.273298410156,-4.02815155478086,0.509992261095901));
#34500=CARTESIAN_POINT('Ctrl Pts',(157.431145426054,-2.63083191649386,-3.09321993275373));
#34501=CARTESIAN_POINT('Ctrl Pts',(157.588992441953,1.14932790535007,-3.89426644772928));
#34502=CARTESIAN_POINT('Ctrl Pts',(157.746839457851,3.8884790677076,-1.16912401597452));
#34503=CARTESIAN_POINT('Ctrl Pts',(157.90468647375,3.1063037483826,2.61500941800772));
#34504=CARTESIAN_POINT('Ctrl Pts',(158.062533489648,-0.488988477053649,
4.03087189984344));
#34505=CARTESIAN_POINT('Ctrl Pts',(158.220380505547,-3.64143065256987,1.79642633305765));
#34506=CARTESIAN_POINT('Ctrl Pts',(158.378227521445,-3.49619755012992,-2.06489389097847));
#34507=CARTESIAN_POINT('Ctrl Pts',(158.536074537343,-0.184796791687261,
-4.05622887980389));
#34508=CARTESIAN_POINT('Ctrl Pts',(158.693921553242,3.29395367989886,-2.37424292862959));
#34509=CARTESIAN_POINT('Ctrl Pts',(158.85176856914,3.78969536832349,1.45786484210508));
#34510=CARTESIAN_POINT('Ctrl Pts',(159.009615585039,0.853481851318687,3.96972605671494));
#34511=CARTESIAN_POINT('Ctrl Pts',(159.167462600937,-2.85564597043241,2.88659742752771));
#34512=CARTESIAN_POINT('Ctrl Pts',(159.325309616835,-3.97869609633737,-0.810639154257264));
#34513=CARTESIAN_POINT('Ctrl Pts',(159.483156632734,-1.49863219029163,-3.77375933554359));
#34514=CARTESIAN_POINT('Ctrl Pts',(159.641003648632,2.33859553970342,-3.31935674108112));
#34515=CARTESIAN_POINT('Ctrl Pts',(159.798850664531,4.057987188022,0.1410610164337));
#34516=CARTESIAN_POINT('Ctrl Pts',(159.956697680429,2.10245872402191,3.47373365282519));
#34517=CARTESIAN_POINT('Ctrl Pts',(160.114544696328,-1.75705993367321,3.66058719404933));
#34518=CARTESIAN_POINT('Ctrl Pts',(160.272391712226,-4.02538212767037,0.532406737005837));
#34519=CARTESIAN_POINT('Ctrl Pts',(160.430238728124,-2.64831141563203,-3.07792216409928));
#34520=CARTESIAN_POINT('Ctrl Pts',(160.588085744023,1.12707462054498,-3.90087951709366));
#34521=CARTESIAN_POINT('Ctrl Pts',(160.745932759921,3.8817799626603,-1.1911937404532));
#34522=CARTESIAN_POINT('Ctrl Pts',(160.90377977582,3.12113876473172,2.59723911426476));
#34523=CARTESIAN_POINT('Ctrl Pts',(161.061626791718,-0.46601100979089,4.03360780749621));
#34524=CARTESIAN_POINT('Ctrl Pts',(161.219473807617,-3.63114042085755,1.81713440607874));
#34525=CARTESIAN_POINT('Ctrl Pts',(161.377320823515,-3.50790288757611,-2.04493900570317));
#34526=CARTESIAN_POINT('Ctrl Pts',(161.535167839414,-0.207902529827338,
-4.05511217401782));
#34527=CARTESIAN_POINT('Ctrl Pts',(161.693014855312,3.28037471273009,-2.39296885684481));
#34528=CARTESIAN_POINT('Ctrl Pts',(161.850861871211,3.79793903314098,1.43625112925684));
#34529=CARTESIAN_POINT('Ctrl Pts',(162.008708887109,0.876083302092013,3.96479964860146));
#34530=CARTESIAN_POINT('Ctrl Pts',(162.166555903007,-2.83915495818497,2.902818859172));
#34531=CARTESIAN_POINT('Ctrl Pts',(162.324402918906,-3.98324965686799,-0.787959628922847));
#34532=CARTESIAN_POINT('Ctrl Pts',(162.482249934804,-1.52010668789534,-3.76516053617476));
#34533=CARTESIAN_POINT('Ctrl Pts',(162.640096950703,2.31964748443918,-3.33262565459826));
#34534=CARTESIAN_POINT('Ctrl Pts',(162.797943966601,4.05872494746307,0.117940690995252));
#34535=CARTESIAN_POINT('Ctrl Pts',(162.9557909825,2.12221419123008,3.46169974612087));
#34536=CARTESIAN_POINT('Ctrl Pts',(163.113637998398,-1.73617734800614,3.67053762029787));
#34537=CARTESIAN_POINT('Ctrl Pts',(163.271485014297,-4.02228372639134,0.555330379286925));
#34538=CARTESIAN_POINT('Ctrl Pts',(163.429332030195,-2.66580311733514,-3.06278499822593));
#34539=CARTESIAN_POINT('Ctrl Pts',(163.587179046093,1.10483333124399,-3.90723706932711));
#34540=CARTESIAN_POINT('Ctrl Pts',(163.745026061992,3.87493083492589,-1.21328860140205));
#34541=CARTESIAN_POINT('Ctrl Pts',(163.90287307789,3.13588438043163,2.57941608863644));
#34542=CARTESIAN_POINT('Ctrl Pts',(164.060720093789,-0.443024305394836,
4.03619717934853));
#34543=CARTESIAN_POINT('Ctrl Pts',(164.218567109687,-3.62072942635015,1.83779123594432));
#34544=CARTESIAN_POINT('Ctrl Pts',(164.376414125586,-3.51949581731641,-2.02492157814664));
#34545=CARTESIAN_POINT('Ctrl Pts',(164.534261141484,-0.231000806906372,
-4.05386196520801));
#34546=CARTESIAN_POINT('Ctrl Pts',(164.692108157383,3.26668892733796,-2.41161805801814));
#34547=CARTESIAN_POINT('Ctrl Pts',(164.849955173281,3.80605960997831,1.41459126642409));
#34548=CARTESIAN_POINT('Ctrl Pts',(165.00780218918,0.898656232954932,3.95974433274711));
#34549=CARTESIAN_POINT('Ctrl Pts',(165.165649205078,-2.82257175789836,2.91894619293781));
#34550=CARTESIAN_POINT('Ctrl Pts',(165.323496220976,-3.98767396155753,-0.765254586440123));
#34551=CARTESIAN_POINT('Ctrl Pts',(165.481343236875,-1.54153183970511,-3.75643951008491));
#34552=CARTESIAN_POINT('Ctrl Pts',(165.639190252773,2.30062413944776,-3.34578642096919));
#34553=CARTESIAN_POINT('Ctrl Pts',(165.797037268672,4.05933098288678,0.0948165445851432));
#34554=CARTESIAN_POINT('Ctrl Pts',(165.95488428457,2.14190078035788,3.44955348601147));
#34555=CARTESIAN_POINT('Ctrl Pts',(166.112731300469,-1.71523841378955,3.68036892031387));
#34556=CARTESIAN_POINT('Ctrl Pts',(166.270578316367,-4.01905478154481,0.578235997403664));
#34557=CARTESIAN_POINT('Ctrl Pts',(166.428425332266,-2.68320829980646,-3.04754842875405));
#34558=CARTESIAN_POINT('Ctrl Pts',(166.586272348164,1.08255618431966,-3.91346781174227));
#34559=CARTESIAN_POINT('Ctrl Pts',(166.744119364062,3.86795594571282,-1.23534408477008));
#34560=CARTESIAN_POINT('Ctrl Pts',(166.901966379961,3.15052822047051,2.56150934758601));
#34561=CARTESIAN_POINT('Ctrl Pts',(167.059813395859,-0.420023222562997,
4.03865555578329));
#34562=CARTESIAN_POINT('Ctrl Pts',(167.217660411758,-3.61020092047943,1.85838841998152));
#34563=CARTESIAN_POINT('Ctrl Pts',(167.375507427656,-3.53097452123983,-2.00483843142192));
#34564=CARTESIAN_POINT('Ctrl Pts',(167.533354443555,-0.254091586817575,
-4.05248018764552));
#34565=CARTESIAN_POINT('Ctrl Pts',(167.691201459453,3.25289712102133,-2.43018898973018));
#34566=CARTESIAN_POINT('Ctrl Pts',(167.849048475351,3.81405666052524,1.3928854927992));
#34567=CARTESIAN_POINT('Ctrl Pts',(168.00689549125,0.921199997783791,3.95456050274001));
#34568=CARTESIAN_POINT('Ctrl Pts',(168.164742507148,-2.80589695058484,2.93497879182709));
#34569=CARTESIAN_POINT('Ctrl Pts',(168.322589523047,-3.99196884562836,-0.74252470749716));
#34570=CARTESIAN_POINT('Ctrl Pts',(168.480436538945,-1.56290696085737,-3.74759656812794));
#34571=CARTESIAN_POINT('Ctrl Pts',(168.638283554844,2.28152612734524,-3.35883859930508));
#34572=CARTESIAN_POINT('Ctrl Pts',(168.796130570742,4.05980527201056,0.0716893209138078));
#34573=CARTESIAN_POINT('Ctrl Pts',(168.953977586641,2.16151785383815,3.43729527002625));
#34574=CARTESIAN_POINT('Ctrl Pts',(169.111824602539,-1.69424381141843,3.69008077345576));
#34575=CARTESIAN_POINT('Ctrl Pts',(169.269671618438,-4.01569539723208,0.601122848567297));
#34576=CARTESIAN_POINT('Ctrl Pts',(169.427518634336,-2.70052639908684,-3.03221295017554));
#34577=CARTESIAN_POINT('Ctrl Pts',(169.585365650234,1.0602439044225,-3.91957154277003));
#34578=CARTESIAN_POINT('Ctrl Pts',(169.743212666133,3.86085551819054,-1.25735947311964));
#34579=CARTESIAN_POINT('Ctrl Pts',(169.901059682031,3.16506981599229,2.54351946884677));
#34580=CARTESIAN_POINT('Ctrl Pts',(170.05890669793,-0.397008520727738,4.0409828640259));
#34581=CARTESIAN_POINT('Ctrl Pts',(170.216753713828,-3.59955521883953,1.87892527549814));
#34582=CARTESIAN_POINT('Ctrl Pts',(170.374600729727,-3.54233867955676,-1.98469018860405));
#34583=CARTESIAN_POINT('Ctrl Pts',(170.532447745625,-0.27717401355112,-4.050966944233));
#34584=CARTESIAN_POINT('Ctrl Pts',(170.690294761523,3.23899952600311,-2.44868093193939));
#34585=CARTESIAN_POINT('Ctrl Pts',(170.848141777422,3.82193036047487,1.37113427578011));
#34586=CARTESIAN_POINT('Ctrl Pts',(171.00598879332,0.943712985438493,3.94924880585936));
#34587=CARTESIAN_POINT('Ctrl Pts',(171.163835809219,-2.78912930028193,2.950915167517));
#34588=CARTESIAN_POINT('Ctrl Pts',(171.321682825117,-3.99613776073605,-0.719768773811534));
#34589=CARTESIAN_POINT('Ctrl Pts',(171.479529841016,-1.58422410125613,-3.73863594972519));
#34590=CARTESIAN_POINT('Ctrl Pts',(171.637376856914,2.26233940515993,-3.37177377940741));
#34591=CARTESIAN_POINT('Ctrl Pts',(171.795223872812,4.06017742829736,0.0485436322247005));
#34592=CARTESIAN_POINT('Ctrl Pts',(171.953070888711,2.1810049044929,3.42495810650385));
#34593=CARTESIAN_POINT('Ctrl Pts',(172.110917904609,-1.67307324287401,3.69960696884215));
#34594=CARTESIAN_POINT('Ctrl Pts',(172.268764920508,-4.01245014574975,0.624123347664986));
#34595=CARTESIAN_POINT('Ctrl Pts',(172.426611936406,-2.71726283523924,-3.01704818305721));
#34596=CARTESIAN_POINT('Ctrl Pts',(172.584458952305,1.03689846178847,-3.92500355511514));
#34597=CARTESIAN_POINT('Ctrl Pts',(172.742305968203,3.85565576660502,-1.28044714573858));
#34598=CARTESIAN_POINT('Ctrl Pts',(172.900152984102,3.17531601965564,2.52780240521317));
#34599=CARTESIAN_POINT('Ctrl Pts',(173.005384328034,0.81604732941719,3.53217463467951));
#34600=CARTESIAN_POINT('Ctrl Pts',(173.058,-0.317020535431506,3.42736954239176));
#34601=CARTESIAN_POINT('Ctrl Pts',(156.751606897708,1.8880930188713,-2.64775541772451));
#34602=CARTESIAN_POINT('Ctrl Pts',(156.804222569674,2.76342511851676,-2.02356316209884));
#34603=CARTESIAN_POINT('Ctrl Pts',(156.909453913606,3.83161668172697,0.150841822481279));
#34604=CARTESIAN_POINT('Ctrl Pts',(157.067300929505,1.96843525126359,3.29529158176895));
#34605=CARTESIAN_POINT('Ctrl Pts',(157.225147945403,-1.68012395504502,3.44800180798677));
#34606=CARTESIAN_POINT('Ctrl Pts',(157.382994961302,-3.80579571648674,0.481840451215513));
#34607=CARTESIAN_POINT('Ctrl Pts',(157.5408419772,-2.48560877177163,-2.92247275459476));
#34608=CARTESIAN_POINT('Ctrl Pts',(157.698688993099,1.08588447071426,-3.67930112958036));
#34609=CARTESIAN_POINT('Ctrl Pts',(157.856536008997,3.67383321562612,-1.10458782683006));
#34610=CARTESIAN_POINT('Ctrl Pts',(158.014383024896,2.93483433751894,2.47065968255699));
#34611=CARTESIAN_POINT('Ctrl Pts',(158.172230040794,-0.461996085815962,
3.80836589723732));
#34612=CARTESIAN_POINT('Ctrl Pts',(158.330077056692,-3.44042198784348,1.69726276441122));
#34613=CARTESIAN_POINT('Ctrl Pts',(158.487924072591,-3.30320582016923,-1.95091078833877));
#34614=CARTESIAN_POINT('Ctrl Pts',(158.645771088489,-0.174595922884049,
-3.83232316011687));
#34615=CARTESIAN_POINT('Ctrl Pts',(158.803618104388,3.11212590558719,-2.24318361531184));
#34616=CARTESIAN_POINT('Ctrl Pts',(158.961465120286,3.58050242236722,1.37739002513823));
#34617=CARTESIAN_POINT('Ctrl Pts',(159.119312136185,0.806369256388234,3.75059533307292));
#34618=CARTESIAN_POINT('Ctrl Pts',(159.277159152083,-2.6980129854289,2.72725590770484));
#34619=CARTESIAN_POINT('Ctrl Pts',(159.435006167981,-3.7590702223385,-0.765891496119899));
#34620=CARTESIAN_POINT('Ctrl Pts',(159.59285318388,-1.4159069967543,-3.56544606600458));
#34621=CARTESIAN_POINT('Ctrl Pts',(159.750700199778,2.20950397882498,-3.13612670598366));
#34622=CARTESIAN_POINT('Ctrl Pts',(159.908547215677,3.83398440890398,0.13327438275493));
#34623=CARTESIAN_POINT('Ctrl Pts',(160.066394231575,1.98640202513631,3.28198194043799));
#34624=CARTESIAN_POINT('Ctrl Pts',(160.224241247473,-1.66006940857215,3.45852107932842));
#34625=CARTESIAN_POINT('Ctrl Pts',(160.382088263372,-3.8031791630401,0.503017637635941));
#34626=CARTESIAN_POINT('Ctrl Pts',(160.53993527927,-2.50212339443211,-2.90801942988115));
#34627=CARTESIAN_POINT('Ctrl Pts',(160.697782295169,1.06485957757476,-3.68554915444177));
#34628=CARTESIAN_POINT('Ctrl Pts',(160.855629311067,3.66750390429149,-1.1254392922585));
#34629=CARTESIAN_POINT('Ctrl Pts',(161.013476326966,2.94885045406958,2.45387030784109));
#34630=CARTESIAN_POINT('Ctrl Pts',(161.171323342864,-0.440286985427089,
3.81095078151588));
#34631=CARTESIAN_POINT('Ctrl Pts',(161.329170358763,-3.43069978170505,1.71682774217548));
#34632=CARTESIAN_POINT('Ctrl Pts',(161.487017374661,-3.31426501754721,-1.93205742200662));
#34633=CARTESIAN_POINT('Ctrl Pts',(161.64486439056,-0.196426213538184,-3.83126809700928));
#34634=CARTESIAN_POINT('Ctrl Pts',(161.802711406458,3.09929650371827,-2.26087586358491));
#34635=CARTESIAN_POINT('Ctrl Pts',(161.960558422357,3.58829103305475,1.35696939928626));
#34636=CARTESIAN_POINT('Ctrl Pts',(162.118405438255,0.827723096572676,3.74594086497732));
#34637=CARTESIAN_POINT('Ctrl Pts',(162.276252454153,-2.68243228472329,2.7425819087819));
#34638=CARTESIAN_POINT('Ctrl Pts',(162.434099470052,-3.76337242421112,-0.74446389112643));
#34639=CARTESIAN_POINT('Ctrl Pts',(162.59194648595,-1.43619609210796,-3.55732192435803));
#34640=CARTESIAN_POINT('Ctrl Pts',(162.749793501849,2.19160186501925,-3.14866316930665));
#34641=CARTESIAN_POINT('Ctrl Pts',(162.907640517747,3.83468144368097,0.111430310028073));
#34642=CARTESIAN_POINT('Ctrl Pts',(163.065487533646,2.00506698137134,3.27061231097766));
#34643=CARTESIAN_POINT('Ctrl Pts',(163.223334549544,-1.64033955134109,3.46792223742261));
#34644=CARTESIAN_POINT('Ctrl Pts',(163.381181565443,-3.80025179495196,0.524675884207151));
#34645=CARTESIAN_POINT('Ctrl Pts',(163.539028581341,-2.51864954607026,-2.89371784260046));
#34646=CARTESIAN_POINT('Ctrl Pts',(163.69687559724,1.04384601778196,-3.69155576683664));
#34647=CARTESIAN_POINT('Ctrl Pts',(163.854722613138,3.66103285159181,-1.14631450661227));
#34648=CARTESIAN_POINT('Ctrl Pts',(164.012569629036,2.96278210492842,2.43703112151242));
#34649=CARTESIAN_POINT('Ctrl Pts',(164.170416644935,-0.418569157798979,
3.81339721883829));
#34650=CARTESIAN_POINT('Ctrl Pts',(164.328263660833,-3.42086347893396,1.73634430543023));
#34651=CARTESIAN_POINT('Ctrl Pts',(164.486110676732,-3.32521801217691,-1.91314496575622));
#34652=CARTESIAN_POINT('Ctrl Pts',(164.64395769263,-0.218249454985314,-3.83008690030693));
#34653=CARTESIAN_POINT('Ctrl Pts',(164.801804708529,3.08636618004157,-2.27849562018446));
#34654=CARTESIAN_POINT('Ctrl Pts',(164.959651724427,3.59596335027584,1.33650517095037));
#34655=CARTESIAN_POINT('Ctrl Pts',(165.117498740325,0.849049991159028,3.74116460490808));
#34656=CARTESIAN_POINT('Ctrl Pts',(165.275345756224,-2.66676448480114,2.75781900622711));
#34657=CARTESIAN_POINT('Ctrl Pts',(165.433192772122,-3.76755250522518,-0.723012177543099));
#34658=CARTESIAN_POINT('Ctrl Pts',(165.591039788021,-1.45643856557843,-3.54908230296227));
#34659=CARTESIAN_POINT('Ctrl Pts',(165.748886803919,2.17362861751428,-3.16109745525618));
#34660=CARTESIAN_POINT('Ctrl Pts',(165.906733819818,3.83525402566757,0.0895826272489707));
#34661=CARTESIAN_POINT('Ctrl Pts',(166.064580835716,2.02366686162806,3.25913653007244));
#34662=CARTESIAN_POINT('Ctrl Pts',(166.222427851615,-1.62055645602664,3.47721084510769));
#34663=CARTESIAN_POINT('Ctrl Pts',(166.380274867513,-3.79720108936192,0.546317101556261));
#34664=CARTESIAN_POINT('Ctrl Pts',(166.538121883412,-2.53509395437843,-2.87932233884608));
#34665=CARTESIAN_POINT('Ctrl Pts',(166.69596889931,1.0227985797233,-3.69744256937415));
#34666=CARTESIAN_POINT('Ctrl Pts',(166.853815915209,3.65444297950556,-1.16715251704597));
#34667=CARTESIAN_POINT('Ctrl Pts',(167.011662931107,2.97661759819002,2.42011284089185));
#34668=CARTESIAN_POINT('Ctrl Pts',(167.169509947005,-0.396837745431416,
3.81571989175109));
#34669=CARTESIAN_POINT('Ctrl Pts',(167.327356962904,-3.41091615148145,1.75580451533406));
#34670=CARTESIAN_POINT('Ctrl Pts',(167.485203978802,-3.33606308630793,-1.89417041806629));
#34671=CARTESIAN_POINT('Ctrl Pts',(167.643050994701,-0.240065613111764,
-3.8287813975082));
#34672=CARTESIAN_POINT('Ctrl Pts',(167.800898010599,3.07333568784469,-2.29604142783338));
#34673=CARTESIAN_POINT('Ctrl Pts',(167.958745026498,3.60351895991518,1.31599756611942));
#34674=CARTESIAN_POINT('Ctrl Pts',(168.116592042396,0.870349329689956,3.73626692472705));
#34675=CARTESIAN_POINT('Ctrl Pts',(168.274439058294,-2.65101013460254,2.77296659820502));
#34676=CARTESIAN_POINT('Ctrl Pts',(168.432286074193,-3.77161030969884,-0.701536998483682));
#34677=CARTESIAN_POINT('Ctrl Pts',(168.590133090091,-1.47663377010695,-3.54072749551193));
#34678=CARTESIAN_POINT('Ctrl Pts',(168.74798010599,2.15558482455746,-3.17342914728068));
#34679=CARTESIAN_POINT('Ctrl Pts',(168.905827121888,3.83570213381125,0.0677320370748901));
#34680=CARTESIAN_POINT('Ctrl Pts',(169.063674137787,2.04220106353329,3.24755497330779));
#34681=CARTESIAN_POINT('Ctrl Pts',(169.221521153685,-1.60072076546566,3.48638659944164));
#34682=CARTESIAN_POINT('Ctrl Pts',(169.379368169583,-3.79402714462485,0.567940587896798));
#34683=CARTESIAN_POINT('Ctrl Pts',(169.537215185482,-2.55145608652828,-2.86483338581374));
#34684=CARTESIAN_POINT('Ctrl Pts',(169.69506220138,1.00171794804823,-3.70320937161189));
#34685=CARTESIAN_POINT('Ctrl Pts',(169.852909217279,3.64773449888311,-1.18795264572487));
#34686=CARTESIAN_POINT('Ctrl Pts',(170.010756233177,2.99035649087939,2.40311601182154));
#34687=CARTESIAN_POINT('Ctrl Pts',(170.168603249076,-0.375093465835755,
3.81791873149687));
#34688=CARTESIAN_POINT('Ctrl Pts',(170.326450264974,-3.40085809752068,1.77520772687968));
#34689=CARTESIAN_POINT('Ctrl Pts',(170.484297280873,-3.34679993780318,-1.87513436761779));
#34690=CARTESIAN_POINT('Ctrl Pts',(170.642144296771,-0.26187387915984,-3.82735168583548));
#34691=CARTESIAN_POINT('Ctrl Pts',(170.79999131267,3.06020524653171,-2.31351260623673));
#34692=CARTESIAN_POINT('Ctrl Pts',(170.957838328568,3.61095802796753,1.29544702639075));
#34693=CARTESIAN_POINT('Ctrl Pts',(171.115685344466,0.891619589961043,3.73124843598334));
#34694=CARTESIAN_POINT('Ctrl Pts',(171.273532360365,-2.63516806639073,2.78802327854887));
#34695=CARTESIAN_POINT('Ctrl Pts',(171.431379376263,-3.77554909875469,-0.680037202915507));
#34696=CARTESIAN_POINT('Ctrl Pts',(171.589226392161,-1.49677419444651,-3.53226150741033));
#34697=CARTESIAN_POINT('Ctrl Pts',(171.74707340806,2.13745721835565,-3.18565029942849));
#34698=CARTESIAN_POINT('Ctrl Pts',(171.904920423959,3.83605374689803,0.0458640011606042));
#34699=CARTESIAN_POINT('Ctrl Pts',(172.062767439857,2.06061241993342,3.2358988269467));
#34700=CARTESIAN_POINT('Ctrl Pts',(172.220614455755,-1.58071882214594,3.49538694441449));
#34701=CARTESIAN_POINT('Ctrl Pts',(172.378461471654,-3.79096103253289,0.589671448752604));
#34702=CARTESIAN_POINT('Ctrl Pts',(172.536308487552,-2.5672686636252,-2.85050572088963));
#34703=CARTESIAN_POINT('Ctrl Pts',(172.694155503451,0.979661184699643,-3.7083415343505));
#34704=CARTESIAN_POINT('Ctrl Pts',(172.852002519349,3.64282177600219,-1.20976586808304));
#34705=CARTESIAN_POINT('Ctrl Pts',(173.009849535247,3.00003709933762,2.38826653740653));
#34706=CARTESIAN_POINT('Ctrl Pts',(173.11508087918,0.77100113749699,3.33719695292788));
#34707=CARTESIAN_POINT('Ctrl Pts',(173.167696551146,-0.29952085450997,3.23817715045265));
#34708=CARTESIAN_POINT('Ctrl Pts',(156.861303448854,1.77778008111438,-2.49305876047737));
#34709=CARTESIAN_POINT('Ctrl Pts',(156.91391912082,2.60197039142016,-1.90533530207459));
#34710=CARTESIAN_POINT('Ctrl Pts',(157.019150464753,3.60775223845264,0.142028800872616));
#34711=CARTESIAN_POINT('Ctrl Pts',(157.176997480651,1.8534282716387,3.10276224581075));
#34712=CARTESIAN_POINT('Ctrl Pts',(157.334844496549,-1.5819617313493,3.24655028783993));
#34713=CARTESIAN_POINT('Ctrl Pts',(157.492691512448,-3.58343987819263,0.453688641335127));
#34714=CARTESIAN_POINT('Ctrl Pts',(157.650538528346,-2.34038562704942,-2.7517255764358));
#34715=CARTESIAN_POINT('Ctrl Pts',(157.808385544245,1.02244103607846,-3.46433581143144));
#34716=CARTESIAN_POINT('Ctrl Pts',(157.966232560143,3.45918736354465,-1.0400516376856));
#34717=CARTESIAN_POINT('Ctrl Pts',(158.124079576042,2.76336492665527,2.32630994710626));
#34718=CARTESIAN_POINT('Ctrl Pts',(158.28192659194,-0.435003694578273,3.5858598946312));
#34719=CARTESIAN_POINT('Ctrl Pts',(158.439773607838,-3.23941332311708,1.59809919576479));
#34720=CARTESIAN_POINT('Ctrl Pts',(158.597620623737,-3.11021409020853,-1.83692768569907));
#34721=CARTESIAN_POINT('Ctrl Pts',(158.755467639635,-0.164395054080841,
-3.60841744042984));
#34722=CARTESIAN_POINT('Ctrl Pts',(158.913314655534,2.93029813127553,-2.1121243019941));
#34723=CARTESIAN_POINT('Ctrl Pts',(159.071161671432,3.37130947641095,1.29691520817138));
#34724=CARTESIAN_POINT('Ctrl Pts',(159.229008687331,0.759256661457781,3.5314646094309));
#34725=CARTESIAN_POINT('Ctrl Pts',(159.386855703229,-2.54038000042538,2.56791438788198));
#34726=CARTESIAN_POINT('Ctrl Pts',(159.544702719127,-3.53944434833963,-0.721143837982535));
#34727=CARTESIAN_POINT('Ctrl Pts',(159.702549735026,-1.33318180321698,-3.35713279646557));
#34728=CARTESIAN_POINT('Ctrl Pts',(159.860396750924,2.08041241794654,-2.9528966708862));
#34729=CARTESIAN_POINT('Ctrl Pts',(160.018243766823,3.60998162978598,0.125487749076156));
#34730=CARTESIAN_POINT('Ctrl Pts',(160.176090782721,1.87034532625072,3.09023022805079));
#34731=CARTESIAN_POINT('Ctrl Pts',(160.33393779862,-1.56307888347109,3.2564549646075));
#34732=CARTESIAN_POINT('Ctrl Pts',(160.491784814518,-3.58097619840984,0.473628538266046));
#34733=CARTESIAN_POINT('Ctrl Pts',(160.649631830416,-2.35593537323219,-2.73811669566301));
#34734=CARTESIAN_POINT('Ctrl Pts',(160.807478846315,1.00264453460455,-3.47021879178988));
#34735=CARTESIAN_POINT('Ctrl Pts',(160.965325862213,3.45322784592268,-1.05968484406379));
#34736=CARTESIAN_POINT('Ctrl Pts',(161.123172878112,2.77656214340745,2.31050150141743));
#34737=CARTESIAN_POINT('Ctrl Pts',(161.28101989401,-0.414562961063291,3.58829375553555));
#34738=CARTESIAN_POINT('Ctrl Pts',(161.438866909909,-3.23025914255255,1.61652107827222));
#34739=CARTESIAN_POINT('Ctrl Pts',(161.596713925807,-3.1206271475183,-1.81917583831006));
#34740=CARTESIAN_POINT('Ctrl Pts',(161.754560941706,-0.184949897249031,
-3.60742402000075));
#34741=CARTESIAN_POINT('Ctrl Pts',(161.912407957604,2.91821829470645,-2.12878287032501));
#34742=CARTESIAN_POINT('Ctrl Pts',(162.070254973503,3.37864303296851,1.27768766931568));
#34743=CARTESIAN_POINT('Ctrl Pts',(162.228101989401,0.77936289105334,3.52708208135319));
#34744=CARTESIAN_POINT('Ctrl Pts',(162.3859490053,-2.52570961126161,2.5823449583918));
#34745=CARTESIAN_POINT('Ctrl Pts',(162.543796021198,-3.54349519155426,-0.700968153330012));
#34746=CARTESIAN_POINT('Ctrl Pts',(162.701643037096,-1.35228549632057,-3.3494833125413));
#34747=CARTESIAN_POINT('Ctrl Pts',(162.859490052995,2.06355624559932,-2.96470068401505));
#34748=CARTESIAN_POINT('Ctrl Pts',(163.017337068893,3.61063793989887,0.104919929060897));
#34749=CARTESIAN_POINT('Ctrl Pts',(163.175184084792,1.88791977151261,3.07952487583444));
#34750=CARTESIAN_POINT('Ctrl Pts',(163.33303110069,-1.54450175467604,3.26530685454736));
#34751=CARTESIAN_POINT('Ctrl Pts',(163.490878116589,-3.57821986351258,0.494021389127376));
#34752=CARTESIAN_POINT('Ctrl Pts',(163.648725132487,-2.37149597480538,-2.72465068697498));
#34753=CARTESIAN_POINT('Ctrl Pts',(163.806572148385,0.982858704319936,-3.47587446434618));
#34754=CARTESIAN_POINT('Ctrl Pts',(163.964419164284,3.44713486825773,-1.07934041182248));
#34755=CARTESIAN_POINT('Ctrl Pts',(164.122266180182,2.78967982942521,2.29464615438841));
#34756=CARTESIAN_POINT('Ctrl Pts',(164.280113196081,-0.394114010203119,
3.59059725832805));
#34757=CARTESIAN_POINT('Ctrl Pts',(164.437960211979,-3.22099753151778,1.63489737491615));
#34758=CARTESIAN_POINT('Ctrl Pts',(164.595807227878,-3.13094020703742,-1.80136835336581));
#34759=CARTESIAN_POINT('Ctrl Pts',(164.753654243776,-0.205498103064254,
-3.60631183540585));
#34760=CARTESIAN_POINT('Ctrl Pts',(164.911501259675,2.90604343274518,-2.14537318235079));
#34761=CARTESIAN_POINT('Ctrl Pts',(165.069348275573,3.38586709057337,1.25841907547666));
#34762=CARTESIAN_POINT('Ctrl Pts',(165.227195291471,0.799443749363122,3.52258487706905));
#34763=CARTESIAN_POINT('Ctrl Pts',(165.38504230737,-2.51095721170392,2.59669181951641));
#34764=CARTESIAN_POINT('Ctrl Pts',(165.542889323268,-3.54743104889283,-0.680769768646074));
#34765=CARTESIAN_POINT('Ctrl Pts',(165.700736339167,-1.37134529145175,-3.34172509583964));
#34766=CARTESIAN_POINT('Ctrl Pts',(165.858583355065,2.04663309558081,-2.97640848954317));
#34767=CARTESIAN_POINT('Ctrl Pts',(166.016430370964,3.61117706844838,0.0843487099127957));
#34768=CARTESIAN_POINT('Ctrl Pts',(166.174277386862,1.90543294289823,3.06871957413341));
#34769=CARTESIAN_POINT('Ctrl Pts',(166.332124402761,-1.52587449826372,3.27405276990151));
#34770=CARTESIAN_POINT('Ctrl Pts',(166.489971418659,-3.57534739717903,0.514398205708856));
#34771=CARTESIAN_POINT('Ctrl Pts',(166.647818434558,-2.3869796089504,-2.71109624893811));
#34772=CARTESIAN_POINT('Ctrl Pts',(166.805665450456,0.963040975126942,-3.48141732700604));
#34773=CARTESIAN_POINT('Ctrl Pts',(166.963512466355,3.44093001329829,-1.09896094932186));
#34774=CARTESIAN_POINT('Ctrl Pts',(167.121359482253,2.80270697590953,2.27871633419769));
#34775=CARTESIAN_POINT('Ctrl Pts',(167.279206498151,-0.373652268299834,
3.5927842277189));
#34776=CARTESIAN_POINT('Ctrl Pts',(167.43705351405,-3.21163138248347,1.6532206106866));
#34777=CARTESIAN_POINT('Ctrl Pts',(167.594900529948,-3.14115165137603,-1.78350240471065));
#34778=CARTESIAN_POINT('Ctrl Pts',(167.752747545847,-0.226039639405949,
-3.60508260737089));
#34779=CARTESIAN_POINT('Ctrl Pts',(167.910594561745,2.89377425466804,-2.16189386593658));
#34780=CARTESIAN_POINT('Ctrl Pts',(168.068441577644,3.39298125930512,1.23910963943965));
#34781=CARTESIAN_POINT('Ctrl Pts',(168.226288593542,0.819498661596119,3.5179733467141));
#34782=CARTESIAN_POINT('Ctrl Pts',(168.38413560944,-2.49612331862024,2.61095440458294));
#34783=CARTESIAN_POINT('Ctrl Pts',(168.541982625339,-3.55125177376932,-0.660549289470204));
#34784=CARTESIAN_POINT('Ctrl Pts',(168.699829641237,-1.39036057935652,-3.33385842289593));
#34785=CARTESIAN_POINT('Ctrl Pts',(168.857676657136,2.02964352176968,-2.98801969525627));
#34786=CARTESIAN_POINT('Ctrl Pts',(169.015523673034,3.61159899561195,0.0637747532359756));
#34787=CARTESIAN_POINT('Ctrl Pts',(169.173370688933,1.92288427322844,3.05781467658932));
#34788=CARTESIAN_POINT('Ctrl Pts',(169.331217704831,-1.50719771951289,3.28269242542751));
#34789=CARTESIAN_POINT('Ctrl Pts',(169.48906472073,-3.57235889201762,0.5347583272263));
#34790=CARTESIAN_POINT('Ctrl Pts',(169.646911736628,-2.40238577396973,-2.69745382145195));
#34791=CARTESIAN_POINT('Ctrl Pts',(169.804758752526,0.943191991673975,-3.48684720045375));
#34792=CARTESIAN_POINT('Ctrl Pts',(169.962605768425,3.43461347957567,-1.1185458183301));
#34793=CARTESIAN_POINT('Ctrl Pts',(170.120452784323,2.8156431657665,2.26271255479631));
#34794=CARTESIAN_POINT('Ctrl Pts',(170.278299800222,-0.353178410943777,
3.59485459896784));
#34795=CARTESIAN_POINT('Ctrl Pts',(170.43614681612,-3.20216097620183,1.67149017826124));
#34796=CARTESIAN_POINT('Ctrl Pts',(170.593993832019,-3.15126119604961,-1.76557854663153));
#34797=CARTESIAN_POINT('Ctrl Pts',(170.751840847917,-0.24657374476856,-3.60373642743796));
#34798=CARTESIAN_POINT('Ctrl Pts',(170.909687863816,2.88141096706031,-2.17834428053408));
#34799=CARTESIAN_POINT('Ctrl Pts',(171.067534879714,3.3999856954602,1.2197597770014));
#34800=CARTESIAN_POINT('Ctrl Pts',(171.225381895613,0.839526194483593,3.51324806610732));
#34801=CARTESIAN_POINT('Ctrl Pts',(171.383228911511,-2.48120683249953,2.62513138958075));
#34802=CARTESIAN_POINT('Ctrl Pts',(171.541075927409,-3.55496043677332,-0.640305632019483));
#34803=CARTESIAN_POINT('Ctrl Pts',(171.698922943308,-1.40932428763688,-3.32588706509546));
#34804=CARTESIAN_POINT('Ctrl Pts',(171.856769959206,2.01257503155137,-2.99952681944957));
#34805=CARTESIAN_POINT('Ctrl Pts',(172.014616975104,3.61193006549869,0.0431843700965086));
#34806=CARTESIAN_POINT('Ctrl Pts',(172.172463991003,1.94021993537395,3.04683954738956));
#34807=CARTESIAN_POINT('Ctrl Pts',(172.330311006901,-1.48836440141788,3.29116691998682));
#34808=CARTESIAN_POINT('Ctrl Pts',(172.4881580228,-3.56947191931603,0.555219549840223));
#34809=CARTESIAN_POINT('Ctrl Pts',(172.646005038698,-2.41727449201117,-2.68396325872204));
#34810=CARTESIAN_POINT('Ctrl Pts',(172.803852054597,0.922423907610818,-3.49167951358586));
#34811=CARTESIAN_POINT('Ctrl Pts',(172.961699070495,3.42998778539936,-1.13908459042749));
#34812=CARTESIAN_POINT('Ctrl Pts',(173.119546086394,2.82475817901961,2.2487306695999));
#34813=CARTESIAN_POINT('Ctrl Pts',(173.224777430326,0.725954945576791,3.14221927117626));
#34814=CARTESIAN_POINT('Ctrl Pts',(173.277393102292,-0.282021173588434,
3.04898475851353));
#34815=CARTESIAN_POINT('Ctrl Pts',(156.971,1.66746714335746,-2.33836210323023));
#34816=CARTESIAN_POINT('Ctrl Pts',(157.023615671966,2.44051566432356,-1.78710744205035));
#34817=CARTESIAN_POINT('Ctrl Pts',(157.128847015899,3.38388779517831,0.133215779263953));
#34818=CARTESIAN_POINT('Ctrl Pts',(157.286694031797,1.73842129201381,2.91023290985255));
#34819=CARTESIAN_POINT('Ctrl Pts',(157.444541047695,-1.48379950765357,3.04509876769309));
#34820=CARTESIAN_POINT('Ctrl Pts',(157.602388063594,-3.36108403989851,0.425536831454739));
#34821=CARTESIAN_POINT('Ctrl Pts',(157.760235079492,-2.19516248232719,-2.58097839827683));
#34822=CARTESIAN_POINT('Ctrl Pts',(157.918082095391,0.958997601442651,-3.24937049328252));
#34823=CARTESIAN_POINT('Ctrl Pts',(158.075929111289,3.24454151146318,-0.97551544854114));
#34824=CARTESIAN_POINT('Ctrl Pts',(158.233776127188,2.5918955157916,2.18196021165553));
#34825=CARTESIAN_POINT('Ctrl Pts',(158.391623143086,-0.408011303340585,
3.36335389202508));
#34826=CARTESIAN_POINT('Ctrl Pts',(158.549470158985,-3.03840465839069,1.49893562711835));
#34827=CARTESIAN_POINT('Ctrl Pts',(158.707317174883,-2.91722236024783,-1.72294458305937));
#34828=CARTESIAN_POINT('Ctrl Pts',(158.865164190781,-0.154194185277631,
-3.38451172074282));
#34829=CARTESIAN_POINT('Ctrl Pts',(159.02301120668,2.74847035696387,-1.98106498867635));
#34830=CARTESIAN_POINT('Ctrl Pts',(159.180858222578,3.16211653045467,1.21644039120453));
#34831=CARTESIAN_POINT('Ctrl Pts',(159.338705238477,0.71214406652733,3.31233388578888));
#34832=CARTESIAN_POINT('Ctrl Pts',(159.496552254375,-2.38274701542186,2.40857286805911));
#34833=CARTESIAN_POINT('Ctrl Pts',(159.654399270273,-3.31981847434075,-0.676396179845171));
#34834=CARTESIAN_POINT('Ctrl Pts',(159.812246286172,-1.25045660967965,-3.14881952692657));
#34835=CARTESIAN_POINT('Ctrl Pts',(159.97009330207,1.9513208570681,-2.76966663578875));
#34836=CARTESIAN_POINT('Ctrl Pts',(160.127940317969,3.38597885066797,0.117701115397386));
#34837=CARTESIAN_POINT('Ctrl Pts',(160.285787333867,1.75428862736512,2.89847851566358));
#34838=CARTESIAN_POINT('Ctrl Pts',(160.443634349766,-1.46608835837003,3.05438884988658));
#34839=CARTESIAN_POINT('Ctrl Pts',(160.601481365664,-3.35877323377958,0.444239438896151));
#34840=CARTESIAN_POINT('Ctrl Pts',(160.759328381563,-2.20974735203226,-2.56821396144488));
#34841=CARTESIAN_POINT('Ctrl Pts',(160.917175397461,0.940429491634335,-3.25488842913799));
#34842=CARTESIAN_POINT('Ctrl Pts',(161.075022413359,3.23895178755388,-0.993930395869087));
#34843=CARTESIAN_POINT('Ctrl Pts',(161.232869429258,2.60427383274531,2.16713269499377));
#34844=CARTESIAN_POINT('Ctrl Pts',(161.390716445156,-0.388838936699488,
3.36563672955522));
#34845=CARTESIAN_POINT('Ctrl Pts',(161.548563461055,-3.02981850340005,1.51621441436896));
#34846=CARTESIAN_POINT('Ctrl Pts',(161.706410476953,-2.9269892774894,-1.70629425461351));
#34847=CARTESIAN_POINT('Ctrl Pts',(161.864257492852,-0.173473580959878,
-3.38357994299221));
#34848=CARTESIAN_POINT('Ctrl Pts',(162.02210450875,2.73714008569463,-1.99668987706511));
#34849=CARTESIAN_POINT('Ctrl Pts',(162.179951524649,3.16899503288228,1.1984059393451));
#34850=CARTESIAN_POINT('Ctrl Pts',(162.337798540547,0.731002685534005,3.30822329772906));
#34851=CARTESIAN_POINT('Ctrl Pts',(162.495645556446,-2.36898693779993,2.4221080080017));
#34852=CARTESIAN_POINT('Ctrl Pts',(162.653492572344,-3.32361795889739,-0.657472415533592));
#34853=CARTESIAN_POINT('Ctrl Pts',(162.811339588242,-1.26837490053319,-3.14164470072457));
#34854=CARTESIAN_POINT('Ctrl Pts',(162.969186604141,1.9355106261794,-2.78073819872344));
#34855=CARTESIAN_POINT('Ctrl Pts',(163.127033620039,3.38659443611677,0.0984095480937175));
#34856=CARTESIAN_POINT('Ctrl Pts',(163.284880635938,1.77077256165387,2.88843744069124));
#34857=CARTESIAN_POINT('Ctrl Pts',(163.442727651836,-1.44866395801099,3.0626914716721));
#34858=CARTESIAN_POINT('Ctrl Pts',(163.600574667735,-3.3561879320732,0.463366894047598));
#34859=CARTESIAN_POINT('Ctrl Pts',(163.758421683633,-2.22434240354049,-2.55558353134951));
#34860=CARTESIAN_POINT('Ctrl Pts',(163.916268699531,0.921871390857911,-3.26019316185573));
#34861=CARTESIAN_POINT('Ctrl Pts',(164.07411571543,3.23323688492365,-1.01236631703268));
#34862=CARTESIAN_POINT('Ctrl Pts',(164.231962731328,2.61657755392199,2.15226118726438));
#34863=CARTESIAN_POINT('Ctrl Pts',(164.389809747227,-0.369658862607259,
3.36779729781782));
#34864=CARTESIAN_POINT('Ctrl Pts',(164.547656763125,-3.0211315841016,1.53345044440206));
#34865=CARTESIAN_POINT('Ctrl Pts',(164.705503779024,-2.93666240189792,-1.6895917409754));
#34866=CARTESIAN_POINT('Ctrl Pts',(164.863350794922,-0.192746751143198,
-3.38253677050477));
#34867=CARTESIAN_POINT('Ctrl Pts',(165.021197810821,2.72572068544879,-2.01225074451711));
#34868=CARTESIAN_POINT('Ctrl Pts',(165.179044826719,3.1757708308709,1.18033298000295));
#34869=CARTESIAN_POINT('Ctrl Pts',(165.336891842617,0.749837507567218,3.30400514923002));
#34870=CARTESIAN_POINT('Ctrl Pts',(165.494738858516,-2.35514993860669,2.43556463280571));
#34871=CARTESIAN_POINT('Ctrl Pts',(165.652585874414,-3.32730959256048,-0.638527359749053));
#34872=CARTESIAN_POINT('Ctrl Pts',(165.810432890313,-1.28625201732507,-3.13436788871701));
#34873=CARTESIAN_POINT('Ctrl Pts',(165.968279906211,1.91963757364734,-2.79171952383016));
#34874=CARTESIAN_POINT('Ctrl Pts',(166.12612692211,3.38710011122917,0.0791147925766244));
#34875=CARTESIAN_POINT('Ctrl Pts',(166.283973938008,1.78719902416841,2.87830261819438));
#34876=CARTESIAN_POINT('Ctrl Pts',(166.441820953907,-1.43119254050081,3.07089469469534));
#34877=CARTESIAN_POINT('Ctrl Pts',(166.599667969805,-3.35349370499614,0.482479309861451));
#34878=CARTESIAN_POINT('Ctrl Pts',(166.757514985703,-2.23886526352237,-2.54287015903015));
#34879=CARTESIAN_POINT('Ctrl Pts',(166.915362001602,0.903283370530585,-3.26539208463793));
#34880=CARTESIAN_POINT('Ctrl Pts',(167.0732090175,3.22741704709102,-1.03076938159775));
#34881=CARTESIAN_POINT('Ctrl Pts',(167.231056033399,2.62879635362904,2.13731982750353));
#34882=CARTESIAN_POINT('Ctrl Pts',(167.388903049297,-0.350466791168255,
3.36984856368669));
#34883=CARTESIAN_POINT('Ctrl Pts',(167.546750065196,-3.01234661348548,1.55063670603914));
#34884=CARTESIAN_POINT('Ctrl Pts',(167.704597081094,-2.94624021644413,-1.67283439135501));
#34885=CARTESIAN_POINT('Ctrl Pts',(167.862444096993,-0.212013665700137,
-3.38138381723357));
#34886=CARTESIAN_POINT('Ctrl Pts',(168.020291112891,2.7142128214914,-2.02774630403978));
#34887=CARTESIAN_POINT('Ctrl Pts',(168.17813812879,3.18244355869507,1.16222171275988));
#34888=CARTESIAN_POINT('Ctrl Pts',(168.335985144688,0.76864799350228,3.29967976870115));
#34889=CARTESIAN_POINT('Ctrl Pts',(168.493832160587,-2.34123650263794,2.44894221096086));
#34890=CARTESIAN_POINT('Ctrl Pts',(168.651679176485,-3.3308932378398,-0.619561580456727));
#34891=CARTESIAN_POINT('Ctrl Pts',(168.809526192383,-1.30408738860609,-3.12698935027992));
#34892=CARTESIAN_POINT('Ctrl Pts',(168.967373208282,1.9037022189819,-2.80261024323187));
#34893=CARTESIAN_POINT('Ctrl Pts',(169.12522022418,3.38749585741264,0.0598174693970574));
#34894=CARTESIAN_POINT('Ctrl Pts',(169.283067240079,1.80356748292359,2.86807437987086));
#34895=CARTESIAN_POINT('Ctrl Pts',(169.440914255977,-1.41367467356012,3.07899825141338));
#34896=CARTESIAN_POINT('Ctrl Pts',(169.598761271876,-3.35069063941039,0.5015760665558));
#34897=CARTESIAN_POINT('Ctrl Pts',(169.756608287774,-2.25331546141117,-2.53007425709015));
#34898=CARTESIAN_POINT('Ctrl Pts',(169.914455303673,0.884666035299711,-3.27048502929561));
#34899=CARTESIAN_POINT('Ctrl Pts',(170.072302319571,3.22149246026824,-1.04913899093533));
#34900=CARTESIAN_POINT('Ctrl Pts',(170.230149335469,2.64092984065361,2.12230909777109));
#34901=CARTESIAN_POINT('Ctrl Pts',(170.387996351368,-0.331263356051794,
3.37179046643881));
#34902=CARTESIAN_POINT('Ctrl Pts',(170.545843367266,-3.00346385488298,1.56777262964278));
#34903=CARTESIAN_POINT('Ctrl Pts',(170.703690383165,-2.95572245429602,-1.65602272564527));
#34904=CARTESIAN_POINT('Ctrl Pts',(170.861537399063,-0.231273610377281,
-3.38012116904044));
#34905=CARTESIAN_POINT('Ctrl Pts',(171.019384414961,2.70261668758891,-2.04317595483142));
#34906=CARTESIAN_POINT('Ctrl Pts',(171.17723143086,3.18901336295286,1.14407252761205));
#34907=CARTESIAN_POINT('Ctrl Pts',(171.335078446758,0.787432799006144,3.2952476962313));
#34908=CARTESIAN_POINT('Ctrl Pts',(171.492925462657,-2.32724559860833,2.46223950061263));
#34909=CARTESIAN_POINT('Ctrl Pts',(171.650772478555,-3.33437177479195,-0.600574061123454));
#34910=CARTESIAN_POINT('Ctrl Pts',(171.808619494454,-1.32187438082726,-3.1195126227806));
#34911=CARTESIAN_POINT('Ctrl Pts',(171.966466510352,1.88769284474709,-2.81340333947064));
#34912=CARTESIAN_POINT('Ctrl Pts',(172.124313526251,3.38780638409936,0.0405047390324093));
#34913=CARTESIAN_POINT('Ctrl Pts',(172.282160542149,1.81982745081448,2.85778026783241));
#34914=CARTESIAN_POINT('Ctrl Pts',(172.440007558048,-1.39600998068982,3.08694689555915));
#34915=CARTESIAN_POINT('Ctrl Pts',(172.597854573946,-3.34798280609916,0.520767650927842));
#34916=CARTESIAN_POINT('Ctrl Pts',(172.755701589844,-2.26728032039713,-2.51742079655446));
#34917=CARTESIAN_POINT('Ctrl Pts',(172.913548605743,0.865186630521988,-3.27501749282122));
#34918=CARTESIAN_POINT('Ctrl Pts',(173.071395621641,3.21715379479654,-1.06840331277194));
#34919=CARTESIAN_POINT('Ctrl Pts',(173.22924263754,2.64947925870158,2.10919480179326));
#34920=CARTESIAN_POINT('Ctrl Pts',(173.334473981472,0.680908753656591,2.94724158942463));
#34921=CARTESIAN_POINT('Ctrl Pts',(173.387089653438,-0.264521492666898,
2.85979236657441));
#34922=CARTESIAN_POINT('Ctrl Pts',(173.058,-0.317020535431409,3.42736954239177));
#34923=CARTESIAN_POINT('Ctrl Pts',(173.005384328034,0.816047329417257,3.53217463467948));
#34924=CARTESIAN_POINT('Ctrl Pts',(172.952768656068,1.99568167453643,3.02998851994632));
#34925=CARTESIAN_POINT('Ctrl Pts',(172.900152984102,2.69888880492091,2.14418720408781));
#34926=CARTESIAN_POINT('Ctrl Pts',(172.847537312136,3.40209593530543,1.25838588822926));
#34927=CARTESIAN_POINT('Ctrl Pts',(172.794921640169,3.62887585095523,-0.0110306287547288));
#34928=CARTESIAN_POINT('Ctrl Pts',(172.742305968203,3.27247292464401,-1.08649828880944));
#34929=CARTESIAN_POINT('Ctrl Pts',(172.689690296237,2.9160699983328,-2.16196594886414));
#34930=CARTESIAN_POINT('Ctrl Pts',(172.637074624271,1.97648423006066,-3.04348475198962));
#34931=CARTESIAN_POINT('Ctrl Pts',(172.584458952305,0.880997796419955,-3.33291825820939));
#34932=CARTESIAN_POINT('Ctrl Pts',(172.531843280339,-0.214488637220761,
-3.62235176442917));
#34933=CARTESIAN_POINT('Ctrl Pts',(172.479227608372,-1.46587573623001,-3.31969997374319));
#34934=CARTESIAN_POINT('Ctrl Pts',(172.426611936406,-2.30743383748638,-2.56151215661316));
#34935=CARTESIAN_POINT('Ctrl Pts',(172.38218144249,-3.01807461619349,-1.92127213044367));
#34936=CARTESIAN_POINT('Ctrl Pts',(172.337750948573,-3.43647871595114,-0.956203123797524));
#34937=CARTESIAN_POINT('Ctrl Pts',(172.293320454657,-3.44466766225695,0.00262740410212479));
#34938=CARTESIAN_POINT('Origin',(36.8,37.284736894758,-9.99041514095732));
#34939=CARTESIAN_POINT('Ctrl Pts',(36.8,31.4347259190859,-4.53355051147316));
#34940=CARTESIAN_POINT('Ctrl Pts',(36.8,31.1968691126063,-6.18280168905533));
#34941=CARTESIAN_POINT('Ctrl Pts',(36.8,30.8293258095436,-7.81258162569767));
#34942=CARTESIAN_POINT('Ctrl Pts',(36.8,30.0846548283827,-10.2137688485759));
#34943=CARTESIAN_POINT('Ctrl Pts',(36.8,29.8028301128151,-11.0089139056503));
#34944=CARTESIAN_POINT('Ctrl Pts',(36.8,29.4900464626661,-11.7911930472673));
#34945=CARTESIAN_POINT('Ctrl Pts',(37.5,32.4,0.));
#34946=CARTESIAN_POINT('Ctrl Pts',(37.5,32.4,32.4));
#34947=CARTESIAN_POINT('Ctrl Pts',(37.5,0.,32.4));
#34948=CARTESIAN_POINT('Ctrl Pts',(37.5,-32.4,32.4));
#34949=CARTESIAN_POINT('Ctrl Pts',(37.5,-32.4,0.));
#34950=CARTESIAN_POINT('Ctrl Pts',(37.5,-32.4,-32.4));
#34951=CARTESIAN_POINT('Ctrl Pts',(37.5,0.,-32.4));
#34952=CARTESIAN_POINT('Ctrl Pts',(37.5,32.4,-32.4));
#34953=CARTESIAN_POINT('Ctrl Pts',(37.5,32.4,0.));
#34954=CARTESIAN_POINT('Ctrl Pts',(37.3389083940589,32.2580145365138,0.));
#34955=CARTESIAN_POINT('Ctrl Pts',(37.3389083940589,32.2580145365137,32.2580145365137));
#34956=CARTESIAN_POINT('Ctrl Pts',(37.3389083940589,0.,32.2580145365138));
#34957=CARTESIAN_POINT('Ctrl Pts',(37.3389083940589,-32.2580145365137,32.2580145365137));
#34958=CARTESIAN_POINT('Ctrl Pts',(37.3389083940589,-32.2580145365138,0.));
#34959=CARTESIAN_POINT('Ctrl Pts',(37.3389083940589,-32.2580145365137,-32.2580145365137));
#34960=CARTESIAN_POINT('Ctrl Pts',(37.3389083940589,0.,-32.2580145365138));
#34961=CARTESIAN_POINT('Ctrl Pts',(37.3389083940589,32.2580145365137,-32.2580145365137));
#34962=CARTESIAN_POINT('Ctrl Pts',(37.3389083940589,32.2580145365138,0.));
#34963=CARTESIAN_POINT('Ctrl Pts',(37.0144855040189,31.9658168899962,0.));
#34964=CARTESIAN_POINT('Ctrl Pts',(37.0144855040189,31.9658168899962,31.9658168899962));
#34965=CARTESIAN_POINT('Ctrl Pts',(37.0144855040189,0.,31.9658168899962));
#34966=CARTESIAN_POINT('Ctrl Pts',(37.0144855040189,-31.9658168899962,31.9658168899962));
#34967=CARTESIAN_POINT('Ctrl Pts',(37.0144855040189,-31.9658168899962,0.));
#34968=CARTESIAN_POINT('Ctrl Pts',(37.0144855040189,-31.9658168899962,-31.9658168899962));
#34969=CARTESIAN_POINT('Ctrl Pts',(37.0144855040189,0.,-31.9658168899962));
#34970=CARTESIAN_POINT('Ctrl Pts',(37.0144855040189,31.9658168899962,-31.9658168899962));
#34971=CARTESIAN_POINT('Ctrl Pts',(37.0144855040189,31.9658168899962,0.));
#34972=CARTESIAN_POINT('Ctrl Pts',(36.5211322358012,31.5028400616267,0.));
#34973=CARTESIAN_POINT('Ctrl Pts',(36.5211322358012,31.5028400616266,31.5028400616266));
#34974=CARTESIAN_POINT('Ctrl Pts',(36.5211322358012,0.,31.5028400616267));
#34975=CARTESIAN_POINT('Ctrl Pts',(36.5211322358012,-31.5028400616266,31.5028400616266));
#34976=CARTESIAN_POINT('Ctrl Pts',(36.5211322358012,-31.5028400616267,0.));
#34977=CARTESIAN_POINT('Ctrl Pts',(36.5211322358012,-31.5028400616266,-31.5028400616266));
#34978=CARTESIAN_POINT('Ctrl Pts',(36.5211322358012,0.,-31.5028400616267));
#34979=CARTESIAN_POINT('Ctrl Pts',(36.5211322358012,31.5028400616266,-31.5028400616266));
#34980=CARTESIAN_POINT('Ctrl Pts',(36.5211322358012,31.5028400616267,0.));
#34981=CARTESIAN_POINT('Ctrl Pts',(35.849854090057,30.8360498427659,0.));
#34982=CARTESIAN_POINT('Ctrl Pts',(35.849854090057,30.8360498427659,30.8360498427659));
#34983=CARTESIAN_POINT('Ctrl Pts',(35.849854090057,0.,30.8360498427659));
#34984=CARTESIAN_POINT('Ctrl Pts',(35.849854090057,-30.8360498427659,30.8360498427659));
#34985=CARTESIAN_POINT('Ctrl Pts',(35.849854090057,-30.8360498427659,0.));
#34986=CARTESIAN_POINT('Ctrl Pts',(35.849854090057,-30.8360498427659,-30.8360498427659));
#34987=CARTESIAN_POINT('Ctrl Pts',(35.849854090057,0.,-30.8360498427659));
#34988=CARTESIAN_POINT('Ctrl Pts',(35.849854090057,30.8360498427659,-30.8360498427659));
#34989=CARTESIAN_POINT('Ctrl Pts',(35.849854090057,30.8360498427659,0.));
#34990=CARTESIAN_POINT('Ctrl Pts',(34.987601126175,29.9204750609072,0.));
#34991=CARTESIAN_POINT('Ctrl Pts',(34.987601126175,29.9204750609072,29.9204750609072));
#34992=CARTESIAN_POINT('Ctrl Pts',(34.987601126175,0.,29.9204750609072));
#34993=CARTESIAN_POINT('Ctrl Pts',(34.987601126175,-29.9204750609072,29.9204750609072));
#34994=CARTESIAN_POINT('Ctrl Pts',(34.987601126175,-29.9204750609072,0.));
#34995=CARTESIAN_POINT('Ctrl Pts',(34.987601126175,-29.9204750609072,-29.9204750609072));
#34996=CARTESIAN_POINT('Ctrl Pts',(34.987601126175,0.,-29.9204750609072));
#34997=CARTESIAN_POINT('Ctrl Pts',(34.987601126175,29.9204750609072,-29.9204750609072));
#34998=CARTESIAN_POINT('Ctrl Pts',(34.987601126175,29.9204750609072,0.));
#34999=CARTESIAN_POINT('Ctrl Pts',(34.1004337719427,28.9253475198501,0.));
#35000=CARTESIAN_POINT('Ctrl Pts',(34.1004337719427,28.9253475198501,28.9253475198501));
#35001=CARTESIAN_POINT('Ctrl Pts',(34.1004337719427,0.,28.9253475198501));
#35002=CARTESIAN_POINT('Ctrl Pts',(34.1004337719427,-28.9253475198501,28.9253475198501));
#35003=CARTESIAN_POINT('Ctrl Pts',(34.1004337719427,-28.9253475198501,0.));
#35004=CARTESIAN_POINT('Ctrl Pts',(34.1004337719427,-28.9253475198501,-28.9253475198501));
#35005=CARTESIAN_POINT('Ctrl Pts',(34.1004337719427,0.,-28.9253475198501));
#35006=CARTESIAN_POINT('Ctrl Pts',(34.1004337719427,28.9253475198501,-28.9253475198501));
#35007=CARTESIAN_POINT('Ctrl Pts',(34.1004337719427,28.9253475198501,0.));
#35008=CARTESIAN_POINT('Ctrl Pts',(33.1851263782876,27.8567138854442,0.));
#35009=CARTESIAN_POINT('Ctrl Pts',(33.1851263782876,27.8567138854442,27.8567138854442));
#35010=CARTESIAN_POINT('Ctrl Pts',(33.1851263782876,0.,27.8567138854442));
#35011=CARTESIAN_POINT('Ctrl Pts',(33.1851263782876,-27.8567138854442,27.8567138854442));
#35012=CARTESIAN_POINT('Ctrl Pts',(33.1851263782876,-27.8567138854442,0.));
#35013=CARTESIAN_POINT('Ctrl Pts',(33.1851263782876,-27.8567138854442,-27.8567138854442));
#35014=CARTESIAN_POINT('Ctrl Pts',(33.1851263782876,0.,-27.8567138854442));
#35015=CARTESIAN_POINT('Ctrl Pts',(33.1851263782876,27.8567138854442,-27.8567138854442));
#35016=CARTESIAN_POINT('Ctrl Pts',(33.1851263782876,27.8567138854442,0.));
#35017=CARTESIAN_POINT('Ctrl Pts',(32.2364640041498,26.7258152226803,0.));
#35018=CARTESIAN_POINT('Ctrl Pts',(32.2364640041498,26.7258152226803,26.7258152226803));
#35019=CARTESIAN_POINT('Ctrl Pts',(32.2364640041498,0.,26.7258152226803));
#35020=CARTESIAN_POINT('Ctrl Pts',(32.2364640041498,-26.7258152226803,26.7258152226803));
#35021=CARTESIAN_POINT('Ctrl Pts',(32.2364640041498,-26.7258152226803,0.));
#35022=CARTESIAN_POINT('Ctrl Pts',(32.2364640041498,-26.7258152226803,-26.7258152226803));
#35023=CARTESIAN_POINT('Ctrl Pts',(32.2364640041498,0.,-26.7258152226803));
#35024=CARTESIAN_POINT('Ctrl Pts',(32.2364640041498,26.7258152226803,-26.7258152226803));
#35025=CARTESIAN_POINT('Ctrl Pts',(32.2364640041498,26.7258152226803,0.));
#35026=CARTESIAN_POINT('Ctrl Pts',(31.2480536381088,25.5477500100038,0.));
#35027=CARTESIAN_POINT('Ctrl Pts',(31.2480536381088,25.5477500100038,25.5477500100038));
#35028=CARTESIAN_POINT('Ctrl Pts',(31.2480536381088,0.,25.5477500100038));
#35029=CARTESIAN_POINT('Ctrl Pts',(31.2480536381087,-25.5477500100038,25.5477500100038));
#35030=CARTESIAN_POINT('Ctrl Pts',(31.2480536381087,-25.5477500100038,0.));
#35031=CARTESIAN_POINT('Ctrl Pts',(31.2480536381087,-25.5477500100038,-25.5477500100038));
#35032=CARTESIAN_POINT('Ctrl Pts',(31.2480536381088,0.,-25.5477500100038));
#35033=CARTESIAN_POINT('Ctrl Pts',(31.2480536381088,25.5477500100038,-25.5477500100038));
#35034=CARTESIAN_POINT('Ctrl Pts',(31.2480536381088,25.5477500100038,0.));
#35035=CARTESIAN_POINT('Ctrl Pts',(30.2132710279087,24.339870673897,0.));
#35036=CARTESIAN_POINT('Ctrl Pts',(30.2132710279087,24.339870673897,24.339870673897));
#35037=CARTESIAN_POINT('Ctrl Pts',(30.2132710279087,0.,24.339870673897));
#35038=CARTESIAN_POINT('Ctrl Pts',(30.2132710279087,-24.339870673897,24.339870673897));
#35039=CARTESIAN_POINT('Ctrl Pts',(30.2132710279087,-24.339870673897,0.));
#35040=CARTESIAN_POINT('Ctrl Pts',(30.2132710279087,-24.339870673897,-24.339870673897));
#35041=CARTESIAN_POINT('Ctrl Pts',(30.2132710279087,0.,-24.339870673897));
#35042=CARTESIAN_POINT('Ctrl Pts',(30.2132710279087,24.339870673897,-24.339870673897));
#35043=CARTESIAN_POINT('Ctrl Pts',(30.2132710279087,24.339870673897,0.));
#35044=CARTESIAN_POINT('Ctrl Pts',(29.1261855002599,23.1203063432132,0.));
#35045=CARTESIAN_POINT('Ctrl Pts',(29.1261855002599,23.1203063432132,23.1203063432132));
#35046=CARTESIAN_POINT('Ctrl Pts',(29.1261855002599,0.,23.1203063432132));
#35047=CARTESIAN_POINT('Ctrl Pts',(29.1261855002599,-23.1203063432132,23.1203063432132));
#35048=CARTESIAN_POINT('Ctrl Pts',(29.1261855002599,-23.1203063432132,0.));
#35049=CARTESIAN_POINT('Ctrl Pts',(29.1261855002599,-23.1203063432132,-23.1203063432132));
#35050=CARTESIAN_POINT('Ctrl Pts',(29.1261855002599,0.,-23.1203063432132));
#35051=CARTESIAN_POINT('Ctrl Pts',(29.1261855002599,23.1203063432132,-23.1203063432132));
#35052=CARTESIAN_POINT('Ctrl Pts',(29.1261855002599,23.1203063432132,0.));
#35053=CARTESIAN_POINT('Ctrl Pts',(27.9824847998069,21.9065059385018,0.));
#35054=CARTESIAN_POINT('Ctrl Pts',(27.9824847998069,21.9065059385018,21.9065059385018));
#35055=CARTESIAN_POINT('Ctrl Pts',(27.9824847998069,0.,21.9065059385018));
#35056=CARTESIAN_POINT('Ctrl Pts',(27.9824847998069,-21.9065059385018,21.9065059385018));
#35057=CARTESIAN_POINT('Ctrl Pts',(27.9824847998069,-21.9065059385018,0.));
#35058=CARTESIAN_POINT('Ctrl Pts',(27.9824847998069,-21.9065059385018,-21.9065059385018));
#35059=CARTESIAN_POINT('Ctrl Pts',(27.9824847998069,0.,-21.9065059385018));
#35060=CARTESIAN_POINT('Ctrl Pts',(27.9824847998069,21.9065059385018,-21.9065059385018));
#35061=CARTESIAN_POINT('Ctrl Pts',(27.9824847998069,21.9065059385018,0.));
#35062=CARTESIAN_POINT('Ctrl Pts',(26.780529153894,20.7136594976185,0.));
#35063=CARTESIAN_POINT('Ctrl Pts',(26.780529153894,20.7136594976185,20.7136594976185));
#35064=CARTESIAN_POINT('Ctrl Pts',(26.780529153894,0.,20.7136594976185));
#35065=CARTESIAN_POINT('Ctrl Pts',(26.780529153894,-20.7136594976185,20.7136594976185));
#35066=CARTESIAN_POINT('Ctrl Pts',(26.780529153894,-20.7136594976185,0.));
#35067=CARTESIAN_POINT('Ctrl Pts',(26.780529153894,-20.7136594976185,-20.7136594976185));
#35068=CARTESIAN_POINT('Ctrl Pts',(26.780529153894,0.,-20.7136594976185));
#35069=CARTESIAN_POINT('Ctrl Pts',(26.780529153894,20.7136594976185,-20.7136594976185));
#35070=CARTESIAN_POINT('Ctrl Pts',(26.780529153894,20.7136594976185,0.));
#35071=CARTESIAN_POINT('Ctrl Pts',(25.5210824112439,19.5548484421686,0.));
#35072=CARTESIAN_POINT('Ctrl Pts',(25.5210824112439,19.5548484421686,19.5548484421686));
#35073=CARTESIAN_POINT('Ctrl Pts',(25.5210824112439,0.,19.5548484421686));
#35074=CARTESIAN_POINT('Ctrl Pts',(25.5210824112439,-19.5548484421686,19.5548484421686));
#35075=CARTESIAN_POINT('Ctrl Pts',(25.5210824112439,-19.5548484421686,0.));
#35076=CARTESIAN_POINT('Ctrl Pts',(25.5210824112439,-19.5548484421686,-19.5548484421686));
#35077=CARTESIAN_POINT('Ctrl Pts',(25.5210824112439,0.,-19.5548484421686));
#35078=CARTESIAN_POINT('Ctrl Pts',(25.5210824112439,19.5548484421686,-19.5548484421686));
#35079=CARTESIAN_POINT('Ctrl Pts',(25.5210824112439,19.5548484421686,0.));
#35080=CARTESIAN_POINT('Ctrl Pts',(24.2069345847179,18.4413554671298,0.));
#35081=CARTESIAN_POINT('Ctrl Pts',(24.2069345847179,18.4413554671298,18.4413554671298));
#35082=CARTESIAN_POINT('Ctrl Pts',(24.2069345847179,0.,18.4413554671298));
#35083=CARTESIAN_POINT('Ctrl Pts',(24.2069345847179,-18.4413554671298,18.4413554671298));
#35084=CARTESIAN_POINT('Ctrl Pts',(24.2069345847179,-18.4413554671298,0.));
#35085=CARTESIAN_POINT('Ctrl Pts',(24.2069345847179,-18.4413554671298,-18.4413554671298));
#35086=CARTESIAN_POINT('Ctrl Pts',(24.2069345847179,0.,-18.4413554671298));
#35087=CARTESIAN_POINT('Ctrl Pts',(24.2069345847179,18.4413554671298,-18.4413554671298));
#35088=CARTESIAN_POINT('Ctrl Pts',(24.2069345847179,18.4413554671298,0.));
#35089=CARTESIAN_POINT('Ctrl Pts',(22.8426190791586,17.3828861014748,0.));
#35090=CARTESIAN_POINT('Ctrl Pts',(22.8426190791586,17.3828861014748,17.3828861014748));
#35091=CARTESIAN_POINT('Ctrl Pts',(22.8426190791586,0.,17.3828861014748));
#35092=CARTESIAN_POINT('Ctrl Pts',(22.8426190791586,-17.3828861014748,17.3828861014748));
#35093=CARTESIAN_POINT('Ctrl Pts',(22.8426190791586,-17.3828861014748,0.));
#35094=CARTESIAN_POINT('Ctrl Pts',(22.8426190791586,-17.3828861014748,-17.3828861014748));
#35095=CARTESIAN_POINT('Ctrl Pts',(22.8426190791586,0.,-17.3828861014748));
#35096=CARTESIAN_POINT('Ctrl Pts',(22.8426190791586,17.3828861014748,-17.3828861014748));
#35097=CARTESIAN_POINT('Ctrl Pts',(22.8426190791586,17.3828861014748,0.));
#35098=CARTESIAN_POINT('Ctrl Pts',(21.4341168715413,16.3877853586665,0.));
#35099=CARTESIAN_POINT('Ctrl Pts',(21.4341168715413,16.3877853586665,16.3877853586665));
#35100=CARTESIAN_POINT('Ctrl Pts',(21.4341168715413,0.,16.3877853586665));
#35101=CARTESIAN_POINT('Ctrl Pts',(21.4341168715413,-16.3877853586665,16.3877853586665));
#35102=CARTESIAN_POINT('Ctrl Pts',(21.4341168715413,-16.3877853586665,0.));
#35103=CARTESIAN_POINT('Ctrl Pts',(21.4341168715413,-16.3877853586665,-16.3877853586665));
#35104=CARTESIAN_POINT('Ctrl Pts',(21.4341168715413,0.,-16.3877853586665));
#35105=CARTESIAN_POINT('Ctrl Pts',(21.4341168715413,16.3877853586665,-16.3877853586665));
#35106=CARTESIAN_POINT('Ctrl Pts',(21.4341168715413,16.3877853586665,0.));
#35107=CARTESIAN_POINT('Ctrl Pts',(19.9886520715334,15.4632288398589,0.));
#35108=CARTESIAN_POINT('Ctrl Pts',(19.9886520715334,15.4632288398589,15.4632288398589));
#35109=CARTESIAN_POINT('Ctrl Pts',(19.9886520715334,0.,15.4632288398589));
#35110=CARTESIAN_POINT('Ctrl Pts',(19.9886520715334,-15.4632288398589,15.4632288398589));
#35111=CARTESIAN_POINT('Ctrl Pts',(19.9886520715334,-15.4632288398589,0.));
#35112=CARTESIAN_POINT('Ctrl Pts',(19.9886520715334,-15.4632288398589,-15.4632288398589));
#35113=CARTESIAN_POINT('Ctrl Pts',(19.9886520715334,0.,-15.4632288398589));
#35114=CARTESIAN_POINT('Ctrl Pts',(19.9886520715334,15.4632288398589,-15.4632288398589));
#35115=CARTESIAN_POINT('Ctrl Pts',(19.9886520715334,15.4632288398589,0.));
#35116=CARTESIAN_POINT('Ctrl Pts',(18.514323186272,14.6153405598521,0.));
#35117=CARTESIAN_POINT('Ctrl Pts',(18.514323186272,14.6153405598521,14.6153405598521));
#35118=CARTESIAN_POINT('Ctrl Pts',(18.514323186272,0.,14.6153405598521));
#35119=CARTESIAN_POINT('Ctrl Pts',(18.514323186272,-14.6153405598521,14.6153405598521));
#35120=CARTESIAN_POINT('Ctrl Pts',(18.514323186272,-14.6153405598521,0.));
#35121=CARTESIAN_POINT('Ctrl Pts',(18.514323186272,-14.6153405598521,-14.6153405598521));
#35122=CARTESIAN_POINT('Ctrl Pts',(18.514323186272,0.,-14.6153405598521));
#35123=CARTESIAN_POINT('Ctrl Pts',(18.514323186272,14.6153405598521,-14.6153405598521));
#35124=CARTESIAN_POINT('Ctrl Pts',(18.514323186272,14.6153405598521,0.));
#35125=CARTESIAN_POINT('Ctrl Pts',(17.0194794456568,13.8492044429491,0.));
#35126=CARTESIAN_POINT('Ctrl Pts',(17.0194794456568,13.8492044429491,13.8492044429491));
#35127=CARTESIAN_POINT('Ctrl Pts',(17.0194794456568,0.,13.8492044429491));
#35128=CARTESIAN_POINT('Ctrl Pts',(17.0194794456568,-13.8492044429491,13.8492044429491));
#35129=CARTESIAN_POINT('Ctrl Pts',(17.0194794456568,-13.8492044429491,0.));
#35130=CARTESIAN_POINT('Ctrl Pts',(17.0194794456568,-13.8492044429491,-13.8492044429491));
#35131=CARTESIAN_POINT('Ctrl Pts',(17.0194794456568,0.,-13.8492044429491));
#35132=CARTESIAN_POINT('Ctrl Pts',(17.0194794456568,13.8492044429491,-13.8492044429491));
#35133=CARTESIAN_POINT('Ctrl Pts',(17.0194794456568,13.8492044429491,0.));
#35134=CARTESIAN_POINT('Ctrl Pts',(15.5121733229441,13.1688616684146,0.));
#35135=CARTESIAN_POINT('Ctrl Pts',(15.5121733229441,13.1688616684146,13.1688616684146));
#35136=CARTESIAN_POINT('Ctrl Pts',(15.5121733229441,0.,13.1688616684146));
#35137=CARTESIAN_POINT('Ctrl Pts',(15.5121733229441,-13.1688616684146,13.1688616684146));
#35138=CARTESIAN_POINT('Ctrl Pts',(15.5121733229441,-13.1688616684146,0.));
#35139=CARTESIAN_POINT('Ctrl Pts',(15.5121733229441,-13.1688616684146,-13.1688616684146));
#35140=CARTESIAN_POINT('Ctrl Pts',(15.5121733229441,0.,-13.1688616684146));
#35141=CARTESIAN_POINT('Ctrl Pts',(15.5121733229441,13.1688616684146,-13.1688616684146));
#35142=CARTESIAN_POINT('Ctrl Pts',(15.5121733229441,13.1688616684146,0.));
#35143=CARTESIAN_POINT('Ctrl Pts',(13.9995910956154,12.5772662595197,0.));
#35144=CARTESIAN_POINT('Ctrl Pts',(13.9995910956154,12.5772662595197,12.5772662595197));
#35145=CARTESIAN_POINT('Ctrl Pts',(13.9995910956154,0.,12.5772662595197));
#35146=CARTESIAN_POINT('Ctrl Pts',(13.9995910956154,-12.5772662595197,12.5772662595197));
#35147=CARTESIAN_POINT('Ctrl Pts',(13.9995910956154,-12.5772662595197,0.));
#35148=CARTESIAN_POINT('Ctrl Pts',(13.9995910956154,-12.5772662595197,-12.5772662595197));
#35149=CARTESIAN_POINT('Ctrl Pts',(13.9995910956154,0.,-12.5772662595197));
#35150=CARTESIAN_POINT('Ctrl Pts',(13.9995910956154,12.5772662595197,-12.5772662595197));
#35151=CARTESIAN_POINT('Ctrl Pts',(13.9995910956154,12.5772662595197,0.));
#35152=CARTESIAN_POINT('Ctrl Pts',(12.4874918670977,12.076207951456,0.));
#35153=CARTESIAN_POINT('Ctrl Pts',(12.4874918670977,12.076207951456,12.076207951456));
#35154=CARTESIAN_POINT('Ctrl Pts',(12.4874918670977,0.,12.076207951456));
#35155=CARTESIAN_POINT('Ctrl Pts',(12.4874918670977,-12.076207951456,12.076207951456));
#35156=CARTESIAN_POINT('Ctrl Pts',(12.4874918670977,-12.076207951456,0.));
#35157=CARTESIAN_POINT('Ctrl Pts',(12.4874918670977,-12.076207951456,-12.076207951456));
#35158=CARTESIAN_POINT('Ctrl Pts',(12.4874918670977,0.,-12.076207951456));
#35159=CARTESIAN_POINT('Ctrl Pts',(12.4874918670977,12.076207951456,-12.076207951456));
#35160=CARTESIAN_POINT('Ctrl Pts',(12.4874918670977,12.076207951456,0.));
#35161=CARTESIAN_POINT('Ctrl Pts',(10.979632440052,11.6661962584503,0.));
#35162=CARTESIAN_POINT('Ctrl Pts',(10.979632440052,11.6661962584503,11.6661962584503));
#35163=CARTESIAN_POINT('Ctrl Pts',(10.979632440052,0.,11.6661962584503));
#35164=CARTESIAN_POINT('Ctrl Pts',(10.979632440052,-11.6661962584503,11.6661962584503));
#35165=CARTESIAN_POINT('Ctrl Pts',(10.979632440052,-11.6661962584503,0.));
#35166=CARTESIAN_POINT('Ctrl Pts',(10.979632440052,-11.6661962584503,-11.6661962584503));
#35167=CARTESIAN_POINT('Ctrl Pts',(10.979632440052,0.,-11.6661962584503));
#35168=CARTESIAN_POINT('Ctrl Pts',(10.979632440052,11.6661962584503,-11.6661962584503));
#35169=CARTESIAN_POINT('Ctrl Pts',(10.979632440052,11.6661962584503,0.));
#35170=CARTESIAN_POINT('Ctrl Pts',(9.4782023240472,11.3469207764071,0.));
#35171=CARTESIAN_POINT('Ctrl Pts',(9.4782023240472,11.3469207764071,11.3469207764071));
#35172=CARTESIAN_POINT('Ctrl Pts',(9.4782023240472,0.,11.3469207764071));
#35173=CARTESIAN_POINT('Ctrl Pts',(9.47820232404719,-11.3469207764071,11.3469207764071));
#35174=CARTESIAN_POINT('Ctrl Pts',(9.47820232404719,-11.3469207764071,0.));
#35175=CARTESIAN_POINT('Ctrl Pts',(9.47820232404719,-11.3469207764071,-11.3469207764071));
#35176=CARTESIAN_POINT('Ctrl Pts',(9.4782023240472,0.,-11.3469207764071));
#35177=CARTESIAN_POINT('Ctrl Pts',(9.4782023240472,11.3469207764071,-11.3469207764071));
#35178=CARTESIAN_POINT('Ctrl Pts',(9.4782023240472,11.3469207764071,0.));
#35179=CARTESIAN_POINT('Ctrl Pts',(8.28303567503975,11.1635245405655,0.));
#35180=CARTESIAN_POINT('Ctrl Pts',(8.28303567503975,11.1635245405655,11.1635245405655));
#35181=CARTESIAN_POINT('Ctrl Pts',(8.28303567503976,0.,11.1635245405655));
#35182=CARTESIAN_POINT('Ctrl Pts',(8.28303567503978,-11.1635245405655,11.1635245405655));
#35183=CARTESIAN_POINT('Ctrl Pts',(8.28303567503978,-11.1635245405655,0.));
#35184=CARTESIAN_POINT('Ctrl Pts',(8.28303567503978,-11.1635245405655,-11.1635245405655));
#35185=CARTESIAN_POINT('Ctrl Pts',(8.28303567503976,0.,-11.1635245405655));
#35186=CARTESIAN_POINT('Ctrl Pts',(8.28303567503975,11.1635245405655,-11.1635245405655));
#35187=CARTESIAN_POINT('Ctrl Pts',(8.28303567503975,11.1635245405655,0.));
#35188=CARTESIAN_POINT('Ctrl Pts',(7.39016039139644,11.0661718180104,0.));
#35189=CARTESIAN_POINT('Ctrl Pts',(7.39016039139644,11.0661718180104,11.0661718180104));
#35190=CARTESIAN_POINT('Ctrl Pts',(7.39016039139642,0.,11.0661718180104));
#35191=CARTESIAN_POINT('Ctrl Pts',(7.3901603913964,-11.0661718180104,11.0661718180104));
#35192=CARTESIAN_POINT('Ctrl Pts',(7.3901603913964,-11.0661718180104,0.));
#35193=CARTESIAN_POINT('Ctrl Pts',(7.3901603913964,-11.0661718180104,-11.0661718180104));
#35194=CARTESIAN_POINT('Ctrl Pts',(7.39016039139642,0.,-11.0661718180104));
#35195=CARTESIAN_POINT('Ctrl Pts',(7.39016039139644,11.0661718180104,-11.0661718180104));
#35196=CARTESIAN_POINT('Ctrl Pts',(7.39016039139644,11.0661718180104,0.));
#35197=CARTESIAN_POINT('Ctrl Pts',(6.79646156908522,11.0190876606754,0.));
#35198=CARTESIAN_POINT('Ctrl Pts',(6.79646156908522,11.0190876606754,11.0190876606754));
#35199=CARTESIAN_POINT('Ctrl Pts',(6.79646156908522,0.,11.0190876606754));
#35200=CARTESIAN_POINT('Ctrl Pts',(6.79646156908521,-11.0190876606754,11.0190876606754));
#35201=CARTESIAN_POINT('Ctrl Pts',(6.79646156908521,-11.0190876606754,0.));
#35202=CARTESIAN_POINT('Ctrl Pts',(6.79646156908521,-11.0190876606754,-11.0190876606754));
#35203=CARTESIAN_POINT('Ctrl Pts',(6.79646156908522,0.,-11.0190876606754));
#35204=CARTESIAN_POINT('Ctrl Pts',(6.79646156908522,11.0190876606754,-11.0190876606754));
#35205=CARTESIAN_POINT('Ctrl Pts',(6.79646156908522,11.0190876606754,0.));
#35206=CARTESIAN_POINT('Ctrl Pts',(6.5,11.,0.));
#35207=CARTESIAN_POINT('Ctrl Pts',(6.5,11.,11.));
#35208=CARTESIAN_POINT('Ctrl Pts',(6.49999999999999,0.,11.));
#35209=CARTESIAN_POINT('Ctrl Pts',(6.49999999999997,-11.,11.));
#35210=CARTESIAN_POINT('Ctrl Pts',(6.49999999999997,-11.,0.));
#35211=CARTESIAN_POINT('Ctrl Pts',(6.49999999999997,-11.,-11.));
#35212=CARTESIAN_POINT('Ctrl Pts',(6.49999999999999,0.,-11.));
#35213=CARTESIAN_POINT('Ctrl Pts',(6.5,11.,-11.));
#35214=CARTESIAN_POINT('Ctrl Pts',(6.5,11.,0.));
#35215=CARTESIAN_POINT('',(37.5,28.7791366260183,-14.8835914705078));
#35216=CARTESIAN_POINT('Origin',(37.5,0.,0.));
#35217=CARTESIAN_POINT('Ctrl Pts',(37.5,28.7791366260183,-14.8835914705078));
#35218=CARTESIAN_POINT('Ctrl Pts',(36.649069632136,28.1289147924197,-14.5081857198467));
#35219=CARTESIAN_POINT('Ctrl Pts',(35.8406537800852,27.4207836130568,-14.09934599282));
#35220=CARTESIAN_POINT('Ctrl Pts',(35.0774452370494,26.7027592162945,-13.6847944140645));
#35221=CARTESIAN_POINT('Ctrl Pts',(34.6958409655315,26.3437470179134,-13.4775186246868));
#35222=CARTESIAN_POINT('Ctrl Pts',(34.325525504156,25.9822790638981,-13.2688250041327));
#35223=CARTESIAN_POINT('Ctrl Pts',(33.9666810635171,25.6244801370594,-13.0622496974066));
#35224=CARTESIAN_POINT('Ctrl Pts',(33.7186145566393,25.3771363861364,-12.9194457162288));
#35225=CARTESIAN_POINT('Ctrl Pts',(33.4671024168736,25.1224476749782,-12.7724011202821));
#35226=CARTESIAN_POINT('Ctrl Pts',(33.240098560953,24.8908093158805,-12.6386646513024));
#35227=CARTESIAN_POINT('Ctrl Pts',(33.1387264796059,24.7873676254901,-12.57894256351));
#35228=CARTESIAN_POINT('Ctrl Pts',(33.0532004124034,24.6997339702839,-12.5283472490867));
#35229=CARTESIAN_POINT('Ctrl Pts',(33.,24.6451817466334,-12.4968515080772));
#35230=CARTESIAN_POINT('Ctrl Pts',(32.9185691495925,24.5616817555094,-12.4486427657244));
#35231=CARTESIAN_POINT('Ctrl Pts',(32.8516820633328,24.4928265642782,-12.409196518007));
#35232=CARTESIAN_POINT('Ctrl Pts',(32.7777321456107,24.4165289206872,-12.3657029367534));
#35233=CARTESIAN_POINT('Ctrl Pts',(32.1788699540342,23.7986543447516,-12.0134826477878));
#35234=CARTESIAN_POINT('Ctrl Pts',(31.5692879871746,23.1567007301737,-11.6640598398951));
#35235=CARTESIAN_POINT('Ctrl Pts',(30.9513498040921,22.5260018679958,-11.3096185478676));
#35236=CARTESIAN_POINT('Ctrl Pts',(30.6423807125509,22.2106524369068,-11.1323979018538));
#35237=CARTESIAN_POINT('Ctrl Pts',(30.3347880607231,21.9015729508235,-10.9558507302175));
#35238=CARTESIAN_POINT('Ctrl Pts',(30.0249306372031,21.5982641082966,-10.7763433330279));
#35239=CARTESIAN_POINT('Ctrl Pts',(29.8700019254431,21.4466096870331,-10.686589634433));
#35240=CARTESIAN_POINT('Ctrl Pts',(29.7145097313607,21.2963965338214,-10.5960927952803));
#35241=CARTESIAN_POINT('Ctrl Pts',(29.5580100720539,21.1475727378965,-10.5043591957328));
#35242=CARTESIAN_POINT('Ctrl Pts',(29.4797602424005,21.073160839934,-10.4584923959591));
#35243=CARTESIAN_POINT('Ctrl Pts',(29.4012586241275,20.9990965425516,-10.4123158264294));
#35244=CARTESIAN_POINT('Ctrl Pts',(29.3224502420548,20.9253755287796,-10.365763682916));
#35245=CARTESIAN_POINT('Ctrl Pts',(29.2736528205758,20.8797281587122,-10.3369390260962));
#35246=CARTESIAN_POINT('Ctrl Pts',(29.224737793648,20.8342124355121,-10.3079703168046));
#35247=CARTESIAN_POINT('Ctrl Pts',(29.1756921968363,20.7888277155615,-10.2788413041483));
#35248=CARTESIAN_POINT('Ctrl Pts',(29.145528605634,20.7609156046197,-10.2609266352074));
#35249=CARTESIAN_POINT('Ctrl Pts',(29.1181490967959,20.7356566759367,-10.244640315201));
#35250=CARTESIAN_POINT('Ctrl Pts',(29.0849408699094,20.7051394327917,-10.2248462834623));
#35251=CARTESIAN_POINT('Ctrl Pts',(29.0475462330933,20.6707750197823,-10.2025569082866));
#35252=CARTESIAN_POINT('Ctrl Pts',(28.9599837407508,20.5905365512908,-10.1505620075807));
#35253=CARTESIAN_POINT('Ctrl Pts',(28.8924081847227,20.5290030523156,-10.1107110564612));
#35254=CARTESIAN_POINT('Ctrl Pts',(28.4410807634675,20.1180296612603,-9.84455228455516));
#35255=CARTESIAN_POINT('Ctrl Pts',(27.9936088567084,19.7235361016838,-9.59004457953207));
#35256=CARTESIAN_POINT('Ctrl Pts',(27.5122543095276,19.323133857666,-9.31395242983164));
#35257=CARTESIAN_POINT('Ctrl Pts',(27.139729410595,19.0132587222617,-9.1002820682123));
#35258=CARTESIAN_POINT('Ctrl Pts',(26.7276341640933,18.6830630721049,-8.8641048839258));
#35259=CARTESIAN_POINT('Ctrl Pts',(26.2530417505368,18.3335669465969,-8.57522710561967));
#35260=CARTESIAN_POINT('Ctrl Pts',(25.8694949138874,18.0511179871724,-8.34176749926539));
#35261=CARTESIAN_POINT('Ctrl Pts',(25.4447383161169,17.7540556187449,-8.07732257196191));
#35262=CARTESIAN_POINT('Ctrl Pts',(24.9635886608471,17.4401876876843,-7.77432947327891));
#35263=CARTESIAN_POINT('Ctrl Pts',(24.6119820459101,17.2108244540856,-7.55291317045008));
#35264=CARTESIAN_POINT('Ctrl Pts',(24.2873626785113,17.0017823418324,-7.34685978855489));
#35265=CARTESIAN_POINT('Ctrl Pts',(23.6426616416151,16.6259529313881,-6.93898570158392));
#35266=CARTESIAN_POINT('Ctrl Pts',(23.5760533210473,16.5871235136936,-6.89684553679212));
#35267=CARTESIAN_POINT('Ctrl Pts',(23.5065967304624,16.546947509807,-6.85292160231549));
#35268=CARTESIAN_POINT('Ctrl Pts',(23.4342591639586,16.5054784159948,-6.80720851268154));
#35269=CARTESIAN_POINT('Ctrl Pts',(22.7443384436259,16.1099662574127,-6.37121917473146));
#35270=CARTESIAN_POINT('Ctrl Pts',(21.7987837593167,15.60840670368,-5.75271743557013));
#35271=CARTESIAN_POINT('Ctrl Pts',(20.5610365528855,15.0432759423309,-4.96573918168373));
#35272=CARTESIAN_POINT('Ctrl Pts',(19.7234582214111,14.660854331766,-4.4331943054991));
#35273=CARTESIAN_POINT('Ctrl Pts',(18.7603809281631,14.261757368588,-3.80221290992202));
#35274=CARTESIAN_POINT('Ctrl Pts',(17.6514222906382,13.8414640697512,-3.1023654549763));
#35275=CARTESIAN_POINT('Ctrl Pts',(16.7565277906389,13.5023006881889,-2.53761072285453));
#35276=CARTESIAN_POINT('Ctrl Pts',(15.7613531057993,13.1550396644396,-1.89251696162035));
#35277=CARTESIAN_POINT('Ctrl Pts',(14.7199456843001,12.8103130578295,-1.24172578532011));
#35278=CARTESIAN_POINT('Ctrl Pts',(14.0653277478803,12.5936214775802,-0.832645181442172));
#35279=CARTESIAN_POINT('Ctrl Pts',(13.4031503824703,12.3831266019898,-0.410460471251366));
#35280=CARTESIAN_POINT('Ctrl Pts',(12.7552064848291,12.1808231353727,-1.04083408558608E-16));
#35281=CARTESIAN_POINT('Origin',(37.75,0.,0.));
#35282=CARTESIAN_POINT('Ctrl Pts',(38.0021093499888,29.2991567049652,-15.1841362142249));
#35283=CARTESIAN_POINT('Ctrl Pts',(37.8357506665067,29.1259188005428,-15.0841362838782));
#35284=CARTESIAN_POINT('Ctrl Pts',(37.6692050584524,28.9524909653522,-14.984024599313));
#35285=CARTESIAN_POINT('Ctrl Pts',(37.5025598114679,28.778970498635,-14.8838564824963));
#35286=CARTESIAN_POINT('Origin',(36.8,27.2943217538007,-27.2943217538008));
#35287=CARTESIAN_POINT('Origin',(36.8,27.2943217538007,-27.2943217538008));
#35288=CARTESIAN_POINT('Origin',(36.8,27.2943217538007,-27.2943217538008));
#35289=CARTESIAN_POINT('Ctrl Pts',(37.5,19.4092743732571,-25.9430157904517));
#35290=CARTESIAN_POINT('Ctrl Pts',(37.5185015343068,19.4038236586252,-25.9748214246283));
#35291=CARTESIAN_POINT('Ctrl Pts',(37.537045458494,19.398593936034,-26.0064935487318));
#35292=CARTESIAN_POINT('Ctrl Pts',(37.599346002575,19.3817798286964,-26.1122358651254));
#35293=CARTESIAN_POINT('Ctrl Pts',(37.6438438231274,19.3710168782448,-26.18666663184));
#35294=CARTESIAN_POINT('Ctrl Pts',(37.6890795305109,19.3613019153151,-26.2612698469762));
#35295=CARTESIAN_POINT('Ctrl Pts',(37.6890795305109,26.2612698469761,-19.3613019153152));
#35296=CARTESIAN_POINT('Ctrl Pts',(37.6438438231274,26.18666663184,-19.3710168782449));
#35297=CARTESIAN_POINT('Ctrl Pts',(37.599346002575,26.1122358651254,-19.3817798286965));
#35298=CARTESIAN_POINT('Ctrl Pts',(37.537045458494,26.0064935487318,-19.3985939360341));
#35299=CARTESIAN_POINT('Ctrl Pts',(37.5185015343068,25.9748214246282,-19.4038236586252));
#35300=CARTESIAN_POINT('Ctrl Pts',(37.5,25.9430157904516,-19.4092743732572));
#35301=CARTESIAN_POINT('Origin',(37.75,0.,0.));
#35302=CARTESIAN_POINT('Ctrl Pts',(38.0020193561147,17.781768196856,-27.7994139997877));
#35303=CARTESIAN_POINT('Ctrl Pts',(37.8356549036389,17.6817410994363,-27.6261918543797));
#35304=CARTESIAN_POINT('Ctrl Pts',(37.6691041509159,17.5816052376133,-27.4527780511187));
#35305=CARTESIAN_POINT('Ctrl Pts',(37.5024547303957,17.4814171457625,-27.2792691849716));
#35306=CARTESIAN_POINT('Origin',(37.75,0.,0.));
#35307=CARTESIAN_POINT('Origin',(36.8,9.9904151409573,-37.284736894758));
#35308=CARTESIAN_POINT('Origin',(36.8,9.99041514095729,-37.284736894758));
#35309=CARTESIAN_POINT('Origin',(36.8,9.99041514095729,-37.284736894758));
#35310=CARTESIAN_POINT('Ctrl Pts',(37.5,3.83741678103716,-32.1719479119405));
#35311=CARTESIAN_POINT('Ctrl Pts',(37.5185015343068,3.81679350660879,-32.196767041805));
#35312=CARTESIAN_POINT('Ctrl Pts',(37.537045458494,3.79642837193836,-32.2215810445749));
#35313=CARTESIAN_POINT('Ctrl Pts',(37.599346002575,3.72899576964523,-32.304749523158));
#35314=CARTESIAN_POINT('Ctrl Pts',(37.6438438231274,3.68245939777719,-32.3638269827301));
#35315=CARTESIAN_POINT('Ctrl Pts',(37.6890795305109,3.63674438551514,-32.4235777807772));
#35316=CARTESIAN_POINT('Ctrl Pts',(37.6890795305109,13.0622758654621,-29.8980142324913));
#35317=CARTESIAN_POINT('Ctrl Pts',(37.6438438231274,12.9928101044853,-29.8691260296172));
#35318=CARTESIAN_POINT('Ctrl Pts',(37.599346002575,12.9229696944615,-29.8412316347707));
#35319=CARTESIAN_POINT('Ctrl Pts',(37.537045458494,12.8229871085408,-29.8029219206701));
#35320=CARTESIAN_POINT('Ctrl Pts',(37.5185015343068,12.7929433831798,-29.791614931237));
#35321=CARTESIAN_POINT('Ctrl Pts',(37.5,12.7626735386834,-29.7804325714888));
#35322=CARTESIAN_POINT('Origin',(37.75,0.,0.));
#35323=CARTESIAN_POINT('Ctrl Pts',(38.0015719566141,1.49985854343196,-32.9658822396213));
#35324=CARTESIAN_POINT('Ctrl Pts',(37.8351948506471,1.49984891222423,-32.7658537908257));
#35325=CARTESIAN_POINT('Ctrl Pts',(37.6686397502842,1.49983991459912,-32.5656049542644));
#35326=CARTESIAN_POINT('Ctrl Pts',(37.5019970368724,1.49983187417044,-32.3652476458237));
#35327=CARTESIAN_POINT('Origin',(37.75,0.,0.));
#35328=CARTESIAN_POINT('Origin',(36.8,-9.99041514095732,-37.284736894758));
#35329=CARTESIAN_POINT('Origin',(36.8,-9.99041514095732,-37.284736894758));
#35330=CARTESIAN_POINT('Origin',(36.8,-9.99041514095732,-37.284736894758));
#35331=CARTESIAN_POINT('Ctrl Pts',(37.5,-12.7626735386834,-29.7804325714888));
#35332=CARTESIAN_POINT('Ctrl Pts',(37.5185015343068,-12.7929433831798,-29.791614931237));
#35333=CARTESIAN_POINT('Ctrl Pts',(37.537045458494,-12.8229871085408,-29.8029219206701));
#35334=CARTESIAN_POINT('Ctrl Pts',(37.599346002575,-12.9229696944615,-29.8412316347707));
#35335=CARTESIAN_POINT('Ctrl Pts',(37.6438438231274,-12.9928101044853,-29.8691260296172));
#35336=CARTESIAN_POINT('Ctrl Pts',(37.6890795305109,-13.0622758654621,-29.8980142324913));
#35337=CARTESIAN_POINT('Ctrl Pts',(37.6890795305109,-3.63674438551516,-32.4235777807772));
#35338=CARTESIAN_POINT('Ctrl Pts',(37.6438438231274,-3.68245939777721,-32.3638269827301));
#35339=CARTESIAN_POINT('Ctrl Pts',(37.599346002575,-3.72899576964525,-32.304749523158));
#35340=CARTESIAN_POINT('Ctrl Pts',(37.537045458494,-3.79642837193839,-32.2215810445749));
#35341=CARTESIAN_POINT('Ctrl Pts',(37.5185015343068,-3.81679350660881,-32.196767041805));
#35342=CARTESIAN_POINT('Ctrl Pts',(37.5,-3.83741678103718,-32.1719479119405));
#35343=CARTESIAN_POINT('Origin',(37.75,0.,0.));
#35344=CARTESIAN_POINT('Ctrl Pts',(38.0021093499887,-15.1841362142249,-29.2991567049651));
#35345=CARTESIAN_POINT('Ctrl Pts',(37.8357506665065,-15.0841362838781,-29.1259188005426));
#35346=CARTESIAN_POINT('Ctrl Pts',(37.6692050584523,-14.9840245993129,-28.952490965352));
#35347=CARTESIAN_POINT('Ctrl Pts',(37.5025598114678,-14.8838564824962,-28.778970498635));
#35348=CARTESIAN_POINT('Origin',(37.75,0.,0.));
#35349=CARTESIAN_POINT('Origin',(36.8,-27.2943217538008,-27.2943217538007));
#35350=CARTESIAN_POINT('Origin',(36.8,-27.2943217538008,-27.2943217538007));
#35351=CARTESIAN_POINT('Origin',(36.8,-27.2943217538008,-27.2943217538007));
#35352=CARTESIAN_POINT('Ctrl Pts',(37.5,-25.9430157904517,-19.4092743732571));
#35353=CARTESIAN_POINT('Ctrl Pts',(37.5185015343068,-25.9748214246283,-19.4038236586252));
#35354=CARTESIAN_POINT('Ctrl Pts',(37.537045458494,-26.0064935487318,-19.398593936034));
#35355=CARTESIAN_POINT('Ctrl Pts',(37.599346002575,-26.1122358651254,-19.3817798286965));
#35356=CARTESIAN_POINT('Ctrl Pts',(37.6438438231274,-26.18666663184,-19.3710168782449));
#35357=CARTESIAN_POINT('Ctrl Pts',(37.6890795305109,-26.2612698469762,-19.3613019153151));
#35358=CARTESIAN_POINT('Ctrl Pts',(37.6890795305109,-19.3613019153151,-26.2612698469761));
#35359=CARTESIAN_POINT('Ctrl Pts',(37.6438438231274,-19.3710168782449,-26.18666663184));
#35360=CARTESIAN_POINT('Ctrl Pts',(37.599346002575,-19.3817798286965,-26.1122358651254));
#35361=CARTESIAN_POINT('Ctrl Pts',(37.537045458494,-19.3985939360341,-26.0064935487318));
#35362=CARTESIAN_POINT('Ctrl Pts',(37.5185015343068,-19.4038236586252,-25.9748214246282));
#35363=CARTESIAN_POINT('Ctrl Pts',(37.5,-19.4092743732572,-25.9430157904516));
#35364=CARTESIAN_POINT('Origin',(37.75,0.,0.));
#35365=CARTESIAN_POINT('Ctrl Pts',(38.0020193561148,-27.7994139997878,-17.7817681968561));
#35366=CARTESIAN_POINT('Ctrl Pts',(37.8356549036392,-27.62619185438,-17.6817410994365));
#35367=CARTESIAN_POINT('Ctrl Pts',(37.6691041509162,-27.452778051119,-17.5816052376135));
#35368=CARTESIAN_POINT('Ctrl Pts',(37.5024547303958,-27.2792691849717,-17.4814171457626));
#35369=CARTESIAN_POINT('Origin',(37.75,0.,0.));
#35370=CARTESIAN_POINT('Origin',(36.8,-37.284736894758,-9.9904151409573));
#35371=CARTESIAN_POINT('Origin',(36.8,-37.284736894758,-9.9904151409573));
#35372=CARTESIAN_POINT('Origin',(36.8,-37.284736894758,-9.9904151409573));
#35373=CARTESIAN_POINT('Ctrl Pts',(37.5,-32.1719479119405,-3.83741678103716));
#35374=CARTESIAN_POINT('Ctrl Pts',(37.5185015343068,-32.196767041805,-3.81679350660879));
#35375=CARTESIAN_POINT('Ctrl Pts',(37.537045458494,-32.2215810445749,-3.79642837193836));
#35376=CARTESIAN_POINT('Ctrl Pts',(37.599346002575,-32.304749523158,-3.72899576964523));
#35377=CARTESIAN_POINT('Ctrl Pts',(37.6438438231274,-32.3638269827301,-3.68245939777719));
#35378=CARTESIAN_POINT('Ctrl Pts',(37.6890795305109,-32.4235777807772,-3.63674438551514));
#35379=CARTESIAN_POINT('Ctrl Pts',(37.6890795305109,-29.8980142324913,-13.062275865462));
#35380=CARTESIAN_POINT('Ctrl Pts',(37.6438438231274,-29.8691260296172,-12.9928101044853));
#35381=CARTESIAN_POINT('Ctrl Pts',(37.599346002575,-29.8412316347707,-12.9229696944615));
#35382=CARTESIAN_POINT('Ctrl Pts',(37.537045458494,-29.8029219206701,-12.8229871085408));
#35383=CARTESIAN_POINT('Ctrl Pts',(37.5185015343068,-29.791614931237,-12.7929433831798));
#35384=CARTESIAN_POINT('Ctrl Pts',(37.5,-29.7804325714888,-12.7626735386834));
#35385=CARTESIAN_POINT('Origin',(37.75,0.,0.));
#35386=CARTESIAN_POINT('Ctrl Pts',(38.0015719566141,-32.9658822396213,-1.49985854343196));
#35387=CARTESIAN_POINT('Ctrl Pts',(37.8351948506461,-32.7658537908245,-1.49984891222423));
#35388=CARTESIAN_POINT('Ctrl Pts',(37.6686397502833,-32.5656049542633,-1.49983991459912));
#35389=CARTESIAN_POINT('Ctrl Pts',(37.5019970368724,-32.3652476458237,-1.49983187417044));
#35390=CARTESIAN_POINT('Origin',(37.75,0.,0.));
#35391=CARTESIAN_POINT('Origin',(36.8,-37.284736894758,9.99041514095732));
#35392=CARTESIAN_POINT('Origin',(36.8,-37.284736894758,9.99041514095732));
#35393=CARTESIAN_POINT('Origin',(36.8,-37.284736894758,9.99041514095732));
#35394=CARTESIAN_POINT('Ctrl Pts',(37.5,-29.7804325714888,12.7626735386834));
#35395=CARTESIAN_POINT('Ctrl Pts',(37.5185015343068,-29.791614931237,12.7929433831798));
#35396=CARTESIAN_POINT('Ctrl Pts',(37.537045458494,-29.8029219206701,12.8229871085408));
#35397=CARTESIAN_POINT('Ctrl Pts',(37.599346002575,-29.8412316347707,12.9229696944615));
#35398=CARTESIAN_POINT('Ctrl Pts',(37.6438438231274,-29.8691260296172,12.9928101044853));
#35399=CARTESIAN_POINT('Ctrl Pts',(37.6890795305109,-29.8980142324913,13.0622758654621));
#35400=CARTESIAN_POINT('Ctrl Pts',(37.6890795305109,-32.4235777807772,3.63674438551516));
#35401=CARTESIAN_POINT('Ctrl Pts',(37.6438438231274,-32.3638269827301,3.68245939777721));
#35402=CARTESIAN_POINT('Ctrl Pts',(37.599346002575,-32.304749523158,3.72899576964525));
#35403=CARTESIAN_POINT('Ctrl Pts',(37.537045458494,-32.2215810445749,3.79642837193838));
#35404=CARTESIAN_POINT('Ctrl Pts',(37.5185015343068,-32.196767041805,3.81679350660881));
#35405=CARTESIAN_POINT('Ctrl Pts',(37.5,-32.1719479119405,3.83741678103718));
#35406=CARTESIAN_POINT('Origin',(37.75,0.,0.));
#35407=CARTESIAN_POINT('Ctrl Pts',(38.0021093499888,-29.2991567049652,15.1841362142249));
#35408=CARTESIAN_POINT('Ctrl Pts',(37.8357506665061,-29.1259188005422,15.0841362838778));
#35409=CARTESIAN_POINT('Ctrl Pts',(37.6692050584519,-28.9524909653516,14.9840245993126));
#35410=CARTESIAN_POINT('Ctrl Pts',(37.5025598114679,-28.778970498635,14.8838564824963));
#35411=CARTESIAN_POINT('Origin',(37.75,0.,0.));
#35412=CARTESIAN_POINT('Origin',(36.8,-27.2943217538007,27.2943217538008));
#35413=CARTESIAN_POINT('Origin',(36.8,-27.2943217538007,27.2943217538008));
#35414=CARTESIAN_POINT('Origin',(36.8,-27.2943217538007,27.2943217538008));
#35415=CARTESIAN_POINT('Ctrl Pts',(37.5,-19.4092743732572,25.9430157904517));
#35416=CARTESIAN_POINT('Ctrl Pts',(37.5185015343068,-19.4038236586252,25.9748214246283));
#35417=CARTESIAN_POINT('Ctrl Pts',(37.537045458494,-19.398593936034,26.0064935487318));
#35418=CARTESIAN_POINT('Ctrl Pts',(37.599346002575,-19.3817798286965,26.1122358651254));
#35419=CARTESIAN_POINT('Ctrl Pts',(37.6438438231274,-19.3710168782449,26.18666663184));
#35420=CARTESIAN_POINT('Ctrl Pts',(37.6890795305109,-19.3613019153151,26.2612698469761));
#35421=CARTESIAN_POINT('Ctrl Pts',(37.6890795305109,-26.2612698469761,19.3613019153151));
#35422=CARTESIAN_POINT('Ctrl Pts',(37.6438438231274,-26.18666663184,19.3710168782449));
#35423=CARTESIAN_POINT('Ctrl Pts',(37.599346002575,-26.1122358651254,19.3817798286965));
#35424=CARTESIAN_POINT('Ctrl Pts',(37.537045458494,-26.0064935487318,19.3985939360341));
#35425=CARTESIAN_POINT('Ctrl Pts',(37.5185015343068,-25.9748214246282,19.4038236586252));
#35426=CARTESIAN_POINT('Ctrl Pts',(37.5,-25.9430157904516,19.4092743732572));
#35427=CARTESIAN_POINT('Origin',(37.75,0.,0.));
#35428=CARTESIAN_POINT('Ctrl Pts',(38.0020193561148,-17.7817681968561,27.7994139997878));
#35429=CARTESIAN_POINT('Ctrl Pts',(37.8356549036384,-17.681741099436,27.6261918543792));
#35430=CARTESIAN_POINT('Ctrl Pts',(37.6691041509155,-17.5816052376131,27.4527780511183));
#35431=CARTESIAN_POINT('Ctrl Pts',(37.5024547303958,-17.4814171457626,27.2792691849717));
#35432=CARTESIAN_POINT('Origin',(37.75,0.,0.));
#35433=CARTESIAN_POINT('Origin',(36.8,-9.9904151409573,37.284736894758));
#35434=CARTESIAN_POINT('Origin',(36.8,-9.9904151409573,37.284736894758));
#35435=CARTESIAN_POINT('Origin',(36.8,-9.9904151409573,37.284736894758));
#35436=CARTESIAN_POINT('Ctrl Pts',(37.5,-3.83741678103716,32.1719479119405));
#35437=CARTESIAN_POINT('Ctrl Pts',(37.5185015343068,-3.81679350660879,32.196767041805));
#35438=CARTESIAN_POINT('Ctrl Pts',(37.537045458494,-3.79642837193837,32.2215810445749));
#35439=CARTESIAN_POINT('Ctrl Pts',(37.599346002575,-3.72899576964524,32.304749523158));
#35440=CARTESIAN_POINT('Ctrl Pts',(37.6438438231274,-3.6824593977772,32.3638269827301));
#35441=CARTESIAN_POINT('Ctrl Pts',(37.6890795305109,-3.63674438551516,32.4235777807772));
#35442=CARTESIAN_POINT('Ctrl Pts',(37.6890795305109,-13.062275865462,29.8980142324913));
#35443=CARTESIAN_POINT('Ctrl Pts',(37.6438438231274,-12.9928101044853,29.8691260296172));
#35444=CARTESIAN_POINT('Ctrl Pts',(37.599346002575,-12.9229696944615,29.8412316347707));
#35445=CARTESIAN_POINT('Ctrl Pts',(37.537045458494,-12.8229871085408,29.8029219206701));
#35446=CARTESIAN_POINT('Ctrl Pts',(37.5185015343068,-12.7929433831798,29.791614931237));
#35447=CARTESIAN_POINT('Ctrl Pts',(37.5,-12.7626735386834,29.7804325714888));
#35448=CARTESIAN_POINT('Origin',(37.75,0.,0.));
#35449=CARTESIAN_POINT('Ctrl Pts',(38.0015568568142,-1.49984972337186,32.9658830225135));
#35450=CARTESIAN_POINT('Ctrl Pts',(37.8351792988183,-1.49983922310652,32.7658546589327));
#35451=CARTESIAN_POINT('Ctrl Pts',(37.6686239963487,-1.4998293398377,32.565605908985));
#35452=CARTESIAN_POINT('Ctrl Pts',(37.5019813987213,-1.49982043004959,32.365248683748));
#35453=CARTESIAN_POINT('Origin',(37.75,0.,0.));
#35454=CARTESIAN_POINT('Origin',(36.8,9.99041514095731,37.284736894758));
#35455=CARTESIAN_POINT('Origin',(36.8,9.99041514095731,37.284736894758));
#35456=CARTESIAN_POINT('Origin',(36.8,9.99041514095731,37.284736894758));
#35457=CARTESIAN_POINT('Ctrl Pts',(37.5,12.7626735386834,29.7804325714888));
#35458=CARTESIAN_POINT('Ctrl Pts',(37.5185015343068,12.7929433831798,29.791614931237));
#35459=CARTESIAN_POINT('Ctrl Pts',(37.537045458494,12.8229871085408,29.8029219206701));
#35460=CARTESIAN_POINT('Ctrl Pts',(37.599346002575,12.9229696944615,29.8412316347707));
#35461=CARTESIAN_POINT('Ctrl Pts',(37.6438438231274,12.9928101044853,29.8691260296172));
#35462=CARTESIAN_POINT('Ctrl Pts',(37.6890795305109,13.062275865462,29.8980142324913));
#35463=CARTESIAN_POINT('Ctrl Pts',(37.6890795305109,3.63674438551516,32.4235777807772));
#35464=CARTESIAN_POINT('Ctrl Pts',(37.6438438231274,3.68245939777721,32.3638269827301));
#35465=CARTESIAN_POINT('Ctrl Pts',(37.599346002575,3.72899576964524,32.304749523158));
#35466=CARTESIAN_POINT('Ctrl Pts',(37.537045458494,3.79642837193838,32.2215810445749));
#35467=CARTESIAN_POINT('Ctrl Pts',(37.5185015343068,3.8167935066088,32.196767041805));
#35468=CARTESIAN_POINT('Ctrl Pts',(37.5,3.83741678103717,32.1719479119405));
#35469=CARTESIAN_POINT('Origin',(37.75,0.,0.));
#35470=CARTESIAN_POINT('Ctrl Pts',(38.0021093499888,15.1841362142249,29.2991567049652));
#35471=CARTESIAN_POINT('Ctrl Pts',(37.8357506665066,15.0841362838781,29.1259188005427));
#35472=CARTESIAN_POINT('Ctrl Pts',(37.6692050584524,14.9840245993129,28.9524909653521));
#35473=CARTESIAN_POINT('Ctrl Pts',(37.5025598114679,14.8838564824963,28.7789704986351));
#35474=CARTESIAN_POINT('Origin',(37.75,0.,0.));
#35475=CARTESIAN_POINT('Origin',(36.8,27.2943217538007,27.2943217538007));
#35476=CARTESIAN_POINT('Origin',(37.75,0.,0.));
#35477=CARTESIAN_POINT('Ctrl Pts',(38.0020193561148,27.7994139997877,17.7817681968561));
#35478=CARTESIAN_POINT('Ctrl Pts',(37.8356549036385,27.6261918543793,17.6817410994361));
#35479=CARTESIAN_POINT('Ctrl Pts',(37.6691041509156,27.4527780511184,17.5816052376131));
#35480=CARTESIAN_POINT('Ctrl Pts',(37.5024547303958,27.2792691849716,17.4814171457626));
#35481=CARTESIAN_POINT('Origin',(37.75,0.,0.));
#35482=CARTESIAN_POINT('Origin',(36.8,37.284736894758,9.9904151409573));
#35483=CARTESIAN_POINT('Origin',(37.75,0.,0.));
#35484=CARTESIAN_POINT('Ctrl Pts',(38.0015719566141,32.9658822396214,1.49985854343197));
#35485=CARTESIAN_POINT('Ctrl Pts',(37.8351948506466,32.7658537908251,1.49984891222424));
#35486=CARTESIAN_POINT('Ctrl Pts',(37.6686397502838,32.5656049542639,1.49983991459913));
#35487=CARTESIAN_POINT('Ctrl Pts',(37.5019970368724,32.3652476458238,1.49983187417045));
#35488=CARTESIAN_POINT('Origin',(37.75,0.,0.));
#35489=CARTESIAN_POINT('Origin',(52.1,0.,0.));
#35490=CARTESIAN_POINT('',(51.6,-8.5,-1.04094977927525E-15));
#35491=CARTESIAN_POINT('Origin',(51.6,0.,0.));
#35492=CARTESIAN_POINT('',(52.6,-8.5,-1.04094977927525E-15));
#35493=CARTESIAN_POINT('',(52.1,-8.5,-1.04094977927525E-15));
#35494=CARTESIAN_POINT('Origin',(52.6,0.,0.));
#35495=CARTESIAN_POINT('Origin',(51.6,9.7,0.));
#35496=CARTESIAN_POINT('Origin',(52.6,8.5,0.));
#35497=CARTESIAN_POINT('',(52.6,-9.2,-1.12667505521557E-15));
#35498=CARTESIAN_POINT('Origin',(52.6,0.,0.));
#35499=CARTESIAN_POINT('Origin',(49.75,0.,0.));
#35500=CARTESIAN_POINT('',(55.1,-9.2,-1.12667505521557E-15));
#35501=CARTESIAN_POINT('Origin',(55.1,0.,0.));
#35502=CARTESIAN_POINT('',(49.75,-9.2,-1.12667505521557E-15));
#35503=CARTESIAN_POINT('Origin',(48.825,0.,0.));
#35504=CARTESIAN_POINT('',(48.825,-7.7,-9.42978035343462E-16));
#35505=CARTESIAN_POINT('Origin',(6.9,25.9807621135332,-15.));
#35506=CARTESIAN_POINT('',(6.9,28.7358750109634,8.61681422303452));
#35507=CARTESIAN_POINT('Ctrl Pts',(6.9,10.3676856018661,3.76156693666918));
#35508=CARTESIAN_POINT('Ctrl Pts',(6.9,14.103554168739,4.66834435251375));
#35509=CARTESIAN_POINT('Ctrl Pts',(6.90000000166257,18.0191477848531,5.70305252110769));
#35510=CARTESIAN_POINT('Ctrl Pts',(6.90000000166257,23.666490663791,7.22296038005705));
#35511=CARTESIAN_POINT('Ctrl Pts',(6.9,26.2182182108371,7.92134750786925));
#35512=CARTESIAN_POINT('Ctrl Pts',(6.9,28.7358750109634,8.61681422303452));
#35513=CARTESIAN_POINT('Origin',(6.9,0.,0.));
#35514=CARTESIAN_POINT('Origin',(40.9,7.79422863405994,-4.5));
#35515=CARTESIAN_POINT('Ctrl Pts',(40.9,30.5996231131986,-15.9346498339374));
#35516=CARTESIAN_POINT('Ctrl Pts',(40.9,30.1661818974695,-15.6844024313584));
#35517=CARTESIAN_POINT('Ctrl Pts',(40.9,29.7327406817405,-15.4341550287793));
#35518=CARTESIAN_POINT('Ctrl Pts',(40.9,29.2992994660114,-15.1839076262003));
#35519=CARTESIAN_POINT('Ctrl Pts',(30.5,29.5001797522422,-18.8345266621011));
#35520=CARTESIAN_POINT('Ctrl Pts',(30.5,29.9204226682664,-18.176307754627));
#35521=CARTESIAN_POINT('Ctrl Pts',(30.5,30.3108891324553,-17.5));
#35522=CARTESIAN_POINT('Ctrl Pts',(30.5,47.8108891324553,12.8108891324553));
#35523=CARTESIAN_POINT('Ctrl Pts',(30.5,17.5,30.3108891324553));
#35524=CARTESIAN_POINT('Ctrl Pts',(30.5,-12.8108891324553,47.8108891324553));
#35525=CARTESIAN_POINT('Ctrl Pts',(30.5,-30.3108891324553,17.5));
#35526=CARTESIAN_POINT('Ctrl Pts',(30.5,-47.8108891324553,-12.8108891324553));
#35527=CARTESIAN_POINT('Ctrl Pts',(30.5,-17.5,-30.3108891324553));
#35528=CARTESIAN_POINT('Ctrl Pts',(30.5,11.4877949884694,-47.0470003722618));
#35529=CARTESIAN_POINT('Ctrl Pts',(30.5,29.5001797522422,-18.8345266621011));
#35530=CARTESIAN_POINT('Ctrl Pts',(30.3311478274255,29.4365936489566,-18.7939298193791));
#35531=CARTESIAN_POINT('Ctrl Pts',(30.3311478274255,29.8559307532302,-18.1371296685291));
#35532=CARTESIAN_POINT('Ctrl Pts',(30.3311478274255,30.245555587262,-17.4622796600955));
#35533=CARTESIAN_POINT('Ctrl Pts',(30.3311478274255,47.7078352473574,12.7832759271664));
#35534=CARTESIAN_POINT('Ctrl Pts',(30.3311478274255,17.4622796600955,30.245555587262));
#35535=CARTESIAN_POINT('Ctrl Pts',(30.3311478274255,-12.7832759271664,47.7078352473574));
#35536=CARTESIAN_POINT('Ctrl Pts',(30.3311478274255,-30.245555587262,17.4622796600955));
#35537=CARTESIAN_POINT('Ctrl Pts',(30.3311478274255,-47.7078352473574,-12.7832759271664));
#35538=CARTESIAN_POINT('Ctrl Pts',(30.3311478274255,-17.4622796600955,-30.245555587262));
#35539=CARTESIAN_POINT('Ctrl Pts',(30.3311478274255,11.4630336437997,-46.9455930096601));
#35540=CARTESIAN_POINT('Ctrl Pts',(30.3311478274255,29.4365936489566,-18.7939298193791));
#35541=CARTESIAN_POINT('Ctrl Pts',(29.9897712690917,29.3077924996107,-18.7116961278613));
#35542=CARTESIAN_POINT('Ctrl Pts',(29.9897712690917,29.7252947753835,-18.0577698358324));
#35543=CARTESIAN_POINT('Ctrl Pts',(29.9897712690917,30.1132147882992,-17.3858726641896));
#35544=CARTESIAN_POINT('Ctrl Pts',(29.9897712690917,47.4990874524888,12.7273421241096));
#35545=CARTESIAN_POINT('Ctrl Pts',(29.9897712690917,17.3858726641896,30.1132147882992));
#35546=CARTESIAN_POINT('Ctrl Pts',(29.9897712690917,-12.7273421241096,47.4990874524888));
#35547=CARTESIAN_POINT('Ctrl Pts',(29.9897712690917,-30.1132147882992,17.3858726641896));
#35548=CARTESIAN_POINT('Ctrl Pts',(29.9897712690917,-47.4990874524888,-12.7273421241096));
#35549=CARTESIAN_POINT('Ctrl Pts',(29.9897712690917,-17.3858726641896,-30.1132147882992));
#35550=CARTESIAN_POINT('Ctrl Pts',(29.9897712690917,11.4128766206768,-46.7401804402414));
#35551=CARTESIAN_POINT('Ctrl Pts',(29.9897712690917,29.3077924996107,-18.7116961278613));
#35552=CARTESIAN_POINT('Ctrl Pts',(29.4666899049319,29.1097034403905,-18.5852252487451));
#35553=CARTESIAN_POINT('Ctrl Pts',(29.4666899049319,29.5243838511923,-17.935718792976));
#35554=CARTESIAN_POINT('Ctrl Pts',(29.4666899049319,29.9096819433198,-17.2683629213518));
#35555=CARTESIAN_POINT('Ctrl Pts',(29.4666899049319,47.1780448646716,12.641319021968));
#35556=CARTESIAN_POINT('Ctrl Pts',(29.4666899049319,17.2683629213518,29.9096819433198));
#35557=CARTESIAN_POINT('Ctrl Pts',(29.4666899049319,-12.641319021968,47.1780448646716));
#35558=CARTESIAN_POINT('Ctrl Pts',(29.4666899049319,-29.9096819433198,17.2683629213518));
#35559=CARTESIAN_POINT('Ctrl Pts',(29.4666899049319,-47.1780448646716,-12.641319021968));
#35560=CARTESIAN_POINT('Ctrl Pts',(29.4666899049319,-17.2683629213518,-29.9096819433198));
#35561=CARTESIAN_POINT('Ctrl Pts',(29.4666899049319,11.3357378872557,-46.4242672450966));
#35562=CARTESIAN_POINT('Ctrl Pts',(29.4666899049319,29.1097034403905,-18.5852252487451));
#35563=CARTESIAN_POINT('Ctrl Pts',(28.7471241621752,28.8357745030392,-18.4103340474916));
#35564=CARTESIAN_POINT('Ctrl Pts',(28.7471241621752,29.246552676757,-17.7669395953572));
#35565=CARTESIAN_POINT('Ctrl Pts',(28.7471241621752,29.6282250261092,-17.105863694435));
#35566=CARTESIAN_POINT('Ctrl Pts',(28.7471241621752,46.7340887205442,12.5223613316742));
#35567=CARTESIAN_POINT('Ctrl Pts',(28.7471241621752,17.105863694435,29.6282250261092));
#35568=CARTESIAN_POINT('Ctrl Pts',(28.7471241621752,-12.5223613316742,46.7340887205442));
#35569=CARTESIAN_POINT('Ctrl Pts',(28.7471241621752,-29.6282250261092,17.105863694435));
#35570=CARTESIAN_POINT('Ctrl Pts',(28.7471241621752,-46.7340887205442,-12.5223613316742));
#35571=CARTESIAN_POINT('Ctrl Pts',(28.7471241621752,-17.105863694435,-29.6282250261092));
#35572=CARTESIAN_POINT('Ctrl Pts',(28.7471241621752,11.2290660127069,-45.9874043199967));
#35573=CARTESIAN_POINT('Ctrl Pts',(28.7471241621752,28.8357745030392,-18.4103340474916));
#35574=CARTESIAN_POINT('Ctrl Pts',(27.8100958442934,28.4776836217162,-18.1817092625453));
#35575=CARTESIAN_POINT('Ctrl Pts',(27.8100958442934,28.8833606347823,-17.5463046664274));
#35576=CARTESIAN_POINT('Ctrl Pts',(27.8100958442934,29.2602932679205,-16.8934381948013));
#35577=CARTESIAN_POINT('Ctrl Pts',(27.8100958442934,46.1537314627218,12.3668550731192));
#35578=CARTESIAN_POINT('Ctrl Pts',(27.8100958442934,16.8934381948013,29.2602932679205));
#35579=CARTESIAN_POINT('Ctrl Pts',(27.8100958442934,-12.3668550731192,46.1537314627218));
#35580=CARTESIAN_POINT('Ctrl Pts',(27.8100958442934,-29.2602932679205,16.8934381948013));
#35581=CARTESIAN_POINT('Ctrl Pts',(27.8100958442934,-46.1537314627218,-12.3668550731192));
#35582=CARTESIAN_POINT('Ctrl Pts',(27.8100958442934,-16.8934381948013,-29.2602932679205));
#35583=CARTESIAN_POINT('Ctrl Pts',(27.8100958442934,11.0896202647003,-45.4163196022628));
#35584=CARTESIAN_POINT('Ctrl Pts',(27.8100958442934,28.4776836217162,-18.1817092625453));
#35585=CARTESIAN_POINT('Ctrl Pts',(26.8343111708818,28.1064299010669,-17.9446806017473));
#35586=CARTESIAN_POINT('Ctrl Pts',(26.8343111708818,28.5068182430991,-17.3175595557791));
#35587=CARTESIAN_POINT('Ctrl Pts',(26.8343111708818,28.8788369357517,-16.6732042787396));
#35588=CARTESIAN_POINT('Ctrl Pts',(26.8343111708818,45.5520412144912,12.2056326570121));
#35589=CARTESIAN_POINT('Ctrl Pts',(26.8343111708818,16.6732042787396,28.8788369357517));
#35590=CARTESIAN_POINT('Ctrl Pts',(26.8343111708818,-12.2056326570121,45.5520412144912));
#35591=CARTESIAN_POINT('Ctrl Pts',(26.8343111708818,-28.8788369357517,16.6732042787396));
#35592=CARTESIAN_POINT('Ctrl Pts',(26.8343111708818,-45.5520412144912,-12.2056326570121));
#35593=CARTESIAN_POINT('Ctrl Pts',(26.8343111708818,-16.6732042787396,-28.8788369357517));
#35594=CARTESIAN_POINT('Ctrl Pts',(26.8343111708818,10.9450487174303,-44.8242427376375));
#35595=CARTESIAN_POINT('Ctrl Pts',(26.8343111708818,28.1064299010669,-17.9446806017473));
#35596=CARTESIAN_POINT('Ctrl Pts',(25.8181479469611,27.7272550606068,-17.7025946652472));
#35597=CARTESIAN_POINT('Ctrl Pts',(25.8181479469611,28.1222418918016,-17.0839339083798));
#35598=CARTESIAN_POINT('Ctrl Pts',(25.8181479469611,28.4892417994668,-16.4482714219305));
#35599=CARTESIAN_POINT('Ctrl Pts',(25.8181479469611,44.9375132213974,12.0409703775363));
#35600=CARTESIAN_POINT('Ctrl Pts',(25.8181479469611,16.4482714219305,28.4892417994668));
#35601=CARTESIAN_POINT('Ctrl Pts',(25.8181479469611,-12.0409703775363,44.9375132213974));
#35602=CARTESIAN_POINT('Ctrl Pts',(25.8181479469611,-28.4892417994668,16.4482714219305));
#35603=CARTESIAN_POINT('Ctrl Pts',(25.8181479469611,-44.9375132213974,-12.0409703775363));
#35604=CARTESIAN_POINT('Ctrl Pts',(25.8181479469611,-16.4482714219305,-28.4892417994668));
#35605=CARTESIAN_POINT('Ctrl Pts',(25.8181479469611,10.7973925719907,-44.2195332406074));
#35606=CARTESIAN_POINT('Ctrl Pts',(25.8181479469611,27.7272550606068,-17.7025946652472));
#35607=CARTESIAN_POINT('Ctrl Pts',(24.7595197917227,27.3496265541183,-17.4614959928472));
#35608=CARTESIAN_POINT('Ctrl Pts',(24.7595197917227,27.739233902677,-16.8512610227058));
#35609=CARTESIAN_POINT('Ctrl Pts',(24.7595197917227,28.1012354927406,-16.2242558762949));
#35610=CARTESIAN_POINT('Ctrl Pts',(24.7595197917227,44.3254913690355,11.8769796164457));
#35611=CARTESIAN_POINT('Ctrl Pts',(24.7595197917227,16.2242558762949,28.1012354927406));
#35612=CARTESIAN_POINT('Ctrl Pts',(24.7595197917227,-11.8769796164457,44.3254913690355));
#35613=CARTESIAN_POINT('Ctrl Pts',(24.7595197917227,-28.1012354927406,16.2242558762949));
#35614=CARTESIAN_POINT('Ctrl Pts',(24.7595197917227,-44.3254913690355,-11.8769796164457));
#35615=CARTESIAN_POINT('Ctrl Pts',(24.7595197917227,-16.2242558762949,-28.1012354927406));
#35616=CARTESIAN_POINT('Ctrl Pts',(24.7595197917227,10.6503385912768,-43.6172898429552));
#35617=CARTESIAN_POINT('Ctrl Pts',(24.7595197917227,27.3496265541183,-17.4614959928472));
#35618=CARTESIAN_POINT('Ctrl Pts',(23.6563574780851,26.9860278023044,-17.229354682426));
#35619=CARTESIAN_POINT('Ctrl Pts',(23.6563574780851,27.370455528196,-16.627232461942));
#35620=CARTESIAN_POINT('Ctrl Pts',(23.6563574780851,27.7276444994825,-16.0085630157705));
#35621=CARTESIAN_POINT('Ctrl Pts',(23.6563574780851,43.736207515253,11.719081483712));
#35622=CARTESIAN_POINT('Ctrl Pts',(23.6563574780851,16.0085630157705,27.7276444994825));
#35623=CARTESIAN_POINT('Ctrl Pts',(23.6563574780851,-11.719081483712,43.736207515253));
#35624=CARTESIAN_POINT('Ctrl Pts',(23.6563574780851,-27.7276444994825,16.0085630157705));
#35625=CARTESIAN_POINT('Ctrl Pts',(23.6563574780851,-43.736207515253,-11.719081483712));
#35626=CARTESIAN_POINT('Ctrl Pts',(23.6563574780851,-16.0085630157705,-27.7276444994825));
#35627=CARTESIAN_POINT('Ctrl Pts',(23.6563574780851,10.5087479991522,-43.0374211521332));
#35628=CARTESIAN_POINT('Ctrl Pts',(23.6563574780851,26.9860278023044,-17.229354682426));
#35629=CARTESIAN_POINT('Ctrl Pts',(22.5073180101405,26.649565639321,-17.0145388530744));
#35630=CARTESIAN_POINT('Ctrl Pts',(22.5073180101405,27.029200315079,-16.419923900654));
#35631=CARTESIAN_POINT('Ctrl Pts',(22.5073180101405,27.3819358493961,-15.8089680335819));
#35632=CARTESIAN_POINT('Ctrl Pts',(22.5073180101405,43.190903882978,11.5729678158142));
#35633=CARTESIAN_POINT('Ctrl Pts',(22.5073180101405,15.8089680335819,27.3819358493961));
#35634=CARTESIAN_POINT('Ctrl Pts',(22.5073180101405,-11.5729678158142,43.190903882978));
#35635=CARTESIAN_POINT('Ctrl Pts',(22.5073180101405,-27.3819358493961,15.8089680335819));
#35636=CARTESIAN_POINT('Ctrl Pts',(22.5073180101405,-43.190903882978,-11.5729678158142));
#35637=CARTESIAN_POINT('Ctrl Pts',(22.5073180101405,-15.8089680335819,-27.3819358493961));
#35638=CARTESIAN_POINT('Ctrl Pts',(22.5073180101405,10.3777247856603,-42.5008299977716));
#35639=CARTESIAN_POINT('Ctrl Pts',(22.5073180101405,26.649565639321,-17.0145388530744));
#35640=CARTESIAN_POINT('Ctrl Pts',(21.3125219557939,26.3518679613905,-16.8244723890963));
#35641=CARTESIAN_POINT('Ctrl Pts',(21.3125219557939,26.727261803997,-16.2364997772301));
#35642=CARTESIAN_POINT('Ctrl Pts',(21.3125219557939,27.0760569908086,-15.632368792237));
#35643=CARTESIAN_POINT('Ctrl Pts',(21.3125219557939,42.7084257830456,11.4436881985716));
#35644=CARTESIAN_POINT('Ctrl Pts',(21.3125219557939,15.632368792237,27.0760569908086));
#35645=CARTESIAN_POINT('Ctrl Pts',(21.3125219557939,-11.4436881985716,42.7084257830456));
#35646=CARTESIAN_POINT('Ctrl Pts',(21.3125219557939,-27.0760569908086,15.632368792237));
#35647=CARTESIAN_POINT('Ctrl Pts',(21.3125219557939,-42.7084257830456,-11.4436881985716));
#35648=CARTESIAN_POINT('Ctrl Pts',(21.3125219557939,-15.632368792237,-27.0760569908086));
#35649=CARTESIAN_POINT('Ctrl Pts',(21.3125219557939,10.2617970211066,-42.0260605935833));
#35650=CARTESIAN_POINT('Ctrl Pts',(21.3125219557939,26.3518679613905,-16.8244723890963));
#35651=CARTESIAN_POINT('Ctrl Pts',(20.0742472323676,26.1010282252799,-16.6643225955233));
#35652=CARTESIAN_POINT('Ctrl Pts',(20.0742472323676,26.4728487465358,-16.0819468125049));
#35653=CARTESIAN_POINT('Ctrl Pts',(20.0742472323676,26.8183238008715,-15.4835664656478));
#35654=CARTESIAN_POINT('Ctrl Pts',(20.0742472323676,42.3018902665193,11.3347573352238));
#35655=CARTESIAN_POINT('Ctrl Pts',(20.0742472323676,15.4835664656478,26.8183238008715));
#35656=CARTESIAN_POINT('Ctrl Pts',(20.0742472323676,-11.3347573352238,42.3018902665193));
#35657=CARTESIAN_POINT('Ctrl Pts',(20.0742472323676,-26.8183238008715,15.4835664656478));
#35658=CARTESIAN_POINT('Ctrl Pts',(20.0742472323676,-42.3018902665193,-11.3347573352238));
#35659=CARTESIAN_POINT('Ctrl Pts',(20.0742472323676,-15.4835664656478,-26.8183238008715));
#35660=CARTESIAN_POINT('Ctrl Pts',(20.0742472323676,10.1641164141543,-41.6260204156154));
#35661=CARTESIAN_POINT('Ctrl Pts',(20.0742472323676,26.1010282252799,-16.6643225955233));
#35662=CARTESIAN_POINT('Ctrl Pts',(18.7979917002302,25.8989065200918,-16.5352770548748));
#35663=CARTESIAN_POINT('Ctrl Pts',(18.7979917002302,26.2678477295776,-15.9574110860028));
#35664=CARTESIAN_POINT('Ctrl Pts',(18.7979917002302,26.6106474867381,-15.3636644897785));
#35665=CARTESIAN_POINT('Ctrl Pts',(18.7979917002302,41.9743119765166,11.2469829969596));
#35666=CARTESIAN_POINT('Ctrl Pts',(18.7979917002302,15.3636644897785,26.6106474867381));
#35667=CARTESIAN_POINT('Ctrl Pts',(18.7979917002302,-11.2469829969596,41.9743119765166));
#35668=CARTESIAN_POINT('Ctrl Pts',(18.7979917002302,-26.6106474867381,15.3636644897785));
#35669=CARTESIAN_POINT('Ctrl Pts',(18.7979917002302,-41.9743119765166,-11.2469829969596));
#35670=CARTESIAN_POINT('Ctrl Pts',(18.7979917002302,-15.3636644897785,-26.6106474867381));
#35671=CARTESIAN_POINT('Ctrl Pts',(18.7979917002302,10.0854073102973,-41.303675941138));
#35672=CARTESIAN_POINT('Ctrl Pts',(18.7979917002302,25.8989065200918,-16.5352770548748));
#35673=CARTESIAN_POINT('Ctrl Pts',(17.4917404060759,25.7420647185138,-16.4351406788133));
#35674=CARTESIAN_POINT('Ctrl Pts',(17.4917404060759,26.1087716481884,-15.8607742221527));
#35675=CARTESIAN_POINT('Ctrl Pts',(17.4917404060759,26.4494954361781,-15.2706233100072));
#35676=CARTESIAN_POINT('Ctrl Pts',(17.4917404060759,41.7201187461852,11.1788721261709));
#35677=CARTESIAN_POINT('Ctrl Pts',(17.4917404060759,15.2706233100072,26.4494954361781));
#35678=CARTESIAN_POINT('Ctrl Pts',(17.4917404060759,-11.1788721261709,41.7201187461852));
#35679=CARTESIAN_POINT('Ctrl Pts',(17.4917404060759,-26.4494954361781,15.2706233100072));
#35680=CARTESIAN_POINT('Ctrl Pts',(17.4917404060759,-41.7201187461852,-11.1788721261709));
#35681=CARTESIAN_POINT('Ctrl Pts',(17.4917404060759,-15.2706233100072,-26.4494954361781));
#35682=CARTESIAN_POINT('Ctrl Pts',(17.4917404060759,10.0243308532288,-41.0535440314616));
#35683=CARTESIAN_POINT('Ctrl Pts',(17.4917404060759,25.7420647185138,-16.4351406788133));
#35684=CARTESIAN_POINT('Ctrl Pts',(16.1647270995715,25.6237637373094,-16.3596108683728));
#35685=CARTESIAN_POINT('Ctrl Pts',(16.1647270995715,25.988785417954,-15.7878839869031));
#35686=CARTESIAN_POINT('Ctrl Pts',(16.1647270995715,26.3279433657953,-15.2004451894512));
#35687=CARTESIAN_POINT('Ctrl Pts',(16.1647270995715,41.5283885552464,11.1274981763441));
#35688=CARTESIAN_POINT('Ctrl Pts',(16.1647270995715,15.2004451894512,26.3279433657953));
#35689=CARTESIAN_POINT('Ctrl Pts',(16.1647270995715,-11.1274981763441,41.5283885552464));
#35690=CARTESIAN_POINT('Ctrl Pts',(16.1647270995715,-26.3279433657953,15.2004451894512));
#35691=CARTESIAN_POINT('Ctrl Pts',(16.1647270995715,-41.5283885552464,-11.1274981763441));
#35692=CARTESIAN_POINT('Ctrl Pts',(16.1647270995715,-15.2004451894512,-26.3279433657953));
#35693=CARTESIAN_POINT('Ctrl Pts',(16.1647270995715,9.97826274685029,-40.8648771706659));
#35694=CARTESIAN_POINT('Ctrl Pts',(16.1647270995715,25.6237637373094,-16.3596108683728));
#35695=CARTESIAN_POINT('Ctrl Pts',(14.8263876417415,25.5355400760542,-16.3032840624315));
#35696=CARTESIAN_POINT('Ctrl Pts',(14.8263876417415,25.8993049721986,-15.7335256598799));
#35697=CARTESIAN_POINT('Ctrl Pts',(14.8263876417415,26.2372951854241,-15.1481094381123));
#35698=CARTESIAN_POINT('Ctrl Pts',(14.8263876417415,41.3854046235364,11.0891857473118));
#35699=CARTESIAN_POINT('Ctrl Pts',(14.8263876417415,15.1481094381123,26.2372951854241));
#35700=CARTESIAN_POINT('Ctrl Pts',(14.8263876417415,-11.0891857473118,41.3854046235364));
#35701=CARTESIAN_POINT('Ctrl Pts',(14.8263876417415,-26.2372951854241,15.1481094381123));
#35702=CARTESIAN_POINT('Ctrl Pts',(14.8263876417415,-41.3854046235364,-11.0891857473118));
#35703=CARTESIAN_POINT('Ctrl Pts',(14.8263876417415,-15.1481094381123,-26.2372951854241));
#35704=CARTESIAN_POINT('Ctrl Pts',(14.8263876417415,9.94390718216752,-40.7241777356532));
#35705=CARTESIAN_POINT('Ctrl Pts',(14.8263876417415,25.5355400760542,-16.3032840624315));
#35706=CARTESIAN_POINT('Ctrl Pts',(13.4853470903953,25.4687774591536,-16.260659159851));
#35707=CARTESIAN_POINT('Ctrl Pts',(13.4853470903953,25.8315912927267,-15.6923903894687));
#35708=CARTESIAN_POINT('Ctrl Pts',(13.4853470903953,26.1686978312363,-15.1085047372063));
#35709=CARTESIAN_POINT('Ctrl Pts',(13.4853470903953,41.2772025684426,11.06019309403));
#35710=CARTESIAN_POINT('Ctrl Pts',(13.4853470903953,15.1085047372063,26.1686978312363));
#35711=CARTESIAN_POINT('Ctrl Pts',(13.4853470903953,-11.06019309403,41.2772025684426));
#35712=CARTESIAN_POINT('Ctrl Pts',(13.4853470903953,-26.1686978312363,15.1085047372063));
#35713=CARTESIAN_POINT('Ctrl Pts',(13.4853470903953,-41.2772025684426,-11.06019309403));
#35714=CARTESIAN_POINT('Ctrl Pts',(13.4853470903953,-15.1085047372063,-26.1686978312363));
#35715=CARTESIAN_POINT('Ctrl Pts',(13.4853470903953,9.91790885733393,-40.617704456895));
#35716=CARTESIAN_POINT('Ctrl Pts',(13.4853470903953,25.4687774591536,-16.260659159851));
#35717=CARTESIAN_POINT('Ctrl Pts',(12.1482076787549,25.4164718226475,-16.2272643834928));
#35718=CARTESIAN_POINT('Ctrl Pts',(12.1482076787549,25.778540539635,-15.660162675793));
#35719=CARTESIAN_POINT('Ctrl Pts',(12.1482076787549,26.1149547570431,-15.0774761588537));
#35720=CARTESIAN_POINT('Ctrl Pts',(12.1482076787549,41.1924309158968,11.0374785981893));
#35721=CARTESIAN_POINT('Ctrl Pts',(12.1482076787549,15.0774761588537,26.1149547570431));
#35722=CARTESIAN_POINT('Ctrl Pts',(12.1482076787549,-11.0374785981893,41.1924309158968));
#35723=CARTESIAN_POINT('Ctrl Pts',(12.1482076787549,-26.1149547570431,15.0774761588537));
#35724=CARTESIAN_POINT('Ctrl Pts',(12.1482076787549,-41.1924309158968,-11.0374785981893));
#35725=CARTESIAN_POINT('Ctrl Pts',(12.1482076787549,-15.0774761588537,-26.1149547570431));
#35726=CARTESIAN_POINT('Ctrl Pts',(12.1482076787549,9.89754028893977,-40.534287226192));
#35727=CARTESIAN_POINT('Ctrl Pts',(12.1482076787549,25.4164718226475,-16.2272643834928));
#35728=CARTESIAN_POINT('Ctrl Pts',(10.8190675759626,25.3740740708084,-16.2001953420791));
#35729=CARTESIAN_POINT('Ctrl Pts',(10.8190675759626,25.7355388133451,-15.6340396286792));
#35730=CARTESIAN_POINT('Ctrl Pts',(10.8190675759626,26.0713918511132,-15.0523251033885));
#35731=CARTESIAN_POINT('Ctrl Pts',(10.8190675759626,41.1237169545017,11.0190667477248));
#35732=CARTESIAN_POINT('Ctrl Pts',(10.8190675759626,15.0523251033885,26.0713918511132));
#35733=CARTESIAN_POINT('Ctrl Pts',(10.8190675759626,-11.0190667477248,41.1237169545017));
#35734=CARTESIAN_POINT('Ctrl Pts',(10.8190675759626,-26.0713918511132,15.0523251033885));
#35735=CARTESIAN_POINT('Ctrl Pts',(10.8190675759626,-41.1237169545017,-11.0190667477248));
#35736=CARTESIAN_POINT('Ctrl Pts',(10.8190675759626,-15.0523251033885,-26.0713918511132));
#35737=CARTESIAN_POINT('Ctrl Pts',(10.8190675759626,9.88102999357242,-40.4666711281441));
#35738=CARTESIAN_POINT('Ctrl Pts',(10.8190675759626,25.3740740708084,-16.2001953420791));
#35739=CARTESIAN_POINT('Ctrl Pts',(9.50027713254189,25.3387651379321,-16.1776521900286));
#35740=CARTESIAN_POINT('Ctrl Pts',(9.50027713254189,25.6997268893331,-15.6122843025816));
#35741=CARTESIAN_POINT('Ctrl Pts',(9.50027713254189,26.0351125755702,-15.0313792538877));
#35742=CARTESIAN_POINT('Ctrl Pts',(9.50027713254189,41.0664918294579,11.0037333216825));
#35743=CARTESIAN_POINT('Ctrl Pts',(9.50027713254189,15.0313792538877,26.0351125755702));
#35744=CARTESIAN_POINT('Ctrl Pts',(9.5002771325419,-11.0037333216825,41.0664918294579));
#35745=CARTESIAN_POINT('Ctrl Pts',(9.5002771325419,-26.0351125755702,15.0313792538877));
#35746=CARTESIAN_POINT('Ctrl Pts',(9.5002771325419,-41.0664918294579,-11.0037333216825));
#35747=CARTESIAN_POINT('Ctrl Pts',(9.50027713254189,-15.0313792538877,-26.0351125755702));
#35748=CARTESIAN_POINT('Ctrl Pts',(9.50027713254189,9.86728018643389,-40.4103603059007));
#35749=CARTESIAN_POINT('Ctrl Pts',(9.50027713254189,25.3387651379321,-16.1776521900286));
#35750=CARTESIAN_POINT('Ctrl Pts',(8.45435372222587,25.3150436214797,-16.1625070777669));
#35751=CARTESIAN_POINT('Ctrl Pts',(8.45435372222587,25.6756674495416,-15.5976684735573));
#35752=CARTESIAN_POINT('Ctrl Pts',(8.45435372222587,26.0107391561104,-15.0173072536015));
#35753=CARTESIAN_POINT('Ctrl Pts',(8.45435372222587,41.0280464097118,10.9934319025089));
#35754=CARTESIAN_POINT('Ctrl Pts',(8.45435372222587,15.0173072536015,26.0107391561104));
#35755=CARTESIAN_POINT('Ctrl Pts',(8.45435372222587,-10.9934319025089,41.0280464097118));
#35756=CARTESIAN_POINT('Ctrl Pts',(8.45435372222587,-26.0107391561104,15.0173072536015));
#35757=CARTESIAN_POINT('Ctrl Pts',(8.45435372222587,-41.0280464097118,-10.9934319025089));
#35758=CARTESIAN_POINT('Ctrl Pts',(8.45435372222587,-15.0173072536015,-26.0107391561104));
#35759=CARTESIAN_POINT('Ctrl Pts',(8.45435372222587,9.85804268618443,-40.3725291400319));
#35760=CARTESIAN_POINT('Ctrl Pts',(8.45435372222587,25.3150436214797,-16.1625070777669));
#35761=CARTESIAN_POINT('Ctrl Pts',(7.67514864245731,25.2995613842179,-16.1526223715399));
#35762=CARTESIAN_POINT('Ctrl Pts',(7.67514864245731,25.6599646610633,-15.5881292127269));
#35763=CARTESIAN_POINT('Ctrl Pts',(7.67514864245731,25.9948314436453,-15.0081229315276));
#35764=CARTESIAN_POINT('Ctrl Pts',(7.67514864245731,41.0029543751729,10.9867085121177));
#35765=CARTESIAN_POINT('Ctrl Pts',(7.67514864245731,15.0081229315276,25.9948314436453));
#35766=CARTESIAN_POINT('Ctrl Pts',(7.67514864245731,-10.9867085121177,41.0029543751729));
#35767=CARTESIAN_POINT('Ctrl Pts',(7.67514864245731,-25.9948314436453,15.0081229315276));
#35768=CARTESIAN_POINT('Ctrl Pts',(7.67514864245731,-41.0029543751729,-10.9867085121177));
#35769=CARTESIAN_POINT('Ctrl Pts',(7.67514864245731,-15.0081229315276,-25.9948314436453));
#35770=CARTESIAN_POINT('Ctrl Pts',(7.67514864245731,9.85201367995056,-40.3478380083732));
#35771=CARTESIAN_POINT('Ctrl Pts',(7.67514864245731,25.2995613842179,-16.1526223715399));
#35772=CARTESIAN_POINT('Ctrl Pts',(7.15799654185577,25.2902623130707,-16.1466853364124));
#35773=CARTESIAN_POINT('Ctrl Pts',(7.15799654185577,25.6505331205953,-15.5823996619098));
#35774=CARTESIAN_POINT('Ctrl Pts',(7.15799654185577,25.9852768200144,-15.0026065670023));
#35775=CARTESIAN_POINT('Ctrl Pts',(7.15799654185577,40.9878833870167,10.9826702530121));
#35776=CARTESIAN_POINT('Ctrl Pts',(7.15799654185577,15.0026065670023,25.9852768200144));
#35777=CARTESIAN_POINT('Ctrl Pts',(7.15799654185577,-10.9826702530121,40.9878833870167));
#35778=CARTESIAN_POINT('Ctrl Pts',(7.15799654185577,-25.9852768200144,15.0026065670023));
#35779=CARTESIAN_POINT('Ctrl Pts',(7.15799654185577,-40.9878833870167,-10.9826702530121));
#35780=CARTESIAN_POINT('Ctrl Pts',(7.15799654185577,-15.0026065670023,-25.9852768200144));
#35781=CARTESIAN_POINT('Ctrl Pts',(7.15799654185577,9.84839248767921,-40.3330078138659));
#35782=CARTESIAN_POINT('Ctrl Pts',(7.15799654185577,25.2902623130707,-16.1466853364124));
#35783=CARTESIAN_POINT('Ctrl Pts',(6.9,25.2858683590648,-16.1438799960867));
#35784=CARTESIAN_POINT('Ctrl Pts',(6.9,25.6460765727998,-15.5796923611089));
#35785=CARTESIAN_POINT('Ctrl Pts',(6.9,25.9807621135332,-15.));
#35786=CARTESIAN_POINT('Ctrl Pts',(6.9,40.9807621135332,10.9807621135331));
#35787=CARTESIAN_POINT('Ctrl Pts',(6.9,15.,25.9807621135332));
#35788=CARTESIAN_POINT('Ctrl Pts',(6.9,-10.9807621135331,40.9807621135332));
#35789=CARTESIAN_POINT('Ctrl Pts',(6.9,-25.9807621135332,15.));
#35790=CARTESIAN_POINT('Ctrl Pts',(6.9,-40.9807621135332,-10.9807621135331));
#35791=CARTESIAN_POINT('Ctrl Pts',(6.9,-15.,-25.9807621135332));
#35792=CARTESIAN_POINT('Ctrl Pts',(6.9,9.84668141868802,-40.3260003190816));
#35793=CARTESIAN_POINT('Ctrl Pts',(6.9,25.2858683590648,-16.1438799960867));
#35794=CARTESIAN_POINT('Ctrl Pts',(6.9,28.7358750109634,8.61681422303452));
#35795=CARTESIAN_POINT('Ctrl Pts',(7.85773098116326,29.3220126177434,6.72950262532882));
#35796=CARTESIAN_POINT('Ctrl Pts',(8.88781981167334,29.7139609348499,4.83176468807715));
#35797=CARTESIAN_POINT('Ctrl Pts',(10.5914578196776,30.0626260759601,1.83991777043966));
#35798=CARTESIAN_POINT('Ctrl Pts',(11.2365058953701,30.1308526921615,0.737334477600518));
#35799=CARTESIAN_POINT('Ctrl Pts',(12.0558885382926,30.1493644860168,-0.564998386426074));
#35800=CARTESIAN_POINT('Ctrl Pts',(12.1875764958397,30.1503477937894,-0.770798830274841));
#35801=CARTESIAN_POINT('Ctrl Pts',(13.194901830313,30.1433772121647,-2.32835059063961));
#35802=CARTESIAN_POINT('Ctrl Pts',(14.2258982134098,30.0606334052373,-3.91692083548089));
#35803=CARTESIAN_POINT('Ctrl Pts',(18.2616480823244,29.4024246647732,-8.94354621773405));
#35804=CARTESIAN_POINT('Ctrl Pts',(21.0496416709525,28.796919295079,-11.660889676038));
#35805=CARTESIAN_POINT('Ctrl Pts',(25.8000196361138,29.3778263502455,-14.7241675584603));
#35806=CARTESIAN_POINT('Ctrl Pts',(26.8976561124457,29.7353019177929,-15.1580512376427));
#35807=CARTESIAN_POINT('Ctrl Pts',(28.0045908801237,30.0977443108623,-15.5447817028247));
#35808=CARTESIAN_POINT('Ctrl Pts',(28.5235971652406,30.2828992744991,-15.6994510084801));
#35809=CARTESIAN_POINT('Ctrl Pts',(29.0834839543824,30.4804113157011,-15.8677990842846));
#35810=CARTESIAN_POINT('Ctrl Pts',(29.1146288039499,30.4913713634453,-15.877207296405));
#35811=CARTESIAN_POINT('Ctrl Pts',(29.5949306848436,30.6609898319163,-16.0210111630069));
#35812=CARTESIAN_POINT('Ctrl Pts',(30.0492939924726,30.8338536064743,-16.1312811324031));
#35813=CARTESIAN_POINT('Ctrl Pts',(30.5,31.0097594187194,-16.229443021655));
#35814=CARTESIAN_POINT('Ctrl Pts',(6.45331003273164,10.2495589536195,4.07387898226151));
#35815=CARTESIAN_POINT('Ctrl Pts',(7.20830533428676,10.4589493929845,3.54117612793134));
#35816=CARTESIAN_POINT('Ctrl Pts',(7.99943720515023,10.6278530262204,3.00808536723907));
#35817=CARTESIAN_POINT('Ctrl Pts',(9.76195392812149,10.8974188156737,1.87226624217412));
#35818=CARTESIAN_POINT('Ctrl Pts',(10.7319699357145,10.978614804603,1.2567580486118));
#35819=CARTESIAN_POINT('Ctrl Pts',(12.6618070777417,11.0581512103982,0.165209663835397));
#35820=CARTESIAN_POINT('Ctrl Pts',(13.6366888866736,11.0460663569154,-0.364704064273055));
#35821=CARTESIAN_POINT('Ctrl Pts',(15.55636942495,10.9884970038505,-1.27025231764747));
#35822=CARTESIAN_POINT('Ctrl Pts',(16.5294822240034,10.9232664847119,-1.69980161462952));
#35823=CARTESIAN_POINT('Ctrl Pts',(18.4405353898674,10.7982950788299,-2.41132585012622));
#35824=CARTESIAN_POINT('Ctrl Pts',(19.4148048972756,10.7128845485963,-2.74047342809724));
#35825=CARTESIAN_POINT('Ctrl Pts',(20.6320159197512,10.6248232626625,-3.07372863623309));
#35826=CARTESIAN_POINT('Ctrl Pts',(21.1045081958649,10.5890632628362,-3.19855905527614));
#35827=CARTESIAN_POINT('Ctrl Pts',(22.0534615876998,10.5175158204589,-3.42883778652051));
#35828=CARTESIAN_POINT('Ctrl Pts',(22.7823820470181,10.4664588970828,-3.58029681662341));
#35829=CARTESIAN_POINT('Ctrl Pts',(23.3297776630266,10.4341170945838,-3.67835397010643));
#35830=CARTESIAN_POINT('Ctrl Pts',(23.4470599317457,10.4271412460567,-3.69902619132824));
#35831=CARTESIAN_POINT('Ctrl Pts',(23.6811266122299,10.4133903945395,-3.73910834650869));
#35832=CARTESIAN_POINT('Ctrl Pts',(24.0941730950848,10.3895545652128,-3.80664723977491));
#35833=CARTESIAN_POINT('Ctrl Pts',(24.6899146335614,10.3570603924451,-3.89464075109997));
#35834=CARTESIAN_POINT('Ctrl Pts',(25.291236117096,10.3283061836387,-3.96994444386566));
#35835=CARTESIAN_POINT('Ctrl Pts',(25.773528518035,10.308597305488,-4.02162740546581));
#35836=CARTESIAN_POINT('Ctrl Pts',(26.0148283477099,10.3000025859217,-4.04448759176678));
#35837=CARTESIAN_POINT('Ctrl Pts',(26.5981242438443,10.2809495486037,-4.0960039723359));
#35838=CARTESIAN_POINT('Ctrl Pts',(27.5413774795629,10.2607319091993,-4.14752077886529));
#35839=CARTESIAN_POINT('Ctrl Pts',(28.5384263877913,10.2503835882543,-4.17105255246826));
#35840=CARTESIAN_POINT('Ctrl Pts',(29.1235503058367,10.244453382669,-4.18584784382924));
#35841=CARTESIAN_POINT('Ctrl Pts',(29.2812719873799,10.2430815653883,-4.18934848102508));
#35842=CARTESIAN_POINT('Ctrl Pts',(29.6033573831698,10.2409825864505,-4.19465178436652));
#35843=CARTESIAN_POINT('Ctrl Pts',(30.1682075695059,10.23904328544,-4.19956029863431));
#35844=CARTESIAN_POINT('Ctrl Pts',(31.3151152846707,10.2404426493561,-4.19601580459663));
#35845=CARTESIAN_POINT('Ctrl Pts',(32.3203773995796,10.2455622764132,-4.18330340731802));
#35846=CARTESIAN_POINT('Ctrl Pts',(33.1677006908682,10.2455713422049,-4.18329188254758));
#35847=CARTESIAN_POINT('Ctrl Pts',(33.494913285099,10.2455724350351,-4.18329063364475));
#35848=CARTESIAN_POINT('Ctrl Pts',(34.1541785734607,10.2455743198855,-4.18328832445806));
#35849=CARTESIAN_POINT('Ctrl Pts',(34.9761291047989,10.2455804319183,-4.18328098024986));
#35850=CARTESIAN_POINT('Ctrl Pts',(35.9637295000903,10.2455829874647,-4.18327789132126));
#35851=CARTESIAN_POINT('Ctrl Pts',(37.9383590406839,10.2455864680815,-4.18327370253669));
#35852=CARTESIAN_POINT('Ctrl Pts',(39.5833333333333,10.2456046429335,-4.18325179103929));
#35853=CARTESIAN_POINT('Ctrl Pts',(40.9,10.2456046429335,-4.18325179103929));
#35854=CARTESIAN_POINT('Ctrl Pts',(6.63336813585096,13.590868440034,4.85602971916216));
#35855=CARTESIAN_POINT('Ctrl Pts',(7.389696336477,13.8391951107513,4.14888858981181));
#35856=CARTESIAN_POINT('Ctrl Pts',(8.18053946683774,14.0346488726453,3.44401143686367));
#35857=CARTESIAN_POINT('Ctrl Pts',(9.9420194768364,14.3333081335907,1.94757748540837));
#35858=CARTESIAN_POINT('Ctrl Pts',(10.9113717350149,14.4104989873604,1.13915583855168));
#35859=CARTESIAN_POINT('Ctrl Pts',(12.834739732217,14.4628660834126,-0.286629408466326));
#35860=CARTESIAN_POINT('Ctrl Pts',(13.8081428716979,14.422640991687,-0.978270473832918));
#35861=CARTESIAN_POINT('Ctrl Pts',(15.7151185916567,14.3061107665235,-2.15221389622411));
#35862=CARTESIAN_POINT('Ctrl Pts',(16.6852254797785,14.2015789338064,-2.70962741922243));
#35863=CARTESIAN_POINT('Ctrl Pts',(18.5768226767694,14.0076819635675,-3.6260862081278));
#35864=CARTESIAN_POINT('Ctrl Pts',(19.5464729449596,13.8818273075211,-4.05120533415427));
#35865=CARTESIAN_POINT('Ctrl Pts',(20.746340681848,13.7535017581768,-4.4779302692017));
#35866=CARTESIAN_POINT('Ctrl Pts',(21.2156214332096,13.70158105669,-4.63869318435442));
#35867=CARTESIAN_POINT('Ctrl Pts',(22.1537708528637,13.5988388255708,-4.93390876526187));
#35868=CARTESIAN_POINT('Ctrl Pts',(22.8728508922896,13.5262523639446,-5.12767073297796));
#35869=CARTESIAN_POINT('Ctrl Pts',(23.4112391022536,13.4803679794399,-5.2528007404175));
#35870=CARTESIAN_POINT('Ctrl Pts',(23.5274006995052,13.4704404449521,-5.27931561824262));
#35871=CARTESIAN_POINT('Ctrl Pts',(23.7586975975698,13.4509289072633,-5.33062970711065));
#35872=CARTESIAN_POINT('Ctrl Pts',(24.1668938536997,13.4171810922988,-5.41708560365393));
#35873=CARTESIAN_POINT('Ctrl Pts',(24.7548128660956,13.3713845002051,-5.5295630582188));
#35874=CARTESIAN_POINT('Ctrl Pts',(25.3473131502195,13.3310219589391,-5.62567073595879));
#35875=CARTESIAN_POINT('Ctrl Pts',(25.8218041556279,13.3034028562424,-5.69154378511349));
#35876=CARTESIAN_POINT('Ctrl Pts',(26.058958766635,13.2913640661323,-5.72065900880544));
#35877=CARTESIAN_POINT('Ctrl Pts',(26.6316948383759,13.2646759506015,-5.7862349204564));
#35878=CARTESIAN_POINT('Ctrl Pts',(27.5576851463964,13.2364409873879,-5.85186367837985));
#35879=CARTESIAN_POINT('Ctrl Pts',(28.5507795710392,13.221915949884,-5.88219883517416));
#35880=CARTESIAN_POINT('Ctrl Pts',(29.1361849357885,13.2135466774644,-5.90128718803099));
#35881=CARTESIAN_POINT('Ctrl Pts',(29.2912521292175,13.2116327381159,-5.90574282943917));
#35882=CARTESIAN_POINT('Ctrl Pts',(29.6100275770337,13.2086893874641,-5.91253309751283));
#35883=CARTESIAN_POINT('Ctrl Pts',(30.1692894984411,13.205972123429,-5.91881362945882));
#35884=CARTESIAN_POINT('Ctrl Pts',(31.3098805820071,13.2079309635127,-5.91428725204098));
#35885=CARTESIAN_POINT('Ctrl Pts',(32.3163182251691,13.215170536538,-5.8978567744948));
#35886=CARTESIAN_POINT('Ctrl Pts',(33.1686695899411,13.2151857432769,-5.8978379745169));
#35887=CARTESIAN_POINT('Ctrl Pts',(33.4952713010557,13.2151875891279,-5.89783593918777));
#35888=CARTESIAN_POINT('Ctrl Pts',(34.1548283685118,13.2151907586342,-5.89783217350438));
#35889=CARTESIAN_POINT('Ctrl Pts',(34.9764778638341,13.2152010495211,-5.89782019909883));
#35890=CARTESIAN_POINT('Ctrl Pts',(35.9641101124161,13.2152053506642,-5.89781516246842));
#35891=CARTESIAN_POINT('Ctrl Pts',(37.9386244259607,13.2152112104218,-5.89780833274505));
#35892=CARTESIAN_POINT('Ctrl Pts',(39.5833333333333,13.2152418049849,-5.89777260594516));
#35893=CARTESIAN_POINT('Ctrl Pts',(40.9,13.2152418049849,-5.89777260594516));
#35894=CARTESIAN_POINT('Ctrl Pts',(6.84649785567288,21.3772113060719,6.71741536412572));
#35895=CARTESIAN_POINT('Ctrl Pts',(7.61279643984166,21.7222003209083,5.5922435141165));
#35896=CARTESIAN_POINT('Ctrl Pts',(8.41290239278215,21.9819683115275,4.47781399151289));
#35897=CARTESIAN_POINT('Ctrl Pts',(10.1883118359637,22.3516942143149,2.12504829883047));
#35898=CARTESIAN_POINT('Ctrl Pts',(11.1645908932198,22.4195115822635,0.860235293933488));
#35899=CARTESIAN_POINT('Ctrl Pts',(13.104616539894,22.4060524143024,-1.36442582505286));
#35900=CARTESIAN_POINT('Ctrl Pts',(14.0814329274866,22.2982732069865,-2.43568052201622));
#35901=CARTESIAN_POINT('Ctrl Pts',(15.9946796213894,22.0394507048972,-4.24582169215594));
#35902=CARTESIAN_POINT('Ctrl Pts',(16.9653275559584,21.84127820419,-5.10151618176832));
#35903=CARTESIAN_POINT('Ctrl Pts',(18.8448710605556,21.4842569534397,-6.49486940232065));
#35904=CARTESIAN_POINT('Ctrl Pts',(19.8101236302158,21.2634255374821,-7.14150804350573));
#35905=CARTESIAN_POINT('Ctrl Pts',(20.9856903475786,21.0426589820634,-7.78021164720297));
#35906=CARTESIAN_POINT('Ctrl Pts',(21.4500377829478,20.9532273635235,-8.02347291078474));
#35907=CARTESIAN_POINT('Ctrl Pts',(22.3710393802636,20.7788884454095,-8.46623345546776));
#35908=CARTESIAN_POINT('Ctrl Pts',(23.071969318899,20.6575298272076,-8.75491470148115));
#35909=CARTESIAN_POINT('Ctrl Pts',(23.5926347936584,20.5813719818059,-8.94023465873166));
#35910=CARTESIAN_POINT('Ctrl Pts',(23.7065892332642,20.5647099449237,-8.98001571960564));
#35911=CARTESIAN_POINT('Ctrl Pts',(23.9323706520525,20.5321468576873,-9.05664995495943));
#35912=CARTESIAN_POINT('Ctrl Pts',(24.3307466212141,20.4759485784749,-9.18574049076623));
#35913=CARTESIAN_POINT('Ctrl Pts',(24.9023508233183,20.4001844372315,-9.35309964749794));
#35914=CARTESIAN_POINT('Ctrl Pts',(25.4757972573109,20.333847241253,-9.49555868076772));
#35915=CARTESIAN_POINT('Ctrl Pts',(25.9330914993693,20.2886464898199,-9.59288697707764));
#35916=CARTESIAN_POINT('Ctrl Pts',(26.160978182331,20.2689918009897,-9.6358170524567));
#35917=CARTESIAN_POINT('Ctrl Pts',(26.7099322414348,20.2254900271806,-9.73235004955929));
#35918=CARTESIAN_POINT('Ctrl Pts',(27.5959509089717,20.1795241403996,-9.82915847887788));
#35919=CARTESIAN_POINT('Ctrl Pts',(28.5797495606368,20.1552722532429,-9.87532060641937));
#35920=CARTESIAN_POINT('Ctrl Pts',(29.1657855350674,20.1412111689924,-9.90441669946586));
#35921=CARTESIAN_POINT('Ctrl Pts',(29.3146731630634,20.1381027603737,-9.91097811975312));
#35922=CARTESIAN_POINT('Ctrl Pts',(29.625730006764,20.1332492263267,-9.92113271524795));
#35923=CARTESIAN_POINT('Ctrl Pts',(30.1719452394074,20.1287785103477,-9.93050366138689));
#35924=CARTESIAN_POINT('Ctrl Pts',(31.297781121968,20.131991612471,-9.92376874726294));
#35925=CARTESIAN_POINT('Ctrl Pts',(32.3069259117669,20.1442225454146,-9.89857089566956));
#35926=CARTESIAN_POINT('Ctrl Pts',(33.1709940314751,20.1442592438602,-9.8985167945155));
#35927=CARTESIAN_POINT('Ctrl Pts',(33.496168048976,20.1442637388651,-9.89851046735385));
#35928=CARTESIAN_POINT('Ctrl Pts',(34.1564024558334,20.1442714128624,-9.89849933968831));
#35929=CARTESIAN_POINT('Ctrl Pts',(34.9773378017947,20.1442963704308,-9.89846345509218));
#35930=CARTESIAN_POINT('Ctrl Pts',(35.965039526566,20.1443067963912,-9.8984484259258));
#35931=CARTESIAN_POINT('Ctrl Pts',(37.9392783163648,20.1443210056783,-9.89842798176079));
#35932=CARTESIAN_POINT('Ctrl Pts',(39.5833333333333,20.1443951831047,-9.89832117405886));
#35933=CARTESIAN_POINT('Ctrl Pts',(40.9,20.1443951831047,-9.89832117405886));
#35934=CARTESIAN_POINT('Ctrl Pts',(6.90857970435318,29.1272609852091,8.71018585725739));
#35935=CARTESIAN_POINT('Ctrl Pts',(7.67983757144493,29.5775536996439,7.16260494418019));
#35936=CARTESIAN_POINT('Ctrl Pts',(8.48457055999566,29.9097225030882,5.63283520142947));
#35937=CARTESIAN_POINT('Ctrl Pts',(10.2689932185249,30.364448769713,2.41146069737716));
#35938=CARTESIAN_POINT('Ctrl Pts',(11.2491988139072,30.4296414097155,0.6836721583184));
#35939=CARTESIAN_POINT('Ctrl Pts',(13.2074449203971,30.3576235761244,-2.36894751212039));
#35940=CARTESIAN_POINT('Ctrl Pts',(14.1878085217557,30.1849659988379,-3.82665309566742));
#35941=CARTESIAN_POINT('Ctrl Pts',(16.1228140255811,29.7814752498472,-6.30658851121943));
#35942=CARTESIAN_POINT('Ctrl Pts',(17.0983171044691,29.4886591763938,-7.46839135173999));
#35943=CARTESIAN_POINT('Ctrl Pts',(18.9977376700381,28.9600828729579,-9.36704911481258));
#35944=CARTESIAN_POINT('Ctrl Pts',(19.9674462816336,28.6415548808292,-10.2409515663327));
#35945=CARTESIAN_POINT('Ctrl Pts',(21.1471060032308,28.3239820751164,-11.1004135437215));
#35946=CARTESIAN_POINT('Ctrl Pts',(21.6116736136673,28.1962714220822,-11.4272945418466));
#35947=CARTESIAN_POINT('Ctrl Pts',(22.5321107331753,27.9485409607958,-12.020283834991));
#35948=CARTESIAN_POINT('Ctrl Pts',(23.2282372947767,27.7781185470826,-12.4035528917692));
#35949=CARTESIAN_POINT('Ctrl Pts',(23.7411423015334,27.6723004799181,-12.6473785079705));
#35950=CARTESIAN_POINT('Ctrl Pts',(23.854105005908,27.6489722597554,-12.7001926206311));
#35951=CARTESIAN_POINT('Ctrl Pts',(24.0772792343327,27.6035767537808,-12.801532363273));
#35952=CARTESIAN_POINT('Ctrl Pts',(24.4706231308704,27.5254067801745,-12.9720321690744));
#35953=CARTESIAN_POINT('Ctrl Pts',(25.0326506601032,27.4207276483817,-13.1919318242547));
#35954=CARTESIAN_POINT('Ctrl Pts',(25.592916616209,27.3299203180181,-13.3777331675808));
#35955=CARTESIAN_POINT('Ctrl Pts',(26.0369869863338,27.2685418387998,-13.5038445845533));
#35956=CARTESIAN_POINT('Ctrl Pts',(26.2572892845278,27.2420133361895,-13.5592118403735));
#35957=CARTESIAN_POINT('Ctrl Pts',(26.7861809172633,27.1835476308025,-13.6833062419415));
#35958=CARTESIAN_POINT('Ctrl Pts',(27.6340630276976,27.1220525704356,-13.8074117592231));
#35959=CARTESIAN_POINT('Ctrl Pts',(28.6084466264572,27.08811764436,-13.8693290201702));
#35960=CARTESIAN_POINT('Ctrl Pts',(29.1951297895237,27.0683644245334,-13.9084309041029));
#35961=CARTESIAN_POINT('Ctrl Pts',(29.3379067795072,27.0642236253564,-13.9168171018366));
#35962=CARTESIAN_POINT('Ctrl Pts',(29.641285245259,27.0575993546199,-13.930094679983));
#35963=CARTESIAN_POINT('Ctrl Pts',(30.17447907441,27.0515191755615,-13.9423073235084));
#35964=CARTESIAN_POINT('Ctrl Pts',(31.2855677213348,27.0558675796334,-13.9335693345849));
#35965=CARTESIAN_POINT('Ctrl Pts',(32.2974599236721,27.0731946134562,-13.8994232817537));
#35966=CARTESIAN_POINT('Ctrl Pts',(33.1732579076351,27.0732696672435,-13.8993047075201));
#35967=CARTESIAN_POINT('Ctrl Pts',(33.4970065888604,27.0732789151667,-13.8992904506871));
#35968=CARTESIAN_POINT('Ctrl Pts',(34.1579215418455,27.0732946436725,-13.8992658208367));
#35969=CARTESIAN_POINT('Ctrl Pts',(34.9781539333148,27.0733458523266,-13.8991859907804));
#35970=CARTESIAN_POINT('Ctrl Pts',(35.9659297143335,27.0733672375488,-13.8991526077107));
#35971=CARTESIAN_POINT('Ctrl Pts',(37.9398993196361,27.0733963900547,-13.8991071452309));
#35972=CARTESIAN_POINT('Ctrl Pts',(39.5833333333333,27.0735485612246,-13.8988697421725));
#35973=CARTESIAN_POINT('Ctrl Pts',(40.9,27.0735485612246,-13.8988697421725));
#35974=CARTESIAN_POINT('Ctrl Pts',(6.93528330520032,33.5512413216408,9.86563481868489));
#35975=CARTESIAN_POINT('Ctrl Pts',(7.70864561497005,34.0623374960229,8.07765806999139));
#35976=CARTESIAN_POINT('Ctrl Pts',(8.51541871352369,34.4367698578613,6.31093086144101));
#35977=CARTESIAN_POINT('Ctrl Pts',(10.3035747340621,34.941954951338,2.59403255178488));
#35978=CARTESIAN_POINT('Ctrl Pts',(11.2855474597114,35.0067705115655,0.601863607331421));
#35979=CARTESIAN_POINT('Ctrl Pts',(13.2510271399958,34.9032893217431,-2.92382891559037));
#35980=CARTESIAN_POINT('Ctrl Pts',(14.2329608248363,34.6945593989858,-4.60257161238984));
#35981=CARTESIAN_POINT('Ctrl Pts',(16.1768697182174,34.2095752766376,-7.46747574760141));
#35982=CARTESIAN_POINT('Ctrl Pts',(17.1545233971705,33.863251175018,-8.8049937479214));
#35983=CARTESIAN_POINT('Ctrl Pts',(19.0635787323924,33.2359528227276,-10.9976618314205));
#35984=CARTESIAN_POINT('Ctrl Pts',(20.0357940514506,32.8613840028833,-12.0029926013878));
#35985=CARTESIAN_POINT('Ctrl Pts',(21.2200273744509,32.4867165469275,-12.9932317593815));
#35986=CARTESIAN_POINT('Ctrl Pts',(21.6852779128343,32.3368305207215,-13.3687144259958));
#35987=CARTESIAN_POINT('Ctrl Pts',(22.6074094382986,32.0460468583649,-14.0501505350055));
#35988=CARTESIAN_POINT('Ctrl Pts',(23.3034045560158,31.8467199720653,-14.48918193341));
#35989=CARTESIAN_POINT('Ctrl Pts',(23.8143672767889,31.7234333079364,-14.7674149360665));
#35990=CARTESIAN_POINT('Ctrl Pts',(23.9270724954073,31.6962311639843,-14.8277950271987));
#35991=CARTESIAN_POINT('Ctrl Pts',(24.1495225469482,31.6433583861173,-14.9435144746796));
#35992=CARTESIAN_POINT('Ctrl Pts',(24.5413305977735,31.5524212197085,-15.1380475804186));
#35993=CARTESIAN_POINT('Ctrl Pts',(25.0999889357198,31.4310156375915,-15.3882930140601));
#35994=CARTESIAN_POINT('Ctrl Pts',(25.654856885479,31.3262265443362,-15.5988027583031));
#35995=CARTESIAN_POINT('Ctrl Pts',(26.0929602492092,31.2557376661539,-15.7410876933159));
#35996=CARTESIAN_POINT('Ctrl Pts',(26.3096479269531,31.2253935968529,-15.8033473177938));
#35997=CARTESIAN_POINT('Ctrl Pts',(26.8287121638339,31.1587088311851,-15.9425694431083));
#35998=CARTESIAN_POINT('Ctrl Pts',(27.6557884297531,31.0890012981154,-16.0810926132798));
#35999=CARTESIAN_POINT('Ctrl Pts',(28.6247091266678,31.0495586097514,-16.1519656805033));
#36000=CARTESIAN_POINT('Ctrl Pts',(29.2117706203406,31.0265558099778,-16.1967753671694));
#36001=CARTESIAN_POINT('Ctrl Pts',(29.3510921954877,31.0218764373727,-16.2061151113189));
#36002=CARTESIAN_POINT('Ctrl Pts',(29.6501043905813,31.0142857961677,-16.2210980111663));
#36003=CARTESIAN_POINT('Ctrl Pts',(30.1758702019788,31.0073340046884,-16.2348498398372));
#36004=CARTESIAN_POINT('Ctrl Pts',(31.2785352103418,31.0122942956315,-16.2250286703998));
#36005=CARTESIAN_POINT('Ctrl Pts',(32.2920164760144,31.0325718136051,-16.1856975481828));
#36006=CARTESIAN_POINT('Ctrl Pts',(33.174523274163,31.0326760798737,-16.1855272745483));
#36007=CARTESIAN_POINT('Ctrl Pts',(33.4974585875215,31.0326890056742,-16.1855064782319));
#36008=CARTESIAN_POINT('Ctrl Pts',(34.158763915549,31.0327109045833,-16.1854709093049));
#36009=CARTESIAN_POINT('Ctrl Pts',(34.9785998474407,31.0327822824582,-16.1853552918984));
#36010=CARTESIAN_POINT('Ctrl Pts',(35.9664200829455,31.0328120805001,-16.1853069853609));
#36011=CARTESIAN_POINT('Ctrl Pts',(37.9402388284556,31.0328527115371,-16.1852411572709));
#36012=CARTESIAN_POINT('Ctrl Pts',(39.5833333333333,31.033064777293,-16.1848974953804));
#36013=CARTESIAN_POINT('Ctrl Pts',(40.9,31.033064777293,-16.1848974953804));
#36014=CARTESIAN_POINT('Origin',(6.9,15.,-25.9807621135332));
#36015=CARTESIAN_POINT('',(6.9,29.194404870986,-6.90555748864274));
#36016=CARTESIAN_POINT('Ctrl Pts',(6.9,10.8594625780008,-1.92623027574191));
#36017=CARTESIAN_POINT('Ctrl Pts',(6.9,14.5482083700348,-3.008872281479));
#36018=CARTESIAN_POINT('Ctrl Pts',(6.90000000166257,18.4565659967827,-4.07058553003039));
#36019=CARTESIAN_POINT('Ctrl Pts',(6.90000000166257,24.1072623232988,-5.5779781522376));
#36020=CARTESIAN_POINT('Ctrl Pts',(6.9,26.6663167664834,-6.24902093139926));
#36021=CARTESIAN_POINT('Ctrl Pts',(6.9,29.194404870986,-6.90555748864274));
#36022=CARTESIAN_POINT('Origin',(6.9,0.,0.));
#36023=CARTESIAN_POINT('Origin',(40.9,4.49999999999999,-7.79422863405995));
#36024=CARTESIAN_POINT('Ctrl Pts',(40.9,18.5327260452907,-29.0996231131986));
#36025=CARTESIAN_POINT('Ctrl Pts',(40.9,18.2824786427117,-28.6661818974695));
#36026=CARTESIAN_POINT('Ctrl Pts',(40.9,18.0322312401326,-28.2327406817405));
#36027=CARTESIAN_POINT('Ctrl Pts',(40.9,17.7819838375536,-27.7992994660114));
#36028=CARTESIAN_POINT('Ctrl Pts',(30.5,16.1306417505985,-31.061268433756));
#36029=CARTESIAN_POINT('Ctrl Pts',(30.5,16.823692245373,-30.7013555966443));
#36030=CARTESIAN_POINT('Ctrl Pts',(30.5,17.5,-30.3108891324554));
#36031=CARTESIAN_POINT('Ctrl Pts',(30.5,47.8108891324553,-12.8108891324554));
#36032=CARTESIAN_POINT('Ctrl Pts',(30.5,30.3108891324554,17.5));
#36033=CARTESIAN_POINT('Ctrl Pts',(30.5,12.8108891324554,47.8108891324553));
#36034=CARTESIAN_POINT('Ctrl Pts',(30.5,-17.5,30.3108891324554));
#36035=CARTESIAN_POINT('Ctrl Pts',(30.5,-47.8108891324553,12.8108891324554));
#36036=CARTESIAN_POINT('Ctrl Pts',(30.5,-30.3108891324554,-17.5));
#36037=CARTESIAN_POINT('Ctrl Pts',(30.5,-13.5747778926489,-46.4877949884694));
#36038=CARTESIAN_POINT('Ctrl Pts',(30.5,16.1306417505985,-31.061268433756));
#36039=CARTESIAN_POINT('Ctrl Pts',(30.3311478274255,16.0958729911865,-30.9943174850025));
#36040=CARTESIAN_POINT('Ctrl Pts',(30.3311478274255,16.7874296516618,-30.6351804212937));
#36041=CARTESIAN_POINT('Ctrl Pts',(30.3311478274255,17.4622796600955,-30.245555587262));
#36042=CARTESIAN_POINT('Ctrl Pts',(30.3311478274255,47.7078352473574,-12.7832759271665));
#36043=CARTESIAN_POINT('Ctrl Pts',(30.3311478274255,30.245555587262,17.4622796600955));
#36044=CARTESIAN_POINT('Ctrl Pts',(30.3311478274255,12.7832759271665,47.7078352473574));
#36045=CARTESIAN_POINT('Ctrl Pts',(30.3311478274255,-17.4622796600955,30.245555587262));
#36046=CARTESIAN_POINT('Ctrl Pts',(30.3311478274255,-47.7078352473574,12.7832759271665));
#36047=CARTESIAN_POINT('Ctrl Pts',(30.3311478274255,-30.245555587262,-17.4622796600955));
#36048=CARTESIAN_POINT('Ctrl Pts',(30.3311478274255,-13.5455181648638,-46.3875929639907));
#36049=CARTESIAN_POINT('Ctrl Pts',(30.3311478274255,16.0958729911865,-30.9943174850025));
#36050=CARTESIAN_POINT('Ctrl Pts',(29.9897712690917,16.0254447695752,-30.8587004444282));
#36051=CARTESIAN_POINT('Ctrl Pts',(29.9897712690917,16.7139754925467,-30.501134801215));
#36052=CARTESIAN_POINT('Ctrl Pts',(29.9897712690917,17.3858726641896,-30.1132147882992));
#36053=CARTESIAN_POINT('Ctrl Pts',(29.9897712690917,47.4990874524888,-12.7273421241097));
#36054=CARTESIAN_POINT('Ctrl Pts',(29.9897712690917,30.1132147882992,17.3858726641896));
#36055=CARTESIAN_POINT('Ctrl Pts',(29.9897712690917,12.7273421241097,47.4990874524888));
#36056=CARTESIAN_POINT('Ctrl Pts',(29.9897712690917,-17.3858726641896,30.1132147882992));
#36057=CARTESIAN_POINT('Ctrl Pts',(29.9897712690917,-47.4990874524888,12.7273421241097));
#36058=CARTESIAN_POINT('Ctrl Pts',(29.9897712690917,-30.1132147882992,-17.3858726641896));
#36059=CARTESIAN_POINT('Ctrl Pts',(29.9897712690917,-13.4862491363571,-46.1846219490559));
#36060=CARTESIAN_POINT('Ctrl Pts',(29.9897712690917,16.0254447695752,-30.8587004444282));
#36061=CARTESIAN_POINT('Ctrl Pts',(29.4666899049319,15.9171300516369,-30.6501289206644));
#36062=CARTESIAN_POINT('Ctrl Pts',(29.4666899049319,16.6010070497276,-30.2949800354474));
#36063=CARTESIAN_POINT('Ctrl Pts',(29.4666899049319,17.2683629213518,-29.9096819433199));
#36064=CARTESIAN_POINT('Ctrl Pts',(29.4666899049319,47.1780448646716,-12.6413190219681));
#36065=CARTESIAN_POINT('Ctrl Pts',(29.4666899049319,29.9096819433199,17.2683629213518));
#36066=CARTESIAN_POINT('Ctrl Pts',(29.4666899049319,12.6413190219681,47.1780448646716));
#36067=CARTESIAN_POINT('Ctrl Pts',(29.4666899049319,-17.2683629213518,29.9096819433199));
#36068=CARTESIAN_POINT('Ctrl Pts',(29.4666899049319,-47.1780448646716,12.6413190219681));
#36069=CARTESIAN_POINT('Ctrl Pts',(29.4666899049319,-29.9096819433199,-17.2683629213518));
#36070=CARTESIAN_POINT('Ctrl Pts',(29.4666899049319,-13.3950966415431,-45.8724637299593));
#36071=CARTESIAN_POINT('Ctrl Pts',(29.4666899049319,15.9171300516369,-30.6501289206644));
#36072=CARTESIAN_POINT('Ctrl Pts',(28.7471241621752,15.7673462336858,-30.3617042288049));
#36073=CARTESIAN_POINT('Ctrl Pts',(28.7471241621752,16.4447877935127,-30.0098973754615));
#36074=CARTESIAN_POINT('Ctrl Pts',(28.7471241621752,17.105863694435,-29.6282250261092));
#36075=CARTESIAN_POINT('Ctrl Pts',(28.7471241621752,46.7340887205442,-12.5223613316743));
#36076=CARTESIAN_POINT('Ctrl Pts',(28.7471241621752,29.6282250261092,17.105863694435));
#36077=CARTESIAN_POINT('Ctrl Pts',(28.7471241621752,12.5223613316743,46.7340887205442));
#36078=CARTESIAN_POINT('Ctrl Pts',(28.7471241621752,-17.105863694435,29.6282250261092));
#36079=CARTESIAN_POINT('Ctrl Pts',(28.7471241621752,-46.7340887205442,12.5223613316743));
#36080=CARTESIAN_POINT('Ctrl Pts',(28.7471241621752,-29.6282250261092,-17.105863694435));
#36081=CARTESIAN_POINT('Ctrl Pts',(28.7471241621752,-13.2690457322218,-45.4407934015768));
#36082=CARTESIAN_POINT('Ctrl Pts',(28.7471241621752,15.7673462336858,-30.3617042288049));
#36083=CARTESIAN_POINT('Ctrl Pts',(27.8100958442934,15.5715428260696,-29.9846639164451));
#36084=CARTESIAN_POINT('Ctrl Pts',(27.8100958442934,16.2405717231752,-29.6372259010587));
#36085=CARTESIAN_POINT('Ctrl Pts',(27.8100958442934,16.8934381948013,-29.2602932679205));
#36086=CARTESIAN_POINT('Ctrl Pts',(27.8100958442934,46.1537314627218,-12.3668550731192));
#36087=CARTESIAN_POINT('Ctrl Pts',(27.8100958442934,29.2602932679205,16.8934381948013));
#36088=CARTESIAN_POINT('Ctrl Pts',(27.8100958442934,12.3668550731192,46.1537314627218));
#36089=CARTESIAN_POINT('Ctrl Pts',(27.8100958442934,-16.8934381948013,29.2602932679205));
#36090=CARTESIAN_POINT('Ctrl Pts',(27.8100958442934,-46.1537314627218,12.3668550731192));
#36091=CARTESIAN_POINT('Ctrl Pts',(27.8100958442934,-29.2602932679205,-16.8934381948013));
#36092=CARTESIAN_POINT('Ctrl Pts',(27.8100958442934,-13.1042669335782,-44.8764966543029));
#36093=CARTESIAN_POINT('Ctrl Pts',(27.8100958442934,15.5715428260696,-29.9846639164451));
#36094=CARTESIAN_POINT('Ctrl Pts',(26.8343111708818,15.3685420031368,-29.5937642144445));
#36095=CARTESIAN_POINT('Ctrl Pts',(26.8343111708818,16.0288490017,-29.2508556284042));
#36096=CARTESIAN_POINT('Ctrl Pts',(26.8343111708818,16.6732042787395,-28.8788369357517));
#36097=CARTESIAN_POINT('Ctrl Pts',(26.8343111708818,45.5520412144912,-12.2056326570122));
#36098=CARTESIAN_POINT('Ctrl Pts',(26.8343111708818,28.8788369357517,16.6732042787395));
#36099=CARTESIAN_POINT('Ctrl Pts',(26.8343111708818,12.2056326570122,45.5520412144912));
#36100=CARTESIAN_POINT('Ctrl Pts',(26.8343111708818,-16.6732042787395,28.8788369357517));
#36101=CARTESIAN_POINT('Ctrl Pts',(26.8343111708818,-45.5520412144912,12.2056326570122));
#36102=CARTESIAN_POINT('Ctrl Pts',(26.8343111708818,-28.8788369357517,-16.6732042787395));
#36103=CARTESIAN_POINT('Ctrl Pts',(26.8343111708818,-12.9334311338659,-44.2914572749094));
#36104=CARTESIAN_POINT('Ctrl Pts',(26.8343111708818,15.3685420031368,-29.5937642144445));
#36105=CARTESIAN_POINT('Ctrl Pts',(25.8181479469611,15.1612099270725,-29.1945242233064));
#36106=CARTESIAN_POINT('Ctrl Pts',(25.8181479469611,15.8126089354813,-28.8562417071321));
#36107=CARTESIAN_POINT('Ctrl Pts',(25.8181479469611,16.4482714219305,-28.4892417994669));
#36108=CARTESIAN_POINT('Ctrl Pts',(25.8181479469611,44.9375132213974,-12.0409703775364));
#36109=CARTESIAN_POINT('Ctrl Pts',(25.8181479469611,28.4892417994669,16.4482714219305));
#36110=CARTESIAN_POINT('Ctrl Pts',(25.8181479469611,12.0409703775364,44.9375132213974));
#36111=CARTESIAN_POINT('Ctrl Pts',(25.8181479469611,-16.4482714219305,28.4892417994669));
#36112=CARTESIAN_POINT('Ctrl Pts',(25.8181479469611,-44.9375132213974,12.0409703775364));
#36113=CARTESIAN_POINT('Ctrl Pts',(25.8181479469611,-28.4892417994669,-16.4482714219305));
#36114=CARTESIAN_POINT('Ctrl Pts',(25.8181479469611,-12.7589503583264,-43.6939354158518));
#36115=CARTESIAN_POINT('Ctrl Pts',(25.8181479469611,15.1612099270725,-29.1945242233064));
#36116=CARTESIAN_POINT('Ctrl Pts',(24.7595197917227,14.9547233834603,-28.796912394945));
#36117=CARTESIAN_POINT('Ctrl Pts',(24.7595197917227,15.5972507298839,-28.4632370828043));
#36118=CARTESIAN_POINT('Ctrl Pts',(24.7595197917227,16.2242558762948,-28.1012354927406));
#36119=CARTESIAN_POINT('Ctrl Pts',(24.7595197917227,44.3254913690355,-11.8769796164458));
#36120=CARTESIAN_POINT('Ctrl Pts',(24.7595197917227,28.1012354927406,16.2242558762948));
#36121=CARTESIAN_POINT('Ctrl Pts',(24.7595197917227,11.8769796164458,44.3254913690355));
#36122=CARTESIAN_POINT('Ctrl Pts',(24.7595197917227,-16.2242558762948,28.1012354927406));
#36123=CARTESIAN_POINT('Ctrl Pts',(24.7595197917227,-44.3254913690355,11.8769796164458));
#36124=CARTESIAN_POINT('Ctrl Pts',(24.7595197917227,-28.1012354927406,-16.2242558762948));
#36125=CARTESIAN_POINT('Ctrl Pts',(24.7595197917227,-12.5851811425261,-43.0988503438666));
#36126=CARTESIAN_POINT('Ctrl Pts',(24.7595197917227,14.9547233834603,-28.796912394945));
#36127=CARTESIAN_POINT('Ctrl Pts',(23.6563574780851,14.7559082828157,-28.4140727469455));
#36128=CARTESIAN_POINT('Ctrl Pts',(23.6563574780851,15.389893569599,-28.084833470769));
#36129=CARTESIAN_POINT('Ctrl Pts',(23.6563574780851,16.0085630157705,-27.7276444994825));
#36130=CARTESIAN_POINT('Ctrl Pts',(23.6563574780851,43.736207515253,-11.7190814837121));
#36131=CARTESIAN_POINT('Ctrl Pts',(23.6563574780851,27.7276444994825,16.0085630157705));
#36132=CARTESIAN_POINT('Ctrl Pts',(23.6563574780851,11.7190814837121,43.736207515253));
#36133=CARTESIAN_POINT('Ctrl Pts',(23.6563574780851,-16.0085630157705,27.7276444994825));
#36134=CARTESIAN_POINT('Ctrl Pts',(23.6563574780851,-43.736207515253,11.7190814837121));
#36135=CARTESIAN_POINT('Ctrl Pts',(23.6563574780851,-27.7276444994825,-16.0085630157705));
#36136=CARTESIAN_POINT('Ctrl Pts',(23.6563574780851,-12.4178678468319,-42.5258740306932));
#36137=CARTESIAN_POINT('Ctrl Pts',(23.6563574780851,14.7559082828157,-28.4140727469455));
#36138=CARTESIAN_POINT('Ctrl Pts',(22.5073180101405,14.5719314169357,-28.0598057001003));
#36139=CARTESIAN_POINT('Ctrl Pts',(22.5073180101405,15.1980121665098,-27.7346713837132));
#36140=CARTESIAN_POINT('Ctrl Pts',(22.5073180101405,15.8089680335819,-27.3819358493961));
#36141=CARTESIAN_POINT('Ctrl Pts',(22.5073180101405,43.190903882978,-11.5729678158142));
#36142=CARTESIAN_POINT('Ctrl Pts',(22.5073180101405,27.3819358493961,15.8089680335819));
#36143=CARTESIAN_POINT('Ctrl Pts',(22.5073180101405,11.5729678158142,43.190903882978));
#36144=CARTESIAN_POINT('Ctrl Pts',(22.5073180101405,-15.8089680335819,27.3819358493961));
#36145=CARTESIAN_POINT('Ctrl Pts',(22.5073180101405,-43.190903882978,11.5729678158142));
#36146=CARTESIAN_POINT('Ctrl Pts',(22.5073180101405,-27.3819358493961,-15.8089680335819));
#36147=CARTESIAN_POINT('Ctrl Pts',(22.5073180101405,-12.2630417010206,-41.9956608528241));
#36148=CARTESIAN_POINT('Ctrl Pts',(22.5073180101405,14.5719314169357,-28.0598057001003));
#36149=CARTESIAN_POINT('Ctrl Pts',(21.3125219557939,14.4091508971892,-27.7463544749225));
#36150=CARTESIAN_POINT('Ctrl Pts',(21.3125219557939,15.0282378072439,-27.4248521776202));
#36151=CARTESIAN_POINT('Ctrl Pts',(21.3125219557939,15.632368792237,-27.0760569908086));
#36152=CARTESIAN_POINT('Ctrl Pts',(21.3125219557939,42.7084257830456,-11.4436881985716));
#36153=CARTESIAN_POINT('Ctrl Pts',(21.3125219557939,27.0760569908086,15.632368792237));
#36154=CARTESIAN_POINT('Ctrl Pts',(21.3125219557939,11.4436881985716,42.7084257830456));
#36155=CARTESIAN_POINT('Ctrl Pts',(21.3125219557939,-15.632368792237,27.0760569908086));
#36156=CARTESIAN_POINT('Ctrl Pts',(21.3125219557939,-42.7084257830456,11.4436881985716));
#36157=CARTESIAN_POINT('Ctrl Pts',(21.3125219557939,-27.0760569908086,-15.632368792237));
#36158=CARTESIAN_POINT('Ctrl Pts',(21.3125219557939,-12.1260533880339,-41.5265346055806));
#36159=CARTESIAN_POINT('Ctrl Pts',(21.3125219557939,14.4091508971892,-27.7463544749225));
#36160=CARTESIAN_POINT('Ctrl Pts',(20.0742472323676,14.2719922102254,-27.4822408172221));
#36161=CARTESIAN_POINT('Ctrl Pts',(20.0742472323676,14.8851861187905,-27.1637988552073));
#36162=CARTESIAN_POINT('Ctrl Pts',(20.0742472323676,15.4835664656477,-26.8183238008716));
#36163=CARTESIAN_POINT('Ctrl Pts',(20.0742472323676,42.3018902665193,-11.3347573352238));
#36164=CARTESIAN_POINT('Ctrl Pts',(20.0742472323676,26.8183238008716,15.4835664656477));
#36165=CARTESIAN_POINT('Ctrl Pts',(20.0742472323676,11.3347573352238,42.3018902665193));
#36166=CARTESIAN_POINT('Ctrl Pts',(20.0742472323676,-15.4835664656477,26.8183238008716));
#36167=CARTESIAN_POINT('Ctrl Pts',(20.0742472323676,-42.3018902665193,11.3347573352238));
#36168=CARTESIAN_POINT('Ctrl Pts',(20.0742472323676,-26.8183238008716,-15.4835664656477));
#36169=CARTESIAN_POINT('Ctrl Pts',(20.0742472323676,-12.0106271861277,-41.1312493454498));
#36170=CARTESIAN_POINT('Ctrl Pts',(20.0742472323676,14.2719922102254,-27.4822408172221));
#36171=CARTESIAN_POINT('Ctrl Pts',(18.7979917002302,14.1614724492005,-27.2694232481814));
#36172=CARTESIAN_POINT('Ctrl Pts',(18.7979917002302,14.7699178935542,-26.9534472438987));
#36173=CARTESIAN_POINT('Ctrl Pts',(18.7979917002302,15.3636644897785,-26.6106474867382));
#36174=CARTESIAN_POINT('Ctrl Pts',(18.7979917002302,41.9743119765166,-11.2469829969597));
#36175=CARTESIAN_POINT('Ctrl Pts',(18.7979917002302,26.6106474867382,15.3636644897785));
#36176=CARTESIAN_POINT('Ctrl Pts',(18.7979917002302,11.2469829969597,41.9743119765166));
#36177=CARTESIAN_POINT('Ctrl Pts',(18.7979917002302,-15.3636644897785,26.6106474867382));
#36178=CARTESIAN_POINT('Ctrl Pts',(18.7979917002302,-41.9743119765166,11.2469829969597));
#36179=CARTESIAN_POINT('Ctrl Pts',(18.7979917002302,-26.6106474867382,-15.3636644897785));
#36180=CARTESIAN_POINT('Ctrl Pts',(18.7979917002302,-11.9176190323383,-40.8127362898543));
#36181=CARTESIAN_POINT('Ctrl Pts',(18.7979917002302,14.1614724492005,-27.2694232481814));
#36182=CARTESIAN_POINT('Ctrl Pts',(17.4917404060759,14.0757116526894,-27.1042817018803));
#36183=CARTESIAN_POINT('Ctrl Pts',(17.4917404060759,14.6804723978617,-26.7902192241678));
#36184=CARTESIAN_POINT('Ctrl Pts',(17.4917404060759,15.2706233100072,-26.4494954361781));
#36185=CARTESIAN_POINT('Ctrl Pts',(17.4917404060759,41.7201187461852,-11.1788721261709));
#36186=CARTESIAN_POINT('Ctrl Pts',(17.4917404060759,26.4494954361781,15.2706233100072));
#36187=CARTESIAN_POINT('Ctrl Pts',(17.4917404060759,11.1788721261709,41.7201187461852));
#36188=CARTESIAN_POINT('Ctrl Pts',(17.4917404060759,-15.2706233100072,26.4494954361781));
#36189=CARTESIAN_POINT('Ctrl Pts',(17.4917404060759,-41.7201187461852,11.1788721261709));
#36190=CARTESIAN_POINT('Ctrl Pts',(17.4917404060759,-26.4494954361781,-15.2706233100072));
#36191=CARTESIAN_POINT('Ctrl Pts',(17.4917404060759,-11.8454468408945,-40.5655774732432));
#36192=CARTESIAN_POINT('Ctrl Pts',(17.4917404060759,14.0757116526894,-27.1042817018803));
#36193=CARTESIAN_POINT('Ctrl Pts',(16.1647270995715,14.011024902894,-26.9797204766935));
#36194=CARTESIAN_POINT('Ctrl Pts',(16.1647270995715,14.6130063919992,-26.6671013136366));
#36195=CARTESIAN_POINT('Ctrl Pts',(16.1647270995715,15.2004451894511,-26.3279433657953));
#36196=CARTESIAN_POINT('Ctrl Pts',(16.1647270995715,41.5283885552464,-11.1274981763442));
#36197=CARTESIAN_POINT('Ctrl Pts',(16.1647270995715,26.3279433657953,15.2004451894511));
#36198=CARTESIAN_POINT('Ctrl Pts',(16.1647270995715,11.1274981763442,41.5283885552464));
#36199=CARTESIAN_POINT('Ctrl Pts',(16.1647270995715,-15.2004451894511,26.3279433657953));
#36200=CARTESIAN_POINT('Ctrl Pts',(16.1647270995715,-41.5283885552464,11.1274981763442));
#36201=CARTESIAN_POINT('Ctrl Pts',(16.1647270995715,-26.3279433657953,-15.2004451894511));
#36202=CARTESIAN_POINT('Ctrl Pts',(16.1647270995715,-11.7910095609247,-40.3791531257526));
#36203=CARTESIAN_POINT('Ctrl Pts',(16.1647270995715,14.011024902894,-26.9797204766935));
#36204=CARTESIAN_POINT('Ctrl Pts',(14.8263876417415,13.9627843740028,-26.8868282012068));
#36205=CARTESIAN_POINT('Ctrl Pts',(14.8263876417415,14.5626932163446,-26.5752853986496));
#36206=CARTESIAN_POINT('Ctrl Pts',(14.8263876417415,15.1481094381123,-26.2372951854241));
#36207=CARTESIAN_POINT('Ctrl Pts',(14.8263876417415,41.3854046235364,-11.0891857473119));
#36208=CARTESIAN_POINT('Ctrl Pts',(14.8263876417415,26.2372951854241,15.1481094381123));
#36209=CARTESIAN_POINT('Ctrl Pts',(14.8263876417415,11.0891857473119,41.3854046235364));
#36210=CARTESIAN_POINT('Ctrl Pts',(14.8263876417415,-15.1481094381123,26.2372951854241));
#36211=CARTESIAN_POINT('Ctrl Pts',(14.8263876417415,-41.3854046235364,11.0891857473119));
#36212=CARTESIAN_POINT('Ctrl Pts',(14.8263876417415,-26.2372951854241,-15.1481094381123));
#36213=CARTESIAN_POINT('Ctrl Pts',(14.8263876417415,-11.750412635195,-40.2401260583921));
#36214=CARTESIAN_POINT('Ctrl Pts',(14.8263876417415,13.9627843740028,-26.8868282012068));
#36215=CARTESIAN_POINT('Ctrl Pts',(13.4853470903953,13.926278703034,-26.8165326442879));
#36216=CARTESIAN_POINT('Ctrl Pts',(13.4853470903953,14.5246190849439,-26.505804369746));
#36217=CARTESIAN_POINT('Ctrl Pts',(13.4853470903953,15.1085047372062,-26.1686978312363));
#36218=CARTESIAN_POINT('Ctrl Pts',(13.4853470903953,41.2772025684426,-11.0601930940301));
#36219=CARTESIAN_POINT('Ctrl Pts',(13.4853470903953,26.1686978312363,15.1085047372062));
#36220=CARTESIAN_POINT('Ctrl Pts',(13.4853470903953,11.0601930940301,41.2772025684426));
#36221=CARTESIAN_POINT('Ctrl Pts',(13.4853470903953,-15.1085047372062,26.1686978312363));
#36222=CARTESIAN_POINT('Ctrl Pts',(13.4853470903953,-41.2772025684426,11.0601930940301));
#36223=CARTESIAN_POINT('Ctrl Pts',(13.4853470903953,-26.1686978312363,-15.1085047372062));
#36224=CARTESIAN_POINT('Ctrl Pts',(13.4853470903953,-11.7196912055777,-40.1349183317465));
#36225=CARTESIAN_POINT('Ctrl Pts',(13.4853470903953,13.926278703034,-26.8165326442879));
#36226=CARTESIAN_POINT('Ctrl Pts',(12.1482076787549,13.8976780812377,-26.7614591013549));
#36227=CARTESIAN_POINT('Ctrl Pts',(12.1482076787549,14.4947896419144,-26.4513689744511));
#36228=CARTESIAN_POINT('Ctrl Pts',(12.1482076787549,15.0774761588537,-26.1149547570431));
#36229=CARTESIAN_POINT('Ctrl Pts',(12.1482076787549,41.1924309158967,-11.0374785981894));
#36230=CARTESIAN_POINT('Ctrl Pts',(12.1482076787549,26.1149547570431,15.0774761588537));
#36231=CARTESIAN_POINT('Ctrl Pts',(12.1482076787549,11.0374785981894,41.1924309158967));
#36232=CARTESIAN_POINT('Ctrl Pts',(12.1482076787549,-15.0774761588537,26.1149547570431));
#36233=CARTESIAN_POINT('Ctrl Pts',(12.1482076787549,-41.1924309158967,11.0374785981894));
#36234=CARTESIAN_POINT('Ctrl Pts',(12.1482076787549,-26.1149547570431,-15.0774761588537));
#36235=CARTESIAN_POINT('Ctrl Pts',(12.1482076787549,-11.6956222878942,-40.0524926066472));
#36236=CARTESIAN_POINT('Ctrl Pts',(12.1482076787549,13.8976780812377,-26.7614591013549));
#36237=CARTESIAN_POINT('Ctrl Pts',(10.8190675759626,13.8744950717886,-26.716817747915));
#36238=CARTESIAN_POINT('Ctrl Pts',(10.8190675759626,14.4706105780977,-26.4072448888814));
#36239=CARTESIAN_POINT('Ctrl Pts',(10.8190675759626,15.0523251033884,-26.0713918511133));
#36240=CARTESIAN_POINT('Ctrl Pts',(10.8190675759626,41.1237169545017,-11.0190667477248));
#36241=CARTESIAN_POINT('Ctrl Pts',(10.8190675759626,26.0713918511133,15.0523251033884));
#36242=CARTESIAN_POINT('Ctrl Pts',(10.8190675759626,11.0190667477248,41.1237169545017));
#36243=CARTESIAN_POINT('Ctrl Pts',(10.8190675759626,-15.0523251033884,26.0713918511133));
#36244=CARTESIAN_POINT('Ctrl Pts',(10.8190675759626,-41.1237169545017,11.0190667477248));
#36245=CARTESIAN_POINT('Ctrl Pts',(10.8190675759626,-26.0713918511133,-15.0523251033884));
#36246=CARTESIAN_POINT('Ctrl Pts',(10.8190675759626,-11.6761125740824,-39.9856802003493));
#36247=CARTESIAN_POINT('Ctrl Pts',(10.8190675759626,13.8744950717886,-26.716817747915));
#36248=CARTESIAN_POINT('Ctrl Pts',(9.50027713254189,13.8551882149624,-26.6796403391198));
#36249=CARTESIAN_POINT('Ctrl Pts',(9.50027713254189,14.4504742051937,-26.3704982618073));
#36250=CARTESIAN_POINT('Ctrl Pts',(9.50027713254189,15.0313792538877,-26.0351125755702));
#36251=CARTESIAN_POINT('Ctrl Pts',(9.50027713254189,41.0664918294579,-11.0037333216826));
#36252=CARTESIAN_POINT('Ctrl Pts',(9.50027713254189,26.0351125755702,15.0313792538877));
#36253=CARTESIAN_POINT('Ctrl Pts',(9.5002771325419,11.0037333216826,41.0664918294579));
#36254=CARTESIAN_POINT('Ctrl Pts',(9.5002771325419,-15.0313792538877,26.0351125755702));
#36255=CARTESIAN_POINT('Ctrl Pts',(9.5002771325419,-41.0664918294579,11.0037333216826));
#36256=CARTESIAN_POINT('Ctrl Pts',(9.50027713254189,-26.0351125755702,-15.0313792538877));
#36257=CARTESIAN_POINT('Ctrl Pts',(9.50027713254189,-11.6598648452398,-39.9300386942093));
#36258=CARTESIAN_POINT('Ctrl Pts',(9.50027713254189,13.8551882149624,-26.6796403391198));
#36259=CARTESIAN_POINT('Ctrl Pts',(8.45435372222587,13.8422173352291,-26.6546635289318));
#36260=CARTESIAN_POINT('Ctrl Pts',(8.45435372222587,14.4369460336456,-26.3458108626791));
#36261=CARTESIAN_POINT('Ctrl Pts',(8.45435372222587,15.0173072536014,-26.0107391561104));
#36262=CARTESIAN_POINT('Ctrl Pts',(8.45435372222587,41.0280464097118,-10.9934319025089));
#36263=CARTESIAN_POINT('Ctrl Pts',(8.45435372222587,26.0107391561104,15.0173072536014));
#36264=CARTESIAN_POINT('Ctrl Pts',(8.45435372222587,10.9934319025089,41.0280464097118));
#36265=CARTESIAN_POINT('Ctrl Pts',(8.45435372222587,-15.0173072536014,26.0107391561104));
#36266=CARTESIAN_POINT('Ctrl Pts',(8.45435372222587,-41.0280464097118,10.9934319025089));
#36267=CARTESIAN_POINT('Ctrl Pts',(8.45435372222587,-26.0107391561104,-15.0173072536014));
#36268=CARTESIAN_POINT('Ctrl Pts',(8.45435372222587,-11.6489491721889,-39.8926571933874));
#36269=CARTESIAN_POINT('Ctrl Pts',(8.45435372222587,13.8422173352291,-26.6546635289318));
#36270=CARTESIAN_POINT('Ctrl Pts',(7.67514864245731,13.8337516775665,-26.6383620035993));
#36271=CARTESIAN_POINT('Ctrl Pts',(7.67514864245731,14.4281166503283,-26.3296982262275));
#36272=CARTESIAN_POINT('Ctrl Pts',(7.67514864245731,15.0081229315276,-25.9948314436454));
#36273=CARTESIAN_POINT('Ctrl Pts',(7.67514864245731,41.0029543751729,-10.9867085121178));
#36274=CARTESIAN_POINT('Ctrl Pts',(7.67514864245731,25.9948314436454,15.0081229315276));
#36275=CARTESIAN_POINT('Ctrl Pts',(7.67514864245731,10.9867085121178,41.0029543751729));
#36276=CARTESIAN_POINT('Ctrl Pts',(7.67514864245731,-15.0081229315276,25.9948314436454));
#36277=CARTESIAN_POINT('Ctrl Pts',(7.67514864245731,-41.0029543751729,10.9867085121178));
#36278=CARTESIAN_POINT('Ctrl Pts',(7.67514864245731,-25.9948314436454,-15.0081229315276));
#36279=CARTESIAN_POINT('Ctrl Pts',(7.67514864245731,-11.6418248789176,-39.8682595430057));
#36280=CARTESIAN_POINT('Ctrl Pts',(7.67514864245731,13.8337516775665,-26.6383620035993));
#36281=CARTESIAN_POINT('Ctrl Pts',(7.15799654185577,13.8286669632852,-26.6285708447822));
#36282=CARTESIAN_POINT('Ctrl Pts',(7.15799654185577,14.4228134720947,-26.3200205194336));
#36283=CARTESIAN_POINT('Ctrl Pts',(7.15799654185577,15.0026065670022,-25.9852768200144));
#36284=CARTESIAN_POINT('Ctrl Pts',(7.15799654185577,40.9878833870167,-10.9826702530122));
#36285=CARTESIAN_POINT('Ctrl Pts',(7.15799654185577,25.9852768200144,15.0026065670022));
#36286=CARTESIAN_POINT('Ctrl Pts',(7.15799654185577,10.9826702530122,40.9878833870167));
#36287=CARTESIAN_POINT('Ctrl Pts',(7.15799654185577,-15.0026065670022,25.9852768200144));
#36288=CARTESIAN_POINT('Ctrl Pts',(7.15799654185577,-40.9878833870167,10.9826702530122));
#36289=CARTESIAN_POINT('Ctrl Pts',(7.15799654185577,-25.9852768200144,-15.0026065670022));
#36290=CARTESIAN_POINT('Ctrl Pts',(7.15799654185577,-11.637545826163,-39.8536056216838));
#36291=CARTESIAN_POINT('Ctrl Pts',(7.15799654185577,13.8286669632852,-26.6285708447822));
#36292=CARTESIAN_POINT('Ctrl Pts',(6.9,13.8262643576559,-26.6239443717909));
#36293=CARTESIAN_POINT('Ctrl Pts',(6.9,14.4203076388911,-26.3154476542665));
#36294=CARTESIAN_POINT('Ctrl Pts',(6.9,15.,-25.9807621135332));
#36295=CARTESIAN_POINT('Ctrl Pts',(6.9,40.9807621135331,-10.9807621135332));
#36296=CARTESIAN_POINT('Ctrl Pts',(6.9,25.9807621135332,15.));
#36297=CARTESIAN_POINT('Ctrl Pts',(6.9,10.9807621135332,40.9807621135331));
#36298=CARTESIAN_POINT('Ctrl Pts',(6.9,-15.,25.9807621135332));
#36299=CARTESIAN_POINT('Ctrl Pts',(6.9,-40.9807621135331,10.9807621135332));
#36300=CARTESIAN_POINT('Ctrl Pts',(6.9,-25.9807621135332,-15.));
#36301=CARTESIAN_POINT('Ctrl Pts',(6.9,-11.6355239079848,-39.846681418688));
#36302=CARTESIAN_POINT('Ctrl Pts',(6.9,13.8262643576559,-26.6239443717909));
#36303=CARTESIAN_POINT('Ctrl Pts',(6.9,29.194404870986,-6.90555748864274));
#36304=CARTESIAN_POINT('Ctrl Pts',(7.85773098116326,28.7583591297181,-8.83308608050288));
#36305=CARTESIAN_POINT('Ctrl Pts',(8.88781981167334,28.148927360677,-10.6725495024415));
#36306=CARTESIAN_POINT('Ctrl Pts',(10.5914578196776,26.9549567714738,-13.4378975079049));
#36307=CARTESIAN_POINT('Ctrl Pts',(11.2365058953701,26.4627511078989,-14.4268759573926));
#36308=CARTESIAN_POINT('Ctrl Pts',(12.0558885382926,25.8276163596339,-15.5639851987506));
#36309=CARTESIAN_POINT('Ctrl Pts',(12.1875764958397,25.7255677072203,-15.7427052651201));
#36310=CARTESIAN_POINT('Ctrl Pts',(13.194901830313,24.9407551262717,-17.0880993664927));
#36311=CARTESIAN_POINT('Ctrl Pts',(14.2258982134098,24.0748117650461,-18.4224696507577));
#36312=CARTESIAN_POINT('Ctrl Pts',(18.2616480823244,20.9914735836847,-22.4465505568645));
#36313=CARTESIAN_POINT('Ctrl Pts',(21.0496416709525,19.1084188222497,-24.4970863377161));
#36314=CARTESIAN_POINT('Ctrl Pts',(25.8000196361138,18.0798601480504,-27.4404163303281));
#36315=CARTESIAN_POINT('Ctrl Pts',(26.8976561124457,18.1725012311874,-27.9949084025612));
#36316=CARTESIAN_POINT('Ctrl Pts',(28.0045908801237,18.293020318403,-28.5110480063609));
#36317=CARTESIAN_POINT('Ctrl Pts',(28.5235971652406,18.3760345677215,-28.7375730360626));
#36318=CARTESIAN_POINT('Ctrl Pts',(29.0834839543824,18.4629109750536,-28.9821227669885));
#36319=CARTESIAN_POINT('Ctrl Pts',(29.1146288039499,18.4676985487665,-28.995750541561));
#36320=CARTESIAN_POINT('Ctrl Pts',(29.5949306848436,18.5426905181124,-29.2050975774362));
#36321=CARTESIAN_POINT('Ctrl Pts',(30.0492939924726,18.6372599535756,-29.3870260594868));
#36322=CARTESIAN_POINT('Ctrl Pts',(30.5,18.7405179110273,-29.559989655385));
#36323=CARTESIAN_POINT('Ctrl Pts',(6.45331003273164,10.9133179225515,-1.5966967862278));
#36324=CARTESIAN_POINT('Ctrl Pts',(7.20830533428676,10.8283039351861,-2.16272621042871));
#36325=CARTESIAN_POINT('Ctrl Pts',(7.9992896214032,10.7080816105349,-2.70879554626308));
#36326=CARTESIAN_POINT('Ctrl Pts',(9.76164489174097,10.3736775708918,-3.82718122480733));
#36327=CARTESIAN_POINT('Ctrl Pts',(10.7316587814816,10.1362456656108,-4.40082635509405));
#36328=CARTESIAN_POINT('Ctrl Pts',(12.6606926111663,9.65961205419966,-5.38563263712134));
#36329=CARTESIAN_POINT('Ctrl Pts',(13.6374431259541,9.3836045062609,-5.83915384029437));
#36330=CARTESIAN_POINT('Ctrl Pts',(14.8679539417017,9.06165302613705,-6.32358226998234));
#36331=CARTESIAN_POINT('Ctrl Pts',(15.8146186835335,8.80867695163279,-6.68453209751777));
#36332=CARTESIAN_POINT('Ctrl Pts',(16.7768279789011,8.55011854625628,-7.00516941257107));
#36333=CARTESIAN_POINT('Ctrl Pts',(18.4426549461008,8.1453397293125,-7.48808598435162));
#36334=CARTESIAN_POINT('Ctrl Pts',(19.4151948753425,7.90738588441818,-7.72973898022664));
#36335=CARTESIAN_POINT('Ctrl Pts',(20.6328868119181,7.66437297695763,-7.97443640583051));
#36336=CARTESIAN_POINT('Ctrl Pts',(21.1054260060183,7.57098863237654,-8.06465516156995));
#36337=CARTESIAN_POINT('Ctrl Pts',(22.0544239964404,7.3938759247956,-8.2283193842106));
#36338=CARTESIAN_POINT('Ctrl Pts',(22.7836594350108,7.27389266543009,-8.33397294082305));
#36339=CARTESIAN_POINT('Ctrl Pts',(23.5025637456199,7.17270583388441,-8.42426711082584));
#36340=CARTESIAN_POINT('Ctrl Pts',(23.9756232708723,7.10861034193422,-8.47952646912202));
#36341=CARTESIAN_POINT('Ctrl Pts',(24.5702383273706,7.0366668150329,-8.53935462310067));
#36342=CARTESIAN_POINT('Ctrl Pts',(25.0506812637274,6.98463603831044,-8.58189400875826));
#36343=CARTESIAN_POINT('Ctrl Pts',(25.4117237717361,6.94891133994683,-8.61093616318041));
#36344=CARTESIAN_POINT('Ctrl Pts',(25.7132331301504,6.92207219011195,-8.63276690479072));
#36345=CARTESIAN_POINT('Ctrl Pts',(25.9243500189533,6.90499555217197,-8.64675417662519));
#36346=CARTESIAN_POINT('Ctrl Pts',(26.04498253513,6.8957416597317,-8.65437719289208));
#36347=CARTESIAN_POINT('Ctrl Pts',(26.1053107047426,6.89128602190947,-8.65806460962785));
#36348=CARTESIAN_POINT('Ctrl Pts',(26.5982868813553,6.85557010312579,-8.68771831234618));
#36349=CARTESIAN_POINT('Ctrl Pts',(27.5414448539111,6.81230249083073,-8.72222386822166));
#36350=CARTESIAN_POINT('Ctrl Pts',(28.5384718269742,6.79157348079194,-8.73742874004834));
#36351=CARTESIAN_POINT('Ctrl Pts',(29.1235718011008,6.77903979219481,-8.7472765876331));
#36352=CARTESIAN_POINT('Ctrl Pts',(29.2812925824006,6.77610142826279,-8.74962231400043));
#36353=CARTESIAN_POINT('Ctrl Pts',(29.6033746665994,6.77163194910156,-8.75316560056394));
#36354=CARTESIAN_POINT('Ctrl Pts',(30.1682156581424,6.76749797708616,-8.75644680260437));
#36355=CARTESIAN_POINT('Ctrl Pts',(31.3151120085297,6.77048174742384,-8.75407681716332));
#36356=CARTESIAN_POINT('Ctrl Pts',(32.3203490755538,6.7812704666075,-8.74562733267071));
#36357=CARTESIAN_POINT('Ctrl Pts',(33.1676615322705,6.78128357449773,-8.74562186943981));
#36358=CARTESIAN_POINT('Ctrl Pts',(33.4948723279892,6.78128505761789,-8.74562133595163));
#36359=CARTESIAN_POINT('Ctrl Pts',(34.1541357431674,6.78128770533515,-8.74562028433962));
#36360=CARTESIAN_POINT('Ctrl Pts',(34.9760826079902,6.78129612595835,-8.74561702798974));
#36361=CARTESIAN_POINT('Ctrl Pts',(35.963684548769,6.78129958330348,-8.74561567977426));
#36362=CARTESIAN_POINT('Ctrl Pts',(37.9383132355671,6.78130435924946,-8.74561382885196));
#36363=CARTESIAN_POINT('Ctrl Pts',(39.5833333333333,6.7813280023926,-8.74560464293356));
#36364=CARTESIAN_POINT('Ctrl Pts',(40.9,6.7813280023926,-8.74560464293356));
#36365=CARTESIAN_POINT('Ctrl Pts',(6.63336813585096,14.1980521881427,-2.58998912169034));
#36366=CARTESIAN_POINT('Ctrl Pts',(7.389696336477,14.0595388287459,-3.32655463912723));
#36367=CARTESIAN_POINT('Ctrl Pts',(8.18035160561763,13.8764440634215,-4.03465273479122));
#36368=CARTESIAN_POINT('Ctrl Pts',(9.94163143861869,13.3869575789582,-5.47986851886094));
#36369=CARTESIAN_POINT('Ctrl Pts',(10.9109664605568,13.0495988183286,-6.21859686207518));
#36370=CARTESIAN_POINT('Ctrl Pts',(12.8334013836927,12.3824387994051,-7.47915893423736));
#36371=CARTESIAN_POINT('Ctrl Pts',(13.8089179831182,12.0008911509523,-8.05904353786121));
#36372=CARTESIAN_POINT('Ctrl Pts',(15.0306778911272,11.5604290689694,-8.67329495695319));
#36373=CARTESIAN_POINT('Ctrl Pts',(15.9745670647921,11.2141745075894,-9.13243737556313));
#36374=CARTESIAN_POINT('Ctrl Pts',(16.9295440841728,10.8635736365945,-9.53704617981301));
#36375=CARTESIAN_POINT('Ctrl Pts',(18.5792362231984,10.3171018918724,-10.1451076803253));
#36376=CARTESIAN_POINT('Ctrl Pts',(19.5469773926754,9.99640408637909,-10.4493242965116));
#36377=CARTESIAN_POINT('Ctrl Pts',(20.7474295734273,9.67172058444851,-10.7549000186159));
#36378=CARTESIAN_POINT('Ctrl Pts',(21.216779417289,9.54637190554464,-10.8681544802445));
#36379=CARTESIAN_POINT('Ctrl Pts',(22.154984393846,9.30976886072804,-11.0724642143301));
#36380=CARTESIAN_POINT('Ctrl Pts',(22.8744776078262,9.1499657882767,-11.2039970972492));
#36381=CARTESIAN_POINT('Ctrl Pts',(23.5816077902756,9.01558422395398,-11.3162019466946));
#36382=CARTESIAN_POINT('Ctrl Pts',(24.0500749276258,8.93008359351409,-11.3851612528791));
#36383=CARTESIAN_POINT('Ctrl Pts',(24.6365533946119,8.83449183240002,-11.459465225808));
#36384=CARTESIAN_POINT('Ctrl Pts',(25.1102835291681,8.76539275960603,-11.5122699159727));
#36385=CARTESIAN_POINT('Ctrl Pts',(25.4658322439322,8.71801358900114,-11.548268841707));
#36386=CARTESIAN_POINT('Ctrl Pts',(25.7624874136677,8.68244638509912,-11.575318037023));
#36387=CARTESIAN_POINT('Ctrl Pts',(25.9700349923404,8.65983585467406,-11.5926401638755));
#36388=CARTESIAN_POINT('Ctrl Pts',(26.0885791323121,8.64758737376027,-11.6020803597249));
#36389=CARTESIAN_POINT('Ctrl Pts',(26.1478525996396,8.64169115913832,-11.6066467500377));
#36390=CARTESIAN_POINT('Ctrl Pts',(26.6319130667255,8.59444428954191,-11.6433645250352));
#36391=CARTESIAN_POINT('Ctrl Pts',(27.5577774489361,8.53717709311563,-11.686082476889));
#36392=CARTESIAN_POINT('Ctrl Pts',(28.5508423746852,8.50942828058708,-11.705090826));
#36393=CARTESIAN_POINT('Ctrl Pts',(29.1362159539418,8.49263545125878,-11.7174369518244));
#36394=CARTESIAN_POINT('Ctrl Pts',(29.2912819508837,8.48875007883402,-11.7203386713974));
#36395=CARTESIAN_POINT('Ctrl Pts',(29.6100529981865,8.48280581727715,-11.7247475094469));
#36396=CARTESIAN_POINT('Ctrl Pts',(30.1693026775043,8.47731190452081,-11.7288279027908));
#36397=CARTESIAN_POINT('Ctrl Pts',(31.3098786008459,8.48127083805319,-11.7258872894479));
#36398=CARTESIAN_POINT('Ctrl Pts',(32.316282704888,8.49575357359979,-11.7152777874897));
#36399=CARTESIAN_POINT('Ctrl Pts',(33.1686195735694,8.49577523975594,-11.7152690782769));
#36400=CARTESIAN_POINT('Ctrl Pts',(33.4952188807556,8.49577770055105,-11.7152682401722));
#36401=CARTESIAN_POINT('Ctrl Pts',(34.154773424404,8.49578208271189,-11.7152665713231));
#36402=CARTESIAN_POINT('Ctrl Pts',(34.9764178792929,8.49579602915739,-11.7152614171756));
#36403=CARTESIAN_POINT('Ctrl Pts',(35.964052055092,8.4958017540615,-11.7152592814564));
#36404=CARTESIAN_POINT('Ctrl Pts',(37.9385651163986,8.49580966365995,-11.7152563511876));
#36405=CARTESIAN_POINT('Ctrl Pts',(39.5833333333333,8.49584881729846,-11.7152418049849));
#36406=CARTESIAN_POINT('Ctrl Pts',(40.9,8.49584881729846,-11.7152418049849));
#36407=CARTESIAN_POINT('Ctrl Pts',(6.84648239176542,21.8719108775553,-4.87117200494631));
#36408=CARTESIAN_POINT('Ctrl Pts',(7.61278097593421,21.6080942034255,-6.01809391809558));
#36409=CARTESIAN_POINT('Ctrl Pts',(8.41274152921386,21.2759544371052,-7.1129769401534));
#36410=CARTESIAN_POINT('Ctrl Pts',(10.1879716557546,20.4198986989574,-9.33526598964861));
#36411=CARTESIAN_POINT('Ctrl Pts',(11.1642573475929,19.8462357742843,-10.4645258845954));
#36412=CARTESIAN_POINT('Ctrl Pts',(13.1034321172788,18.7228640453273,-12.3837514736036));
#36413=CARTESIAN_POINT('Ctrl Pts',(14.0822646095709,18.0925354910949,-13.259092905625));
#36414=CARTESIAN_POINT('Ctrl Pts',(15.3084001581866,17.369341405527,-14.1807147676624));
#36415=CARTESIAN_POINT('Ctrl Pts',(16.2531227144981,16.8032299545451,-14.8695159890907));
#36416=CARTESIAN_POINT('Ctrl Pts',(17.2084375604976,16.2348330754282,-15.4708786153411));
#36417=CARTESIAN_POINT('Ctrl Pts',(18.8473961588576,15.3570672461536,-16.3684102669436));
#36418=CARTESIAN_POINT('Ctrl Pts',(19.8110405035778,14.8437940564495,-16.8164458459156));
#36419=CARTESIAN_POINT('Ctrl Pts',(20.9872655006156,14.3329359049564,-17.2594998647321));
#36420=CARTESIAN_POINT('Ctrl Pts',(21.451734623773,14.1338378277509,-17.4254488483259));
#36421=CARTESIAN_POINT('Ctrl Pts',(22.372798484146,13.7614448137585,-17.7217491293397));
#36422=CARTESIAN_POINT('Ctrl Pts',(23.0743543377555,13.5118529399619,-17.9111527143531));
#36423=CARTESIAN_POINT('Ctrl Pts',(23.7582742987057,13.3034745440376,-18.0719640430557));
#36424=CARTESIAN_POINT('Ctrl Pts',(24.2174386855888,13.1693266480663,-18.1719103336472));
#36425=CARTESIAN_POINT('Ctrl Pts',(24.787021394358,13.0207037868377,-18.2785218143403));
#36426=CARTESIAN_POINT('Ctrl Pts',(25.2463470121627,12.9133861579979,-18.3542161979467));
#36427=CARTESIAN_POINT('Ctrl Pts',(25.5899787396412,12.8400372670535,-18.4056632423981));
#36428=CARTESIAN_POINT('Ctrl Pts',(25.8759048428216,12.7850917865301,-18.4442660174715));
#36429=CARTESIAN_POINT('Ctrl Pts',(26.0755068065021,12.750236170981,-18.4689567859635));
#36430=CARTESIAN_POINT('Ctrl Pts',(26.1893780149121,12.7313725692324,-18.4824083304406));
#36431=CARTESIAN_POINT('Ctrl Pts',(26.2462863876012,12.722296957459,-18.4889145361413));
#36432=CARTESIAN_POINT('Ctrl Pts',(26.7102722067264,12.6496548741733,-18.5411896593424));
#36433=CARTESIAN_POINT('Ctrl Pts',(27.596090538688,12.5614420302552,-18.6020458648117));
#36434=CARTESIAN_POINT('Ctrl Pts',(28.5798438027281,12.5173520665106,-18.6298999603236));
#36435=CARTESIAN_POINT('Ctrl Pts',(29.1658297917573,12.4906249890437,-18.6480680632811));
#36436=CARTESIAN_POINT('Ctrl Pts',(29.3147155528133,12.4846522276653,-18.6521962493028));
#36437=CARTESIAN_POINT('Ctrl Pts',(29.6257654938386,12.4753713397179,-18.658563739707));
#36438=CARTESIAN_POINT('Ctrl Pts',(30.1719616098273,12.4668129248997,-18.6644443298451));
#36439=CARTESIAN_POINT('Ctrl Pts',(31.297773841033,12.4729611884878,-18.6602190141084));
#36440=CARTESIAN_POINT('Ctrl Pts',(32.3068669150105,12.4961463862895,-18.6445149503824));
#36441=CARTESIAN_POINT('Ctrl Pts',(33.170912704073,12.4962026881971,-18.6444874715364));
#36442=CARTESIAN_POINT('Ctrl Pts',(33.4960830255431,12.4962093123003,-18.6444844180378));
#36443=CARTESIAN_POINT('Ctrl Pts',(34.156313582216,12.4962208405722,-18.6444789016082));
#36444=CARTESIAN_POINT('Ctrl Pts',(34.9772414248896,12.4962577684094,-18.6444614154563));
#36445=CARTESIAN_POINT('Ctrl Pts',(35.9649463721128,12.4962728966389,-18.6444542286037));
#36446=CARTESIAN_POINT('Ctrl Pts',(37.9391834323221,12.4962938290756,-18.6444443083028));
#36447=CARTESIAN_POINT('Ctrl Pts',(39.5833333333333,12.4963973854121,-18.6443951831047));
#36448=CARTESIAN_POINT('Ctrl Pts',(40.9,12.4963973854121,-18.6443951831047));
#36449=CARTESIAN_POINT('Ctrl Pts',(6.90857970435318,29.5800408844791,-7.02038826853571));
#36450=CARTESIAN_POINT('Ctrl Pts',(7.67983757144493,29.1962153577801,-8.5857790108899));
#36451=CARTESIAN_POINT('Ctrl Pts',(8.48446296596919,28.7191114013952,-10.0765485557758));
#36452=CARTESIAN_POINT('Ctrl Pts',(10.2687526859613,27.5023711977385,-13.0935628879538));
#36453=CARTESIAN_POINT('Ctrl Pts',(11.2489627292759,26.6949552438923,-14.6224501564806));
#36454=CARTESIAN_POINT('Ctrl Pts',(13.2065810728343,25.1069038454382,-17.2294066625499));
#36455=CARTESIAN_POINT('Ctrl Pts',(14.1884325798659,24.2271697832518,-18.406995285395));
#36456=CARTESIAN_POINT('Ctrl Pts',(15.4296983589675,23.2080338536348,-19.6550892131211));
#36457=CARTESIAN_POINT('Ctrl Pts',(16.3788042670986,22.4189011948388,-20.5796860932724));
#36458=CARTESIAN_POINT('Ctrl Pts',(17.3450159165717,21.621722459271,-21.3903231452906));
#36459=CARTESIAN_POINT('Ctrl Pts',(18.999996264546,20.3951481814248,-22.5937460627633));
#36460=CARTESIAN_POINT('Ctrl Pts',(19.9686658165162,19.6835411202357,-23.1898054127386));
#36461=CARTESIAN_POINT('Ctrl Pts',(21.1489437168837,18.9783964629484,-23.7756910485746));
#36462=CARTESIAN_POINT('Ctrl Pts',(21.6136662410163,18.7043064424583,-23.9949385633149));
#36463=CARTESIAN_POINT('Ctrl Pts',(22.5341605437878,18.1932305660764,-24.384652173758));
#36464=CARTESIAN_POINT('Ctrl Pts',(23.2310352415758,17.8537326154784,-24.6315178872705));
#36465=CARTESIAN_POINT('Ctrl Pts',(23.9047680627604,17.5731511638348,-24.8394315921362));
#36466=CARTESIAN_POINT('Ctrl Pts',(24.3593217251587,17.3912549800687,-24.9695871891295));
#36467=CARTESIAN_POINT('Ctrl Pts',(24.9191284505002,17.1917285847403,-25.1069751863352));
#36468=CARTESIAN_POINT('Ctrl Pts',(25.3687829483019,17.0482631873588,-25.2041659752928));
#36469=CARTESIAN_POINT('Ctrl Pts',(25.7038809466233,16.9507036504238,-25.2699171894914));
#36470=CARTESIAN_POINT('Ctrl Pts',(25.9815275275372,16.8779731233099,-25.3190677310916));
#36471=CARTESIAN_POINT('Ctrl Pts',(26.17472557473,16.8320233777005,-25.350412411697));
#36472=CARTESIAN_POINT('Ctrl Pts',(26.2847430019933,16.8072090098448,-25.3674660195519));
#36473=CARTESIAN_POINT('Ctrl Pts',(26.3396756125245,16.795284989838,-25.3757090167846));
#36474=CARTESIAN_POINT('Ctrl Pts',(26.7867185605541,16.7000344271693,-25.4418392909468));
#36475=CARTESIAN_POINT('Ctrl Pts',(27.6343089133545,16.5847364280859,-25.5185659559037));
#36476=CARTESIAN_POINT('Ctrl Pts',(28.6086204191326,16.524382058732,-25.555224257615));
#36477=CARTESIAN_POINT('Ctrl Pts',(29.1952293795944,16.4877244301022,-25.5792110357042));
#36478=CARTESIAN_POINT('Ctrl Pts',(29.3380035933314,16.4799452423706,-25.5844033272726));
#36479=CARTESIAN_POINT('Ctrl Pts',(29.6413717635317,16.467569571443,-25.5925899885787));
#36480=CARTESIAN_POINT('Ctrl Pts',(30.1745368065166,16.456196787226,-25.6001268754991));
#36481=CARTESIAN_POINT('Ctrl Pts',(31.2855894033319,16.4643300419838,-25.594734665506));
#36482=CARTESIAN_POINT('Ctrl Pts',(32.2974015084452,16.4964013295027,-25.5738307704498));
#36483=CARTESIAN_POINT('Ctrl Pts',(33.173165111218,16.4965224425525,-25.5737672879572));
#36484=CARTESIAN_POINT('Ctrl Pts',(33.4969081472869,16.4965369996127,-25.5737598716198));
#36485=CARTESIAN_POINT('Ctrl Pts',(34.1578169391037,16.4965619872357,-25.5737469053192));
#36486=CARTESIAN_POINT('Ctrl Pts',(34.9780359591177,16.4966423446109,-25.5737054251285));
#36487=CARTESIAN_POINT('Ctrl Pts',(35.9658147840132,16.4966752246751,-25.5736884251094));
#36488=CARTESIAN_POINT('Ctrl Pts',(37.939780228271,16.4967207607425,-25.5736649097448));
#36489=CARTESIAN_POINT('Ctrl Pts',(39.5833333333333,16.4969459535258,-25.5735485612246));
#36490=CARTESIAN_POINT('Ctrl Pts',(40.9,16.4969459535258,-25.5735485612246));
#36491=CARTESIAN_POINT('Ctrl Pts',(6.93528330520032,33.9890447223856,-8.23173028337902));
#36492=CARTESIAN_POINT('Ctrl Pts',(7.70864561497005,33.5376786188307,-10.0357116563145));
#36493=CARTESIAN_POINT('Ctrl Pts',(8.51532719250786,32.9786927413523,-11.7528338486872));
#36494=CARTESIAN_POINT('Ctrl Pts',(10.3033707684643,31.5578840442132,-15.2242195800702));
#36495=CARTESIAN_POINT('Ctrl Pts',(11.285359425586,30.6179424293771,-16.9818886494149));
#36496=CARTESIAN_POINT('Ctrl Pts',(13.2503075123955,28.7660858779662,-19.9828238609275));
#36497=CARTESIAN_POINT('Ctrl Pts',(14.2335802328307,27.7445903826109,-21.333808720003));
#36498=CARTESIAN_POINT('Ctrl Pts',(15.4809874764708,26.5562215055806,-22.7701484639683));
#36499=CARTESIAN_POINT('Ctrl Pts',(16.4318967140332,25.6398645222147,-23.8303538982283));
#36500=CARTESIAN_POINT('Ctrl Pts',(17.402786088206,24.711406834453,-24.7620955812503));
#36501=CARTESIAN_POINT('Ctrl Pts',(19.0657008739462,23.2827894621992,-26.143876791427));
#36502=CARTESIAN_POINT('Ctrl Pts',(20.0370987955261,22.4568785783622,-26.8257745442824));
#36503=CARTESIAN_POINT('Ctrl Pts',(21.2219373681816,21.6368752952078,-27.4963832022119));
#36504=CARTESIAN_POINT('Ctrl Pts',(21.6873545199144,21.3192655757677,-27.7466423667123));
#36505=CARTESIAN_POINT('Ctrl Pts',(22.6095407883912,20.7266792263563,-28.1914275999314));
#36506=CARTESIAN_POINT('Ctrl Pts',(23.3063195468715,20.3342063552496,-28.4721721598027));
#36507=CARTESIAN_POINT('Ctrl Pts',(23.9774915837894,20.0111563083461,-28.7077527668373));
#36508=CARTESIAN_POINT('Ctrl Pts',(24.4307021142568,19.8016082531837,-28.8553793495029));
#36509=CARTESIAN_POINT('Ctrl Pts',(24.9871188326855,19.5726095610114,-29.0105626137829));
#36510=CARTESIAN_POINT('Ctrl Pts',(25.4329141726807,19.4084486444517,-29.1200357132456));
#36511=CARTESIAN_POINT('Ctrl Pts',(25.764395055469,19.2971155191101,-29.1939083663015));
#36512=CARTESIAN_POINT('Ctrl Pts',(26.0382972138567,19.2143910494167,-29.248971810693));
#36513=CARTESIAN_POINT('Ctrl Pts',(26.2284820979125,19.1622606931663,-29.2840172105118));
#36514=CARTESIAN_POINT('Ctrl Pts',(26.3366494455053,19.134150744928,-29.3030632173385));
#36515=CARTESIAN_POINT('Ctrl Pts',(26.3906225284356,19.120654372709,-29.3122642693055));
#36516=CARTESIAN_POINT('Ctrl Pts',(26.8293654116024,19.0129885834585,-29.3859982106881));
#36517=CARTESIAN_POINT('Ctrl Pts',(27.6560988760138,18.8833816200188,-29.4710985842859));
#36518=CARTESIAN_POINT('Ctrl Pts',(28.6249317030313,18.8137794716611,-29.5127595133991));
#36519=CARTESIAN_POINT('Ctrl Pts',(29.2119052185268,18.7714558506411,-29.5400636810172));
#36520=CARTESIAN_POINT('Ctrl Pts',(29.3512234939535,18.7627335234212,-29.5458124634019));
#36521=CARTESIAN_POINT('Ctrl Pts',(29.6502234545146,18.7486685476096,-29.5549926880428));
#36522=CARTESIAN_POINT('Ctrl Pts',(30.1759548990661,18.7357718416963,-29.5634265890416));
#36523=CARTESIAN_POINT('Ctrl Pts',(31.2785766862297,18.7449771625328,-29.5574021311853));
#36524=CARTESIAN_POINT('Ctrl Pts',(32.2919610610306,18.7821959068191,-29.5334837411521));
#36525=CARTESIAN_POINT('Ctrl Pts',(33.1744263360523,18.7823679845322,-29.5333904072538));
#36526=CARTESIAN_POINT('Ctrl Pts',(33.4973548461806,18.782388929425,-29.5333792377696));
#36527=CARTESIAN_POINT('Ctrl Pts',(34.1586526208333,18.7824245927185,-29.5333600113091));
#36528=CARTESIAN_POINT('Ctrl Pts',(34.9784715438078,18.7825395490481,-29.5332982308029));
#36529=CARTESIAN_POINT('Ctrl Pts',(35.9662945600332,18.7825865524219,-29.5332729456426));
#36530=CARTESIAN_POINT('Ctrl Pts',(37.9401075800397,18.7826516826342,-29.5332379342859));
#36531=CARTESIAN_POINT('Ctrl Pts',(39.5833333333333,18.7829737067336,-29.533064777293));
#36532=CARTESIAN_POINT('Ctrl Pts',(40.9,18.7829737067336,-29.533064777293));
#36533=CARTESIAN_POINT('Origin',(6.9,-5.51091059616309E-15,-30.));
#36534=CARTESIAN_POINT('',(6.9,21.8303175223207,-20.5775906479515));
#36535=CARTESIAN_POINT('Ctrl Pts',(6.9,8.44145532612415,-7.09789564133157));
#36536=CARTESIAN_POINT('Ctrl Pts',(6.9,11.09468188726,-9.87986401752105));
#36537=CARTESIAN_POINT('Ctrl Pts',(6.90000000166257,13.9485622548227,-12.753513475675));
#36538=CARTESIAN_POINT('Ctrl Pts',(6.90000000166257,18.0885125115534,-16.8843019432417));
#36539=CARTESIAN_POINT('Ctrl Pts',(6.9,19.9691972794379,-18.7449692586141));
#36540=CARTESIAN_POINT('Ctrl Pts',(6.9,21.8303175223207,-20.5775906479515));
#36541=CARTESIAN_POINT('Origin',(6.9,0.,0.));
#36542=CARTESIAN_POINT('Origin',(40.9,-1.65327317884893E-15,-9.));
#36543=CARTESIAN_POINT('Ctrl Pts',(40.9,1.5,-34.4673758792282));
#36544=CARTESIAN_POINT('Ctrl Pts',(40.9,1.5,-33.9668810740701));
#36545=CARTESIAN_POINT('Ctrl Pts',(40.9,1.49999999999999,-33.466386268912));
#36546=CARTESIAN_POINT('Ctrl Pts',(40.9,1.5,-32.9658914637539));
#36547=CARTESIAN_POINT('Ctrl Pts',(30.5,-1.56108868151375,-34.9651684126997));
#36548=CARTESIAN_POINT('Ctrl Pts',(30.5,-0.780932928377886,-35.));
#36549=CARTESIAN_POINT('Ctrl Pts',(30.5,-6.4293956955236E-15,-35.));
#36550=CARTESIAN_POINT('Ctrl Pts',(30.5,35.,-35.));
#36551=CARTESIAN_POINT('Ctrl Pts',(30.5,35.,-6.4293956955236E-15));
#36552=CARTESIAN_POINT('Ctrl Pts',(30.5,35.,35.));
#36553=CARTESIAN_POINT('Ctrl Pts',(30.5,6.4293956955236E-15,35.));
#36554=CARTESIAN_POINT('Ctrl Pts',(30.5,-35.,35.));
#36555=CARTESIAN_POINT('Ctrl Pts',(30.5,-35.,6.4293956955236E-15));
#36556=CARTESIAN_POINT('Ctrl Pts',(30.5,-35.,-33.472222479613));
#36557=CARTESIAN_POINT('Ctrl Pts',(30.5,-1.56108868151375,-34.9651684126997));
#36558=CARTESIAN_POINT('Ctrl Pts',(30.3311478274255,-1.55772383604588,-34.8898028105656));
#36559=CARTESIAN_POINT('Ctrl Pts',(30.3311478274255,-0.779249668063541,
-34.924559320191));
#36560=CARTESIAN_POINT('Ctrl Pts',(30.3311478274255,-6.41553746746556E-15,
-34.924559320191));
#36561=CARTESIAN_POINT('Ctrl Pts',(30.3311478274255,34.924559320191,-34.924559320191));
#36562=CARTESIAN_POINT('Ctrl Pts',(30.3311478274255,34.924559320191,-6.41553746746556E-15));
#36563=CARTESIAN_POINT('Ctrl Pts',(30.3311478274255,34.924559320191,34.924559320191));
#36564=CARTESIAN_POINT('Ctrl Pts',(30.3311478274255,6.41553746746556E-15,
34.924559320191));
#36565=CARTESIAN_POINT('Ctrl Pts',(30.3311478274255,-34.924559320191,34.924559320191));
#36566=CARTESIAN_POINT('Ctrl Pts',(30.3311478274255,-34.924559320191,6.41553746746556E-15));
#36567=CARTESIAN_POINT('Ctrl Pts',(30.3311478274255,-34.924559320191,-33.4000748447964));
#36568=CARTESIAN_POINT('Ctrl Pts',(30.3311478274255,-1.55772383604588,-34.8898028105656));
#36569=CARTESIAN_POINT('Ctrl Pts',(29.9897712690917,-1.55090794481747,-34.7371408974366));
#36570=CARTESIAN_POINT('Ctrl Pts',(29.9897712690917,-0.775840025831463,
-34.7717453283792));
#36571=CARTESIAN_POINT('Ctrl Pts',(29.9897712690917,-6.38746599257497E-15,
-34.7717453283792));
#36572=CARTESIAN_POINT('Ctrl Pts',(29.9897712690917,34.7717453283791,-34.7717453283791));
#36573=CARTESIAN_POINT('Ctrl Pts',(29.9897712690917,34.7717453283792,-6.38746599257497E-15));
#36574=CARTESIAN_POINT('Ctrl Pts',(29.9897712690917,34.7717453283791,34.7717453283791));
#36575=CARTESIAN_POINT('Ctrl Pts',(29.9897712690917,6.38746599257497E-15,
34.7717453283792));
#36576=CARTESIAN_POINT('Ctrl Pts',(29.9897712690917,-34.7717453283791,34.7717453283791));
#36577=CARTESIAN_POINT('Ctrl Pts',(29.9897712690917,-34.7717453283792,6.38746599257497E-15));
#36578=CARTESIAN_POINT('Ctrl Pts',(29.9897712690917,-34.7717453283791,-33.2539313038843));
#36579=CARTESIAN_POINT('Ctrl Pts',(29.9897712690917,-1.55090794481747,-34.7371408974366));
#36580=CARTESIAN_POINT('Ctrl Pts',(29.4666899049319,-1.54042548027395,-34.5023553003819));
#36581=CARTESIAN_POINT('Ctrl Pts',(29.4666899049319,-0.770596184255049,
-34.5367258427036));
#36582=CARTESIAN_POINT('Ctrl Pts',(29.4666899049319,-6.34429361344449E-15,
-34.5367258427036));
#36583=CARTESIAN_POINT('Ctrl Pts',(29.4666899049319,34.5367258427036,-34.5367258427036));
#36584=CARTESIAN_POINT('Ctrl Pts',(29.4666899049319,34.5367258427036,-6.34429361344449E-15));
#36585=CARTESIAN_POINT('Ctrl Pts',(29.4666899049319,34.5367258427036,34.5367258427036));
#36586=CARTESIAN_POINT('Ctrl Pts',(29.4666899049319,6.34429361344449E-15,
34.5367258427036));
#36587=CARTESIAN_POINT('Ctrl Pts',(29.4666899049319,-34.5367258427036,34.5367258427036));
#36588=CARTESIAN_POINT('Ctrl Pts',(29.4666899049319,-34.5367258427036,6.34429361344449E-15));
#36589=CARTESIAN_POINT('Ctrl Pts',(29.4666899049319,-34.5367258427036,-33.0291706035535));
#36590=CARTESIAN_POINT('Ctrl Pts',(29.4666899049319,-1.54042548027395,-34.5023553003819));
#36591=CARTESIAN_POINT('Ctrl Pts',(28.7471241621752,-1.52592972576568,-34.1776802811774));
#36592=CARTESIAN_POINT('Ctrl Pts',(28.7471241621752,-0.763344698704461,
-34.21172738887));
#36593=CARTESIAN_POINT('Ctrl Pts',(28.7471241621752,-6.28459236601221E-15,
-34.21172738887));
#36594=CARTESIAN_POINT('Ctrl Pts',(28.7471241621752,34.2117273888699,-34.2117273888699));
#36595=CARTESIAN_POINT('Ctrl Pts',(28.7471241621752,34.21172738887,-6.28459236601221E-15));
#36596=CARTESIAN_POINT('Ctrl Pts',(28.7471241621752,34.2117273888699,34.2117273888699));
#36597=CARTESIAN_POINT('Ctrl Pts',(28.7471241621752,6.28459236601221E-15,
34.21172738887));
#36598=CARTESIAN_POINT('Ctrl Pts',(28.7471241621752,-34.2117273888699,34.2117273888699));
#36599=CARTESIAN_POINT('Ctrl Pts',(28.7471241621752,-34.21172738887,6.28459236601221E-15));
#36600=CARTESIAN_POINT('Ctrl Pts',(28.7471241621752,-34.2117273888699,-32.718358587775));
#36601=CARTESIAN_POINT('Ctrl Pts',(28.7471241621752,-1.52592972576568,-34.1776802811774));
#36602=CARTESIAN_POINT('Ctrl Pts',(27.8100958442934,-1.50698029472894,-33.7532520886149));
#36603=CARTESIAN_POINT('Ctrl Pts',(27.8100958442934,-0.7538652662764,-33.7868763896026));
#36604=CARTESIAN_POINT('Ctrl Pts',(27.8100958442934,-6.20654850355712E-15,
-33.7868763896026));
#36605=CARTESIAN_POINT('Ctrl Pts',(27.8100958442934,33.7868763896026,-33.7868763896026));
#36606=CARTESIAN_POINT('Ctrl Pts',(27.8100958442934,33.7868763896026,-6.20654850355712E-15));
#36607=CARTESIAN_POINT('Ctrl Pts',(27.8100958442934,33.7868763896026,33.7868763896026));
#36608=CARTESIAN_POINT('Ctrl Pts',(27.8100958442934,6.20654850355712E-15,
33.7868763896026));
#36609=CARTESIAN_POINT('Ctrl Pts',(27.8100958442934,-33.7868763896026,33.7868763896026));
#36610=CARTESIAN_POINT('Ctrl Pts',(27.8100958442934,-33.7868763896026,6.20654850355712E-15));
#36611=CARTESIAN_POINT('Ctrl Pts',(27.8100958442934,-33.7868763896026,-32.3120526686846));
#36612=CARTESIAN_POINT('Ctrl Pts',(27.8100958442934,-1.50698029472894,-33.7532520886149));
#36613=CARTESIAN_POINT('Ctrl Pts',(26.8343111708818,-1.48733431337754,-33.3132226048841));
#36614=CARTESIAN_POINT('Ctrl Pts',(26.8343111708818,-0.744037385305072,
-33.3464085574791));
#36615=CARTESIAN_POINT('Ctrl Pts',(26.8343111708818,-6.1256358754465E-15,
-33.3464085574791));
#36616=CARTESIAN_POINT('Ctrl Pts',(26.8343111708818,33.3464085574791,-33.3464085574791));
#36617=CARTESIAN_POINT('Ctrl Pts',(26.8343111708818,33.3464085574791,-6.1256358754465E-15));
#36618=CARTESIAN_POINT('Ctrl Pts',(26.8343111708818,33.3464085574791,33.3464085574791));
#36619=CARTESIAN_POINT('Ctrl Pts',(26.8343111708818,6.1256358754465E-15,
33.3464085574791));
#36620=CARTESIAN_POINT('Ctrl Pts',(26.8343111708818,-33.3464085574791,33.3464085574791));
#36621=CARTESIAN_POINT('Ctrl Pts',(26.8343111708818,-33.3464085574791,6.1256358754465E-15));
#36622=CARTESIAN_POINT('Ctrl Pts',(26.8343111708818,-33.3464085574791,-31.8908116037717));
#36623=CARTESIAN_POINT('Ctrl Pts',(26.8343111708818,-1.48733431337754,-33.3132226048841));
#36624=CARTESIAN_POINT('Ctrl Pts',(25.8181479469611,-1.46726916269954,-32.8638045923198));
#36625=CARTESIAN_POINT('Ctrl Pts',(25.8181479469611,-0.733999815330429,
-32.8965428438611));
#36626=CARTESIAN_POINT('Ctrl Pts',(25.8181479469611,-6.04299688451223E-15,
-32.8965428438611));
#36627=CARTESIAN_POINT('Ctrl Pts',(25.8181479469611,32.896542843861,-32.896542843861));
#36628=CARTESIAN_POINT('Ctrl Pts',(25.8181479469611,32.8965428438611,-6.04299688451223E-15));
#36629=CARTESIAN_POINT('Ctrl Pts',(25.8181479469611,32.896542843861,32.896542843861));
#36630=CARTESIAN_POINT('Ctrl Pts',(25.8181479469611,6.04299688451223E-15,
32.8965428438611));
#36631=CARTESIAN_POINT('Ctrl Pts',(25.8181479469611,-32.896542843861,32.896542843861));
#36632=CARTESIAN_POINT('Ctrl Pts',(25.8181479469611,-32.8965428438611,6.04299688451223E-15));
#36633=CARTESIAN_POINT('Ctrl Pts',(25.8181479469611,-32.896542843861,-31.4605828822811));
#36634=CARTESIAN_POINT('Ctrl Pts',(25.8181479469611,-1.46726916269954,-32.8638045923198));
#36635=CARTESIAN_POINT('Ctrl Pts',(24.7595197917227,-1.44728584082668,-32.4162193763075));
#36636=CARTESIAN_POINT('Ctrl Pts',(24.7595197917227,-0.724003180127261,
-32.4485117525897));
#36637=CARTESIAN_POINT('Ctrl Pts',(24.7595197917227,-5.96069490823564E-15,
-32.4485117525897));
#36638=CARTESIAN_POINT('Ctrl Pts',(24.7595197917227,32.4485117525897,-32.4485117525897));
#36639=CARTESIAN_POINT('Ctrl Pts',(24.7595197917227,32.4485117525897,-5.96069490823564E-15));
#36640=CARTESIAN_POINT('Ctrl Pts',(24.7595197917227,32.4485117525897,32.4485117525897));
#36641=CARTESIAN_POINT('Ctrl Pts',(24.7595197917227,5.96069490823564E-15,
32.4485117525897));
#36642=CARTESIAN_POINT('Ctrl Pts',(24.7595197917227,-32.4485117525897,32.4485117525897));
#36643=CARTESIAN_POINT('Ctrl Pts',(24.7595197917227,-32.4485117525897,5.96069490823564E-15));
#36644=CARTESIAN_POINT('Ctrl Pts',(24.7595197917227,-32.4485117525897,-31.0321087004291));
#36645=CARTESIAN_POINT('Ctrl Pts',(24.7595197917227,-1.44728584082668,-32.4162193763075));
#36646=CARTESIAN_POINT('Ctrl Pts',(23.6563574780851,-1.42804494464108,-31.9852629652417));
#36647=CARTESIAN_POINT('Ctrl Pts',(23.6563574780851,-0.714377942573004,
-32.017126031541));
#36648=CARTESIAN_POINT('Ctrl Pts',(23.6563574780851,-5.88145063686361E-15,
-32.017126031541));
#36649=CARTESIAN_POINT('Ctrl Pts',(23.6563574780851,32.017126031541,-32.017126031541));
#36650=CARTESIAN_POINT('Ctrl Pts',(23.6563574780851,32.017126031541,-5.88145063686361E-15));
#36651=CARTESIAN_POINT('Ctrl Pts',(23.6563574780851,32.017126031541,32.017126031541));
#36652=CARTESIAN_POINT('Ctrl Pts',(23.6563574780851,5.88145063686361E-15,
32.017126031541));
#36653=CARTESIAN_POINT('Ctrl Pts',(23.6563574780851,-32.017126031541,32.017126031541));
#36654=CARTESIAN_POINT('Ctrl Pts',(23.6563574780851,-32.017126031541,5.88145063686361E-15));
#36655=CARTESIAN_POINT('Ctrl Pts',(23.6563574780851,-32.017126031541,-30.6195533053013));
#36656=CARTESIAN_POINT('Ctrl Pts',(23.6563574780851,-1.42804494464108,-31.9852629652417));
#36657=CARTESIAN_POINT('Ctrl Pts',(22.5073180101405,-1.41024006077928,-31.5864702700101));
#36658=CARTESIAN_POINT('Ctrl Pts',(22.5073180101405,-0.705471068634144,
-31.6179360671638));
#36659=CARTESIAN_POINT('Ctrl Pts',(22.5073180101405,-5.80812063004468E-15,
-31.6179360671638));
#36660=CARTESIAN_POINT('Ctrl Pts',(22.5073180101405,31.6179360671638,-31.6179360671638));
#36661=CARTESIAN_POINT('Ctrl Pts',(22.5073180101405,31.6179360671638,-5.80812063004468E-15));
#36662=CARTESIAN_POINT('Ctrl Pts',(22.5073180101405,31.6179360671638,31.6179360671638));
#36663=CARTESIAN_POINT('Ctrl Pts',(22.5073180101405,5.80812063004468E-15,
31.6179360671638));
#36664=CARTESIAN_POINT('Ctrl Pts',(22.5073180101405,-31.6179360671638,31.6179360671638));
#36665=CARTESIAN_POINT('Ctrl Pts',(22.5073180101405,-31.6179360671638,5.80812063004468E-15));
#36666=CARTESIAN_POINT('Ctrl Pts',(22.5073180101405,-31.6179360671638,-30.237788296751));
#36667=CARTESIAN_POINT('Ctrl Pts',(22.5073180101405,-1.41024006077928,-31.5864702700101));
#36668=CARTESIAN_POINT('Ctrl Pts',(21.3125219557939,-1.394486513532,-31.2336232862855));
#36669=CARTESIAN_POINT('Ctrl Pts',(21.3125219557939,-0.697590373623126,
-31.264737584474));
#36670=CARTESIAN_POINT('Ctrl Pts',(21.3125219557939,-5.7432391213512E-15,
-31.264737584474));
#36671=CARTESIAN_POINT('Ctrl Pts',(21.3125219557939,31.264737584474,-31.264737584474));
#36672=CARTESIAN_POINT('Ctrl Pts',(21.3125219557939,31.264737584474,-5.7432391213512E-15));
#36673=CARTESIAN_POINT('Ctrl Pts',(21.3125219557939,31.264737584474,31.264737584474));
#36674=CARTESIAN_POINT('Ctrl Pts',(21.3125219557939,5.7432391213512E-15,
31.264737584474));
#36675=CARTESIAN_POINT('Ctrl Pts',(21.3125219557939,-31.264737584474,31.264737584474));
#36676=CARTESIAN_POINT('Ctrl Pts',(21.3125219557939,-31.264737584474,5.7432391213512E-15));
#36677=CARTESIAN_POINT('Ctrl Pts',(21.3125219557939,-31.264737584474,-29.9000072055494));
#36678=CARTESIAN_POINT('Ctrl Pts',(21.3125219557939,-1.394486513532,-31.2336232862855));
#36679=CARTESIAN_POINT('Ctrl Pts',(20.0742472323676,-1.38121259194221,-30.9363148057487));
#36680=CARTESIAN_POINT('Ctrl Pts',(20.0742472323676,-0.690950108671538,
-30.9671329312955));
#36681=CARTESIAN_POINT('Ctrl Pts',(20.0742472323676,-5.68857003346224E-15,
-30.9671329312955));
#36682=CARTESIAN_POINT('Ctrl Pts',(20.0742472323676,30.9671329312955,-30.9671329312955));
#36683=CARTESIAN_POINT('Ctrl Pts',(20.0742472323676,30.9671329312955,-5.68857003346224E-15));
#36684=CARTESIAN_POINT('Ctrl Pts',(20.0742472323676,30.9671329312955,30.9671329312955));
#36685=CARTESIAN_POINT('Ctrl Pts',(20.0742472323676,5.68857003346224E-15,
30.9671329312955));
#36686=CARTESIAN_POINT('Ctrl Pts',(20.0742472323676,-30.9671329312955,30.9671329312955));
#36687=CARTESIAN_POINT('Ctrl Pts',(20.0742472323676,-30.9671329312955,5.68857003346224E-15));
#36688=CARTESIAN_POINT('Ctrl Pts',(20.0742472323676,-30.9671329312955,-29.6153932294878));
#36689=CARTESIAN_POINT('Ctrl Pts',(20.0742472323676,-1.38121259194221,-30.9363148057487));
#36690=CARTESIAN_POINT('Ctrl Pts',(18.7979917002302,-1.3705167280896,-30.6967495040754));
#36691=CARTESIAN_POINT('Ctrl Pts',(18.7979917002302,-0.685599514321032,
-30.727328979557));
#36692=CARTESIAN_POINT('Ctrl Pts',(18.7979917002302,-5.64451876217433E-15,
-30.727328979557));
#36693=CARTESIAN_POINT('Ctrl Pts',(18.7979917002302,30.727328979557,-30.727328979557));
#36694=CARTESIAN_POINT('Ctrl Pts',(18.7979917002302,30.727328979557,-5.64451876217433E-15));
#36695=CARTESIAN_POINT('Ctrl Pts',(18.7979917002302,30.727328979557,30.727328979557));
#36696=CARTESIAN_POINT('Ctrl Pts',(18.7979917002302,5.64451876217433E-15,
30.727328979557));
#36697=CARTESIAN_POINT('Ctrl Pts',(18.7979917002302,-30.727328979557,30.727328979557));
#36698=CARTESIAN_POINT('Ctrl Pts',(18.7979917002302,-30.727328979557,5.64451876217433E-15));
#36699=CARTESIAN_POINT('Ctrl Pts',(18.7979917002302,-30.727328979557,-29.3860569087997));
#36700=CARTESIAN_POINT('Ctrl Pts',(18.7979917002302,-1.3705167280896,-30.6967495040754));
#36701=CARTESIAN_POINT('Ctrl Pts',(17.4917404060759,-1.36221698336642,-30.5108523315028));
#36702=CARTESIAN_POINT('Ctrl Pts',(17.4917404060759,-0.681447575979401,
-30.5412466200144));
#36703=CARTESIAN_POINT('Ctrl Pts',(17.4917404060759,-5.61033598727558E-15,
-30.5412466200144));
#36704=CARTESIAN_POINT('Ctrl Pts',(17.4917404060759,30.5412466200144,-30.5412466200144));
#36705=CARTESIAN_POINT('Ctrl Pts',(17.4917404060759,30.5412466200144,-5.61033598727558E-15));
#36706=CARTESIAN_POINT('Ctrl Pts',(17.4917404060759,30.5412466200144,30.5412466200144));
#36707=CARTESIAN_POINT('Ctrl Pts',(17.4917404060759,5.61033598727558E-15,
30.5412466200144));
#36708=CARTESIAN_POINT('Ctrl Pts',(17.4917404060759,-30.5412466200144,30.5412466200144));
#36709=CARTESIAN_POINT('Ctrl Pts',(17.4917404060759,-30.5412466200144,5.61033598727558E-15));
#36710=CARTESIAN_POINT('Ctrl Pts',(17.4917404060759,-30.5412466200144,-29.2080971905671));
#36711=CARTESIAN_POINT('Ctrl Pts',(17.4917404060759,-1.36221698336642,-30.5108523315028));
#36712=CARTESIAN_POINT('Ctrl Pts',(16.1647270995715,-1.35595673938413,-30.3706357712668));
#36713=CARTESIAN_POINT('Ctrl Pts',(16.1647270995715,-0.678315895682607,
-30.4008903789023));
#36714=CARTESIAN_POINT('Ctrl Pts',(16.1647270995715,-5.58455296406284E-15,
-30.4008903789023));
#36715=CARTESIAN_POINT('Ctrl Pts',(16.1647270995715,30.4008903789023,-30.4008903789023));
#36716=CARTESIAN_POINT('Ctrl Pts',(16.1647270995715,30.4008903789023,-5.58455296406284E-15));
#36717=CARTESIAN_POINT('Ctrl Pts',(16.1647270995715,30.4008903789023,30.4008903789023));
#36718=CARTESIAN_POINT('Ctrl Pts',(16.1647270995715,5.58455296406284E-15,
30.4008903789023));
#36719=CARTESIAN_POINT('Ctrl Pts',(16.1647270995715,-30.4008903789023,30.4008903789023));
#36720=CARTESIAN_POINT('Ctrl Pts',(16.1647270995715,-30.4008903789023,5.58455296406284E-15));
#36721=CARTESIAN_POINT('Ctrl Pts',(16.1647270995715,-30.4008903789023,-29.0738676097412));
#36722=CARTESIAN_POINT('Ctrl Pts',(16.1647270995715,-1.35595673938413,-30.3706357712668));
#36723=CARTESIAN_POINT('Ctrl Pts',(14.8263876417415,-1.3512881251525,-30.2660684364343));
#36724=CARTESIAN_POINT('Ctrl Pts',(14.8263876417415,-0.675980426451069,
-30.2962188762245));
#36725=CARTESIAN_POINT('Ctrl Pts',(14.8263876417415,-5.5653251209554E-15,
-30.2962188762246));
#36726=CARTESIAN_POINT('Ctrl Pts',(14.8263876417415,30.2962188762245,-30.2962188762245));
#36727=CARTESIAN_POINT('Ctrl Pts',(14.8263876417415,30.2962188762246,-5.5653251209554E-15));
#36728=CARTESIAN_POINT('Ctrl Pts',(14.8263876417415,30.2962188762245,30.2962188762245));
#36729=CARTESIAN_POINT('Ctrl Pts',(14.8263876417415,5.5653251209554E-15,
30.2962188762246));
#36730=CARTESIAN_POINT('Ctrl Pts',(14.8263876417415,-30.2962188762245,30.2962188762245));
#36731=CARTESIAN_POINT('Ctrl Pts',(14.8263876417415,-30.2962188762246,5.5653251209554E-15));
#36732=CARTESIAN_POINT('Ctrl Pts',(14.8263876417415,-30.2962188762245,-28.9737651004582));
#36733=CARTESIAN_POINT('Ctrl Pts',(14.8263876417415,-1.3512881251525,-30.2660684364343));
#36734=CARTESIAN_POINT('Ctrl Pts',(13.4853470903953,-1.34775518513426,-30.186937862885));
#36735=CARTESIAN_POINT('Ctrl Pts',(13.4853470903953,-0.674213077019295,
-30.2170094744125));
#36736=CARTESIAN_POINT('Ctrl Pts',(13.4853470903953,-5.55077458989668E-15,
-30.2170094744125));
#36737=CARTESIAN_POINT('Ctrl Pts',(13.4853470903953,30.2170094744125,-30.2170094744125));
#36738=CARTESIAN_POINT('Ctrl Pts',(13.4853470903953,30.2170094744125,-5.55077458989668E-15));
#36739=CARTESIAN_POINT('Ctrl Pts',(13.4853470903953,30.2170094744125,30.2170094744125));
#36740=CARTESIAN_POINT('Ctrl Pts',(13.4853470903953,5.55077458989668E-15,
30.2170094744125));
#36741=CARTESIAN_POINT('Ctrl Pts',(13.4853470903953,-30.2170094744125,30.2170094744125));
#36742=CARTESIAN_POINT('Ctrl Pts',(13.4853470903953,-30.2170094744125,5.55077458989668E-15));
#36743=CARTESIAN_POINT('Ctrl Pts',(13.4853470903953,-30.2170094744125,-28.8980132513174));
#36744=CARTESIAN_POINT('Ctrl Pts',(13.4853470903953,-1.34775518513426,-30.186937862885));
#36745=CARTESIAN_POINT('Ctrl Pts',(12.1482076787549,-1.34498727870743,-30.1249424647305));
#36746=CARTESIAN_POINT('Ctrl Pts',(12.1482076787549,-0.672828434816079,
-30.1549523177074));
#36747=CARTESIAN_POINT('Ctrl Pts',(12.1482076787549,-5.53937487514822E-15,
-30.1549523177074));
#36748=CARTESIAN_POINT('Ctrl Pts',(12.1482076787549,30.1549523177074,-30.1549523177074));
#36749=CARTESIAN_POINT('Ctrl Pts',(12.1482076787549,30.1549523177074,-5.53937487514822E-15));
#36750=CARTESIAN_POINT('Ctrl Pts',(12.1482076787549,30.1549523177074,30.1549523177074));
#36751=CARTESIAN_POINT('Ctrl Pts',(12.1482076787549,5.53937487514822E-15,
30.1549523177074));
#36752=CARTESIAN_POINT('Ctrl Pts',(12.1482076787549,-30.1549523177074,30.1549523177074));
#36753=CARTESIAN_POINT('Ctrl Pts',(12.1482076787549,-30.1549523177074,5.53937487514822E-15));
#36754=CARTESIAN_POINT('Ctrl Pts',(12.1482076787549,-30.1549523177074,-28.8386649382978));
#36755=CARTESIAN_POINT('Ctrl Pts',(12.1482076787549,-1.34498727870743,-30.1249424647305));
#36756=CARTESIAN_POINT('Ctrl Pts',(10.8190675759626,-1.34274367710657,-30.0746904138676));
#36757=CARTESIAN_POINT('Ctrl Pts',(10.8190675759626,-0.671706075536292,
-30.1046502067769));
#36758=CARTESIAN_POINT('Ctrl Pts',(10.8190675759626,-5.530134527277E-15,
-30.1046502067769));
#36759=CARTESIAN_POINT('Ctrl Pts',(10.8190675759626,30.1046502067769,-30.1046502067769));
#36760=CARTESIAN_POINT('Ctrl Pts',(10.8190675759626,30.1046502067769,-5.530134527277E-15));
#36761=CARTESIAN_POINT('Ctrl Pts',(10.8190675759626,30.1046502067769,30.1046502067769));
#36762=CARTESIAN_POINT('Ctrl Pts',(10.8190675759626,5.530134527277E-15,
30.1046502067769));
#36763=CARTESIAN_POINT('Ctrl Pts',(10.8190675759626,-30.1046502067769,30.1046502067769));
#36764=CARTESIAN_POINT('Ctrl Pts',(10.8190675759626,-30.1046502067769,5.530134527277E-15));
#36765=CARTESIAN_POINT('Ctrl Pts',(10.8190675759626,-30.1046502067769,-28.7905585540618));
#36766=CARTESIAN_POINT('Ctrl Pts',(10.8190675759626,-1.34274367710657,-30.0746904138676));
#36767=CARTESIAN_POINT('Ctrl Pts',(9.50027713254189,-1.3408752011877,-30.032840404991));
#36768=CARTESIAN_POINT('Ctrl Pts',(9.50027713254189,-0.67077137247412,-30.0627585077754));
#36769=CARTESIAN_POINT('Ctrl Pts',(9.50027713254189,-5.52243914701304E-15,
-30.0627585077754));
#36770=CARTESIAN_POINT('Ctrl Pts',(9.50027713254189,30.0627585077753,-30.0627585077753));
#36771=CARTESIAN_POINT('Ctrl Pts',(9.50027713254189,30.0627585077754,-5.52243914701304E-15));
#36772=CARTESIAN_POINT('Ctrl Pts',(9.5002771325419,30.0627585077753,30.0627585077753));
#36773=CARTESIAN_POINT('Ctrl Pts',(9.5002771325419,5.52243914701304E-15,
30.0627585077754));
#36774=CARTESIAN_POINT('Ctrl Pts',(9.5002771325419,-30.0627585077753,30.0627585077753));
#36775=CARTESIAN_POINT('Ctrl Pts',(9.50027713254189,-30.0627585077754,5.52243914701304E-15));
#36776=CARTESIAN_POINT('Ctrl Pts',(9.50027713254189,-30.0627585077754,-28.750495460661));
#36777=CARTESIAN_POINT('Ctrl Pts',(9.50027713254189,-1.3408752011877,-30.032840404991));
#36778=CARTESIAN_POINT('Ctrl Pts',(8.45435372222587,-1.33961990745209,-30.0047244129961));
#36779=CARTESIAN_POINT('Ctrl Pts',(8.45435372222587,-0.670143413137455,
-30.0346145072029));
#36780=CARTESIAN_POINT('Ctrl Pts',(8.45435372222587,-5.51726917798061E-15,
-30.0346145072029));
#36781=CARTESIAN_POINT('Ctrl Pts',(8.45435372222587,30.0346145072029,-30.0346145072029));
#36782=CARTESIAN_POINT('Ctrl Pts',(8.45435372222587,30.0346145072029,-5.51726917798061E-15));
#36783=CARTESIAN_POINT('Ctrl Pts',(8.45435372222587,30.0346145072029,30.0346145072029));
#36784=CARTESIAN_POINT('Ctrl Pts',(8.45435372222587,5.51726917798061E-15,
30.0346145072029));
#36785=CARTESIAN_POINT('Ctrl Pts',(8.45435372222587,-30.0346145072029,30.0346145072029));
#36786=CARTESIAN_POINT('Ctrl Pts',(8.45435372222587,-30.0346145072029,5.51726917798061E-15));
#36787=CARTESIAN_POINT('Ctrl Pts',(8.45435372222587,-30.0346145072029,-28.7235799678431));
#36788=CARTESIAN_POINT('Ctrl Pts',(8.45435372222587,-1.33961990745209,-30.0047244129961));
#36789=CARTESIAN_POINT('Ctrl Pts',(7.67514864245731,-1.33880061938141,-29.9863740491064));
#36790=CARTESIAN_POINT('Ctrl Pts',(7.67514864245731,-0.66973356516418,-30.0162458630552));
#36791=CARTESIAN_POINT('Ctrl Pts',(7.67514864245731,-5.51389491279158E-15,
-30.0162458630552));
#36792=CARTESIAN_POINT('Ctrl Pts',(7.67514864245731,30.0162458630552,-30.0162458630552));
#36793=CARTESIAN_POINT('Ctrl Pts',(7.67514864245731,30.0162458630552,-5.51389491279158E-15));
#36794=CARTESIAN_POINT('Ctrl Pts',(7.67514864245731,30.0162458630552,30.0162458630552));
#36795=CARTESIAN_POINT('Ctrl Pts',(7.67514864245731,5.51389491279158E-15,
30.0162458630552));
#36796=CARTESIAN_POINT('Ctrl Pts',(7.67514864245731,-30.0162458630552,30.0162458630552));
#36797=CARTESIAN_POINT('Ctrl Pts',(7.67514864245731,-30.0162458630552,5.51389491279158E-15));
#36798=CARTESIAN_POINT('Ctrl Pts',(7.67514864245731,-30.0162458630552,-28.7060131294556));
#36799=CARTESIAN_POINT('Ctrl Pts',(7.67514864245731,-1.33880061938141,-29.9863740491064));
#36800=CARTESIAN_POINT('Ctrl Pts',(7.15799654185577,-1.33830853171149,-29.9753522996976));
#36801=CARTESIAN_POINT('Ctrl Pts',(7.15799654185577,-0.669487398838308,
-30.0052131340045));
#36802=CARTESIAN_POINT('Ctrl Pts',(7.15799654185577,-5.51186823334392E-15,
-30.0052131340045));
#36803=CARTESIAN_POINT('Ctrl Pts',(7.15799654185577,30.0052131340045,-30.0052131340045));
#36804=CARTESIAN_POINT('Ctrl Pts',(7.15799654185577,30.0052131340045,-5.51186823334392E-15));
#36805=CARTESIAN_POINT('Ctrl Pts',(7.15799654185577,30.0052131340045,30.0052131340045));
#36806=CARTESIAN_POINT('Ctrl Pts',(7.15799654185577,5.51186823334392E-15,
30.0052131340045));
#36807=CARTESIAN_POINT('Ctrl Pts',(7.15799654185577,-30.0052131340045,30.0052131340045));
#36808=CARTESIAN_POINT('Ctrl Pts',(7.15799654185577,-30.0052131340045,5.51186823334392E-15));
#36809=CARTESIAN_POINT('Ctrl Pts',(7.15799654185577,-30.0052131340045,-28.695461987703));
#36810=CARTESIAN_POINT('Ctrl Pts',(7.15799654185577,-1.33830853171149,-29.9753522996976));
#36811=CARTESIAN_POINT('Ctrl Pts',(6.9,-1.33807601272607,-29.9701443537426));
#36812=CARTESIAN_POINT('Ctrl Pts',(6.9,-0.669371081466759,-30.));
#36813=CARTESIAN_POINT('Ctrl Pts',(6.9,-5.51091059616309E-15,-30.));
#36814=CARTESIAN_POINT('Ctrl Pts',(6.9,30.,-30.));
#36815=CARTESIAN_POINT('Ctrl Pts',(6.9,30.,-5.51091059616309E-15));
#36816=CARTESIAN_POINT('Ctrl Pts',(6.9,30.,30.));
#36817=CARTESIAN_POINT('Ctrl Pts',(6.9,5.51091059616309E-15,30.));
#36818=CARTESIAN_POINT('Ctrl Pts',(6.9,-30.,30.));
#36819=CARTESIAN_POINT('Ctrl Pts',(6.9,-30.,5.51091059616309E-15));
#36820=CARTESIAN_POINT('Ctrl Pts',(6.9,-30.,-28.6904764110968));
#36821=CARTESIAN_POINT('Ctrl Pts',(6.9,-1.33807601272607,-29.9701443537426));
#36822=CARTESIAN_POINT('Ctrl Pts',(6.9,21.8303175223207,-20.5775906479515));
#36823=CARTESIAN_POINT('Ctrl Pts',(7.85773098116326,20.4889265372405,-22.0288565043892));
#36824=CARTESIAN_POINT('Ctrl Pts',(8.88781981167334,19.0414114324084,-23.3171626725998));
#36825=CARTESIAN_POINT('Ctrl Pts',(10.5914578196776,16.6247285680552,-25.1150390010341));
#36826=CARTESIAN_POINT('Ctrl Pts',(11.2365058953701,15.703976734769,-25.7254166302984));
#36827=CARTESIAN_POINT('Ctrl Pts',(12.0558885382926,14.5853792872662,-26.3926147460599));
#36828=CARTESIAN_POINT('Ctrl Pts',(12.1875764958397,14.4076425286694,-26.4963665374952));
#36829=CARTESIAN_POINT('Ctrl Pts',(13.194901830313,13.0552778456719,-27.2691057169114));
#36830=CARTESIAN_POINT('Ctrl Pts',(14.2258982134098,11.6381637544796,-27.991732600527));
#36831=CARTESIAN_POINT('Ctrl Pts',(18.2616480823244,6.95587410790868,-29.9350198014187));
#36832=CARTESIAN_POINT('Ctrl Pts',(21.0496416709525,4.29983295736293,-30.7693084982877));
#36833=CARTESIAN_POINT('Ctrl Pts',(25.8000196361138,1.93741001991748,-32.8040277065106));
#36834=CARTESIAN_POINT('Ctrl Pts',(26.8976561124457,1.74039351523169,-33.3305524688301));
#36835=CARTESIAN_POINT('Ctrl Pts',(28.0045908801237,1.58669630450145,-33.8378020212277));
#36836=CARTESIAN_POINT('Ctrl Pts',(28.5235971652406,1.54532623843658,-34.0754855762016));
#36837=CARTESIAN_POINT('Ctrl Pts',(29.0834839543824,1.4982885487127,-34.3307100593381));
#36838=CARTESIAN_POINT('Ctrl Pts',(29.1146288039499,1.49562082188433,-34.3449058451715));
#36839=CARTESIAN_POINT('Ctrl Pts',(29.5949306848436,1.45589225448013,-34.5637016811193));
#36840=CARTESIAN_POINT('Ctrl Pts',(30.0492939924726,1.44682754698747,-34.7685410859787));
#36841=CARTESIAN_POINT('Ctrl Pts',(30.5,1.44976976333441,-34.9699609326822));
#36842=CARTESIAN_POINT('Ctrl Pts',(6.45331003273164,8.65286216739172,-6.83943894028999));
#36843=CARTESIAN_POINT('Ctrl Pts',(7.20830533428676,8.29622318255582,-7.28712780725476));
#36844=CARTESIAN_POINT('Ctrl Pts',(7.99924796920645,7.91909532230128,-7.69991572864563));
#36845=CARTESIAN_POINT('Ctrl Pts',(9.76163642871394,7.0702837202071,-8.50127829248443));
#36846=CARTESIAN_POINT('Ctrl Pts',(10.7316626231511,6.57783879792861,-8.8793528128254));
#36847=CARTESIAN_POINT('Ctrl Pts',(12.6608237755523,5.67260683532432,-9.49392179513702));
#36848=CARTESIAN_POINT('Ctrl Pts',(13.6376935580087,5.20677839827646,-9.74868549844379));
#36849=CARTESIAN_POINT('Ctrl Pts',(14.8683081444882,4.68571756497415,-10.0072371758851));
#36850=CARTESIAN_POINT('Ctrl Pts',(15.814981546047,4.28615487511135,-10.1933420307132));
#36851=CARTESIAN_POINT('Ctrl Pts',(16.7774761024725,3.90183726466219,-10.3417484740057));
#36852=CARTESIAN_POINT('Ctrl Pts',(18.4438470226175,3.30966453460613,-10.5575964922699));
#36853=CARTESIAN_POINT('Ctrl Pts',(19.4166260537867,2.98271399009539,-10.6478897990578));
#36854=CARTESIAN_POINT('Ctrl Pts',(20.8624415465507,2.5875063027773,-10.7552000633454));
#36855=CARTESIAN_POINT('Ctrl Pts',(21.8144010701944,2.34040933534244,-10.8125125199159));
#36856=CARTESIAN_POINT('Ctrl Pts',(22.7817704456175,2.13286375196528,-10.8543372932887));
#36857=CARTESIAN_POINT('Ctrl Pts',(23.3296603631195,2.03163991938108,-10.8753724962822));
#36858=CARTESIAN_POINT('Ctrl Pts',(23.4469280425869,2.01025391532517,-10.8796667005723));
#36859=CARTESIAN_POINT('Ctrl Pts',(23.6810288813553,1.96865773783264,-10.8878000542956));
#36860=CARTESIAN_POINT('Ctrl Pts',(24.0941214149603,1.89824222375215,-10.9009272596696));
#36861=CARTESIAN_POINT('Ctrl Pts',(24.6899984645715,1.80575737992304,-10.9167861221079));
#36862=CARTESIAN_POINT('Ctrl Pts',(25.4117472347965,1.71023812556292,-10.9320835607493));
#36863=CARTESIAN_POINT('Ctrl Pts',(25.8944359856997,1.65861072075244,-10.9403877892627));
#36864=CARTESIAN_POINT('Ctrl Pts',(26.3669426319602,1.61476081138877,-10.9478841337461));
#36865=CARTESIAN_POINT('Ctrl Pts',(27.2927605647398,1.54499465236548,-10.9593568588012));
#36866=CARTESIAN_POINT('Ctrl Pts',(28.2852623623168,1.51981821556059,-10.9616475307267));
#36867=CARTESIAN_POINT('Ctrl Pts',(29.2044123671999,1.49506529955051,-10.9652006081482));
#36868=CARTESIAN_POINT('Ctrl Pts',(29.5205491106405,1.48868169066078,-10.9661656603817));
#36869=CARTESIAN_POINT('Ctrl Pts',(30.1691034959588,1.48263221141176,-10.9670510696507));
#36870=CARTESIAN_POINT('Ctrl Pts',(31.3134334344234,1.4864605825931,-10.9664912432219));
#36871=CARTESIAN_POINT('Ctrl Pts',(32.3203424123247,1.49997009105206,-10.9645690748214));
#36872=CARTESIAN_POINT('Ctrl Pts',(33.1675465322482,1.49998069520818,-10.9645713457497));
#36873=CARTESIAN_POINT('Ctrl Pts',(33.4947519346945,1.49998093738942,-10.9645717110255));
#36874=CARTESIAN_POINT('Ctrl Pts',(34.1540738134336,1.49998231763443,-10.9645721532421));
#36875=CARTESIAN_POINT('Ctrl Pts',(34.81145110075,1.499985805429,-10.9645737361772));
#36876=CARTESIAN_POINT('Ctrl Pts',(35.7991041415374,1.49998654292927,-10.9645740230236));
#36877=CARTESIAN_POINT('Ctrl Pts',(37.7734954411133,1.49999064614178,-10.9645758157224));
#36878=CARTESIAN_POINT('Ctrl Pts',(39.5833333333333,1.5,-10.9645797934319));
#36879=CARTESIAN_POINT('Ctrl Pts',(40.9,1.5,-10.9645797934319));
#36880=CARTESIAN_POINT('Ctrl Pts',(6.63336813585096,11.0008793183436,-9.34202246898051));
#36881=CARTESIAN_POINT('Ctrl Pts',(7.389696336477,10.5126404716241,-9.9106502389341));
#36882=CARTESIAN_POINT('Ctrl Pts',(8.18028889045472,10.0000669136624,-10.4323217834721));
#36883=CARTESIAN_POINT('Ctrl Pts',(9.94159575574687,8.85353468669098,-11.439192222287));
#36884=CARTESIAN_POINT('Ctrl Pts',(10.9109419422817,8.192010210379,-11.9102705993651));
#36885=CARTESIAN_POINT('Ctrl Pts',(12.8335218625484,6.98387303125937,-12.6683977976686));
#36886=CARTESIAN_POINT('Ctrl Pts',(13.8091851210584,6.36343771133682,-12.9798296118147));
#36887=CARTESIAN_POINT('Ctrl Pts',(15.0310774900381,5.67481209887734,-13.2915570052697));
#36888=CARTESIAN_POINT('Ctrl Pts',(15.9749773134882,5.14536755152679,-13.5160612446606));
#36889=CARTESIAN_POINT('Ctrl Pts',(16.930312943506,4.63930769376668,-13.6911692618857));
#36890=CARTESIAN_POINT('Ctrl Pts',(18.5806860927912,3.86175938608204,-13.9445588072223));
#36891=CARTESIAN_POINT('Ctrl Pts',(19.548719041905,3.43185831734755,-14.047648520923));
#36892=CARTESIAN_POINT('Ctrl Pts',(20.9744115808253,2.91639691217872,-14.1690991173097));
#36893=CARTESIAN_POINT('Ctrl Pts',(21.9189583606345,2.59280390983887,-14.2328177454448));
#36894=CARTESIAN_POINT('Ctrl Pts',(22.8721113115929,2.32284159836073,-14.2778669302766));
#36895=CARTESIAN_POINT('Ctrl Pts',(23.4111206282029,2.1913240624154,-14.300719458499));
#36896=CARTESIAN_POINT('Ctrl Pts',(23.5272640974129,2.16340494095905,-14.3053783578071));
#36897=CARTESIAN_POINT('Ctrl Pts',(23.7586042074435,2.10919630050476,-14.3141392731538));
#36898=CARTESIAN_POINT('Ctrl Pts',(24.1668594457504,2.01743796447889,-14.3281409258012));
#36899=CARTESIAN_POINT('Ctrl Pts',(24.7549510427126,1.89707890772754,-14.3447231768686));
#36900=CARTESIAN_POINT('Ctrl Pts',(25.4661619742724,1.77296928480105,-14.3604369110458));
#36901=CARTESIAN_POINT('Ctrl Pts',(25.940793652308,1.7060154102986,-14.3689791856741));
#36902=CARTESIAN_POINT('Ctrl Pts',(26.4047985025956,1.64920950338615,-14.3768131131953));
#36903=CARTESIAN_POINT('Ctrl Pts',(27.3109130873601,1.55899536298034,-14.3886741790609));
#36904=CARTESIAN_POINT('Ctrl Pts',(28.2968127703992,1.52586579774316,-14.3906288624532));
#36905=CARTESIAN_POINT('Ctrl Pts',(29.216365869052,1.49337715415662,-14.3942351181099));
#36906=CARTESIAN_POINT('Ctrl Pts',(29.5273677411776,1.48510498656914,-14.3952146919186));
#36907=CARTESIAN_POINT('Ctrl Pts',(30.1704748351474,1.47720108681952,-14.3961140069303));
#36908=CARTESIAN_POINT('Ctrl Pts',(31.3076822233502,1.48219673215098,-14.3955480332033));
#36909=CARTESIAN_POINT('Ctrl Pts',(32.3162781940781,1.49994928257769,-14.3936026936296));
#36910=CARTESIAN_POINT('Ctrl Pts',(33.1684720644413,1.49996698297726,-14.3936066618446));
#36911=CARTESIAN_POINT('Ctrl Pts',(33.4950641584122,1.49996744488463,-14.3936073001223));
#36912=CARTESIAN_POINT('Ctrl Pts',(34.1546952525893,1.49996977575843,-14.3936080728485));
#36913=CARTESIAN_POINT('Ctrl Pts',(34.811773768313,1.49997575137035,-14.3936108388537));
#36914=CARTESIAN_POINT('Ctrl Pts',(35.7994747102212,1.49997700611746,-14.3936113400865));
#36915=CARTESIAN_POINT('Ctrl Pts',(37.7736758948774,1.499984023326,-14.3936144726314));
#36916=CARTESIAN_POINT('Ctrl Pts',(39.5833333333333,1.5,-14.3936214232436));
#36917=CARTESIAN_POINT('Ctrl Pts',(40.9,1.5,-14.3936214232436));
#36918=CARTESIAN_POINT('Ctrl Pts',(6.84643360079894,16.506001665025,-15.1545575883324));
#36919=CARTESIAN_POINT('Ctrl Pts',(7.61273218496772,15.7040687667121,-16.0159127642118));
#36920=CARTESIAN_POINT('Ctrl Pts',(8.4126771054426,14.8690272591124,-16.7980113101253));
#36921=CARTESIAN_POINT('Ctrl Pts',(10.1879439641556,13.0164926384401,-18.2945580567154));
#36922=CARTESIAN_POINT('Ctrl Pts',(11.1642689802371,11.9550510602025,-18.9856854823124));
#36923=CARTESIAN_POINT('Ctrl Pts',(13.1036036726265,10.022452207883,-20.0861315198186));
#36924=CARTESIAN_POINT('Ctrl Pts',(14.0826172183607,9.03879487952599,-20.5290484396468));
#36925=CARTESIAN_POINT('Ctrl Pts',(15.3089235211201,7.95158583831005,-20.9656035967448));
#36926=CARTESIAN_POINT('Ctrl Pts',(16.2536562498252,7.11690983506512,-21.279069264144));
#36927=CARTESIAN_POINT('Ctrl Pts',(17.2094234535123,6.32372298857519,-21.5156901422925));
#36928=CARTESIAN_POINT('Ctrl Pts',(18.8492103514785,5.11428176787038,-21.8541559656567));
#36929=CARTESIAN_POINT('Ctrl Pts',(19.8132789859546,4.44555314736778,-21.9855288021884));
#36930=CARTESIAN_POINT('Ctrl Pts',(21.2105274130183,3.65671370764623,-22.1378650260475));
#36931=CARTESIAN_POINT('Ctrl Pts',(22.1435262947165,3.15760868632205,-22.2155499994866));
#36932=CARTESIAN_POINT('Ctrl Pts',(23.0712019161591,2.74759983583376,-22.2672966100825));
#36933=CARTESIAN_POINT('Ctrl Pts',(23.5926643019347,2.54861011877026,-22.2940508574536));
#36934=CARTESIAN_POINT('Ctrl Pts',(23.7065967589747,2.50584172092975,-22.2995097248263));
#36935=CARTESIAN_POINT('Ctrl Pts',(23.9324349207315,2.42316535684894,-22.3096292230893));
#36936=CARTESIAN_POINT('Ctrl Pts',(24.3308966188196,2.28324508302851,-22.3255066595418));
#36937=CARTESIAN_POINT('Ctrl Pts',(24.9027307486989,2.10031694390082,-22.3435822260678));
#36938=CARTESIAN_POINT('Ctrl Pts',(25.5912058020402,1.91242242103884,-22.3601136597686));
#36939=CARTESIAN_POINT('Ctrl Pts',(26.0479116166522,1.81155274261715,-22.3691489781576));
#36940=CARTESIAN_POINT('Ctrl Pts',(26.4927766852066,1.72621142470537,-22.3777261422415));
#36941=CARTESIAN_POINT('Ctrl Pts',(27.3538144829414,1.59133675559696,-22.3904445374985));
#36942=CARTESIAN_POINT('Ctrl Pts',(28.3239440765631,1.5395372712982,-22.3916143651133));
#36943=CARTESIAN_POINT('Ctrl Pts',(29.2444087331683,1.48903537353033,-22.3953365265065));
#36944=CARTESIAN_POINT('Ctrl Pts',(29.5434413064006,1.4765958448865,-22.3963491807022));
#36945=CARTESIAN_POINT('Ctrl Pts',(30.1738228526165,1.46445321166481,-22.3972793088217));
#36946=CARTESIAN_POINT('Ctrl Pts',(31.2943937060125,1.47211763918551,-22.3966964278384));
#36947=CARTESIAN_POINT('Ctrl Pts',(32.3068807810285,1.49983279134388,-22.394691709999));
#36948=CARTESIAN_POINT('Ctrl Pts',(33.1706991860564,1.49988437406509,-22.3946974029306));
#36949=CARTESIAN_POINT('Ctrl Pts',(33.4958573126069,1.49988713027318,-22.3946983171245));
#36950=CARTESIAN_POINT('Ctrl Pts',(34.1562063695874,1.49989458266054,-22.394699425001));
#36951=CARTESIAN_POINT('Ctrl Pts',(34.8125750960603,1.49991575825724,-22.3947033892012));
#36952=CARTESIAN_POINT('Ctrl Pts',(35.8003855127833,1.49991999484082,-22.3947041076692));
#36953=CARTESIAN_POINT('Ctrl Pts',(37.7741287617181,1.49994455667285,-22.394708597346));
#36954=CARTESIAN_POINT('Ctrl Pts',(39.5833333333333,1.5,-22.394718559471));
#36955=CARTESIAN_POINT('Ctrl Pts',(40.9,1.5,-22.394718559471));
#36956=CARTESIAN_POINT('Ctrl Pts',(6.90857970435319,22.1068727166734,-20.8698550272217));
#36957=CARTESIAN_POINT('Ctrl Pts',(7.67983757144493,20.991774688754,-22.0336104135999));
#36958=CARTESIAN_POINT('Ctrl Pts',(8.48444928201916,19.8332461961107,-23.0860770683301));
#36959=CARTESIAN_POINT('Ctrl Pts',(10.2687663769551,17.2709888357559,-25.0905346149111));
#36960=CARTESIAN_POINT('Ctrl Pts',(11.2490111943913,15.8072894822424,-26.0108786577409));
#36961=CARTESIAN_POINT('Ctrl Pts',(13.2067599054631,13.1283892637642,-27.4745835397));
#36962=CARTESIAN_POINT('Ctrl Pts',(14.1887708824687,11.7775873547894,-28.0545611646472));
#36963=CARTESIAN_POINT('Ctrl Pts',(15.4301927253883,10.2708149751555,-28.6258871350548));
#36964=CARTESIAN_POINT('Ctrl Pts',(16.3793034376203,9.12509880827948,-29.0320485193235));
#36965=CARTESIAN_POINT('Ctrl Pts',(17.3459407209746,8.02905385413649,-29.335531334809));
#36966=CARTESIAN_POINT('Ctrl Pts',(19.0016786397101,6.36442803225958,-29.764530122403));
#36967=CARTESIAN_POINT('Ctrl Pts',(19.9708024570658,5.44984750618438,-29.9249381814107));
#36968=CARTESIAN_POINT('Ctrl Pts',(21.3726541621532,4.37628680649797,-30.1088343166975));
#36969=CARTESIAN_POINT('Ctrl Pts',(22.305997327355,3.69883691082954,-30.2002109026539));
#36970=CARTESIAN_POINT('Ctrl Pts',(23.2278577930096,3.14826448808768,-30.2581794306256));
#36971=CARTESIAN_POINT('Ctrl Pts',(23.7415516356673,2.88362049576681,-30.2885183156943));
#36972=CARTESIAN_POINT('Ctrl Pts',(23.8544946510481,2.82623659223922,-30.2947200062415));
#36973=CARTESIAN_POINT('Ctrl Pts',(24.0777274663499,2.71573667925152,-30.3060802342181));
#36974=CARTESIAN_POINT('Ctrl Pts',(24.4711727956187,2.52895535356898,-30.32363513723));
#36975=CARTESIAN_POINT('Ctrl Pts',(25.0334457271175,2.28601411482693,-30.3429441514165));
#36976=CARTESIAN_POINT('Ctrl Pts',(25.706214488466,2.03835403030808,-30.3600503901637));
#36977=CARTESIAN_POINT('Ctrl Pts',(26.1486936133439,1.90670660027133,-30.3694723684124));
#36978=CARTESIAN_POINT('Ctrl Pts',(26.5774366289031,1.79594947825407,-30.3787139799022));
#36979=CARTESIAN_POINT('Ctrl Pts',(27.3975110717084,1.62272694197858,-30.392198133447));
#36980=CARTESIAN_POINT('Ctrl Pts',(28.3508259392473,1.55227638555954,-30.3926064111246));
#36981=CARTESIAN_POINT('Ctrl Pts',(29.2723062856311,1.48380439950633,-30.3964396342324));
#36982=CARTESIAN_POINT('Ctrl Pts',(29.5594622066961,1.46775103384065,-30.3974855836748));
#36983=CARTESIAN_POINT('Ctrl Pts',(30.1771168569175,1.45157152773897,-30.3984465770314));
#36984=CARTESIAN_POINT('Ctrl Pts',(31.281071177308,1.46177125475314,-30.3978463334884));
#36985=CARTESIAN_POINT('Ctrl Pts',(32.297455993961,1.49958178095818,-30.3957818406259));
#36986=CARTESIAN_POINT('Ctrl Pts',(33.1729044426911,1.49970257782127,-30.395789026338));
#36987=CARTESIAN_POINT('Ctrl Pts',(33.4966295876142,1.4997109685702,-30.3957901777219));
#36988=CARTESIAN_POINT('Ctrl Pts',(34.1576977268014,1.49972932651149,-30.3957915749198));
#36989=CARTESIAN_POINT('Ctrl Pts',(34.813360769929,1.4997840805116,-30.3957965718591));
#36990=CARTESIAN_POINT('Ctrl Pts',(35.8012813983216,1.49979479816102,-30.3957974776821));
#36991=CARTESIAN_POINT('Ctrl Pts',(37.7745713511015,1.49985796376524,-30.395803137258));
#36992=CARTESIAN_POINT('Ctrl Pts',(39.5833333333333,1.49999999999999,-30.3958156956984));
#36993=CARTESIAN_POINT('Ctrl Pts',(40.9,1.49999999999999,-30.3958156956984));
#36994=CARTESIAN_POINT('Ctrl Pts',(6.93528330520032,25.3195110382618,-24.1234099037007));
#36995=CARTESIAN_POINT('Ctrl Pts',(7.70864561497005,24.0266258397084,-25.4600205488393));
#36996=CARTESIAN_POINT('Ctrl Pts',(8.51531156164573,22.6840056101462,-26.6675788409114));
#36997=CARTESIAN_POINT('Ctrl Pts',(10.3033767345502,19.7178334181139,-28.9634999585434));
#36998=CARTESIAN_POINT('Ctrl Pts',(11.2853975328499,18.024966824446,-30.0157138764657));
#36999=CARTESIAN_POINT('Ctrl Pts',(13.2504656206425,14.920608256729,-31.6887121402305));
#37000=CARTESIAN_POINT('Ctrl Pts',(14.2338911783743,13.360326515741,-32.3479754973602));
#37001=CARTESIAN_POINT('Ctrl Pts',(15.4814489736579,11.6128587845954,-32.9977120049688));
#37002=CARTESIAN_POINT('Ctrl Pts',(16.4323633322631,10.2891584164032,-33.457701559807));
#37003=CARTESIAN_POINT('Ctrl Pts',(17.4036580739675,9.01884161707319,-33.8004278805126));
#37004=CARTESIAN_POINT('Ctrl Pts',(19.0672887678302,7.09001985912387,-34.2828730898379));
#37005=CARTESIAN_POINT('Ctrl Pts',(20.0391149919151,6.03348815316116,-34.4604737318843));
#37006=CARTESIAN_POINT('Ctrl Pts',(21.4462778487112,4.79159535501522,-34.6632929668281));
#37007=CARTESIAN_POINT('Ctrl Pts',(22.3811728101678,4.01020122074908,-34.7627792680187));
#37008=CARTESIAN_POINT('Ctrl Pts',(23.3032595484893,3.37635643636738,-34.8244923190156));
#37009=CARTESIAN_POINT('Ctrl Pts',(23.8149974822583,3.07312481135075,-34.8569118346709));
#37010=CARTESIAN_POINT('Ctrl Pts',(23.9276845297173,3.00725282827683,-34.8635414236987));
#37011=CARTESIAN_POINT('Ctrl Pts',(24.1501932465709,2.88055633977638,-34.8756163196445));
#37012=CARTESIAN_POINT('Ctrl Pts',(24.5421106234083,2.66656979475214,-34.8941314993696));
#37013=CARTESIAN_POINT('Ctrl Pts',(25.1010166003946,2.38896069563579,-34.9141289755492));
#37014=CARTESIAN_POINT('Ctrl Pts',(25.7673676623321,2.10719515267299,-34.9315307898229));
#37015=CARTESIAN_POINT('Ctrl Pts',(26.2032614590243,1.95837832513291,-34.9411502230501));
#37016=CARTESIAN_POINT('Ctrl Pts',(26.6241220770206,1.83365744353248,-34.9507523611205));
#37017=CARTESIAN_POINT('Ctrl Pts',(27.4227877709103,1.64008822157604,-34.9646463474546));
#37018=CARTESIAN_POINT('Ctrl Pts',(28.3660425122777,1.55920845841384,-34.9646178111257));
#37019=CARTESIAN_POINT('Ctrl Pts',(29.288154079426,1.48047877405357,-34.9685099768711));
#37020=CARTESIAN_POINT('Ctrl Pts',(29.5685743108623,1.46254110097229,-34.9695745039167));
#37021=CARTESIAN_POINT('Ctrl Pts',(30.1789566228709,1.44412472938078,-34.9705522790041));
#37022=CARTESIAN_POINT('Ctrl Pts',(31.273428633048,1.45573528147978,-34.9699406754865));
#37023=CARTESIAN_POINT('Ctrl Pts',(32.2920480078111,1.49937027232428,-34.9678391394653));
#37024=CARTESIAN_POINT('Ctrl Pts',(33.1741467941405,1.49954725443549,-34.9678459524317));
#37025=CARTESIAN_POINT('Ctrl Pts',(33.4970538821705,1.49956078207587,-34.9678470414555));
#37026=CARTESIAN_POINT('Ctrl Pts',(34.1585338443542,1.49958825610693,-34.9678483649439));
#37027=CARTESIAN_POINT('Ctrl Pts',(34.8137969787743,1.49967176946747,-34.9678530956496));
#37028=CARTESIAN_POINT('Ctrl Pts',(35.8017811867034,1.49968797974803,-34.9678539534013));
#37029=CARTESIAN_POINT('Ctrl Pts',(37.7748158892396,1.49978412416472,-34.9678593117153));
#37030=CARTESIAN_POINT('Ctrl Pts',(39.5833333333333,1.49999999999999,-34.967871202114));
#37031=CARTESIAN_POINT('Ctrl Pts',(40.9,1.49999999999999,-34.967871202114));
#37032=CARTESIAN_POINT('Origin',(6.9,-15.,-25.9807621135332));
#37033=CARTESIAN_POINT('',(6.9,8.61681422303452,-28.7358750109634));
#37034=CARTESIAN_POINT('Ctrl Pts',(6.9,3.76156693666918,-10.3676856018661));
#37035=CARTESIAN_POINT('Ctrl Pts',(6.9,4.66834435251375,-14.103554168739));
#37036=CARTESIAN_POINT('Ctrl Pts',(6.90000000166257,5.70305252110769,-18.0191477848531));
#37037=CARTESIAN_POINT('Ctrl Pts',(6.90000000166257,7.22296038005705,-23.666490663791));
#37038=CARTESIAN_POINT('Ctrl Pts',(6.9,7.92134750786925,-26.2182182108371));
#37039=CARTESIAN_POINT('Ctrl Pts',(6.9,8.61681422303452,-28.7358750109634));
#37040=CARTESIAN_POINT('Origin',(6.9,0.,0.));
#37041=CARTESIAN_POINT('Origin',(40.9,-4.5,-7.79422863405994));
#37042=CARTESIAN_POINT('Ctrl Pts',(40.9,-15.9346498339374,-30.5996231131986));
#37043=CARTESIAN_POINT('Ctrl Pts',(40.9,-15.6844024313584,-30.1661818974695));
#37044=CARTESIAN_POINT('Ctrl Pts',(40.9,-15.4341550287793,-29.7327406817405));
#37045=CARTESIAN_POINT('Ctrl Pts',(40.9,-15.1839076262003,-29.2992994660114));
#37046=CARTESIAN_POINT('Ctrl Pts',(30.5,-18.8345266621011,-29.5001797522422));
#37047=CARTESIAN_POINT('Ctrl Pts',(30.5,-18.176307754627,-29.9204226682664));
#37048=CARTESIAN_POINT('Ctrl Pts',(30.5,-17.5,-30.3108891324553));
#37049=CARTESIAN_POINT('Ctrl Pts',(30.5,12.8108891324553,-47.8108891324553));
#37050=CARTESIAN_POINT('Ctrl Pts',(30.5,30.3108891324553,-17.5));
#37051=CARTESIAN_POINT('Ctrl Pts',(30.5,47.8108891324553,12.8108891324553));
#37052=CARTESIAN_POINT('Ctrl Pts',(30.5,17.5,30.3108891324553));
#37053=CARTESIAN_POINT('Ctrl Pts',(30.5,-12.8108891324553,47.8108891324553));
#37054=CARTESIAN_POINT('Ctrl Pts',(30.5,-30.3108891324553,17.5));
#37055=CARTESIAN_POINT('Ctrl Pts',(30.5,-47.0470003722618,-11.4877949884694));
#37056=CARTESIAN_POINT('Ctrl Pts',(30.5,-18.8345266621011,-29.5001797522422));
#37057=CARTESIAN_POINT('Ctrl Pts',(30.3311478274255,-18.7939298193791,-29.4365936489566));
#37058=CARTESIAN_POINT('Ctrl Pts',(30.3311478274255,-18.1371296685291,-29.8559307532302));
#37059=CARTESIAN_POINT('Ctrl Pts',(30.3311478274255,-17.4622796600955,-30.245555587262));
#37060=CARTESIAN_POINT('Ctrl Pts',(30.3311478274255,12.7832759271664,-47.7078352473574));
#37061=CARTESIAN_POINT('Ctrl Pts',(30.3311478274255,30.245555587262,-17.4622796600955));
#37062=CARTESIAN_POINT('Ctrl Pts',(30.3311478274255,47.7078352473574,12.7832759271664));
#37063=CARTESIAN_POINT('Ctrl Pts',(30.3311478274255,17.4622796600955,30.245555587262));
#37064=CARTESIAN_POINT('Ctrl Pts',(30.3311478274255,-12.7832759271664,47.7078352473574));
#37065=CARTESIAN_POINT('Ctrl Pts',(30.3311478274255,-30.245555587262,17.4622796600955));
#37066=CARTESIAN_POINT('Ctrl Pts',(30.3311478274255,-46.9455930096601,-11.4630336437997));
#37067=CARTESIAN_POINT('Ctrl Pts',(30.3311478274255,-18.7939298193791,-29.4365936489566));
#37068=CARTESIAN_POINT('Ctrl Pts',(29.9897712690917,-18.7116961278613,-29.3077924996107));
#37069=CARTESIAN_POINT('Ctrl Pts',(29.9897712690917,-18.0577698358324,-29.7252947753835));
#37070=CARTESIAN_POINT('Ctrl Pts',(29.9897712690917,-17.3858726641896,-30.1132147882992));
#37071=CARTESIAN_POINT('Ctrl Pts',(29.9897712690917,12.7273421241096,-47.4990874524888));
#37072=CARTESIAN_POINT('Ctrl Pts',(29.9897712690917,30.1132147882992,-17.3858726641896));
#37073=CARTESIAN_POINT('Ctrl Pts',(29.9897712690917,47.4990874524888,12.7273421241096));
#37074=CARTESIAN_POINT('Ctrl Pts',(29.9897712690917,17.3858726641896,30.1132147882992));
#37075=CARTESIAN_POINT('Ctrl Pts',(29.9897712690917,-12.7273421241096,47.4990874524888));
#37076=CARTESIAN_POINT('Ctrl Pts',(29.9897712690917,-30.1132147882992,17.3858726641896));
#37077=CARTESIAN_POINT('Ctrl Pts',(29.9897712690917,-46.7401804402414,-11.4128766206768));
#37078=CARTESIAN_POINT('Ctrl Pts',(29.9897712690917,-18.7116961278613,-29.3077924996107));
#37079=CARTESIAN_POINT('Ctrl Pts',(29.4666899049319,-18.5852252487451,-29.1097034403905));
#37080=CARTESIAN_POINT('Ctrl Pts',(29.4666899049319,-17.935718792976,-29.5243838511923));
#37081=CARTESIAN_POINT('Ctrl Pts',(29.4666899049319,-17.2683629213518,-29.9096819433198));
#37082=CARTESIAN_POINT('Ctrl Pts',(29.4666899049319,12.641319021968,-47.1780448646716));
#37083=CARTESIAN_POINT('Ctrl Pts',(29.4666899049319,29.9096819433198,-17.2683629213518));
#37084=CARTESIAN_POINT('Ctrl Pts',(29.4666899049319,47.1780448646716,12.641319021968));
#37085=CARTESIAN_POINT('Ctrl Pts',(29.4666899049319,17.2683629213518,29.9096819433198));
#37086=CARTESIAN_POINT('Ctrl Pts',(29.4666899049319,-12.641319021968,47.1780448646716));
#37087=CARTESIAN_POINT('Ctrl Pts',(29.4666899049319,-29.9096819433198,17.2683629213518));
#37088=CARTESIAN_POINT('Ctrl Pts',(29.4666899049319,-46.4242672450966,-11.3357378872557));
#37089=CARTESIAN_POINT('Ctrl Pts',(29.4666899049319,-18.5852252487451,-29.1097034403905));
#37090=CARTESIAN_POINT('Ctrl Pts',(28.7471241621752,-18.4103340474916,-28.8357745030392));
#37091=CARTESIAN_POINT('Ctrl Pts',(28.7471241621752,-17.7669395953572,-29.246552676757));
#37092=CARTESIAN_POINT('Ctrl Pts',(28.7471241621752,-17.105863694435,-29.6282250261092));
#37093=CARTESIAN_POINT('Ctrl Pts',(28.7471241621752,12.5223613316742,-46.7340887205442));
#37094=CARTESIAN_POINT('Ctrl Pts',(28.7471241621752,29.6282250261092,-17.105863694435));
#37095=CARTESIAN_POINT('Ctrl Pts',(28.7471241621752,46.7340887205442,12.5223613316742));
#37096=CARTESIAN_POINT('Ctrl Pts',(28.7471241621752,17.105863694435,29.6282250261092));
#37097=CARTESIAN_POINT('Ctrl Pts',(28.7471241621752,-12.5223613316742,46.7340887205442));
#37098=CARTESIAN_POINT('Ctrl Pts',(28.7471241621752,-29.6282250261092,17.105863694435));
#37099=CARTESIAN_POINT('Ctrl Pts',(28.7471241621752,-45.9874043199967,-11.2290660127069));
#37100=CARTESIAN_POINT('Ctrl Pts',(28.7471241621752,-18.4103340474916,-28.8357745030392));
#37101=CARTESIAN_POINT('Ctrl Pts',(27.8100958442934,-18.1817092625453,-28.4776836217162));
#37102=CARTESIAN_POINT('Ctrl Pts',(27.8100958442934,-17.5463046664274,-28.8833606347823));
#37103=CARTESIAN_POINT('Ctrl Pts',(27.8100958442934,-16.8934381948013,-29.2602932679205));
#37104=CARTESIAN_POINT('Ctrl Pts',(27.8100958442934,12.3668550731192,-46.1537314627218));
#37105=CARTESIAN_POINT('Ctrl Pts',(27.8100958442934,29.2602932679205,-16.8934381948013));
#37106=CARTESIAN_POINT('Ctrl Pts',(27.8100958442934,46.1537314627218,12.3668550731192));
#37107=CARTESIAN_POINT('Ctrl Pts',(27.8100958442934,16.8934381948013,29.2602932679205));
#37108=CARTESIAN_POINT('Ctrl Pts',(27.8100958442934,-12.3668550731192,46.1537314627218));
#37109=CARTESIAN_POINT('Ctrl Pts',(27.8100958442934,-29.2602932679205,16.8934381948013));
#37110=CARTESIAN_POINT('Ctrl Pts',(27.8100958442934,-45.4163196022628,-11.0896202647003));
#37111=CARTESIAN_POINT('Ctrl Pts',(27.8100958442934,-18.1817092625453,-28.4776836217162));
#37112=CARTESIAN_POINT('Ctrl Pts',(26.8343111708818,-17.9446806017473,-28.1064299010669));
#37113=CARTESIAN_POINT('Ctrl Pts',(26.8343111708818,-17.3175595557791,-28.5068182430991));
#37114=CARTESIAN_POINT('Ctrl Pts',(26.8343111708818,-16.6732042787396,-28.8788369357517));
#37115=CARTESIAN_POINT('Ctrl Pts',(26.8343111708818,12.2056326570121,-45.5520412144912));
#37116=CARTESIAN_POINT('Ctrl Pts',(26.8343111708818,28.8788369357517,-16.6732042787396));
#37117=CARTESIAN_POINT('Ctrl Pts',(26.8343111708818,45.5520412144912,12.2056326570121));
#37118=CARTESIAN_POINT('Ctrl Pts',(26.8343111708818,16.6732042787396,28.8788369357517));
#37119=CARTESIAN_POINT('Ctrl Pts',(26.8343111708818,-12.2056326570121,45.5520412144912));
#37120=CARTESIAN_POINT('Ctrl Pts',(26.8343111708818,-28.8788369357517,16.6732042787396));
#37121=CARTESIAN_POINT('Ctrl Pts',(26.8343111708818,-44.8242427376375,-10.9450487174303));
#37122=CARTESIAN_POINT('Ctrl Pts',(26.8343111708818,-17.9446806017473,-28.1064299010669));
#37123=CARTESIAN_POINT('Ctrl Pts',(25.8181479469611,-17.7025946652472,-27.7272550606068));
#37124=CARTESIAN_POINT('Ctrl Pts',(25.8181479469611,-17.0839339083798,-28.1222418918016));
#37125=CARTESIAN_POINT('Ctrl Pts',(25.8181479469611,-16.4482714219305,-28.4892417994668));
#37126=CARTESIAN_POINT('Ctrl Pts',(25.8181479469611,12.0409703775363,-44.9375132213974));
#37127=CARTESIAN_POINT('Ctrl Pts',(25.8181479469611,28.4892417994668,-16.4482714219305));
#37128=CARTESIAN_POINT('Ctrl Pts',(25.8181479469611,44.9375132213974,12.0409703775363));
#37129=CARTESIAN_POINT('Ctrl Pts',(25.8181479469611,16.4482714219305,28.4892417994668));
#37130=CARTESIAN_POINT('Ctrl Pts',(25.8181479469611,-12.0409703775363,44.9375132213974));
#37131=CARTESIAN_POINT('Ctrl Pts',(25.8181479469611,-28.4892417994668,16.4482714219305));
#37132=CARTESIAN_POINT('Ctrl Pts',(25.8181479469611,-44.2195332406074,-10.7973925719907));
#37133=CARTESIAN_POINT('Ctrl Pts',(25.8181479469611,-17.7025946652472,-27.7272550606068));
#37134=CARTESIAN_POINT('Ctrl Pts',(24.7595197917227,-17.4614959928472,-27.3496265541183));
#37135=CARTESIAN_POINT('Ctrl Pts',(24.7595197917227,-16.8512610227058,-27.739233902677));
#37136=CARTESIAN_POINT('Ctrl Pts',(24.7595197917227,-16.2242558762949,-28.1012354927406));
#37137=CARTESIAN_POINT('Ctrl Pts',(24.7595197917227,11.8769796164457,-44.3254913690355));
#37138=CARTESIAN_POINT('Ctrl Pts',(24.7595197917227,28.1012354927406,-16.2242558762949));
#37139=CARTESIAN_POINT('Ctrl Pts',(24.7595197917227,44.3254913690355,11.8769796164457));
#37140=CARTESIAN_POINT('Ctrl Pts',(24.7595197917227,16.2242558762949,28.1012354927406));
#37141=CARTESIAN_POINT('Ctrl Pts',(24.7595197917227,-11.8769796164457,44.3254913690355));
#37142=CARTESIAN_POINT('Ctrl Pts',(24.7595197917227,-28.1012354927406,16.2242558762949));
#37143=CARTESIAN_POINT('Ctrl Pts',(24.7595197917227,-43.6172898429552,-10.6503385912768));
#37144=CARTESIAN_POINT('Ctrl Pts',(24.7595197917227,-17.4614959928472,-27.3496265541183));
#37145=CARTESIAN_POINT('Ctrl Pts',(23.6563574780851,-17.229354682426,-26.9860278023044));
#37146=CARTESIAN_POINT('Ctrl Pts',(23.6563574780851,-16.627232461942,-27.370455528196));
#37147=CARTESIAN_POINT('Ctrl Pts',(23.6563574780851,-16.0085630157705,-27.7276444994825));
#37148=CARTESIAN_POINT('Ctrl Pts',(23.6563574780851,11.719081483712,-43.736207515253));
#37149=CARTESIAN_POINT('Ctrl Pts',(23.6563574780851,27.7276444994825,-16.0085630157705));
#37150=CARTESIAN_POINT('Ctrl Pts',(23.6563574780851,43.736207515253,11.719081483712));
#37151=CARTESIAN_POINT('Ctrl Pts',(23.6563574780851,16.0085630157705,27.7276444994825));
#37152=CARTESIAN_POINT('Ctrl Pts',(23.6563574780851,-11.719081483712,43.736207515253));
#37153=CARTESIAN_POINT('Ctrl Pts',(23.6563574780851,-27.7276444994825,16.0085630157705));
#37154=CARTESIAN_POINT('Ctrl Pts',(23.6563574780851,-43.0374211521332,-10.5087479991522));
#37155=CARTESIAN_POINT('Ctrl Pts',(23.6563574780851,-17.229354682426,-26.9860278023044));
#37156=CARTESIAN_POINT('Ctrl Pts',(22.5073180101405,-17.0145388530744,-26.649565639321));
#37157=CARTESIAN_POINT('Ctrl Pts',(22.5073180101405,-16.419923900654,-27.029200315079));
#37158=CARTESIAN_POINT('Ctrl Pts',(22.5073180101405,-15.8089680335819,-27.3819358493961));
#37159=CARTESIAN_POINT('Ctrl Pts',(22.5073180101405,11.5729678158142,-43.190903882978));
#37160=CARTESIAN_POINT('Ctrl Pts',(22.5073180101405,27.3819358493961,-15.8089680335819));
#37161=CARTESIAN_POINT('Ctrl Pts',(22.5073180101405,43.190903882978,11.5729678158142));
#37162=CARTESIAN_POINT('Ctrl Pts',(22.5073180101405,15.8089680335819,27.3819358493961));
#37163=CARTESIAN_POINT('Ctrl Pts',(22.5073180101405,-11.5729678158142,43.190903882978));
#37164=CARTESIAN_POINT('Ctrl Pts',(22.5073180101405,-27.3819358493961,15.8089680335819));
#37165=CARTESIAN_POINT('Ctrl Pts',(22.5073180101405,-42.5008299977716,-10.3777247856603));
#37166=CARTESIAN_POINT('Ctrl Pts',(22.5073180101405,-17.0145388530744,-26.649565639321));
#37167=CARTESIAN_POINT('Ctrl Pts',(21.3125219557939,-16.8244723890963,-26.3518679613905));
#37168=CARTESIAN_POINT('Ctrl Pts',(21.3125219557939,-16.2364997772301,-26.727261803997));
#37169=CARTESIAN_POINT('Ctrl Pts',(21.3125219557939,-15.632368792237,-27.0760569908086));
#37170=CARTESIAN_POINT('Ctrl Pts',(21.3125219557939,11.4436881985716,-42.7084257830456));
#37171=CARTESIAN_POINT('Ctrl Pts',(21.3125219557939,27.0760569908086,-15.632368792237));
#37172=CARTESIAN_POINT('Ctrl Pts',(21.3125219557939,42.7084257830456,11.4436881985716));
#37173=CARTESIAN_POINT('Ctrl Pts',(21.3125219557939,15.632368792237,27.0760569908086));
#37174=CARTESIAN_POINT('Ctrl Pts',(21.3125219557939,-11.4436881985716,42.7084257830456));
#37175=CARTESIAN_POINT('Ctrl Pts',(21.3125219557939,-27.0760569908086,15.632368792237));
#37176=CARTESIAN_POINT('Ctrl Pts',(21.3125219557939,-42.0260605935833,-10.2617970211066));
#37177=CARTESIAN_POINT('Ctrl Pts',(21.3125219557939,-16.8244723890963,-26.3518679613905));
#37178=CARTESIAN_POINT('Ctrl Pts',(20.0742472323676,-16.6643225955233,-26.1010282252799));
#37179=CARTESIAN_POINT('Ctrl Pts',(20.0742472323676,-16.0819468125049,-26.4728487465358));
#37180=CARTESIAN_POINT('Ctrl Pts',(20.0742472323676,-15.4835664656478,-26.8183238008715));
#37181=CARTESIAN_POINT('Ctrl Pts',(20.0742472323676,11.3347573352238,-42.3018902665193));
#37182=CARTESIAN_POINT('Ctrl Pts',(20.0742472323676,26.8183238008715,-15.4835664656478));
#37183=CARTESIAN_POINT('Ctrl Pts',(20.0742472323676,42.3018902665193,11.3347573352238));
#37184=CARTESIAN_POINT('Ctrl Pts',(20.0742472323676,15.4835664656478,26.8183238008715));
#37185=CARTESIAN_POINT('Ctrl Pts',(20.0742472323676,-11.3347573352238,42.3018902665193));
#37186=CARTESIAN_POINT('Ctrl Pts',(20.0742472323676,-26.8183238008715,15.4835664656478));
#37187=CARTESIAN_POINT('Ctrl Pts',(20.0742472323676,-41.6260204156154,-10.1641164141543));
#37188=CARTESIAN_POINT('Ctrl Pts',(20.0742472323676,-16.6643225955233,-26.1010282252799));
#37189=CARTESIAN_POINT('Ctrl Pts',(18.7979917002302,-16.5352770548748,-25.8989065200918));
#37190=CARTESIAN_POINT('Ctrl Pts',(18.7979917002302,-15.9574110860028,-26.2678477295776));
#37191=CARTESIAN_POINT('Ctrl Pts',(18.7979917002302,-15.3636644897785,-26.6106474867381));
#37192=CARTESIAN_POINT('Ctrl Pts',(18.7979917002302,11.2469829969596,-41.9743119765166));
#37193=CARTESIAN_POINT('Ctrl Pts',(18.7979917002302,26.6106474867381,-15.3636644897785));
#37194=CARTESIAN_POINT('Ctrl Pts',(18.7979917002302,41.9743119765166,11.2469829969596));
#37195=CARTESIAN_POINT('Ctrl Pts',(18.7979917002302,15.3636644897785,26.6106474867381));
#37196=CARTESIAN_POINT('Ctrl Pts',(18.7979917002302,-11.2469829969596,41.9743119765166));
#37197=CARTESIAN_POINT('Ctrl Pts',(18.7979917002302,-26.6106474867381,15.3636644897785));
#37198=CARTESIAN_POINT('Ctrl Pts',(18.7979917002302,-41.303675941138,-10.0854073102973));
#37199=CARTESIAN_POINT('Ctrl Pts',(18.7979917002302,-16.5352770548748,-25.8989065200918));
#37200=CARTESIAN_POINT('Ctrl Pts',(17.4917404060759,-16.4351406788133,-25.7420647185138));
#37201=CARTESIAN_POINT('Ctrl Pts',(17.4917404060759,-15.8607742221527,-26.1087716481884));
#37202=CARTESIAN_POINT('Ctrl Pts',(17.4917404060759,-15.2706233100072,-26.4494954361781));
#37203=CARTESIAN_POINT('Ctrl Pts',(17.4917404060759,11.1788721261709,-41.7201187461852));
#37204=CARTESIAN_POINT('Ctrl Pts',(17.4917404060759,26.4494954361781,-15.2706233100072));
#37205=CARTESIAN_POINT('Ctrl Pts',(17.4917404060759,41.7201187461852,11.1788721261709));
#37206=CARTESIAN_POINT('Ctrl Pts',(17.4917404060759,15.2706233100072,26.4494954361781));
#37207=CARTESIAN_POINT('Ctrl Pts',(17.4917404060759,-11.1788721261709,41.7201187461852));
#37208=CARTESIAN_POINT('Ctrl Pts',(17.4917404060759,-26.4494954361781,15.2706233100072));
#37209=CARTESIAN_POINT('Ctrl Pts',(17.4917404060759,-41.0535440314616,-10.0243308532288));
#37210=CARTESIAN_POINT('Ctrl Pts',(17.4917404060759,-16.4351406788133,-25.7420647185138));
#37211=CARTESIAN_POINT('Ctrl Pts',(16.1647270995715,-16.3596108683728,-25.6237637373094));
#37212=CARTESIAN_POINT('Ctrl Pts',(16.1647270995715,-15.7878839869031,-25.988785417954));
#37213=CARTESIAN_POINT('Ctrl Pts',(16.1647270995715,-15.2004451894512,-26.3279433657953));
#37214=CARTESIAN_POINT('Ctrl Pts',(16.1647270995715,11.1274981763441,-41.5283885552464));
#37215=CARTESIAN_POINT('Ctrl Pts',(16.1647270995715,26.3279433657953,-15.2004451894512));
#37216=CARTESIAN_POINT('Ctrl Pts',(16.1647270995715,41.5283885552464,11.1274981763441));
#37217=CARTESIAN_POINT('Ctrl Pts',(16.1647270995715,15.2004451894512,26.3279433657953));
#37218=CARTESIAN_POINT('Ctrl Pts',(16.1647270995715,-11.1274981763441,41.5283885552464));
#37219=CARTESIAN_POINT('Ctrl Pts',(16.1647270995715,-26.3279433657953,15.2004451894512));
#37220=CARTESIAN_POINT('Ctrl Pts',(16.1647270995715,-40.8648771706659,-9.97826274685029));
#37221=CARTESIAN_POINT('Ctrl Pts',(16.1647270995715,-16.3596108683728,-25.6237637373094));
#37222=CARTESIAN_POINT('Ctrl Pts',(14.8263876417415,-16.3032840624315,-25.5355400760542));
#37223=CARTESIAN_POINT('Ctrl Pts',(14.8263876417415,-15.7335256598799,-25.8993049721986));
#37224=CARTESIAN_POINT('Ctrl Pts',(14.8263876417415,-15.1481094381123,-26.2372951854241));
#37225=CARTESIAN_POINT('Ctrl Pts',(14.8263876417415,11.0891857473118,-41.3854046235364));
#37226=CARTESIAN_POINT('Ctrl Pts',(14.8263876417415,26.2372951854241,-15.1481094381123));
#37227=CARTESIAN_POINT('Ctrl Pts',(14.8263876417415,41.3854046235364,11.0891857473118));
#37228=CARTESIAN_POINT('Ctrl Pts',(14.8263876417415,15.1481094381123,26.2372951854241));
#37229=CARTESIAN_POINT('Ctrl Pts',(14.8263876417415,-11.0891857473118,41.3854046235364));
#37230=CARTESIAN_POINT('Ctrl Pts',(14.8263876417415,-26.2372951854241,15.1481094381123));
#37231=CARTESIAN_POINT('Ctrl Pts',(14.8263876417415,-40.7241777356532,-9.94390718216752));
#37232=CARTESIAN_POINT('Ctrl Pts',(14.8263876417415,-16.3032840624315,-25.5355400760542));
#37233=CARTESIAN_POINT('Ctrl Pts',(13.4853470903953,-16.260659159851,-25.4687774591536));
#37234=CARTESIAN_POINT('Ctrl Pts',(13.4853470903953,-15.6923903894687,-25.8315912927267));
#37235=CARTESIAN_POINT('Ctrl Pts',(13.4853470903953,-15.1085047372063,-26.1686978312363));
#37236=CARTESIAN_POINT('Ctrl Pts',(13.4853470903953,11.06019309403,-41.2772025684426));
#37237=CARTESIAN_POINT('Ctrl Pts',(13.4853470903953,26.1686978312363,-15.1085047372063));
#37238=CARTESIAN_POINT('Ctrl Pts',(13.4853470903953,41.2772025684426,11.06019309403));
#37239=CARTESIAN_POINT('Ctrl Pts',(13.4853470903953,15.1085047372063,26.1686978312363));
#37240=CARTESIAN_POINT('Ctrl Pts',(13.4853470903953,-11.06019309403,41.2772025684426));
#37241=CARTESIAN_POINT('Ctrl Pts',(13.4853470903953,-26.1686978312363,15.1085047372063));
#37242=CARTESIAN_POINT('Ctrl Pts',(13.4853470903953,-40.617704456895,-9.91790885733393));
#37243=CARTESIAN_POINT('Ctrl Pts',(13.4853470903953,-16.260659159851,-25.4687774591536));
#37244=CARTESIAN_POINT('Ctrl Pts',(12.1482076787549,-16.2272643834928,-25.4164718226475));
#37245=CARTESIAN_POINT('Ctrl Pts',(12.1482076787549,-15.660162675793,-25.778540539635));
#37246=CARTESIAN_POINT('Ctrl Pts',(12.1482076787549,-15.0774761588537,-26.1149547570431));
#37247=CARTESIAN_POINT('Ctrl Pts',(12.1482076787549,11.0374785981893,-41.1924309158968));
#37248=CARTESIAN_POINT('Ctrl Pts',(12.1482076787549,26.1149547570431,-15.0774761588537));
#37249=CARTESIAN_POINT('Ctrl Pts',(12.1482076787549,41.1924309158968,11.0374785981893));
#37250=CARTESIAN_POINT('Ctrl Pts',(12.1482076787549,15.0774761588537,26.1149547570431));
#37251=CARTESIAN_POINT('Ctrl Pts',(12.1482076787549,-11.0374785981893,41.1924309158968));
#37252=CARTESIAN_POINT('Ctrl Pts',(12.1482076787549,-26.1149547570431,15.0774761588537));
#37253=CARTESIAN_POINT('Ctrl Pts',(12.1482076787549,-40.534287226192,-9.89754028893977));
#37254=CARTESIAN_POINT('Ctrl Pts',(12.1482076787549,-16.2272643834928,-25.4164718226475));
#37255=CARTESIAN_POINT('Ctrl Pts',(10.8190675759626,-16.2001953420791,-25.3740740708084));
#37256=CARTESIAN_POINT('Ctrl Pts',(10.8190675759626,-15.6340396286792,-25.7355388133451));
#37257=CARTESIAN_POINT('Ctrl Pts',(10.8190675759626,-15.0523251033885,-26.0713918511132));
#37258=CARTESIAN_POINT('Ctrl Pts',(10.8190675759626,11.0190667477248,-41.1237169545017));
#37259=CARTESIAN_POINT('Ctrl Pts',(10.8190675759626,26.0713918511132,-15.0523251033885));
#37260=CARTESIAN_POINT('Ctrl Pts',(10.8190675759626,41.1237169545017,11.0190667477248));
#37261=CARTESIAN_POINT('Ctrl Pts',(10.8190675759626,15.0523251033885,26.0713918511132));
#37262=CARTESIAN_POINT('Ctrl Pts',(10.8190675759626,-11.0190667477248,41.1237169545017));
#37263=CARTESIAN_POINT('Ctrl Pts',(10.8190675759626,-26.0713918511132,15.0523251033885));
#37264=CARTESIAN_POINT('Ctrl Pts',(10.8190675759626,-40.4666711281441,-9.88102999357242));
#37265=CARTESIAN_POINT('Ctrl Pts',(10.8190675759626,-16.2001953420791,-25.3740740708084));
#37266=CARTESIAN_POINT('Ctrl Pts',(9.50027713254189,-16.1776521900286,-25.3387651379321));
#37267=CARTESIAN_POINT('Ctrl Pts',(9.50027713254189,-15.6122843025816,-25.6997268893331));
#37268=CARTESIAN_POINT('Ctrl Pts',(9.50027713254189,-15.0313792538877,-26.0351125755702));
#37269=CARTESIAN_POINT('Ctrl Pts',(9.50027713254189,11.0037333216825,-41.0664918294579));
#37270=CARTESIAN_POINT('Ctrl Pts',(9.50027713254189,26.0351125755702,-15.0313792538877));
#37271=CARTESIAN_POINT('Ctrl Pts',(9.5002771325419,41.0664918294579,11.0037333216825));
#37272=CARTESIAN_POINT('Ctrl Pts',(9.5002771325419,15.0313792538877,26.0351125755702));
#37273=CARTESIAN_POINT('Ctrl Pts',(9.5002771325419,-11.0037333216825,41.0664918294579));
#37274=CARTESIAN_POINT('Ctrl Pts',(9.50027713254189,-26.0351125755702,15.0313792538877));
#37275=CARTESIAN_POINT('Ctrl Pts',(9.50027713254189,-40.4103603059007,-9.86728018643389));
#37276=CARTESIAN_POINT('Ctrl Pts',(9.50027713254189,-16.1776521900286,-25.3387651379321));
#37277=CARTESIAN_POINT('Ctrl Pts',(8.45435372222587,-16.1625070777669,-25.3150436214797));
#37278=CARTESIAN_POINT('Ctrl Pts',(8.45435372222587,-15.5976684735573,-25.6756674495416));
#37279=CARTESIAN_POINT('Ctrl Pts',(8.45435372222587,-15.0173072536015,-26.0107391561104));
#37280=CARTESIAN_POINT('Ctrl Pts',(8.45435372222587,10.9934319025089,-41.0280464097118));
#37281=CARTESIAN_POINT('Ctrl Pts',(8.45435372222587,26.0107391561104,-15.0173072536015));
#37282=CARTESIAN_POINT('Ctrl Pts',(8.45435372222587,41.0280464097118,10.9934319025089));
#37283=CARTESIAN_POINT('Ctrl Pts',(8.45435372222587,15.0173072536015,26.0107391561104));
#37284=CARTESIAN_POINT('Ctrl Pts',(8.45435372222587,-10.9934319025089,41.0280464097118));
#37285=CARTESIAN_POINT('Ctrl Pts',(8.45435372222587,-26.0107391561104,15.0173072536015));
#37286=CARTESIAN_POINT('Ctrl Pts',(8.45435372222587,-40.3725291400319,-9.85804268618443));
#37287=CARTESIAN_POINT('Ctrl Pts',(8.45435372222587,-16.1625070777669,-25.3150436214797));
#37288=CARTESIAN_POINT('Ctrl Pts',(7.67514864245731,-16.1526223715399,-25.2995613842179));
#37289=CARTESIAN_POINT('Ctrl Pts',(7.67514864245731,-15.5881292127269,-25.6599646610633));
#37290=CARTESIAN_POINT('Ctrl Pts',(7.67514864245731,-15.0081229315276,-25.9948314436453));
#37291=CARTESIAN_POINT('Ctrl Pts',(7.67514864245731,10.9867085121177,-41.0029543751729));
#37292=CARTESIAN_POINT('Ctrl Pts',(7.67514864245731,25.9948314436453,-15.0081229315276));
#37293=CARTESIAN_POINT('Ctrl Pts',(7.67514864245731,41.0029543751729,10.9867085121177));
#37294=CARTESIAN_POINT('Ctrl Pts',(7.67514864245731,15.0081229315276,25.9948314436453));
#37295=CARTESIAN_POINT('Ctrl Pts',(7.67514864245731,-10.9867085121177,41.0029543751729));
#37296=CARTESIAN_POINT('Ctrl Pts',(7.67514864245731,-25.9948314436453,15.0081229315276));
#37297=CARTESIAN_POINT('Ctrl Pts',(7.67514864245731,-40.3478380083732,-9.85201367995056));
#37298=CARTESIAN_POINT('Ctrl Pts',(7.67514864245731,-16.1526223715399,-25.2995613842179));
#37299=CARTESIAN_POINT('Ctrl Pts',(7.15799654185577,-16.1466853364124,-25.2902623130707));
#37300=CARTESIAN_POINT('Ctrl Pts',(7.15799654185577,-15.5823996619098,-25.6505331205953));
#37301=CARTESIAN_POINT('Ctrl Pts',(7.15799654185577,-15.0026065670023,-25.9852768200144));
#37302=CARTESIAN_POINT('Ctrl Pts',(7.15799654185577,10.9826702530121,-40.9878833870167));
#37303=CARTESIAN_POINT('Ctrl Pts',(7.15799654185577,25.9852768200144,-15.0026065670023));
#37304=CARTESIAN_POINT('Ctrl Pts',(7.15799654185577,40.9878833870167,10.9826702530121));
#37305=CARTESIAN_POINT('Ctrl Pts',(7.15799654185577,15.0026065670023,25.9852768200144));
#37306=CARTESIAN_POINT('Ctrl Pts',(7.15799654185577,-10.9826702530121,40.9878833870167));
#37307=CARTESIAN_POINT('Ctrl Pts',(7.15799654185577,-25.9852768200144,15.0026065670023));
#37308=CARTESIAN_POINT('Ctrl Pts',(7.15799654185577,-40.3330078138659,-9.84839248767921));
#37309=CARTESIAN_POINT('Ctrl Pts',(7.15799654185577,-16.1466853364124,-25.2902623130707));
#37310=CARTESIAN_POINT('Ctrl Pts',(6.9,-16.1438799960867,-25.2858683590648));
#37311=CARTESIAN_POINT('Ctrl Pts',(6.9,-15.5796923611089,-25.6460765727998));
#37312=CARTESIAN_POINT('Ctrl Pts',(6.9,-15.,-25.9807621135332));
#37313=CARTESIAN_POINT('Ctrl Pts',(6.9,10.9807621135331,-40.9807621135332));
#37314=CARTESIAN_POINT('Ctrl Pts',(6.9,25.9807621135332,-15.));
#37315=CARTESIAN_POINT('Ctrl Pts',(6.9,40.9807621135332,10.9807621135331));
#37316=CARTESIAN_POINT('Ctrl Pts',(6.9,15.,25.9807621135332));
#37317=CARTESIAN_POINT('Ctrl Pts',(6.9,-10.9807621135331,40.9807621135332));
#37318=CARTESIAN_POINT('Ctrl Pts',(6.9,-25.9807621135332,15.));
#37319=CARTESIAN_POINT('Ctrl Pts',(6.9,-40.3260003190816,-9.84668141868802));
#37320=CARTESIAN_POINT('Ctrl Pts',(6.9,-16.1438799960867,-25.2858683590648));
#37321=CARTESIAN_POINT('Ctrl Pts',(6.9,8.61681422303452,-28.7358750109634));
#37322=CARTESIAN_POINT('Ctrl Pts',(7.85773098116326,6.72950262532882,-29.3220126177434));
#37323=CARTESIAN_POINT('Ctrl Pts',(8.88781981167334,4.83176468807715,-29.7139609348499));
#37324=CARTESIAN_POINT('Ctrl Pts',(10.5914578196776,1.83991777043966,-30.0626260759601));
#37325=CARTESIAN_POINT('Ctrl Pts',(11.2365058953701,0.737334477600518,-30.1308526921615));
#37326=CARTESIAN_POINT('Ctrl Pts',(12.0558885382926,-0.564998386426074,
-30.1493644860168));
#37327=CARTESIAN_POINT('Ctrl Pts',(12.1875764958397,-0.770798830274841,
-30.1503477937894));
#37328=CARTESIAN_POINT('Ctrl Pts',(13.194901830313,-2.32835059063961,-30.1433772121647));
#37329=CARTESIAN_POINT('Ctrl Pts',(14.2258982134098,-3.91692083548089,-30.0606334052373));
#37330=CARTESIAN_POINT('Ctrl Pts',(18.2616480823244,-8.94354621773405,-29.4024246647732));
#37331=CARTESIAN_POINT('Ctrl Pts',(21.0496416709525,-11.660889676038,-28.796919295079));
#37332=CARTESIAN_POINT('Ctrl Pts',(25.8000196361138,-14.7241675584603,-29.3778263502455));
#37333=CARTESIAN_POINT('Ctrl Pts',(26.8976561124457,-15.1580512376427,-29.7353019177929));
#37334=CARTESIAN_POINT('Ctrl Pts',(28.0045908801237,-15.5447817028247,-30.0977443108623));
#37335=CARTESIAN_POINT('Ctrl Pts',(28.5235971652406,-15.6994510084801,-30.2828992744991));
#37336=CARTESIAN_POINT('Ctrl Pts',(29.0834839543824,-15.8677990842846,-30.4804113157011));
#37337=CARTESIAN_POINT('Ctrl Pts',(29.1146288039499,-15.877207296405,-30.4913713634453));
#37338=CARTESIAN_POINT('Ctrl Pts',(29.5949306848436,-16.0210111630069,-30.6609898319163));
#37339=CARTESIAN_POINT('Ctrl Pts',(30.0492939924726,-16.1312811324031,-30.8338536064743));
#37340=CARTESIAN_POINT('Ctrl Pts',(30.5,-16.229443021655,-31.0097594187194));
#37341=CARTESIAN_POINT('Ctrl Pts',(6.45331003273164,4.07387898226151,-10.2495589536195));
#37342=CARTESIAN_POINT('Ctrl Pts',(7.20830533428676,3.54117612793134,-10.4589493929845));
#37343=CARTESIAN_POINT('Ctrl Pts',(7.99943720515023,3.00808536723907,-10.6278530262204));
#37344=CARTESIAN_POINT('Ctrl Pts',(9.76195392812149,1.87226624217412,-10.8974188156737));
#37345=CARTESIAN_POINT('Ctrl Pts',(10.7319699357145,1.2567580486118,-10.978614804603));
#37346=CARTESIAN_POINT('Ctrl Pts',(12.6618070777417,0.165209663835397,-11.0581512103982));
#37347=CARTESIAN_POINT('Ctrl Pts',(13.6366888866736,-0.364704064273056,
-11.0460663569154));
#37348=CARTESIAN_POINT('Ctrl Pts',(15.55636942495,-1.27025231764748,-10.9884970038505));
#37349=CARTESIAN_POINT('Ctrl Pts',(16.5294822240034,-1.69980161462952,-10.9232664847119));
#37350=CARTESIAN_POINT('Ctrl Pts',(18.4405353898674,-2.41132585012622,-10.79829507883));
#37351=CARTESIAN_POINT('Ctrl Pts',(19.4148048972756,-2.74047342809724,-10.7128845485963));
#37352=CARTESIAN_POINT('Ctrl Pts',(20.6320159197513,-3.0737286362331,-10.6248232626625));
#37353=CARTESIAN_POINT('Ctrl Pts',(21.104508195865,-3.19855905527614,-10.5890632628362));
#37354=CARTESIAN_POINT('Ctrl Pts',(22.0534615876999,-3.42883778652051,-10.5175158204589));
#37355=CARTESIAN_POINT('Ctrl Pts',(22.7823820470182,-3.58029681662341,-10.4664588970829));
#37356=CARTESIAN_POINT('Ctrl Pts',(23.3297776630266,-3.67835397010644,-10.4341170945838));
#37357=CARTESIAN_POINT('Ctrl Pts',(23.4470599317458,-3.69902619132825,-10.4271412460567));
#37358=CARTESIAN_POINT('Ctrl Pts',(23.6811266122299,-3.73910834650869,-10.4133903945396));
#37359=CARTESIAN_POINT('Ctrl Pts',(24.0941730950848,-3.80664723977492,-10.3895545652128));
#37360=CARTESIAN_POINT('Ctrl Pts',(24.6899146335615,-3.89464075109998,-10.3570603924451));
#37361=CARTESIAN_POINT('Ctrl Pts',(25.291236117096,-3.96994444386567,-10.3283061836387));
#37362=CARTESIAN_POINT('Ctrl Pts',(25.7735285180351,-4.02162740546582,-10.308597305488));
#37363=CARTESIAN_POINT('Ctrl Pts',(26.0148283477099,-4.04448759176679,-10.3000025859217));
#37364=CARTESIAN_POINT('Ctrl Pts',(26.5981242438444,-4.09600397233591,-10.2809495486037));
#37365=CARTESIAN_POINT('Ctrl Pts',(27.5413774795629,-4.1475207788653,-10.2607319091994));
#37366=CARTESIAN_POINT('Ctrl Pts',(28.5384263877914,-4.17105255246827,-10.2503835882543));
#37367=CARTESIAN_POINT('Ctrl Pts',(29.1235503058368,-4.18584784382925,-10.2444533826691));
#37368=CARTESIAN_POINT('Ctrl Pts',(29.28127198738,-4.1893484810251,-10.2430815653883));
#37369=CARTESIAN_POINT('Ctrl Pts',(29.6033573831699,-4.19465178436654,-10.2409825864505));
#37370=CARTESIAN_POINT('Ctrl Pts',(30.1682075695059,-4.19956029863432,-10.23904328544));
#37371=CARTESIAN_POINT('Ctrl Pts',(31.3151152846708,-4.19601580459665,-10.2404426493562));
#37372=CARTESIAN_POINT('Ctrl Pts',(32.3203773995796,-4.18330340731801,-10.2455622764131));
#37373=CARTESIAN_POINT('Ctrl Pts',(33.1677006908681,-4.18329188254757,-10.2455713422049));
#37374=CARTESIAN_POINT('Ctrl Pts',(33.4949132850989,-4.18329063364474,-10.2455724350351));
#37375=CARTESIAN_POINT('Ctrl Pts',(34.1541785734606,-4.18328832445805,-10.2455743198854));
#37376=CARTESIAN_POINT('Ctrl Pts',(34.9761291047989,-4.18328098024985,-10.2455804319183));
#37377=CARTESIAN_POINT('Ctrl Pts',(35.9637295000903,-4.18327789132126,-10.2455829874647));
#37378=CARTESIAN_POINT('Ctrl Pts',(37.9383590406839,-4.18327370253668,-10.2455864680815));
#37379=CARTESIAN_POINT('Ctrl Pts',(39.5833333333333,-4.18325179103929,-10.2456046429335));
#37380=CARTESIAN_POINT('Ctrl Pts',(40.9,-4.18325179103929,-10.2456046429335));
#37381=CARTESIAN_POINT('Ctrl Pts',(6.63336813585096,4.85602971916216,-13.590868440034));
#37382=CARTESIAN_POINT('Ctrl Pts',(7.389696336477,4.14888858981181,-13.8391951107513));
#37383=CARTESIAN_POINT('Ctrl Pts',(8.18053946683774,3.44401143686367,-14.0346488726453));
#37384=CARTESIAN_POINT('Ctrl Pts',(9.94201947683641,1.94757748540837,-14.3333081335907));
#37385=CARTESIAN_POINT('Ctrl Pts',(10.9113717350149,1.13915583855168,-14.4104989873604));
#37386=CARTESIAN_POINT('Ctrl Pts',(12.834739732217,-0.286629408466326,-14.4628660834126));
#37387=CARTESIAN_POINT('Ctrl Pts',(13.808142871698,-0.978270473832919,-14.422640991687));
#37388=CARTESIAN_POINT('Ctrl Pts',(15.7151185916567,-2.15221389622411,-14.3061107665235));
#37389=CARTESIAN_POINT('Ctrl Pts',(16.6852254797785,-2.70962741922243,-14.2015789338064));
#37390=CARTESIAN_POINT('Ctrl Pts',(18.5768226767694,-3.62608620812781,-14.0076819635675));
#37391=CARTESIAN_POINT('Ctrl Pts',(19.5464729449596,-4.05120533415428,-13.8818273075211));
#37392=CARTESIAN_POINT('Ctrl Pts',(20.7463406818481,-4.47793026920171,-13.7535017581768));
#37393=CARTESIAN_POINT('Ctrl Pts',(21.2156214332096,-4.63869318435443,-13.7015810566901));
#37394=CARTESIAN_POINT('Ctrl Pts',(22.1537708528638,-4.93390876526188,-13.5988388255708));
#37395=CARTESIAN_POINT('Ctrl Pts',(22.8728508922896,-5.12767073297797,-13.5262523639446));
#37396=CARTESIAN_POINT('Ctrl Pts',(23.4112391022537,-5.25280074041751,-13.4803679794399));
#37397=CARTESIAN_POINT('Ctrl Pts',(23.5274006995053,-5.27931561824263,-13.4704404449521));
#37398=CARTESIAN_POINT('Ctrl Pts',(23.7586975975699,-5.33062970711066,-13.4509289072633));
#37399=CARTESIAN_POINT('Ctrl Pts',(24.1668938536998,-5.41708560365394,-13.4171810922989));
#37400=CARTESIAN_POINT('Ctrl Pts',(24.7548128660956,-5.52956305821881,-13.3713845002051));
#37401=CARTESIAN_POINT('Ctrl Pts',(25.3473131502196,-5.6256707359588,-13.3310219589391));
#37402=CARTESIAN_POINT('Ctrl Pts',(25.821804155628,-5.6915437851135,-13.3034028562424));
#37403=CARTESIAN_POINT('Ctrl Pts',(26.0589587666351,-5.72065900880545,-13.2913640661324));
#37404=CARTESIAN_POINT('Ctrl Pts',(26.631694838376,-5.78623492045641,-13.2646759506015));
#37405=CARTESIAN_POINT('Ctrl Pts',(27.5576851463965,-5.85186367837986,-13.2364409873879));
#37406=CARTESIAN_POINT('Ctrl Pts',(28.5507795710393,-5.88219883517418,-13.221915949884));
#37407=CARTESIAN_POINT('Ctrl Pts',(29.1361849357886,-5.90128718803101,-13.2135466774644));
#37408=CARTESIAN_POINT('Ctrl Pts',(29.2912521292176,-5.90574282943919,-13.2116327381159));
#37409=CARTESIAN_POINT('Ctrl Pts',(29.6100275770337,-5.91253309751285,-13.2086893874641));
#37410=CARTESIAN_POINT('Ctrl Pts',(30.1692894984411,-5.91881362945883,-13.2059721234291));
#37411=CARTESIAN_POINT('Ctrl Pts',(31.3098805820072,-5.91428725204099,-13.2079309635128));
#37412=CARTESIAN_POINT('Ctrl Pts',(32.3163182251691,-5.8978567744948,-13.215170536538));
#37413=CARTESIAN_POINT('Ctrl Pts',(33.168669589941,-5.89783797451689,-13.2151857432769));
#37414=CARTESIAN_POINT('Ctrl Pts',(33.4952713010556,-5.89783593918776,-13.2151875891279));
#37415=CARTESIAN_POINT('Ctrl Pts',(34.1548283685117,-5.89783217350437,-13.2151907586341));
#37416=CARTESIAN_POINT('Ctrl Pts',(34.9764778638341,-5.89782019909881,-13.2152010495211));
#37417=CARTESIAN_POINT('Ctrl Pts',(35.964110112416,-5.89781516246841,-13.2152053506642));
#37418=CARTESIAN_POINT('Ctrl Pts',(37.9386244259606,-5.89780833274504,-13.2152112104218));
#37419=CARTESIAN_POINT('Ctrl Pts',(39.5833333333333,-5.89777260594516,-13.2152418049849));
#37420=CARTESIAN_POINT('Ctrl Pts',(40.9,-5.89777260594516,-13.2152418049849));
#37421=CARTESIAN_POINT('Ctrl Pts',(6.84649785567288,6.71741536412572,-21.3772113060719));
#37422=CARTESIAN_POINT('Ctrl Pts',(7.61279643984166,5.5922435141165,-21.7222003209083));
#37423=CARTESIAN_POINT('Ctrl Pts',(8.41290239278216,4.4778139915129,-21.9819683115275));
#37424=CARTESIAN_POINT('Ctrl Pts',(10.1883118359637,2.12504829883047,-22.3516942143149));
#37425=CARTESIAN_POINT('Ctrl Pts',(11.1645908932198,0.860235293933488,-22.4195115822635));
#37426=CARTESIAN_POINT('Ctrl Pts',(13.104616539894,-1.36442582505286,-22.4060524143024));
#37427=CARTESIAN_POINT('Ctrl Pts',(14.0814329274866,-2.43568052201622,-22.2982732069865));
#37428=CARTESIAN_POINT('Ctrl Pts',(15.9946796213894,-4.24582169215594,-22.0394507048972));
#37429=CARTESIAN_POINT('Ctrl Pts',(16.9653275559585,-5.10151618176832,-21.84127820419));
#37430=CARTESIAN_POINT('Ctrl Pts',(18.8448710605556,-6.49486940232066,-21.4842569534398));
#37431=CARTESIAN_POINT('Ctrl Pts',(19.8101236302159,-7.14150804350575,-21.2634255374821));
#37432=CARTESIAN_POINT('Ctrl Pts',(20.9856903475787,-7.78021164720299,-21.0426589820635));
#37433=CARTESIAN_POINT('Ctrl Pts',(21.4500377829479,-8.02347291078476,-20.9532273635235));
#37434=CARTESIAN_POINT('Ctrl Pts',(22.3710393802637,-8.46623345546778,-20.7788884454095));
#37435=CARTESIAN_POINT('Ctrl Pts',(23.071969318899,-8.75491470148117,-20.6575298272076));
#37436=CARTESIAN_POINT('Ctrl Pts',(23.5926347936585,-8.94023465873168,-20.581371981806));
#37437=CARTESIAN_POINT('Ctrl Pts',(23.7065892332643,-8.98001571960566,-20.5647099449238));
#37438=CARTESIAN_POINT('Ctrl Pts',(23.9323706520526,-9.05664995495945,-20.5321468576874));
#37439=CARTESIAN_POINT('Ctrl Pts',(24.3307466212142,-9.18574049076626,-20.475948578475));
#37440=CARTESIAN_POINT('Ctrl Pts',(24.9023508233184,-9.35309964749796,-20.4001844372315));
#37441=CARTESIAN_POINT('Ctrl Pts',(25.475797257311,-9.49555868076774,-20.333847241253));
#37442=CARTESIAN_POINT('Ctrl Pts',(25.9330914993693,-9.59288697707766,-20.2886464898199));
#37443=CARTESIAN_POINT('Ctrl Pts',(26.160978182331,-9.63581705245673,-20.2689918009897));
#37444=CARTESIAN_POINT('Ctrl Pts',(26.7099322414348,-9.73235004955931,-20.2254900271806));
#37445=CARTESIAN_POINT('Ctrl Pts',(27.5959509089717,-9.8291584788779,-20.1795241403996));
#37446=CARTESIAN_POINT('Ctrl Pts',(28.5797495606368,-9.8753206064194,-20.1552722532429));
#37447=CARTESIAN_POINT('Ctrl Pts',(29.1657855350675,-9.9044166994659,-20.1412111689924));
#37448=CARTESIAN_POINT('Ctrl Pts',(29.3146731630635,-9.91097811975316,-20.1381027603738));
#37449=CARTESIAN_POINT('Ctrl Pts',(29.6257300067641,-9.92113271524799,-20.1332492263267));
#37450=CARTESIAN_POINT('Ctrl Pts',(30.1719452394075,-9.93050366138692,-20.1287785103478));
#37451=CARTESIAN_POINT('Ctrl Pts',(31.2977811219681,-9.92376874726296,-20.131991612471));
#37452=CARTESIAN_POINT('Ctrl Pts',(32.3069259117669,-9.89857089566955,-20.1442225454145));
#37453=CARTESIAN_POINT('Ctrl Pts',(33.1709940314751,-9.89851679451548,-20.1442592438602));
#37454=CARTESIAN_POINT('Ctrl Pts',(33.4961680489759,-9.89851046735383,-20.144263738865));
#37455=CARTESIAN_POINT('Ctrl Pts',(34.1564024558334,-9.89849933968829,-20.1442714128623));
#37456=CARTESIAN_POINT('Ctrl Pts',(34.9773378017946,-9.89846345509216,-20.1442963704307));
#37457=CARTESIAN_POINT('Ctrl Pts',(35.965039526566,-9.89844842592579,-20.1443067963912));
#37458=CARTESIAN_POINT('Ctrl Pts',(37.9392783163647,-9.89842798176077,-20.1443210056783));
#37459=CARTESIAN_POINT('Ctrl Pts',(39.5833333333333,-9.89832117405886,-20.1443951831047));
#37460=CARTESIAN_POINT('Ctrl Pts',(40.9,-9.89832117405886,-20.1443951831047));
#37461=CARTESIAN_POINT('Ctrl Pts',(6.90857970435318,8.71018585725739,-29.1272609852091));
#37462=CARTESIAN_POINT('Ctrl Pts',(7.67983757144493,7.16260494418019,-29.5775536996439));
#37463=CARTESIAN_POINT('Ctrl Pts',(8.48457055999567,5.63283520142948,-29.9097225030882));
#37464=CARTESIAN_POINT('Ctrl Pts',(10.2689932185249,2.41146069737717,-30.3644487697131));
#37465=CARTESIAN_POINT('Ctrl Pts',(11.2491988139072,0.683672158318399,-30.4296414097155));
#37466=CARTESIAN_POINT('Ctrl Pts',(13.2074449203971,-2.36894751212039,-30.3576235761244));
#37467=CARTESIAN_POINT('Ctrl Pts',(14.1878085217557,-3.82665309566743,-30.1849659988379));
#37468=CARTESIAN_POINT('Ctrl Pts',(16.1228140255811,-6.30658851121944,-29.7814752498472));
#37469=CARTESIAN_POINT('Ctrl Pts',(17.0983171044691,-7.46839135174,-29.4886591763938));
#37470=CARTESIAN_POINT('Ctrl Pts',(18.9977376700381,-9.36704911481259,-28.960082872958));
#37471=CARTESIAN_POINT('Ctrl Pts',(19.9674462816336,-10.2409515663328,-28.6415548808293));
#37472=CARTESIAN_POINT('Ctrl Pts',(21.1471060032309,-11.1004135437215,-28.3239820751164));
#37473=CARTESIAN_POINT('Ctrl Pts',(21.6116736136673,-11.4272945418467,-28.1962714220823));
#37474=CARTESIAN_POINT('Ctrl Pts',(22.5321107331753,-12.020283834991,-27.9485409607958));
#37475=CARTESIAN_POINT('Ctrl Pts',(23.2282372947767,-12.4035528917693,-27.7781185470826));
#37476=CARTESIAN_POINT('Ctrl Pts',(23.7411423015334,-12.6473785079705,-27.6723004799182));
#37477=CARTESIAN_POINT('Ctrl Pts',(23.8541050059081,-12.7001926206311,-27.6489722597555));
#37478=CARTESIAN_POINT('Ctrl Pts',(24.0772792343327,-12.801532363273,-27.6035767537809));
#37479=CARTESIAN_POINT('Ctrl Pts',(24.4706231308704,-12.9720321690744,-27.5254067801745));
#37480=CARTESIAN_POINT('Ctrl Pts',(25.0326506601032,-13.1919318242547,-27.4207276483817));
#37481=CARTESIAN_POINT('Ctrl Pts',(25.592916616209,-13.3777331675808,-27.3299203180182));
#37482=CARTESIAN_POINT('Ctrl Pts',(26.0369869863338,-13.5038445845533,-27.2685418387999));
#37483=CARTESIAN_POINT('Ctrl Pts',(26.2572892845279,-13.5592118403735,-27.2420133361896));
#37484=CARTESIAN_POINT('Ctrl Pts',(26.7861809172633,-13.6833062419415,-27.1835476308026));
#37485=CARTESIAN_POINT('Ctrl Pts',(27.6340630276977,-13.8074117592231,-27.1220525704356));
#37486=CARTESIAN_POINT('Ctrl Pts',(28.6084466264573,-13.8693290201702,-27.0881176443601));
#37487=CARTESIAN_POINT('Ctrl Pts',(29.1951297895238,-13.9084309041029,-27.0683644245335));
#37488=CARTESIAN_POINT('Ctrl Pts',(29.3379067795073,-13.9168171018366,-27.0642236253565));
#37489=CARTESIAN_POINT('Ctrl Pts',(29.6412852452591,-13.9300946799831,-27.05759935462));
#37490=CARTESIAN_POINT('Ctrl Pts',(30.1744790744101,-13.9423073235084,-27.0515191755616));
#37491=CARTESIAN_POINT('Ctrl Pts',(31.2855677213348,-13.9335693345849,-27.0558675796334));
#37492=CARTESIAN_POINT('Ctrl Pts',(32.297459923672,-13.8994232817536,-27.0731946134561));
#37493=CARTESIAN_POINT('Ctrl Pts',(33.173257907635,-13.89930470752,-27.0732696672435));
#37494=CARTESIAN_POINT('Ctrl Pts',(33.4970065888604,-13.899290450687,-27.0732789151666));
#37495=CARTESIAN_POINT('Ctrl Pts',(34.1579215418454,-13.8992658208366,-27.0732946436724));
#37496=CARTESIAN_POINT('Ctrl Pts',(34.9781539333148,-13.8991859907804,-27.0733458523265));
#37497=CARTESIAN_POINT('Ctrl Pts',(35.9659297143335,-13.8991526077107,-27.0733672375488));
#37498=CARTESIAN_POINT('Ctrl Pts',(37.9398993196361,-13.8991071452309,-27.0733963900546));
#37499=CARTESIAN_POINT('Ctrl Pts',(39.5833333333333,-13.8988697421725,-27.0735485612246));
#37500=CARTESIAN_POINT('Ctrl Pts',(40.9,-13.8988697421725,-27.0735485612246));
#37501=CARTESIAN_POINT('Ctrl Pts',(6.93528330520032,9.86563481868489,-33.5512413216408));
#37502=CARTESIAN_POINT('Ctrl Pts',(7.70864561497005,8.07765806999139,-34.0623374960229));
#37503=CARTESIAN_POINT('Ctrl Pts',(8.51541871352369,6.31093086144101,-34.4367698578614));
#37504=CARTESIAN_POINT('Ctrl Pts',(10.3035747340621,2.59403255178488,-34.941954951338));
#37505=CARTESIAN_POINT('Ctrl Pts',(11.2855474597114,0.601863607331421,-35.0067705115655));
#37506=CARTESIAN_POINT('Ctrl Pts',(13.2510271399958,-2.92382891559037,-34.9032893217431));
#37507=CARTESIAN_POINT('Ctrl Pts',(14.2329608248363,-4.60257161238984,-34.6945593989858));
#37508=CARTESIAN_POINT('Ctrl Pts',(16.1768697182174,-7.46747574760142,-34.2095752766376));
#37509=CARTESIAN_POINT('Ctrl Pts',(17.1545233971705,-8.80499374792142,-33.863251175018));
#37510=CARTESIAN_POINT('Ctrl Pts',(19.0635787323924,-10.9976618314205,-33.2359528227276));
#37511=CARTESIAN_POINT('Ctrl Pts',(20.0357940514506,-12.0029926013879,-32.8613840028834));
#37512=CARTESIAN_POINT('Ctrl Pts',(21.220027374451,-12.9932317593815,-32.4867165469275));
#37513=CARTESIAN_POINT('Ctrl Pts',(21.6852779128343,-13.3687144259958,-32.3368305207216));
#37514=CARTESIAN_POINT('Ctrl Pts',(22.6074094382986,-14.0501505350056,-32.046046858365));
#37515=CARTESIAN_POINT('Ctrl Pts',(23.3034045560159,-14.48918193341,-31.8467199720654));
#37516=CARTESIAN_POINT('Ctrl Pts',(23.8143672767889,-14.7674149360665,-31.7234333079364));
#37517=CARTESIAN_POINT('Ctrl Pts',(23.9270724954073,-14.8277950271987,-31.6962311639844));
#37518=CARTESIAN_POINT('Ctrl Pts',(24.1495225469483,-14.9435144746796,-31.6433583861174));
#37519=CARTESIAN_POINT('Ctrl Pts',(24.5413305977735,-15.1380475804187,-31.5524212197085));
#37520=CARTESIAN_POINT('Ctrl Pts',(25.0999889357198,-15.3882930140602,-31.4310156375915));
#37521=CARTESIAN_POINT('Ctrl Pts',(25.6548568854791,-15.5988027583031,-31.3262265443362));
#37522=CARTESIAN_POINT('Ctrl Pts',(26.0929602492092,-15.7410876933159,-31.2557376661539));
#37523=CARTESIAN_POINT('Ctrl Pts',(26.3096479269531,-15.8033473177939,-31.2253935968529));
#37524=CARTESIAN_POINT('Ctrl Pts',(26.828712163834,-15.9425694431083,-31.1587088311852));
#37525=CARTESIAN_POINT('Ctrl Pts',(27.6557884297531,-16.0810926132799,-31.0890012981155));
#37526=CARTESIAN_POINT('Ctrl Pts',(28.6247091266679,-16.1519656805033,-31.0495586097515));
#37527=CARTESIAN_POINT('Ctrl Pts',(29.2117706203407,-16.1967753671695,-31.0265558099779));
#37528=CARTESIAN_POINT('Ctrl Pts',(29.3510921954878,-16.206115111319,-31.0218764373728));
#37529=CARTESIAN_POINT('Ctrl Pts',(29.6501043905814,-16.2210980111664,-31.0142857961678));
#37530=CARTESIAN_POINT('Ctrl Pts',(30.1758702019789,-16.2348498398373,-31.0073340046884));
#37531=CARTESIAN_POINT('Ctrl Pts',(31.2785352103419,-16.2250286703998,-31.0122942956316));
#37532=CARTESIAN_POINT('Ctrl Pts',(32.2920164760144,-16.1856975481828,-31.0325718136051));
#37533=CARTESIAN_POINT('Ctrl Pts',(33.1745232741629,-16.1855272745483,-31.0326760798737));
#37534=CARTESIAN_POINT('Ctrl Pts',(33.4974585875214,-16.1855064782318,-31.0326890056741));
#37535=CARTESIAN_POINT('Ctrl Pts',(34.1587639155489,-16.1854709093048,-31.0327109045832));
#37536=CARTESIAN_POINT('Ctrl Pts',(34.9785998474406,-16.1853552918984,-31.0327822824582));
#37537=CARTESIAN_POINT('Ctrl Pts',(35.9664200829454,-16.1853069853609,-31.0328120805001));
#37538=CARTESIAN_POINT('Ctrl Pts',(37.9402388284555,-16.1852411572709,-31.032852711537));
#37539=CARTESIAN_POINT('Ctrl Pts',(39.5833333333333,-16.1848974953804,-31.033064777293));
#37540=CARTESIAN_POINT('Ctrl Pts',(40.9,-16.1848974953804,-31.033064777293));
#37541=CARTESIAN_POINT('Origin',(6.9,-25.9807621135332,-15.));
#37542=CARTESIAN_POINT('',(6.9,-6.90555748864273,-29.194404870986));
#37543=CARTESIAN_POINT('Ctrl Pts',(6.9,-1.92623027574191,-10.8594625780007));
#37544=CARTESIAN_POINT('Ctrl Pts',(6.9,-3.00887228147899,-14.5482083700348));
#37545=CARTESIAN_POINT('Ctrl Pts',(6.90000000166257,-4.07058553003038,-18.4565659967827));
#37546=CARTESIAN_POINT('Ctrl Pts',(6.90000000166257,-5.57797815223759,-24.1072623232988));
#37547=CARTESIAN_POINT('Ctrl Pts',(6.9,-6.24902093139925,-26.6663167664834));
#37548=CARTESIAN_POINT('Ctrl Pts',(6.9,-6.90555748864273,-29.194404870986));
#37549=CARTESIAN_POINT('Origin',(6.9,0.,0.));
#37550=CARTESIAN_POINT('Origin',(40.9,-7.79422863405995,-4.5));
#37551=CARTESIAN_POINT('Ctrl Pts',(40.9,-29.0996231131986,-18.5327260452907));
#37552=CARTESIAN_POINT('Ctrl Pts',(40.9,-28.6661818974695,-18.2824786427117));
#37553=CARTESIAN_POINT('Ctrl Pts',(40.9,-28.2327406817405,-18.0322312401326));
#37554=CARTESIAN_POINT('Ctrl Pts',(40.9,-27.7992994660114,-17.7819838375536));
#37555=CARTESIAN_POINT('Ctrl Pts',(30.5,-31.061268433756,-16.1306417505986));
#37556=CARTESIAN_POINT('Ctrl Pts',(30.5,-30.7013555966443,-16.823692245373));
#37557=CARTESIAN_POINT('Ctrl Pts',(30.5,-30.3108891324554,-17.5));
#37558=CARTESIAN_POINT('Ctrl Pts',(30.5,-12.8108891324554,-47.8108891324553));
#37559=CARTESIAN_POINT('Ctrl Pts',(30.5,17.5,-30.3108891324554));
#37560=CARTESIAN_POINT('Ctrl Pts',(30.5,47.8108891324553,-12.8108891324554));
#37561=CARTESIAN_POINT('Ctrl Pts',(30.5,30.3108891324554,17.5));
#37562=CARTESIAN_POINT('Ctrl Pts',(30.5,12.8108891324554,47.8108891324553));
#37563=CARTESIAN_POINT('Ctrl Pts',(30.5,-17.5,30.3108891324554));
#37564=CARTESIAN_POINT('Ctrl Pts',(30.5,-46.4877949884694,13.5747778926489));
#37565=CARTESIAN_POINT('Ctrl Pts',(30.5,-31.061268433756,-16.1306417505986));
#37566=CARTESIAN_POINT('Ctrl Pts',(30.3311478274255,-30.9943174850025,-16.0958729911865));
#37567=CARTESIAN_POINT('Ctrl Pts',(30.3311478274255,-30.6351804212937,-16.7874296516619));
#37568=CARTESIAN_POINT('Ctrl Pts',(30.3311478274255,-30.245555587262,-17.4622796600955));
#37569=CARTESIAN_POINT('Ctrl Pts',(30.3311478274255,-12.7832759271665,-47.7078352473574));
#37570=CARTESIAN_POINT('Ctrl Pts',(30.3311478274255,17.4622796600955,-30.245555587262));
#37571=CARTESIAN_POINT('Ctrl Pts',(30.3311478274255,47.7078352473574,-12.7832759271665));
#37572=CARTESIAN_POINT('Ctrl Pts',(30.3311478274255,30.245555587262,17.4622796600955));
#37573=CARTESIAN_POINT('Ctrl Pts',(30.3311478274255,12.7832759271665,47.7078352473574));
#37574=CARTESIAN_POINT('Ctrl Pts',(30.3311478274255,-17.4622796600955,30.245555587262));
#37575=CARTESIAN_POINT('Ctrl Pts',(30.3311478274255,-46.3875929639907,13.5455181648638));
#37576=CARTESIAN_POINT('Ctrl Pts',(30.3311478274255,-30.9943174850025,-16.0958729911865));
#37577=CARTESIAN_POINT('Ctrl Pts',(29.9897712690917,-30.8587004444282,-16.0254447695752));
#37578=CARTESIAN_POINT('Ctrl Pts',(29.9897712690917,-30.501134801215,-16.7139754925467));
#37579=CARTESIAN_POINT('Ctrl Pts',(29.9897712690917,-30.1132147882992,-17.3858726641896));
#37580=CARTESIAN_POINT('Ctrl Pts',(29.9897712690917,-12.7273421241097,-47.4990874524888));
#37581=CARTESIAN_POINT('Ctrl Pts',(29.9897712690917,17.3858726641896,-30.1132147882992));
#37582=CARTESIAN_POINT('Ctrl Pts',(29.9897712690917,47.4990874524888,-12.7273421241097));
#37583=CARTESIAN_POINT('Ctrl Pts',(29.9897712690917,30.1132147882992,17.3858726641896));
#37584=CARTESIAN_POINT('Ctrl Pts',(29.9897712690917,12.7273421241097,47.4990874524888));
#37585=CARTESIAN_POINT('Ctrl Pts',(29.9897712690917,-17.3858726641896,30.1132147882992));
#37586=CARTESIAN_POINT('Ctrl Pts',(29.9897712690917,-46.1846219490559,13.4862491363571));
#37587=CARTESIAN_POINT('Ctrl Pts',(29.9897712690917,-30.8587004444282,-16.0254447695752));
#37588=CARTESIAN_POINT('Ctrl Pts',(29.4666899049319,-30.6501289206644,-15.9171300516369));
#37589=CARTESIAN_POINT('Ctrl Pts',(29.4666899049319,-30.2949800354474,-16.6010070497276));
#37590=CARTESIAN_POINT('Ctrl Pts',(29.4666899049319,-29.9096819433198,-17.2683629213518));
#37591=CARTESIAN_POINT('Ctrl Pts',(29.4666899049319,-12.6413190219681,-47.1780448646716));
#37592=CARTESIAN_POINT('Ctrl Pts',(29.4666899049319,17.2683629213518,-29.9096819433198));
#37593=CARTESIAN_POINT('Ctrl Pts',(29.4666899049319,47.1780448646716,-12.6413190219681));
#37594=CARTESIAN_POINT('Ctrl Pts',(29.4666899049319,29.9096819433198,17.2683629213518));
#37595=CARTESIAN_POINT('Ctrl Pts',(29.4666899049319,12.6413190219681,47.1780448646716));
#37596=CARTESIAN_POINT('Ctrl Pts',(29.4666899049319,-17.2683629213518,29.9096819433198));
#37597=CARTESIAN_POINT('Ctrl Pts',(29.4666899049319,-45.8724637299593,13.3950966415431));
#37598=CARTESIAN_POINT('Ctrl Pts',(29.4666899049319,-30.6501289206644,-15.9171300516369));
#37599=CARTESIAN_POINT('Ctrl Pts',(28.7471241621752,-30.3617042288049,-15.7673462336858));
#37600=CARTESIAN_POINT('Ctrl Pts',(28.7471241621752,-30.0098973754615,-16.4447877935127));
#37601=CARTESIAN_POINT('Ctrl Pts',(28.7471241621752,-29.6282250261092,-17.105863694435));
#37602=CARTESIAN_POINT('Ctrl Pts',(28.7471241621752,-12.5223613316743,-46.7340887205442));
#37603=CARTESIAN_POINT('Ctrl Pts',(28.7471241621752,17.105863694435,-29.6282250261092));
#37604=CARTESIAN_POINT('Ctrl Pts',(28.7471241621752,46.7340887205442,-12.5223613316743));
#37605=CARTESIAN_POINT('Ctrl Pts',(28.7471241621752,29.6282250261092,17.105863694435));
#37606=CARTESIAN_POINT('Ctrl Pts',(28.7471241621752,12.5223613316743,46.7340887205442));
#37607=CARTESIAN_POINT('Ctrl Pts',(28.7471241621752,-17.105863694435,29.6282250261092));
#37608=CARTESIAN_POINT('Ctrl Pts',(28.7471241621752,-45.4407934015768,13.2690457322218));
#37609=CARTESIAN_POINT('Ctrl Pts',(28.7471241621752,-30.3617042288049,-15.7673462336858));
#37610=CARTESIAN_POINT('Ctrl Pts',(27.8100958442934,-29.9846639164451,-15.5715428260696));
#37611=CARTESIAN_POINT('Ctrl Pts',(27.8100958442934,-29.6372259010587,-16.2405717231752));
#37612=CARTESIAN_POINT('Ctrl Pts',(27.8100958442934,-29.2602932679205,-16.8934381948013));
#37613=CARTESIAN_POINT('Ctrl Pts',(27.8100958442934,-12.3668550731192,-46.1537314627218));
#37614=CARTESIAN_POINT('Ctrl Pts',(27.8100958442934,16.8934381948013,-29.2602932679205));
#37615=CARTESIAN_POINT('Ctrl Pts',(27.8100958442934,46.1537314627218,-12.3668550731192));
#37616=CARTESIAN_POINT('Ctrl Pts',(27.8100958442934,29.2602932679205,16.8934381948013));
#37617=CARTESIAN_POINT('Ctrl Pts',(27.8100958442934,12.3668550731192,46.1537314627218));
#37618=CARTESIAN_POINT('Ctrl Pts',(27.8100958442934,-16.8934381948013,29.2602932679205));
#37619=CARTESIAN_POINT('Ctrl Pts',(27.8100958442934,-44.8764966543029,13.1042669335782));
#37620=CARTESIAN_POINT('Ctrl Pts',(27.8100958442934,-29.9846639164451,-15.5715428260696));
#37621=CARTESIAN_POINT('Ctrl Pts',(26.8343111708818,-29.5937642144445,-15.3685420031368));
#37622=CARTESIAN_POINT('Ctrl Pts',(26.8343111708818,-29.2508556284042,-16.0288490017));
#37623=CARTESIAN_POINT('Ctrl Pts',(26.8343111708818,-28.8788369357517,-16.6732042787395));
#37624=CARTESIAN_POINT('Ctrl Pts',(26.8343111708818,-12.2056326570122,-45.5520412144912));
#37625=CARTESIAN_POINT('Ctrl Pts',(26.8343111708818,16.6732042787395,-28.8788369357517));
#37626=CARTESIAN_POINT('Ctrl Pts',(26.8343111708818,45.5520412144912,-12.2056326570122));
#37627=CARTESIAN_POINT('Ctrl Pts',(26.8343111708818,28.8788369357517,16.6732042787395));
#37628=CARTESIAN_POINT('Ctrl Pts',(26.8343111708818,12.2056326570122,45.5520412144912));
#37629=CARTESIAN_POINT('Ctrl Pts',(26.8343111708818,-16.6732042787395,28.8788369357517));
#37630=CARTESIAN_POINT('Ctrl Pts',(26.8343111708818,-44.2914572749094,12.9334311338658));
#37631=CARTESIAN_POINT('Ctrl Pts',(26.8343111708818,-29.5937642144445,-15.3685420031368));
#37632=CARTESIAN_POINT('Ctrl Pts',(25.8181479469611,-29.1945242233064,-15.1612099270726));
#37633=CARTESIAN_POINT('Ctrl Pts',(25.8181479469611,-28.8562417071321,-15.8126089354813));
#37634=CARTESIAN_POINT('Ctrl Pts',(25.8181479469611,-28.4892417994669,-16.4482714219305));
#37635=CARTESIAN_POINT('Ctrl Pts',(25.8181479469611,-12.0409703775363,-44.9375132213974));
#37636=CARTESIAN_POINT('Ctrl Pts',(25.8181479469611,16.4482714219305,-28.4892417994669));
#37637=CARTESIAN_POINT('Ctrl Pts',(25.8181479469611,44.9375132213974,-12.0409703775363));
#37638=CARTESIAN_POINT('Ctrl Pts',(25.8181479469611,28.4892417994669,16.4482714219305));
#37639=CARTESIAN_POINT('Ctrl Pts',(25.8181479469611,12.0409703775363,44.9375132213974));
#37640=CARTESIAN_POINT('Ctrl Pts',(25.8181479469611,-16.4482714219305,28.4892417994669));
#37641=CARTESIAN_POINT('Ctrl Pts',(25.8181479469611,-43.6939354158518,12.7589503583263));
#37642=CARTESIAN_POINT('Ctrl Pts',(25.8181479469611,-29.1945242233064,-15.1612099270726));
#37643=CARTESIAN_POINT('Ctrl Pts',(24.7595197917227,-28.796912394945,-14.9547233834603));
#37644=CARTESIAN_POINT('Ctrl Pts',(24.7595197917227,-28.4632370828042,-15.5972507298839));
#37645=CARTESIAN_POINT('Ctrl Pts',(24.7595197917227,-28.1012354927406,-16.2242558762949));
#37646=CARTESIAN_POINT('Ctrl Pts',(24.7595197917227,-11.8769796164458,-44.3254913690355));
#37647=CARTESIAN_POINT('Ctrl Pts',(24.7595197917227,16.2242558762949,-28.1012354927406));
#37648=CARTESIAN_POINT('Ctrl Pts',(24.7595197917227,44.3254913690355,-11.8769796164458));
#37649=CARTESIAN_POINT('Ctrl Pts',(24.7595197917227,28.1012354927406,16.2242558762949));
#37650=CARTESIAN_POINT('Ctrl Pts',(24.7595197917227,11.8769796164458,44.3254913690355));
#37651=CARTESIAN_POINT('Ctrl Pts',(24.7595197917227,-16.2242558762949,28.1012354927406));
#37652=CARTESIAN_POINT('Ctrl Pts',(24.7595197917227,-43.0988503438666,12.5851811425261));
#37653=CARTESIAN_POINT('Ctrl Pts',(24.7595197917227,-28.796912394945,-14.9547233834603));
#37654=CARTESIAN_POINT('Ctrl Pts',(23.6563574780851,-28.4140727469455,-14.7559082828157));
#37655=CARTESIAN_POINT('Ctrl Pts',(23.6563574780851,-28.084833470769,-15.389893569599));
#37656=CARTESIAN_POINT('Ctrl Pts',(23.6563574780851,-27.7276444994825,-16.0085630157705));
#37657=CARTESIAN_POINT('Ctrl Pts',(23.6563574780851,-11.7190814837121,-43.736207515253));
#37658=CARTESIAN_POINT('Ctrl Pts',(23.6563574780851,16.0085630157705,-27.7276444994825));
#37659=CARTESIAN_POINT('Ctrl Pts',(23.6563574780851,43.736207515253,-11.7190814837121));
#37660=CARTESIAN_POINT('Ctrl Pts',(23.6563574780851,27.7276444994825,16.0085630157705));
#37661=CARTESIAN_POINT('Ctrl Pts',(23.6563574780851,11.7190814837121,43.736207515253));
#37662=CARTESIAN_POINT('Ctrl Pts',(23.6563574780851,-16.0085630157705,27.7276444994825));
#37663=CARTESIAN_POINT('Ctrl Pts',(23.6563574780851,-42.5258740306932,12.4178678468319));
#37664=CARTESIAN_POINT('Ctrl Pts',(23.6563574780851,-28.4140727469455,-14.7559082828157));
#37665=CARTESIAN_POINT('Ctrl Pts',(22.5073180101405,-28.0598057001003,-14.5719314169357));
#37666=CARTESIAN_POINT('Ctrl Pts',(22.5073180101405,-27.7346713837132,-15.1980121665098));
#37667=CARTESIAN_POINT('Ctrl Pts',(22.5073180101405,-27.3819358493961,-15.8089680335819));
#37668=CARTESIAN_POINT('Ctrl Pts',(22.5073180101405,-11.5729678158142,-43.190903882978));
#37669=CARTESIAN_POINT('Ctrl Pts',(22.5073180101405,15.8089680335819,-27.3819358493961));
#37670=CARTESIAN_POINT('Ctrl Pts',(22.5073180101405,43.190903882978,-11.5729678158142));
#37671=CARTESIAN_POINT('Ctrl Pts',(22.5073180101405,27.3819358493961,15.8089680335819));
#37672=CARTESIAN_POINT('Ctrl Pts',(22.5073180101405,11.5729678158142,43.190903882978));
#37673=CARTESIAN_POINT('Ctrl Pts',(22.5073180101405,-15.8089680335819,27.3819358493961));
#37674=CARTESIAN_POINT('Ctrl Pts',(22.5073180101405,-41.9956608528241,12.2630417010206));
#37675=CARTESIAN_POINT('Ctrl Pts',(22.5073180101405,-28.0598057001003,-14.5719314169357));
#37676=CARTESIAN_POINT('Ctrl Pts',(21.3125219557939,-27.7463544749225,-14.4091508971893));
#37677=CARTESIAN_POINT('Ctrl Pts',(21.3125219557939,-27.4248521776202,-15.0282378072439));
#37678=CARTESIAN_POINT('Ctrl Pts',(21.3125219557939,-27.0760569908086,-15.632368792237));
#37679=CARTESIAN_POINT('Ctrl Pts',(21.3125219557939,-11.4436881985716,-42.7084257830456));
#37680=CARTESIAN_POINT('Ctrl Pts',(21.3125219557939,15.632368792237,-27.0760569908086));
#37681=CARTESIAN_POINT('Ctrl Pts',(21.3125219557939,42.7084257830456,-11.4436881985716));
#37682=CARTESIAN_POINT('Ctrl Pts',(21.3125219557939,27.0760569908086,15.632368792237));
#37683=CARTESIAN_POINT('Ctrl Pts',(21.3125219557939,11.4436881985716,42.7084257830456));
#37684=CARTESIAN_POINT('Ctrl Pts',(21.3125219557939,-15.632368792237,27.0760569908086));
#37685=CARTESIAN_POINT('Ctrl Pts',(21.3125219557939,-41.5265346055806,12.1260533880339));
#37686=CARTESIAN_POINT('Ctrl Pts',(21.3125219557939,-27.7463544749225,-14.4091508971893));
#37687=CARTESIAN_POINT('Ctrl Pts',(20.0742472323676,-27.4822408172221,-14.2719922102254));
#37688=CARTESIAN_POINT('Ctrl Pts',(20.0742472323676,-27.1637988552073,-14.8851861187906));
#37689=CARTESIAN_POINT('Ctrl Pts',(20.0742472323676,-26.8183238008716,-15.4835664656477));
#37690=CARTESIAN_POINT('Ctrl Pts',(20.0742472323676,-11.3347573352238,-42.3018902665193));
#37691=CARTESIAN_POINT('Ctrl Pts',(20.0742472323676,15.4835664656477,-26.8183238008716));
#37692=CARTESIAN_POINT('Ctrl Pts',(20.0742472323676,42.3018902665193,-11.3347573352238));
#37693=CARTESIAN_POINT('Ctrl Pts',(20.0742472323676,26.8183238008716,15.4835664656477));
#37694=CARTESIAN_POINT('Ctrl Pts',(20.0742472323676,11.3347573352238,42.3018902665193));
#37695=CARTESIAN_POINT('Ctrl Pts',(20.0742472323676,-15.4835664656477,26.8183238008716));
#37696=CARTESIAN_POINT('Ctrl Pts',(20.0742472323676,-41.1312493454498,12.0106271861277));
#37697=CARTESIAN_POINT('Ctrl Pts',(20.0742472323676,-27.4822408172221,-14.2719922102254));
#37698=CARTESIAN_POINT('Ctrl Pts',(18.7979917002302,-27.2694232481814,-14.1614724492006));
#37699=CARTESIAN_POINT('Ctrl Pts',(18.7979917002302,-26.9534472438987,-14.7699178935542));
#37700=CARTESIAN_POINT('Ctrl Pts',(18.7979917002302,-26.6106474867381,-15.3636644897785));
#37701=CARTESIAN_POINT('Ctrl Pts',(18.7979917002302,-11.2469829969596,-41.9743119765166));
#37702=CARTESIAN_POINT('Ctrl Pts',(18.7979917002302,15.3636644897785,-26.6106474867381));
#37703=CARTESIAN_POINT('Ctrl Pts',(18.7979917002302,41.9743119765166,-11.2469829969596));
#37704=CARTESIAN_POINT('Ctrl Pts',(18.7979917002302,26.6106474867381,15.3636644897785));
#37705=CARTESIAN_POINT('Ctrl Pts',(18.7979917002302,11.2469829969596,41.9743119765166));
#37706=CARTESIAN_POINT('Ctrl Pts',(18.7979917002302,-15.3636644897785,26.6106474867381));
#37707=CARTESIAN_POINT('Ctrl Pts',(18.7979917002302,-40.8127362898543,11.9176190323383));
#37708=CARTESIAN_POINT('Ctrl Pts',(18.7979917002302,-27.2694232481814,-14.1614724492006));
#37709=CARTESIAN_POINT('Ctrl Pts',(17.4917404060759,-27.1042817018803,-14.0757116526895));
#37710=CARTESIAN_POINT('Ctrl Pts',(17.4917404060759,-26.7902192241678,-14.6804723978617));
#37711=CARTESIAN_POINT('Ctrl Pts',(17.4917404060759,-26.4494954361781,-15.2706233100072));
#37712=CARTESIAN_POINT('Ctrl Pts',(17.4917404060759,-11.1788721261709,-41.7201187461852));
#37713=CARTESIAN_POINT('Ctrl Pts',(17.4917404060759,15.2706233100072,-26.4494954361781));
#37714=CARTESIAN_POINT('Ctrl Pts',(17.4917404060759,41.7201187461852,-11.1788721261709));
#37715=CARTESIAN_POINT('Ctrl Pts',(17.4917404060759,26.4494954361781,15.2706233100072));
#37716=CARTESIAN_POINT('Ctrl Pts',(17.4917404060759,11.1788721261709,41.7201187461852));
#37717=CARTESIAN_POINT('Ctrl Pts',(17.4917404060759,-15.2706233100072,26.4494954361781));
#37718=CARTESIAN_POINT('Ctrl Pts',(17.4917404060759,-40.5655774732432,11.8454468408945));
#37719=CARTESIAN_POINT('Ctrl Pts',(17.4917404060759,-27.1042817018803,-14.0757116526895));
#37720=CARTESIAN_POINT('Ctrl Pts',(16.1647270995715,-26.9797204766935,-14.011024902894));
#37721=CARTESIAN_POINT('Ctrl Pts',(16.1647270995715,-26.6671013136366,-14.6130063919992));
#37722=CARTESIAN_POINT('Ctrl Pts',(16.1647270995715,-26.3279433657953,-15.2004451894511));
#37723=CARTESIAN_POINT('Ctrl Pts',(16.1647270995715,-11.1274981763442,-41.5283885552464));
#37724=CARTESIAN_POINT('Ctrl Pts',(16.1647270995715,15.2004451894511,-26.3279433657953));
#37725=CARTESIAN_POINT('Ctrl Pts',(16.1647270995715,41.5283885552464,-11.1274981763442));
#37726=CARTESIAN_POINT('Ctrl Pts',(16.1647270995715,26.3279433657953,15.2004451894511));
#37727=CARTESIAN_POINT('Ctrl Pts',(16.1647270995715,11.1274981763442,41.5283885552464));
#37728=CARTESIAN_POINT('Ctrl Pts',(16.1647270995715,-15.2004451894511,26.3279433657953));
#37729=CARTESIAN_POINT('Ctrl Pts',(16.1647270995715,-40.3791531257526,11.7910095609247));
#37730=CARTESIAN_POINT('Ctrl Pts',(16.1647270995715,-26.9797204766935,-14.011024902894));
#37731=CARTESIAN_POINT('Ctrl Pts',(14.8263876417415,-26.8868282012067,-13.9627843740029));
#37732=CARTESIAN_POINT('Ctrl Pts',(14.8263876417415,-26.5752853986496,-14.5626932163446));
#37733=CARTESIAN_POINT('Ctrl Pts',(14.8263876417415,-26.2372951854241,-15.1481094381123));
#37734=CARTESIAN_POINT('Ctrl Pts',(14.8263876417415,-11.0891857473118,-41.3854046235364));
#37735=CARTESIAN_POINT('Ctrl Pts',(14.8263876417415,15.1481094381123,-26.2372951854241));
#37736=CARTESIAN_POINT('Ctrl Pts',(14.8263876417415,41.3854046235364,-11.0891857473118));
#37737=CARTESIAN_POINT('Ctrl Pts',(14.8263876417415,26.2372951854241,15.1481094381123));
#37738=CARTESIAN_POINT('Ctrl Pts',(14.8263876417415,11.0891857473118,41.3854046235364));
#37739=CARTESIAN_POINT('Ctrl Pts',(14.8263876417415,-15.1481094381123,26.2372951854241));
#37740=CARTESIAN_POINT('Ctrl Pts',(14.8263876417415,-40.2401260583921,11.750412635195));
#37741=CARTESIAN_POINT('Ctrl Pts',(14.8263876417415,-26.8868282012067,-13.9627843740029));
#37742=CARTESIAN_POINT('Ctrl Pts',(13.4853470903953,-26.8165326442879,-13.926278703034));
#37743=CARTESIAN_POINT('Ctrl Pts',(13.4853470903953,-26.505804369746,-14.5246190849439));
#37744=CARTESIAN_POINT('Ctrl Pts',(13.4853470903953,-26.1686978312363,-15.1085047372063));
#37745=CARTESIAN_POINT('Ctrl Pts',(13.4853470903953,-11.0601930940301,-41.2772025684426));
#37746=CARTESIAN_POINT('Ctrl Pts',(13.4853470903953,15.1085047372063,-26.1686978312363));
#37747=CARTESIAN_POINT('Ctrl Pts',(13.4853470903953,41.2772025684426,-11.0601930940301));
#37748=CARTESIAN_POINT('Ctrl Pts',(13.4853470903953,26.1686978312363,15.1085047372063));
#37749=CARTESIAN_POINT('Ctrl Pts',(13.4853470903953,11.0601930940301,41.2772025684426));
#37750=CARTESIAN_POINT('Ctrl Pts',(13.4853470903953,-15.1085047372063,26.1686978312363));
#37751=CARTESIAN_POINT('Ctrl Pts',(13.4853470903953,-40.1349183317465,11.7196912055776));
#37752=CARTESIAN_POINT('Ctrl Pts',(13.4853470903953,-26.8165326442879,-13.926278703034));
#37753=CARTESIAN_POINT('Ctrl Pts',(12.1482076787549,-26.7614591013549,-13.8976780812377));
#37754=CARTESIAN_POINT('Ctrl Pts',(12.1482076787549,-26.4513689744511,-14.4947896419145));
#37755=CARTESIAN_POINT('Ctrl Pts',(12.1482076787549,-26.1149547570431,-15.0774761588537));
#37756=CARTESIAN_POINT('Ctrl Pts',(12.1482076787549,-11.0374785981894,-41.1924309158968));
#37757=CARTESIAN_POINT('Ctrl Pts',(12.1482076787549,15.0774761588537,-26.1149547570431));
#37758=CARTESIAN_POINT('Ctrl Pts',(12.1482076787549,41.1924309158968,-11.0374785981894));
#37759=CARTESIAN_POINT('Ctrl Pts',(12.1482076787549,26.1149547570431,15.0774761588537));
#37760=CARTESIAN_POINT('Ctrl Pts',(12.1482076787549,11.0374785981894,41.1924309158968));
#37761=CARTESIAN_POINT('Ctrl Pts',(12.1482076787549,-15.0774761588537,26.1149547570431));
#37762=CARTESIAN_POINT('Ctrl Pts',(12.1482076787549,-40.0524926066472,11.6956222878942));
#37763=CARTESIAN_POINT('Ctrl Pts',(12.1482076787549,-26.7614591013549,-13.8976780812377));
#37764=CARTESIAN_POINT('Ctrl Pts',(10.8190675759626,-26.716817747915,-13.8744950717886));
#37765=CARTESIAN_POINT('Ctrl Pts',(10.8190675759626,-26.4072448888814,-14.4706105780977));
#37766=CARTESIAN_POINT('Ctrl Pts',(10.8190675759626,-26.0713918511132,-15.0523251033884));
#37767=CARTESIAN_POINT('Ctrl Pts',(10.8190675759626,-11.0190667477248,-41.1237169545017));
#37768=CARTESIAN_POINT('Ctrl Pts',(10.8190675759626,15.0523251033884,-26.0713918511132));
#37769=CARTESIAN_POINT('Ctrl Pts',(10.8190675759626,41.1237169545017,-11.0190667477248));
#37770=CARTESIAN_POINT('Ctrl Pts',(10.8190675759626,26.0713918511132,15.0523251033884));
#37771=CARTESIAN_POINT('Ctrl Pts',(10.8190675759626,11.0190667477248,41.1237169545017));
#37772=CARTESIAN_POINT('Ctrl Pts',(10.8190675759626,-15.0523251033884,26.0713918511132));
#37773=CARTESIAN_POINT('Ctrl Pts',(10.8190675759626,-39.9856802003493,11.6761125740824));
#37774=CARTESIAN_POINT('Ctrl Pts',(10.8190675759626,-26.716817747915,-13.8744950717886));
#37775=CARTESIAN_POINT('Ctrl Pts',(9.50027713254189,-26.6796403391198,-13.8551882149624));
#37776=CARTESIAN_POINT('Ctrl Pts',(9.50027713254189,-26.3704982618073,-14.4504742051937));
#37777=CARTESIAN_POINT('Ctrl Pts',(9.50027713254189,-26.0351125755702,-15.0313792538877));
#37778=CARTESIAN_POINT('Ctrl Pts',(9.50027713254189,-11.0037333216826,-41.0664918294579));
#37779=CARTESIAN_POINT('Ctrl Pts',(9.50027713254189,15.0313792538877,-26.0351125755702));
#37780=CARTESIAN_POINT('Ctrl Pts',(9.5002771325419,41.0664918294579,-11.0037333216826));
#37781=CARTESIAN_POINT('Ctrl Pts',(9.5002771325419,26.0351125755702,15.0313792538877));
#37782=CARTESIAN_POINT('Ctrl Pts',(9.5002771325419,11.0037333216826,41.0664918294579));
#37783=CARTESIAN_POINT('Ctrl Pts',(9.50027713254189,-15.0313792538877,26.0351125755702));
#37784=CARTESIAN_POINT('Ctrl Pts',(9.50027713254189,-39.9300386942093,11.6598648452397));
#37785=CARTESIAN_POINT('Ctrl Pts',(9.50027713254189,-26.6796403391198,-13.8551882149624));
#37786=CARTESIAN_POINT('Ctrl Pts',(8.45435372222587,-26.6546635289318,-13.8422173352292));
#37787=CARTESIAN_POINT('Ctrl Pts',(8.45435372222587,-26.3458108626791,-14.4369460336456));
#37788=CARTESIAN_POINT('Ctrl Pts',(8.45435372222587,-26.0107391561104,-15.0173072536015));
#37789=CARTESIAN_POINT('Ctrl Pts',(8.45435372222587,-10.9934319025089,-41.0280464097118));
#37790=CARTESIAN_POINT('Ctrl Pts',(8.45435372222587,15.0173072536015,-26.0107391561104));
#37791=CARTESIAN_POINT('Ctrl Pts',(8.45435372222587,41.0280464097118,-10.9934319025089));
#37792=CARTESIAN_POINT('Ctrl Pts',(8.45435372222587,26.0107391561104,15.0173072536015));
#37793=CARTESIAN_POINT('Ctrl Pts',(8.45435372222587,10.9934319025089,41.0280464097118));
#37794=CARTESIAN_POINT('Ctrl Pts',(8.45435372222587,-15.0173072536015,26.0107391561104));
#37795=CARTESIAN_POINT('Ctrl Pts',(8.45435372222587,-39.8926571933874,11.6489491721888));
#37796=CARTESIAN_POINT('Ctrl Pts',(8.45435372222587,-26.6546635289318,-13.8422173352292));
#37797=CARTESIAN_POINT('Ctrl Pts',(7.67514864245731,-26.6383620035993,-13.8337516775665));
#37798=CARTESIAN_POINT('Ctrl Pts',(7.67514864245731,-26.3296982262274,-14.4281166503283));
#37799=CARTESIAN_POINT('Ctrl Pts',(7.67514864245731,-25.9948314436454,-15.0081229315276));
#37800=CARTESIAN_POINT('Ctrl Pts',(7.67514864245731,-10.9867085121178,-41.0029543751729));
#37801=CARTESIAN_POINT('Ctrl Pts',(7.67514864245731,15.0081229315276,-25.9948314436454));
#37802=CARTESIAN_POINT('Ctrl Pts',(7.67514864245731,41.0029543751729,-10.9867085121178));
#37803=CARTESIAN_POINT('Ctrl Pts',(7.67514864245731,25.9948314436454,15.0081229315276));
#37804=CARTESIAN_POINT('Ctrl Pts',(7.67514864245731,10.9867085121178,41.0029543751729));
#37805=CARTESIAN_POINT('Ctrl Pts',(7.67514864245731,-15.0081229315276,25.9948314436454));
#37806=CARTESIAN_POINT('Ctrl Pts',(7.67514864245731,-39.8682595430058,11.6418248789176));
#37807=CARTESIAN_POINT('Ctrl Pts',(7.67514864245731,-26.6383620035993,-13.8337516775665));
#37808=CARTESIAN_POINT('Ctrl Pts',(7.15799654185577,-26.6285708447822,-13.8286669632852));
#37809=CARTESIAN_POINT('Ctrl Pts',(7.15799654185577,-26.3200205194336,-14.4228134720947));
#37810=CARTESIAN_POINT('Ctrl Pts',(7.15799654185577,-25.9852768200144,-15.0026065670023));
#37811=CARTESIAN_POINT('Ctrl Pts',(7.15799654185577,-10.9826702530122,-40.9878833870167));
#37812=CARTESIAN_POINT('Ctrl Pts',(7.15799654185577,15.0026065670023,-25.9852768200144));
#37813=CARTESIAN_POINT('Ctrl Pts',(7.15799654185577,40.9878833870167,-10.9826702530122));
#37814=CARTESIAN_POINT('Ctrl Pts',(7.15799654185577,25.9852768200144,15.0026065670023));
#37815=CARTESIAN_POINT('Ctrl Pts',(7.15799654185577,10.9826702530122,40.9878833870167));
#37816=CARTESIAN_POINT('Ctrl Pts',(7.15799654185577,-15.0026065670023,25.9852768200144));
#37817=CARTESIAN_POINT('Ctrl Pts',(7.15799654185577,-39.8536056216838,11.6375458261629));
#37818=CARTESIAN_POINT('Ctrl Pts',(7.15799654185577,-26.6285708447822,-13.8286669632852));
#37819=CARTESIAN_POINT('Ctrl Pts',(6.9,-26.6239443717909,-13.8262643576559));
#37820=CARTESIAN_POINT('Ctrl Pts',(6.9,-26.3154476542665,-14.4203076388911));
#37821=CARTESIAN_POINT('Ctrl Pts',(6.9,-25.9807621135332,-15.));
#37822=CARTESIAN_POINT('Ctrl Pts',(6.9,-10.9807621135332,-40.9807621135331));
#37823=CARTESIAN_POINT('Ctrl Pts',(6.9,15.,-25.9807621135332));
#37824=CARTESIAN_POINT('Ctrl Pts',(6.9,40.9807621135331,-10.9807621135332));
#37825=CARTESIAN_POINT('Ctrl Pts',(6.9,25.9807621135332,15.));
#37826=CARTESIAN_POINT('Ctrl Pts',(6.9,10.9807621135332,40.9807621135331));
#37827=CARTESIAN_POINT('Ctrl Pts',(6.9,-15.,25.9807621135332));
#37828=CARTESIAN_POINT('Ctrl Pts',(6.9,-39.846681418688,11.6355239079848));
#37829=CARTESIAN_POINT('Ctrl Pts',(6.9,-26.6239443717909,-13.8262643576559));
#37830=CARTESIAN_POINT('Ctrl Pts',(6.9,-6.90555748864273,-29.194404870986));
#37831=CARTESIAN_POINT('Ctrl Pts',(7.85773098116326,-8.83308608050287,-28.7583591297181));
#37832=CARTESIAN_POINT('Ctrl Pts',(8.88781981167334,-10.6725495024415,-28.148927360677));
#37833=CARTESIAN_POINT('Ctrl Pts',(10.5914578196776,-13.4378975079049,-26.9549567714738));
#37834=CARTESIAN_POINT('Ctrl Pts',(11.2365058953701,-14.4268759573926,-26.4627511078989));
#37835=CARTESIAN_POINT('Ctrl Pts',(12.0558885382926,-15.5639851987506,-25.8276163596339));
#37836=CARTESIAN_POINT('Ctrl Pts',(12.1875764958397,-15.7427052651201,-25.7255677072203));
#37837=CARTESIAN_POINT('Ctrl Pts',(13.194901830313,-17.0880993664927,-24.9407551262718));
#37838=CARTESIAN_POINT('Ctrl Pts',(14.2258982134098,-18.4224696507577,-24.0748117650462));
#37839=CARTESIAN_POINT('Ctrl Pts',(18.2616480823244,-22.4465505568645,-20.9914735836847));
#37840=CARTESIAN_POINT('Ctrl Pts',(21.0496416709525,-24.4970863377161,-19.1084188222497));
#37841=CARTESIAN_POINT('Ctrl Pts',(25.8000196361138,-27.440416330328,-18.0798601480504));
#37842=CARTESIAN_POINT('Ctrl Pts',(26.8976561124457,-27.9949084025612,-18.1725012311874));
#37843=CARTESIAN_POINT('Ctrl Pts',(28.0045908801237,-28.5110480063609,-18.293020318403));
#37844=CARTESIAN_POINT('Ctrl Pts',(28.5235971652406,-28.7375730360626,-18.3760345677215));
#37845=CARTESIAN_POINT('Ctrl Pts',(29.0834839543824,-28.9821227669885,-18.4629109750536));
#37846=CARTESIAN_POINT('Ctrl Pts',(29.1146288039499,-28.995750541561,-18.4676985487665));
#37847=CARTESIAN_POINT('Ctrl Pts',(29.5949306848436,-29.2050975774362,-18.5426905181125));
#37848=CARTESIAN_POINT('Ctrl Pts',(30.0492939924726,-29.3870260594868,-18.6372599535756));
#37849=CARTESIAN_POINT('Ctrl Pts',(30.5,-29.559989655385,-18.7405179110273));
#37850=CARTESIAN_POINT('Ctrl Pts',(6.45331003273164,-1.59669678622779,-10.9133179225515));
#37851=CARTESIAN_POINT('Ctrl Pts',(7.20830533428676,-2.1627262104287,-10.8283039351861));
#37852=CARTESIAN_POINT('Ctrl Pts',(7.99928962140321,-2.70879554626307,-10.7080816105349));
#37853=CARTESIAN_POINT('Ctrl Pts',(9.76164489174098,-3.82718122480732,-10.3736775708918));
#37854=CARTESIAN_POINT('Ctrl Pts',(10.7316587814816,-4.40082635509405,-10.1362456656108));
#37855=CARTESIAN_POINT('Ctrl Pts',(12.6606926111663,-5.38563263712134,-9.65961205419967));
#37856=CARTESIAN_POINT('Ctrl Pts',(13.6374431259542,-5.83915384029438,-9.38360450626091));
#37857=CARTESIAN_POINT('Ctrl Pts',(14.8679539417017,-6.32358226998235,-9.06165302613707));
#37858=CARTESIAN_POINT('Ctrl Pts',(15.8146186835336,-6.68453209751778,-8.8086769516328));
#37859=CARTESIAN_POINT('Ctrl Pts',(16.7768279789012,-7.0051694125711,-8.55011854625631));
#37860=CARTESIAN_POINT('Ctrl Pts',(18.442654946101,-7.48808598435167,-8.14533972931254));
#37861=CARTESIAN_POINT('Ctrl Pts',(19.4151948753428,-7.72973898022672,-7.90738588441825));
#37862=CARTESIAN_POINT('Ctrl Pts',(20.6328868119184,-7.97443640583061,-7.66437297695772));
#37863=CARTESIAN_POINT('Ctrl Pts',(21.1054260060187,-8.06465516157007,-7.57098863237664));
#37864=CARTESIAN_POINT('Ctrl Pts',(22.0544239964408,-8.22831938421071,-7.39387592479571));
#37865=CARTESIAN_POINT('Ctrl Pts',(22.7836594350113,-8.33397294082321,-7.27389266543022));
#37866=CARTESIAN_POINT('Ctrl Pts',(23.5025637456205,-8.42426711082603,-7.17270583388456));
#37867=CARTESIAN_POINT('Ctrl Pts',(23.9756232708729,-8.47952646912222,-7.10861034193438));
#37868=CARTESIAN_POINT('Ctrl Pts',(24.5702383273712,-8.53935462310088,-7.03666681503307));
#37869=CARTESIAN_POINT('Ctrl Pts',(25.0506812637281,-8.58189400875848,-6.98463603831063));
#37870=CARTESIAN_POINT('Ctrl Pts',(25.4117237717368,-8.61093616318064,-6.94891133994702));
#37871=CARTESIAN_POINT('Ctrl Pts',(25.7132331301511,-8.63276690479097,-6.92207219011215));
#37872=CARTESIAN_POINT('Ctrl Pts',(25.924350018954,-8.64675417662544,-6.90499555217217));
#37873=CARTESIAN_POINT('Ctrl Pts',(26.0449825351307,-8.65437719289233,-6.8957416597319));
#37874=CARTESIAN_POINT('Ctrl Pts',(26.1053107047433,-8.6580646096281,-6.89128602190967));
#37875=CARTESIAN_POINT('Ctrl Pts',(26.598286881356,-8.68771831234641,-6.85557010312598));
#37876=CARTESIAN_POINT('Ctrl Pts',(27.5414448539117,-8.72222386822184,-6.81230249083088));
#37877=CARTESIAN_POINT('Ctrl Pts',(28.5384718269747,-8.7374287400485,-6.79157348079207));
#37878=CARTESIAN_POINT('Ctrl Pts',(29.1235718011012,-8.74727658763324,-6.77903979219493));
#37879=CARTESIAN_POINT('Ctrl Pts',(29.281292582401,-8.74962231400058,-6.77610142826291));
#37880=CARTESIAN_POINT('Ctrl Pts',(29.6033746665999,-8.75316560056407,-6.77163194910168));
#37881=CARTESIAN_POINT('Ctrl Pts',(30.1682156581428,-8.7564468026045,-6.76749797708626));
#37882=CARTESIAN_POINT('Ctrl Pts',(31.3151120085301,-8.75407681716344,-6.77048174742394));
#37883=CARTESIAN_POINT('Ctrl Pts',(32.320349075554,-8.74562733267079,-6.78127046660757));
#37884=CARTESIAN_POINT('Ctrl Pts',(33.1676615322708,-8.74562186943988,-6.7812835744978));
#37885=CARTESIAN_POINT('Ctrl Pts',(33.4948723279895,-8.7456213359517,-6.78128505761795));
#37886=CARTESIAN_POINT('Ctrl Pts',(34.1541357431676,-8.74562028433968,-6.78128770533521));
#37887=CARTESIAN_POINT('Ctrl Pts',(34.9760826079903,-8.74561702798979,-6.7812961259584));
#37888=CARTESIAN_POINT('Ctrl Pts',(35.9636845487692,-8.7456156797743,-6.78129958330352));
#37889=CARTESIAN_POINT('Ctrl Pts',(37.9383132355672,-8.745613828852,-6.7813043592495));
#37890=CARTESIAN_POINT('Ctrl Pts',(39.5833333333333,-8.74560464293355,-6.7813280023926));
#37891=CARTESIAN_POINT('Ctrl Pts',(40.9,-8.74560464293355,-6.7813280023926));
#37892=CARTESIAN_POINT('Ctrl Pts',(6.63336813585096,-2.58998912169034,-14.1980521881427));
#37893=CARTESIAN_POINT('Ctrl Pts',(7.389696336477,-3.32655463912722,-14.0595388287459));
#37894=CARTESIAN_POINT('Ctrl Pts',(8.18035160561764,-4.03465273479121,-13.8764440634215));
#37895=CARTESIAN_POINT('Ctrl Pts',(9.9416314386187,-5.47986851886094,-13.3869575789582));
#37896=CARTESIAN_POINT('Ctrl Pts',(10.9109664605569,-6.21859686207519,-13.0495988183286));
#37897=CARTESIAN_POINT('Ctrl Pts',(12.8334013836927,-7.47915893423736,-12.3824387994051));
#37898=CARTESIAN_POINT('Ctrl Pts',(13.8089179831182,-8.05904353786122,-12.0008911509523));
#37899=CARTESIAN_POINT('Ctrl Pts',(15.0306778911273,-8.67329495695321,-11.5604290689694));
#37900=CARTESIAN_POINT('Ctrl Pts',(15.9745670647922,-9.13243737556314,-11.2141745075895));
#37901=CARTESIAN_POINT('Ctrl Pts',(16.9295440841729,-9.53704617981305,-10.8635736365946));
#37902=CARTESIAN_POINT('Ctrl Pts',(18.5792362231986,-10.1451076803253,-10.3171018918725));
#37903=CARTESIAN_POINT('Ctrl Pts',(19.5469773926757,-10.4493242965117,-9.99640408637918));
#37904=CARTESIAN_POINT('Ctrl Pts',(20.7474295734276,-10.754900018616,-9.67172058444863));
#37905=CARTESIAN_POINT('Ctrl Pts',(21.2167794172894,-10.8681544802446,-9.54637190554476));
#37906=CARTESIAN_POINT('Ctrl Pts',(22.1549843938464,-11.0724642143303,-9.30976886072817));
#37907=CARTESIAN_POINT('Ctrl Pts',(22.8744776078266,-11.2039970972494,-9.14996578827687));
#37908=CARTESIAN_POINT('Ctrl Pts',(23.5816077902762,-11.3162019466949,-9.01558422395417));
#37909=CARTESIAN_POINT('Ctrl Pts',(24.0500749276264,-11.3851612528794,-8.9300835935143));
#37910=CARTESIAN_POINT('Ctrl Pts',(24.6365533946126,-11.4594652258083,-8.83449183240024));
#37911=CARTESIAN_POINT('Ctrl Pts',(25.1102835291688,-11.512269915973,-8.76539275960627));
#37912=CARTESIAN_POINT('Ctrl Pts',(25.4658322439329,-11.5482688417073,-8.71801358900138));
#37913=CARTESIAN_POINT('Ctrl Pts',(25.7624874136685,-11.5753180370233,-8.68244638509938));
#37914=CARTESIAN_POINT('Ctrl Pts',(25.9700349923411,-11.5926401638759,-8.65983585467432));
#37915=CARTESIAN_POINT('Ctrl Pts',(26.0885791323129,-11.6020803597253,-8.64758737376053));
#37916=CARTESIAN_POINT('Ctrl Pts',(26.1478525996404,-11.6066467500381,-8.64169115913858));
#37917=CARTESIAN_POINT('Ctrl Pts',(26.6319130667262,-11.6433645250355,-8.59444428954215));
#37918=CARTESIAN_POINT('Ctrl Pts',(27.5577774489367,-11.6860824768893,-8.53717709311581));
#37919=CARTESIAN_POINT('Ctrl Pts',(28.5508423746857,-11.7050908260002,-8.50942828058724));
#37920=CARTESIAN_POINT('Ctrl Pts',(29.1362159539423,-11.7174369518246,-8.49263545125893));
#37921=CARTESIAN_POINT('Ctrl Pts',(29.2912819508841,-11.7203386713976,-8.48875007883417));
#37922=CARTESIAN_POINT('Ctrl Pts',(29.610052998187,-11.7247475094471,-8.4828058172773));
#37923=CARTESIAN_POINT('Ctrl Pts',(30.1693026775047,-11.728827902791,-8.47731190452095));
#37924=CARTESIAN_POINT('Ctrl Pts',(31.3098786008463,-11.7258872894481,-8.48127083805332));
#37925=CARTESIAN_POINT('Ctrl Pts',(32.3162827048883,-11.7152777874898,-8.49575357359988));
#37926=CARTESIAN_POINT('Ctrl Pts',(33.1686195735696,-11.715269078277,-8.49577523975602));
#37927=CARTESIAN_POINT('Ctrl Pts',(33.4952188807558,-11.7152682401723,-8.49577770055113));
#37928=CARTESIAN_POINT('Ctrl Pts',(34.1547734244042,-11.7152665713231,-8.49578208271196));
#37929=CARTESIAN_POINT('Ctrl Pts',(34.9764178792931,-11.7152614171757,-8.49579602915745));
#37930=CARTESIAN_POINT('Ctrl Pts',(35.9640520550922,-11.7152592814565,-8.49580175406155));
#37931=CARTESIAN_POINT('Ctrl Pts',(37.9385651163988,-11.7152563511877,-8.49580966365999));
#37932=CARTESIAN_POINT('Ctrl Pts',(39.5833333333333,-11.7152418049849,-8.49584881729847));
#37933=CARTESIAN_POINT('Ctrl Pts',(40.9,-11.7152418049849,-8.49584881729847));
#37934=CARTESIAN_POINT('Ctrl Pts',(6.84648239176542,-4.87117200494631,-21.8719108775553));
#37935=CARTESIAN_POINT('Ctrl Pts',(7.61278097593421,-6.01809391809558,-21.6080942034255));
#37936=CARTESIAN_POINT('Ctrl Pts',(8.41274152921386,-7.11297694015339,-21.2759544371052));
#37937=CARTESIAN_POINT('Ctrl Pts',(10.1879716557546,-9.3352659896486,-20.4198986989574));
#37938=CARTESIAN_POINT('Ctrl Pts',(11.1642573475929,-10.4645258845954,-19.8462357742843));
#37939=CARTESIAN_POINT('Ctrl Pts',(13.1034321172788,-12.3837514736036,-18.7228640453274));
#37940=CARTESIAN_POINT('Ctrl Pts',(14.0822646095709,-13.259092905625,-18.0925354910949));
#37941=CARTESIAN_POINT('Ctrl Pts',(15.3084001581866,-14.1807147676625,-17.369341405527));
#37942=CARTESIAN_POINT('Ctrl Pts',(16.2531227144981,-14.8695159890908,-16.8032299545452));
#37943=CARTESIAN_POINT('Ctrl Pts',(17.2084375604977,-15.4708786153412,-16.2348330754283));
#37944=CARTESIAN_POINT('Ctrl Pts',(18.8473961588578,-16.3684102669437,-15.3570672461537));
#37945=CARTESIAN_POINT('Ctrl Pts',(19.8110405035781,-16.8164458459158,-14.8437940564497));
#37946=CARTESIAN_POINT('Ctrl Pts',(20.987265500616,-17.2594998647323,-14.3329359049566));
#37947=CARTESIAN_POINT('Ctrl Pts',(21.4517346237734,-17.4254488483261,-14.1338378277511));
#37948=CARTESIAN_POINT('Ctrl Pts',(22.3727984841464,-17.72174912934,-13.7614448137587));
#37949=CARTESIAN_POINT('Ctrl Pts',(23.074354337756,-17.9111527143534,-13.5118529399621));
#37950=CARTESIAN_POINT('Ctrl Pts',(23.7582742987063,-18.0719640430561,-13.3034745440379));
#37951=CARTESIAN_POINT('Ctrl Pts',(24.2174386855894,-18.1719103336477,-13.1693266480666));
#37952=CARTESIAN_POINT('Ctrl Pts',(24.7870213943587,-18.2785218143408,-13.020703786838));
#37953=CARTESIAN_POINT('Ctrl Pts',(25.2463470121634,-18.3542161979472,-12.9133861579982));
#37954=CARTESIAN_POINT('Ctrl Pts',(25.5899787396419,-18.4056632423986,-12.8400372670538));
#37955=CARTESIAN_POINT('Ctrl Pts',(25.8759048428224,-18.444266017472,-12.7850917865304));
#37956=CARTESIAN_POINT('Ctrl Pts',(26.0755068065029,-18.4689567859641,-12.7502361709813));
#37957=CARTESIAN_POINT('Ctrl Pts',(26.1893780149128,-18.4824083304412,-12.7313725692328));
#37958=CARTESIAN_POINT('Ctrl Pts',(26.2462863876019,-18.4889145361419,-12.7222969574594));
#37959=CARTESIAN_POINT('Ctrl Pts',(26.7102722067271,-18.5411896593429,-12.6496548741737));
#37960=CARTESIAN_POINT('Ctrl Pts',(27.5960905386886,-18.6020458648121,-12.5614420302555));
#37961=CARTESIAN_POINT('Ctrl Pts',(28.5798438027286,-18.629899960324,-12.5173520665108));
#37962=CARTESIAN_POINT('Ctrl Pts',(29.1658297917577,-18.6480680632814,-12.4906249890439));
#37963=CARTESIAN_POINT('Ctrl Pts',(29.3147155528138,-18.6521962493032,-12.4846522276656));
#37964=CARTESIAN_POINT('Ctrl Pts',(29.6257654938391,-18.6585637397073,-12.4753713397182));
#37965=CARTESIAN_POINT('Ctrl Pts',(30.1719616098277,-18.6644443298454,-12.4668129248999));
#37966=CARTESIAN_POINT('Ctrl Pts',(31.2977738410334,-18.6602190141086,-12.472961188488));
#37967=CARTESIAN_POINT('Ctrl Pts',(32.3068669150108,-18.6445149503826,-12.4961463862896));
#37968=CARTESIAN_POINT('Ctrl Pts',(33.1709127040733,-18.6444874715365,-12.4962026881972));
#37969=CARTESIAN_POINT('Ctrl Pts',(33.4960830255433,-18.644484418038,-12.4962093123004));
#37970=CARTESIAN_POINT('Ctrl Pts',(34.1563135822162,-18.6444789016084,-12.4962208405723));
#37971=CARTESIAN_POINT('Ctrl Pts',(34.9772414248898,-18.6444614154564,-12.4962577684095));
#37972=CARTESIAN_POINT('Ctrl Pts',(35.964946372113,-18.6444542286038,-12.496272896639));
#37973=CARTESIAN_POINT('Ctrl Pts',(37.9391834323222,-18.6444443083029,-12.4962938290756));
#37974=CARTESIAN_POINT('Ctrl Pts',(39.5833333333333,-18.6443951831047,-12.4963973854122));
#37975=CARTESIAN_POINT('Ctrl Pts',(40.9,-18.6443951831047,-12.4963973854122));
#37976=CARTESIAN_POINT('Ctrl Pts',(6.90857970435318,-7.02038826853569,-29.5800408844791));
#37977=CARTESIAN_POINT('Ctrl Pts',(7.67983757144493,-8.58577901088989,-29.1962153577801));
#37978=CARTESIAN_POINT('Ctrl Pts',(8.4844629659692,-10.0765485557758,-28.7191114013952));
#37979=CARTESIAN_POINT('Ctrl Pts',(10.2687526859613,-13.0935628879538,-27.5023711977385));
#37980=CARTESIAN_POINT('Ctrl Pts',(11.2489627292759,-14.6224501564806,-26.6949552438923));
#37981=CARTESIAN_POINT('Ctrl Pts',(13.2065810728343,-17.2294066625499,-25.1069038454382));
#37982=CARTESIAN_POINT('Ctrl Pts',(14.188432579866,-18.4069952853951,-24.2271697832519));
#37983=CARTESIAN_POINT('Ctrl Pts',(15.4296983589676,-19.6550892131211,-23.2080338536349));
#37984=CARTESIAN_POINT('Ctrl Pts',(16.3788042670986,-20.5796860932724,-22.4189011948389));
#37985=CARTESIAN_POINT('Ctrl Pts',(17.3450159165718,-21.3903231452907,-21.6217224592711));
#37986=CARTESIAN_POINT('Ctrl Pts',(18.9999962645462,-22.5937460627634,-20.3951481814249));
#37987=CARTESIAN_POINT('Ctrl Pts',(19.9686658165165,-23.1898054127389,-19.6835411202358));
#37988=CARTESIAN_POINT('Ctrl Pts',(21.1489437168841,-23.7756910485749,-18.9783964629487));
#37989=CARTESIAN_POINT('Ctrl Pts',(21.6136662410167,-23.9949385633152,-18.7043064424585));
#37990=CARTESIAN_POINT('Ctrl Pts',(22.5341605437882,-24.3846521737583,-18.1932305660766));
#37991=CARTESIAN_POINT('Ctrl Pts',(23.2310352415763,-24.631517887271,-17.8537326154787));
#37992=CARTESIAN_POINT('Ctrl Pts',(23.904768062761,-24.8394315921367,-17.5731511638352));
#37993=CARTESIAN_POINT('Ctrl Pts',(24.3593217251593,-24.9695871891301,-17.3912549800691));
#37994=CARTESIAN_POINT('Ctrl Pts',(24.9191284505008,-25.1069751863358,-17.1917285847407));
#37995=CARTESIAN_POINT('Ctrl Pts',(25.3687829483026,-25.2041659752935,-17.0482631873592));
#37996=CARTESIAN_POINT('Ctrl Pts',(25.703880946624,-25.269917189492,-16.9507036504243));
#37997=CARTESIAN_POINT('Ctrl Pts',(25.981527527538,-25.3190677310923,-16.8779731233104));
#37998=CARTESIAN_POINT('Ctrl Pts',(26.1747255747308,-25.3504124116977,-16.832023377701));
#37999=CARTESIAN_POINT('Ctrl Pts',(26.2847430019941,-25.3674660195527,-16.8072090098453));
#38000=CARTESIAN_POINT('Ctrl Pts',(26.3396756125252,-25.3757090167854,-16.7952849898385));
#38001=CARTESIAN_POINT('Ctrl Pts',(26.7867185605548,-25.4418392909474,-16.7000344271697));
#38002=CARTESIAN_POINT('Ctrl Pts',(27.6343089133551,-25.5185659559043,-16.5847364280863));
#38003=CARTESIAN_POINT('Ctrl Pts',(28.6086204191331,-25.5552242576154,-16.5243820587323));
#38004=CARTESIAN_POINT('Ctrl Pts',(29.1952293795949,-25.5792110357046,-16.4877244301025));
#38005=CARTESIAN_POINT('Ctrl Pts',(29.3380035933319,-25.584403327273,-16.4799452423709));
#38006=CARTESIAN_POINT('Ctrl Pts',(29.6413717635321,-25.5925899885791,-16.4675695714433));
#38007=CARTESIAN_POINT('Ctrl Pts',(30.174536806517,-25.6001268754995,-16.4561967872262));
#38008=CARTESIAN_POINT('Ctrl Pts',(31.2855894033322,-25.5947346655064,-16.464330041984));
#38009=CARTESIAN_POINT('Ctrl Pts',(32.2974015084455,-25.5738307704501,-16.4964013295029));
#38010=CARTESIAN_POINT('Ctrl Pts',(33.1731651112182,-25.5737672879574,-16.4965224425527));
#38011=CARTESIAN_POINT('Ctrl Pts',(33.4969081472871,-25.57375987162,-16.4965369996129));
#38012=CARTESIAN_POINT('Ctrl Pts',(34.1578169391039,-25.5737469053194,-16.4965619872358));
#38013=CARTESIAN_POINT('Ctrl Pts',(34.9780359591179,-25.5737054251286,-16.496642344611));
#38014=CARTESIAN_POINT('Ctrl Pts',(35.9658147840134,-25.5736884251095,-16.4966752246752));
#38015=CARTESIAN_POINT('Ctrl Pts',(37.9397802282712,-25.5736649097449,-16.4967207607426));
#38016=CARTESIAN_POINT('Ctrl Pts',(39.5833333333333,-25.5735485612246,-16.4969459535258));
#38017=CARTESIAN_POINT('Ctrl Pts',(40.9,-25.5735485612246,-16.4969459535258));
#38018=CARTESIAN_POINT('Ctrl Pts',(6.93528330520032,-8.231730283379,-33.9890447223856));
#38019=CARTESIAN_POINT('Ctrl Pts',(7.70864561497005,-10.0357116563145,-33.5376786188307));
#38020=CARTESIAN_POINT('Ctrl Pts',(8.51532719250786,-11.7528338486872,-32.9786927413523));
#38021=CARTESIAN_POINT('Ctrl Pts',(10.3033707684643,-15.2242195800702,-31.5578840442132));
#38022=CARTESIAN_POINT('Ctrl Pts',(11.285359425586,-16.9818886494149,-30.6179424293771));
#38023=CARTESIAN_POINT('Ctrl Pts',(13.2503075123955,-19.9828238609275,-28.7660858779662));
#38024=CARTESIAN_POINT('Ctrl Pts',(14.2335802328307,-21.333808720003,-27.744590382611));
#38025=CARTESIAN_POINT('Ctrl Pts',(15.4809874764708,-22.7701484639683,-26.5562215055806));
#38026=CARTESIAN_POINT('Ctrl Pts',(16.4318967140332,-23.8303538982284,-25.6398645222147));
#38027=CARTESIAN_POINT('Ctrl Pts',(17.4027860882061,-24.7620955812504,-24.7114068344531));
#38028=CARTESIAN_POINT('Ctrl Pts',(19.0657008739464,-26.1438767914272,-23.2827894621994));
#38029=CARTESIAN_POINT('Ctrl Pts',(20.0370987955263,-26.8257745442827,-22.4568785783624));
#38030=CARTESIAN_POINT('Ctrl Pts',(21.2219373681819,-27.4963832022122,-21.6368752952081));
#38031=CARTESIAN_POINT('Ctrl Pts',(21.6873545199147,-27.7466423667127,-21.3192655757679));
#38032=CARTESIAN_POINT('Ctrl Pts',(22.6095407883916,-28.1914275999318,-20.7266792263566));
#38033=CARTESIAN_POINT('Ctrl Pts',(23.306319546872,-28.4721721598033,-20.33420635525));
#38034=CARTESIAN_POINT('Ctrl Pts',(23.97749158379,-28.7077527668379,-20.0111563083465));
#38035=CARTESIAN_POINT('Ctrl Pts',(24.4307021142574,-28.8553793495036,-19.8016082531842));
#38036=CARTESIAN_POINT('Ctrl Pts',(24.9871188326861,-29.0105626137836,-19.5726095610119));
#38037=CARTESIAN_POINT('Ctrl Pts',(25.4329141726814,-29.1200357132464,-19.4084486444522));
#38038=CARTESIAN_POINT('Ctrl Pts',(25.7643950554697,-29.1939083663023,-19.2971155191107));
#38039=CARTESIAN_POINT('Ctrl Pts',(26.0382972138575,-29.2489718106938,-19.2143910494173));
#38040=CARTESIAN_POINT('Ctrl Pts',(26.2284820979133,-29.2840172105126,-19.1622606931669));
#38041=CARTESIAN_POINT('Ctrl Pts',(26.336649445506,-29.3030632173394,-19.1341507449285));
#38042=CARTESIAN_POINT('Ctrl Pts',(26.3906225284364,-29.3122642693063,-19.1206543727096));
#38043=CARTESIAN_POINT('Ctrl Pts',(26.8293654116031,-29.3859982106889,-19.012988583459));
#38044=CARTESIAN_POINT('Ctrl Pts',(27.6560988760144,-29.4710985842865,-18.8833816200193));
#38045=CARTESIAN_POINT('Ctrl Pts',(28.6249317030318,-29.5127595133997,-18.8137794716615));
#38046=CARTESIAN_POINT('Ctrl Pts',(29.2119052185273,-29.5400636810177,-18.7714558506415));
#38047=CARTESIAN_POINT('Ctrl Pts',(29.351223493954,-29.5458124634024,-18.7627335234215));
#38048=CARTESIAN_POINT('Ctrl Pts',(29.6502234545151,-29.5549926880432,-18.7486685476099));
#38049=CARTESIAN_POINT('Ctrl Pts',(30.1759548990665,-29.5634265890421,-18.7357718416966));
#38050=CARTESIAN_POINT('Ctrl Pts',(31.2785766862301,-29.5574021311857,-18.7449771625331));
#38051=CARTESIAN_POINT('Ctrl Pts',(32.2919610610309,-29.5334837411524,-18.7821959068194));
#38052=CARTESIAN_POINT('Ctrl Pts',(33.1744263360525,-29.533390407254,-18.7823679845324));
#38053=CARTESIAN_POINT('Ctrl Pts',(33.4973548461808,-29.5333792377698,-18.7823889294252));
#38054=CARTESIAN_POINT('Ctrl Pts',(34.1586526208335,-29.5333600113094,-18.7824245927187));
#38055=CARTESIAN_POINT('Ctrl Pts',(34.978471543808,-29.5332982308031,-18.7825395490483));
#38056=CARTESIAN_POINT('Ctrl Pts',(35.9662945600334,-29.5332729456428,-18.782586552422));
#38057=CARTESIAN_POINT('Ctrl Pts',(37.9401075800399,-29.533237934286,-18.7826516826344));
#38058=CARTESIAN_POINT('Ctrl Pts',(39.5833333333333,-29.533064777293,-18.7829737067337));
#38059=CARTESIAN_POINT('Ctrl Pts',(40.9,-29.533064777293,-18.7829737067337));
#38060=CARTESIAN_POINT('Origin',(6.9,-30.,3.67394039744206E-15));
#38061=CARTESIAN_POINT('',(6.9,-20.5775906479515,-21.8303175223207));
#38062=CARTESIAN_POINT('Ctrl Pts',(6.9,-7.09789564133157,-8.44145532612415));
#38063=CARTESIAN_POINT('Ctrl Pts',(6.9,-9.87986401752105,-11.09468188726));
#38064=CARTESIAN_POINT('Ctrl Pts',(6.90000000166257,-12.753513475675,-13.9485622548227));
#38065=CARTESIAN_POINT('Ctrl Pts',(6.90000000166257,-16.8843019432417,-18.0885125115534));
#38066=CARTESIAN_POINT('Ctrl Pts',(6.9,-18.7449692586141,-19.9691972794379));
#38067=CARTESIAN_POINT('Ctrl Pts',(6.9,-20.5775906479515,-21.8303175223207));
#38068=CARTESIAN_POINT('Origin',(6.9,0.,0.));
#38069=CARTESIAN_POINT('Origin',(40.9,-9.,1.10218211923262E-15));
#38070=CARTESIAN_POINT('Ctrl Pts',(40.9,-34.4673758792282,-1.5));
#38071=CARTESIAN_POINT('Ctrl Pts',(40.9,-33.9668810740701,-1.5));
#38072=CARTESIAN_POINT('Ctrl Pts',(40.9,-33.466386268912,-1.5));
#38073=CARTESIAN_POINT('Ctrl Pts',(40.9,-32.9658914637539,-1.5));
#38074=CARTESIAN_POINT('Ctrl Pts',(30.5,-34.9651684126997,1.56108868151375));
#38075=CARTESIAN_POINT('Ctrl Pts',(30.5,-35.,0.780932928377884));
#38076=CARTESIAN_POINT('Ctrl Pts',(30.5,-35.,4.28626379701574E-15));
#38077=CARTESIAN_POINT('Ctrl Pts',(30.5,-35.,-35.));
#38078=CARTESIAN_POINT('Ctrl Pts',(30.5,-4.28626379701574E-15,-35.));
#38079=CARTESIAN_POINT('Ctrl Pts',(30.5,35.,-35.));
#38080=CARTESIAN_POINT('Ctrl Pts',(30.5,35.,-4.28626379701574E-15));
#38081=CARTESIAN_POINT('Ctrl Pts',(30.5,35.,35.));
#38082=CARTESIAN_POINT('Ctrl Pts',(30.5,4.28626379701574E-15,35.));
#38083=CARTESIAN_POINT('Ctrl Pts',(30.5,-33.472222479613,35.));
#38084=CARTESIAN_POINT('Ctrl Pts',(30.5,-34.9651684126997,1.56108868151375));
#38085=CARTESIAN_POINT('Ctrl Pts',(30.3311478274255,-34.8898028105656,1.55772383604588));
#38086=CARTESIAN_POINT('Ctrl Pts',(30.3311478274255,-34.924559320191,0.779249668063539));
#38087=CARTESIAN_POINT('Ctrl Pts',(30.3311478274255,-34.924559320191,4.27702497831037E-15));
#38088=CARTESIAN_POINT('Ctrl Pts',(30.3311478274255,-34.924559320191,-34.924559320191));
#38089=CARTESIAN_POINT('Ctrl Pts',(30.3311478274255,-4.27702497831037E-15,
-34.924559320191));
#38090=CARTESIAN_POINT('Ctrl Pts',(30.3311478274255,34.924559320191,-34.924559320191));
#38091=CARTESIAN_POINT('Ctrl Pts',(30.3311478274255,34.924559320191,-4.27702497831037E-15));
#38092=CARTESIAN_POINT('Ctrl Pts',(30.3311478274255,34.924559320191,34.924559320191));
#38093=CARTESIAN_POINT('Ctrl Pts',(30.3311478274255,4.27702497831037E-15,
34.924559320191));
#38094=CARTESIAN_POINT('Ctrl Pts',(30.3311478274255,-33.4000748447964,34.924559320191));
#38095=CARTESIAN_POINT('Ctrl Pts',(30.3311478274255,-34.8898028105656,1.55772383604588));
#38096=CARTESIAN_POINT('Ctrl Pts',(29.9897712690917,-34.7371408974366,1.55090794481747));
#38097=CARTESIAN_POINT('Ctrl Pts',(29.9897712690917,-34.7717453283792,0.775840025831461));
#38098=CARTESIAN_POINT('Ctrl Pts',(29.9897712690917,-34.7717453283792,4.25831066171665E-15));
#38099=CARTESIAN_POINT('Ctrl Pts',(29.9897712690917,-34.7717453283791,-34.7717453283791));
#38100=CARTESIAN_POINT('Ctrl Pts',(29.9897712690917,-4.25831066171665E-15,
-34.7717453283792));
#38101=CARTESIAN_POINT('Ctrl Pts',(29.9897712690917,34.7717453283791,-34.7717453283791));
#38102=CARTESIAN_POINT('Ctrl Pts',(29.9897712690917,34.7717453283792,-4.25831066171665E-15));
#38103=CARTESIAN_POINT('Ctrl Pts',(29.9897712690917,34.7717453283791,34.7717453283791));
#38104=CARTESIAN_POINT('Ctrl Pts',(29.9897712690917,4.25831066171665E-15,
34.7717453283792));
#38105=CARTESIAN_POINT('Ctrl Pts',(29.9897712690917,-33.2539313038843,34.7717453283791));
#38106=CARTESIAN_POINT('Ctrl Pts',(29.9897712690917,-34.7371408974366,1.55090794481747));
#38107=CARTESIAN_POINT('Ctrl Pts',(29.4666899049319,-34.5023553003819,1.54042548027394));
#38108=CARTESIAN_POINT('Ctrl Pts',(29.4666899049319,-34.5367258427036,0.770596184255047));
#38109=CARTESIAN_POINT('Ctrl Pts',(29.4666899049319,-34.5367258427036,4.22952907562966E-15));
#38110=CARTESIAN_POINT('Ctrl Pts',(29.4666899049319,-34.5367258427036,-34.5367258427036));
#38111=CARTESIAN_POINT('Ctrl Pts',(29.4666899049319,-4.22952907562966E-15,
-34.5367258427036));
#38112=CARTESIAN_POINT('Ctrl Pts',(29.4666899049319,34.5367258427036,-34.5367258427036));
#38113=CARTESIAN_POINT('Ctrl Pts',(29.4666899049319,34.5367258427036,-4.22952907562966E-15));
#38114=CARTESIAN_POINT('Ctrl Pts',(29.4666899049319,34.5367258427036,34.5367258427036));
#38115=CARTESIAN_POINT('Ctrl Pts',(29.4666899049319,4.22952907562966E-15,
34.5367258427036));
#38116=CARTESIAN_POINT('Ctrl Pts',(29.4666899049319,-33.0291706035535,34.5367258427036));
#38117=CARTESIAN_POINT('Ctrl Pts',(29.4666899049319,-34.5023553003819,1.54042548027394));
#38118=CARTESIAN_POINT('Ctrl Pts',(28.7471241621752,-34.1776802811774,1.52592972576568));
#38119=CARTESIAN_POINT('Ctrl Pts',(28.7471241621752,-34.21172738887,0.763344698704459));
#38120=CARTESIAN_POINT('Ctrl Pts',(28.7471241621752,-34.21172738887,4.18972824400814E-15));
#38121=CARTESIAN_POINT('Ctrl Pts',(28.7471241621752,-34.2117273888699,-34.2117273888699));
#38122=CARTESIAN_POINT('Ctrl Pts',(28.7471241621752,-4.18972824400814E-15,
-34.21172738887));
#38123=CARTESIAN_POINT('Ctrl Pts',(28.7471241621752,34.2117273888699,-34.2117273888699));
#38124=CARTESIAN_POINT('Ctrl Pts',(28.7471241621752,34.21172738887,-4.18972824400814E-15));
#38125=CARTESIAN_POINT('Ctrl Pts',(28.7471241621752,34.2117273888699,34.2117273888699));
#38126=CARTESIAN_POINT('Ctrl Pts',(28.7471241621752,4.18972824400814E-15,
34.21172738887));
#38127=CARTESIAN_POINT('Ctrl Pts',(28.7471241621752,-32.718358587775,34.2117273888699));
#38128=CARTESIAN_POINT('Ctrl Pts',(28.7471241621752,-34.1776802811774,1.52592972576568));
#38129=CARTESIAN_POINT('Ctrl Pts',(27.8100958442934,-33.7532520886149,1.50698029472894));
#38130=CARTESIAN_POINT('Ctrl Pts',(27.8100958442934,-33.7868763896026,0.753865266276398));
#38131=CARTESIAN_POINT('Ctrl Pts',(27.8100958442934,-33.7868763896026,4.13769900237141E-15));
#38132=CARTESIAN_POINT('Ctrl Pts',(27.8100958442934,-33.7868763896026,-33.7868763896026));
#38133=CARTESIAN_POINT('Ctrl Pts',(27.8100958442934,-4.13769900237141E-15,
-33.7868763896026));
#38134=CARTESIAN_POINT('Ctrl Pts',(27.8100958442934,33.7868763896026,-33.7868763896026));
#38135=CARTESIAN_POINT('Ctrl Pts',(27.8100958442934,33.7868763896026,-4.13769900237141E-15));
#38136=CARTESIAN_POINT('Ctrl Pts',(27.8100958442934,33.7868763896026,33.7868763896026));
#38137=CARTESIAN_POINT('Ctrl Pts',(27.8100958442934,4.13769900237141E-15,
33.7868763896026));
#38138=CARTESIAN_POINT('Ctrl Pts',(27.8100958442934,-32.3120526686846,33.7868763896026));
#38139=CARTESIAN_POINT('Ctrl Pts',(27.8100958442934,-33.7532520886149,1.50698029472894));
#38140=CARTESIAN_POINT('Ctrl Pts',(26.8343111708818,-33.3132226048841,1.48733431337754));
#38141=CARTESIAN_POINT('Ctrl Pts',(26.8343111708818,-33.3464085574791,0.74403738530507));
#38142=CARTESIAN_POINT('Ctrl Pts',(26.8343111708818,-33.3464085574791,4.08375725029767E-15));
#38143=CARTESIAN_POINT('Ctrl Pts',(26.8343111708818,-33.3464085574791,-33.3464085574791));
#38144=CARTESIAN_POINT('Ctrl Pts',(26.8343111708818,-4.08375725029767E-15,
-33.3464085574791));
#38145=CARTESIAN_POINT('Ctrl Pts',(26.8343111708818,33.3464085574791,-33.3464085574791));
#38146=CARTESIAN_POINT('Ctrl Pts',(26.8343111708818,33.3464085574791,-4.08375725029767E-15));
#38147=CARTESIAN_POINT('Ctrl Pts',(26.8343111708818,33.3464085574791,33.3464085574791));
#38148=CARTESIAN_POINT('Ctrl Pts',(26.8343111708818,4.08375725029767E-15,
33.3464085574791));
#38149=CARTESIAN_POINT('Ctrl Pts',(26.8343111708818,-31.8908116037717,33.3464085574791));
#38150=CARTESIAN_POINT('Ctrl Pts',(26.8343111708818,-33.3132226048841,1.48733431337754));
#38151=CARTESIAN_POINT('Ctrl Pts',(25.8181479469611,-32.8638045923198,1.46726916269953));
#38152=CARTESIAN_POINT('Ctrl Pts',(25.8181479469611,-32.8965428438611,0.733999815330427));
#38153=CARTESIAN_POINT('Ctrl Pts',(25.8181479469611,-32.8965428438611,4.02866458967482E-15));
#38154=CARTESIAN_POINT('Ctrl Pts',(25.8181479469611,-32.896542843861,-32.896542843861));
#38155=CARTESIAN_POINT('Ctrl Pts',(25.8181479469611,-4.02866458967482E-15,
-32.8965428438611));
#38156=CARTESIAN_POINT('Ctrl Pts',(25.8181479469611,32.896542843861,-32.896542843861));
#38157=CARTESIAN_POINT('Ctrl Pts',(25.8181479469611,32.8965428438611,-4.02866458967482E-15));
#38158=CARTESIAN_POINT('Ctrl Pts',(25.8181479469611,32.896542843861,32.896542843861));
#38159=CARTESIAN_POINT('Ctrl Pts',(25.8181479469611,4.02866458967482E-15,
32.8965428438611));
#38160=CARTESIAN_POINT('Ctrl Pts',(25.8181479469611,-31.4605828822811,32.896542843861));
#38161=CARTESIAN_POINT('Ctrl Pts',(25.8181479469611,-32.8638045923198,1.46726916269953));
#38162=CARTESIAN_POINT('Ctrl Pts',(24.7595197917227,-32.4162193763075,1.44728584082668));
#38163=CARTESIAN_POINT('Ctrl Pts',(24.7595197917227,-32.4485117525897,0.724003180127259));
#38164=CARTESIAN_POINT('Ctrl Pts',(24.7595197917227,-32.4485117525897,3.97379660549043E-15));
#38165=CARTESIAN_POINT('Ctrl Pts',(24.7595197917227,-32.4485117525897,-32.4485117525897));
#38166=CARTESIAN_POINT('Ctrl Pts',(24.7595197917227,-3.97379660549043E-15,
-32.4485117525897));
#38167=CARTESIAN_POINT('Ctrl Pts',(24.7595197917227,32.4485117525897,-32.4485117525897));
#38168=CARTESIAN_POINT('Ctrl Pts',(24.7595197917227,32.4485117525897,-3.97379660549043E-15));
#38169=CARTESIAN_POINT('Ctrl Pts',(24.7595197917227,32.4485117525897,32.4485117525897));
#38170=CARTESIAN_POINT('Ctrl Pts',(24.7595197917227,3.97379660549043E-15,
32.4485117525897));
#38171=CARTESIAN_POINT('Ctrl Pts',(24.7595197917227,-31.0321087004291,32.4485117525897));
#38172=CARTESIAN_POINT('Ctrl Pts',(24.7595197917227,-32.4162193763075,1.44728584082668));
#38173=CARTESIAN_POINT('Ctrl Pts',(23.6563574780851,-31.9852629652417,1.42804494464108));
#38174=CARTESIAN_POINT('Ctrl Pts',(23.6563574780851,-32.017126031541,0.714377942573002));
#38175=CARTESIAN_POINT('Ctrl Pts',(23.6563574780851,-32.017126031541,3.92096709124241E-15));
#38176=CARTESIAN_POINT('Ctrl Pts',(23.6563574780851,-32.017126031541,-32.017126031541));
#38177=CARTESIAN_POINT('Ctrl Pts',(23.6563574780851,-3.92096709124241E-15,
-32.017126031541));
#38178=CARTESIAN_POINT('Ctrl Pts',(23.6563574780851,32.017126031541,-32.017126031541));
#38179=CARTESIAN_POINT('Ctrl Pts',(23.6563574780851,32.017126031541,-3.92096709124241E-15));
#38180=CARTESIAN_POINT('Ctrl Pts',(23.6563574780851,32.017126031541,32.017126031541));
#38181=CARTESIAN_POINT('Ctrl Pts',(23.6563574780851,3.92096709124241E-15,
32.017126031541));
#38182=CARTESIAN_POINT('Ctrl Pts',(23.6563574780851,-30.6195533053013,32.017126031541));
#38183=CARTESIAN_POINT('Ctrl Pts',(23.6563574780851,-31.9852629652417,1.42804494464108));
#38184=CARTESIAN_POINT('Ctrl Pts',(22.5073180101405,-31.5864702700101,1.41024006077928));
#38185=CARTESIAN_POINT('Ctrl Pts',(22.5073180101405,-31.6179360671638,0.705471068634142));
#38186=CARTESIAN_POINT('Ctrl Pts',(22.5073180101405,-31.6179360671638,3.87208042002978E-15));
#38187=CARTESIAN_POINT('Ctrl Pts',(22.5073180101405,-31.6179360671638,-31.6179360671638));
#38188=CARTESIAN_POINT('Ctrl Pts',(22.5073180101405,-3.87208042002978E-15,
-31.6179360671638));
#38189=CARTESIAN_POINT('Ctrl Pts',(22.5073180101405,31.6179360671638,-31.6179360671638));
#38190=CARTESIAN_POINT('Ctrl Pts',(22.5073180101405,31.6179360671638,-3.87208042002978E-15));
#38191=CARTESIAN_POINT('Ctrl Pts',(22.5073180101405,31.6179360671638,31.6179360671638));
#38192=CARTESIAN_POINT('Ctrl Pts',(22.5073180101405,3.87208042002978E-15,
31.6179360671638));
#38193=CARTESIAN_POINT('Ctrl Pts',(22.5073180101405,-30.237788296751,31.6179360671638));
#38194=CARTESIAN_POINT('Ctrl Pts',(22.5073180101405,-31.5864702700101,1.41024006077928));
#38195=CARTESIAN_POINT('Ctrl Pts',(21.3125219557939,-31.2336232862855,1.394486513532));
#38196=CARTESIAN_POINT('Ctrl Pts',(21.3125219557939,-31.264737584474,0.697590373623125));
#38197=CARTESIAN_POINT('Ctrl Pts',(21.3125219557939,-31.264737584474,3.8288260809008E-15));
#38198=CARTESIAN_POINT('Ctrl Pts',(21.3125219557939,-31.264737584474,-31.264737584474));
#38199=CARTESIAN_POINT('Ctrl Pts',(21.3125219557939,-3.8288260809008E-15,
-31.264737584474));
#38200=CARTESIAN_POINT('Ctrl Pts',(21.3125219557939,31.264737584474,-31.264737584474));
#38201=CARTESIAN_POINT('Ctrl Pts',(21.3125219557939,31.264737584474,-3.8288260809008E-15));
#38202=CARTESIAN_POINT('Ctrl Pts',(21.3125219557939,31.264737584474,31.264737584474));
#38203=CARTESIAN_POINT('Ctrl Pts',(21.3125219557939,3.8288260809008E-15,
31.264737584474));
#38204=CARTESIAN_POINT('Ctrl Pts',(21.3125219557939,-29.9000072055494,31.264737584474));
#38205=CARTESIAN_POINT('Ctrl Pts',(21.3125219557939,-31.2336232862855,1.394486513532));
#38206=CARTESIAN_POINT('Ctrl Pts',(20.0742472323676,-30.9363148057487,1.3812125919422));
#38207=CARTESIAN_POINT('Ctrl Pts',(20.0742472323676,-30.9671329312955,0.690950108671537));
#38208=CARTESIAN_POINT('Ctrl Pts',(20.0742472323676,-30.9671329312955,3.79238002230816E-15));
#38209=CARTESIAN_POINT('Ctrl Pts',(20.0742472323676,-30.9671329312955,-30.9671329312955));
#38210=CARTESIAN_POINT('Ctrl Pts',(20.0742472323676,-3.79238002230816E-15,
-30.9671329312955));
#38211=CARTESIAN_POINT('Ctrl Pts',(20.0742472323676,30.9671329312955,-30.9671329312955));
#38212=CARTESIAN_POINT('Ctrl Pts',(20.0742472323676,30.9671329312955,-3.79238002230816E-15));
#38213=CARTESIAN_POINT('Ctrl Pts',(20.0742472323676,30.9671329312955,30.9671329312955));
#38214=CARTESIAN_POINT('Ctrl Pts',(20.0742472323676,3.79238002230816E-15,
30.9671329312955));
#38215=CARTESIAN_POINT('Ctrl Pts',(20.0742472323676,-29.6153932294878,30.9671329312955));
#38216=CARTESIAN_POINT('Ctrl Pts',(20.0742472323676,-30.9363148057487,1.3812125919422));
#38217=CARTESIAN_POINT('Ctrl Pts',(18.7979917002302,-30.6967495040754,1.3705167280896));
#38218=CARTESIAN_POINT('Ctrl Pts',(18.7979917002302,-30.727328979557,0.685599514321031));
#38219=CARTESIAN_POINT('Ctrl Pts',(18.7979917002302,-30.727328979557,3.76301250811622E-15));
#38220=CARTESIAN_POINT('Ctrl Pts',(18.7979917002302,-30.727328979557,-30.727328979557));
#38221=CARTESIAN_POINT('Ctrl Pts',(18.7979917002302,-3.76301250811622E-15,
-30.727328979557));
#38222=CARTESIAN_POINT('Ctrl Pts',(18.7979917002302,30.727328979557,-30.727328979557));
#38223=CARTESIAN_POINT('Ctrl Pts',(18.7979917002302,30.727328979557,-3.76301250811622E-15));
#38224=CARTESIAN_POINT('Ctrl Pts',(18.7979917002302,30.727328979557,30.727328979557));
#38225=CARTESIAN_POINT('Ctrl Pts',(18.7979917002302,3.76301250811622E-15,
30.727328979557));
#38226=CARTESIAN_POINT('Ctrl Pts',(18.7979917002302,-29.3860569087997,30.727328979557));
#38227=CARTESIAN_POINT('Ctrl Pts',(18.7979917002302,-30.6967495040754,1.3705167280896));
#38228=CARTESIAN_POINT('Ctrl Pts',(17.4917404060759,-30.5108523315028,1.36221698336642));
#38229=CARTESIAN_POINT('Ctrl Pts',(17.4917404060759,-30.5412466200144,0.681447575979399));
#38230=CARTESIAN_POINT('Ctrl Pts',(17.4917404060759,-30.5412466200144,3.74022399151705E-15));
#38231=CARTESIAN_POINT('Ctrl Pts',(17.4917404060759,-30.5412466200144,-30.5412466200144));
#38232=CARTESIAN_POINT('Ctrl Pts',(17.4917404060759,-3.74022399151705E-15,
-30.5412466200144));
#38233=CARTESIAN_POINT('Ctrl Pts',(17.4917404060759,30.5412466200144,-30.5412466200144));
#38234=CARTESIAN_POINT('Ctrl Pts',(17.4917404060759,30.5412466200144,-3.74022399151705E-15));
#38235=CARTESIAN_POINT('Ctrl Pts',(17.4917404060759,30.5412466200144,30.5412466200144));
#38236=CARTESIAN_POINT('Ctrl Pts',(17.4917404060759,3.74022399151705E-15,
30.5412466200144));
#38237=CARTESIAN_POINT('Ctrl Pts',(17.4917404060759,-29.2080971905671,30.5412466200144));
#38238=CARTESIAN_POINT('Ctrl Pts',(17.4917404060759,-30.5108523315028,1.36221698336642));
#38239=CARTESIAN_POINT('Ctrl Pts',(16.1647270995715,-30.3706357712668,1.35595673938413));
#38240=CARTESIAN_POINT('Ctrl Pts',(16.1647270995715,-30.4008903789023,0.678315895682606));
#38241=CARTESIAN_POINT('Ctrl Pts',(16.1647270995715,-30.4008903789023,3.72303530937522E-15));
#38242=CARTESIAN_POINT('Ctrl Pts',(16.1647270995715,-30.4008903789023,-30.4008903789023));
#38243=CARTESIAN_POINT('Ctrl Pts',(16.1647270995715,-3.72303530937522E-15,
-30.4008903789023));
#38244=CARTESIAN_POINT('Ctrl Pts',(16.1647270995715,30.4008903789023,-30.4008903789023));
#38245=CARTESIAN_POINT('Ctrl Pts',(16.1647270995715,30.4008903789023,-3.72303530937522E-15));
#38246=CARTESIAN_POINT('Ctrl Pts',(16.1647270995715,30.4008903789023,30.4008903789023));
#38247=CARTESIAN_POINT('Ctrl Pts',(16.1647270995715,3.72303530937522E-15,
30.4008903789023));
#38248=CARTESIAN_POINT('Ctrl Pts',(16.1647270995715,-29.0738676097412,30.4008903789023));
#38249=CARTESIAN_POINT('Ctrl Pts',(16.1647270995715,-30.3706357712668,1.35595673938413));
#38250=CARTESIAN_POINT('Ctrl Pts',(14.8263876417415,-30.2660684364343,1.3512881251525));
#38251=CARTESIAN_POINT('Ctrl Pts',(14.8263876417415,-30.2962188762245,0.675980426451068));
#38252=CARTESIAN_POINT('Ctrl Pts',(14.8263876417415,-30.2962188762246,3.7102167473036E-15));
#38253=CARTESIAN_POINT('Ctrl Pts',(14.8263876417415,-30.2962188762245,-30.2962188762245));
#38254=CARTESIAN_POINT('Ctrl Pts',(14.8263876417415,-3.7102167473036E-15,
-30.2962188762246));
#38255=CARTESIAN_POINT('Ctrl Pts',(14.8263876417415,30.2962188762245,-30.2962188762245));
#38256=CARTESIAN_POINT('Ctrl Pts',(14.8263876417415,30.2962188762246,-3.7102167473036E-15));
#38257=CARTESIAN_POINT('Ctrl Pts',(14.8263876417415,30.2962188762245,30.2962188762245));
#38258=CARTESIAN_POINT('Ctrl Pts',(14.8263876417415,3.7102167473036E-15,
30.2962188762246));
#38259=CARTESIAN_POINT('Ctrl Pts',(14.8263876417415,-28.9737651004582,30.2962188762245));
#38260=CARTESIAN_POINT('Ctrl Pts',(14.8263876417415,-30.2660684364343,1.3512881251525));
#38261=CARTESIAN_POINT('Ctrl Pts',(13.4853470903953,-30.186937862885,1.34775518513426));
#38262=CARTESIAN_POINT('Ctrl Pts',(13.4853470903953,-30.2170094744125,0.674213077019293));
#38263=CARTESIAN_POINT('Ctrl Pts',(13.4853470903953,-30.2170094744125,3.70051639326446E-15));
#38264=CARTESIAN_POINT('Ctrl Pts',(13.4853470903953,-30.2170094744125,-30.2170094744125));
#38265=CARTESIAN_POINT('Ctrl Pts',(13.4853470903953,-3.70051639326446E-15,
-30.2170094744125));
#38266=CARTESIAN_POINT('Ctrl Pts',(13.4853470903953,30.2170094744125,-30.2170094744125));
#38267=CARTESIAN_POINT('Ctrl Pts',(13.4853470903953,30.2170094744125,-3.70051639326446E-15));
#38268=CARTESIAN_POINT('Ctrl Pts',(13.4853470903953,30.2170094744125,30.2170094744125));
#38269=CARTESIAN_POINT('Ctrl Pts',(13.4853470903953,3.70051639326446E-15,
30.2170094744125));
#38270=CARTESIAN_POINT('Ctrl Pts',(13.4853470903953,-28.8980132513174,30.2170094744125));
#38271=CARTESIAN_POINT('Ctrl Pts',(13.4853470903953,-30.186937862885,1.34775518513426));
#38272=CARTESIAN_POINT('Ctrl Pts',(12.1482076787549,-30.1249424647305,1.34498727870743));
#38273=CARTESIAN_POINT('Ctrl Pts',(12.1482076787549,-30.1549523177074,0.672828434816078));
#38274=CARTESIAN_POINT('Ctrl Pts',(12.1482076787549,-30.1549523177074,3.69291658343215E-15));
#38275=CARTESIAN_POINT('Ctrl Pts',(12.1482076787549,-30.1549523177074,-30.1549523177074));
#38276=CARTESIAN_POINT('Ctrl Pts',(12.1482076787549,-3.69291658343215E-15,
-30.1549523177074));
#38277=CARTESIAN_POINT('Ctrl Pts',(12.1482076787549,30.1549523177074,-30.1549523177074));
#38278=CARTESIAN_POINT('Ctrl Pts',(12.1482076787549,30.1549523177074,-3.69291658343215E-15));
#38279=CARTESIAN_POINT('Ctrl Pts',(12.1482076787549,30.1549523177074,30.1549523177074));
#38280=CARTESIAN_POINT('Ctrl Pts',(12.1482076787549,3.69291658343215E-15,
30.1549523177074));
#38281=CARTESIAN_POINT('Ctrl Pts',(12.1482076787549,-28.8386649382978,30.1549523177074));
#38282=CARTESIAN_POINT('Ctrl Pts',(12.1482076787549,-30.1249424647305,1.34498727870743));
#38283=CARTESIAN_POINT('Ctrl Pts',(10.8190675759626,-30.0746904138676,1.34274367710657));
#38284=CARTESIAN_POINT('Ctrl Pts',(10.8190675759626,-30.1046502067769,0.67170607553629));
#38285=CARTESIAN_POINT('Ctrl Pts',(10.8190675759626,-30.1046502067769,3.686756351518E-15));
#38286=CARTESIAN_POINT('Ctrl Pts',(10.8190675759626,-30.1046502067769,-30.1046502067769));
#38287=CARTESIAN_POINT('Ctrl Pts',(10.8190675759626,-3.686756351518E-15,
-30.1046502067769));
#38288=CARTESIAN_POINT('Ctrl Pts',(10.8190675759626,30.1046502067769,-30.1046502067769));
#38289=CARTESIAN_POINT('Ctrl Pts',(10.8190675759626,30.1046502067769,-3.686756351518E-15));
#38290=CARTESIAN_POINT('Ctrl Pts',(10.8190675759626,30.1046502067769,30.1046502067769));
#38291=CARTESIAN_POINT('Ctrl Pts',(10.8190675759626,3.686756351518E-15,
30.1046502067769));
#38292=CARTESIAN_POINT('Ctrl Pts',(10.8190675759626,-28.7905585540618,30.1046502067769));
#38293=CARTESIAN_POINT('Ctrl Pts',(10.8190675759626,-30.0746904138676,1.34274367710657));
#38294=CARTESIAN_POINT('Ctrl Pts',(9.50027713254189,-30.032840404991,1.3408752011877));
#38295=CARTESIAN_POINT('Ctrl Pts',(9.50027713254189,-30.0627585077754,0.670771372474119));
#38296=CARTESIAN_POINT('Ctrl Pts',(9.50027713254189,-30.0627585077754,3.68162609800869E-15));
#38297=CARTESIAN_POINT('Ctrl Pts',(9.50027713254189,-30.0627585077753,-30.0627585077753));
#38298=CARTESIAN_POINT('Ctrl Pts',(9.50027713254189,-3.68162609800869E-15,
-30.0627585077754));
#38299=CARTESIAN_POINT('Ctrl Pts',(9.5002771325419,30.0627585077753,-30.0627585077753));
#38300=CARTESIAN_POINT('Ctrl Pts',(9.5002771325419,30.0627585077754,-3.68162609800869E-15));
#38301=CARTESIAN_POINT('Ctrl Pts',(9.5002771325419,30.0627585077753,30.0627585077753));
#38302=CARTESIAN_POINT('Ctrl Pts',(9.50027713254189,3.68162609800869E-15,
30.0627585077754));
#38303=CARTESIAN_POINT('Ctrl Pts',(9.50027713254189,-28.750495460661,30.0627585077754));
#38304=CARTESIAN_POINT('Ctrl Pts',(9.50027713254189,-30.032840404991,1.3408752011877));
#38305=CARTESIAN_POINT('Ctrl Pts',(8.45435372222587,-30.0047244129961,1.33961990745209));
#38306=CARTESIAN_POINT('Ctrl Pts',(8.45435372222587,-30.0346145072029,0.670143413137453));
#38307=CARTESIAN_POINT('Ctrl Pts',(8.45435372222587,-30.0346145072029,3.67817945198707E-15));
#38308=CARTESIAN_POINT('Ctrl Pts',(8.45435372222587,-30.0346145072029,-30.0346145072029));
#38309=CARTESIAN_POINT('Ctrl Pts',(8.45435372222587,-3.67817945198707E-15,
-30.0346145072029));
#38310=CARTESIAN_POINT('Ctrl Pts',(8.45435372222587,30.0346145072029,-30.0346145072029));
#38311=CARTESIAN_POINT('Ctrl Pts',(8.45435372222587,30.0346145072029,-3.67817945198707E-15));
#38312=CARTESIAN_POINT('Ctrl Pts',(8.45435372222587,30.0346145072029,30.0346145072029));
#38313=CARTESIAN_POINT('Ctrl Pts',(8.45435372222587,3.67817945198707E-15,
30.0346145072029));
#38314=CARTESIAN_POINT('Ctrl Pts',(8.45435372222587,-28.7235799678431,30.0346145072029));
#38315=CARTESIAN_POINT('Ctrl Pts',(8.45435372222587,-30.0047244129961,1.33961990745209));
#38316=CARTESIAN_POINT('Ctrl Pts',(7.67514864245731,-29.9863740491064,1.33880061938141));
#38317=CARTESIAN_POINT('Ctrl Pts',(7.67514864245731,-30.0162458630552,0.669733565164178));
#38318=CARTESIAN_POINT('Ctrl Pts',(7.67514864245731,-30.0162458630552,3.67592994186105E-15));
#38319=CARTESIAN_POINT('Ctrl Pts',(7.67514864245731,-30.0162458630552,-30.0162458630552));
#38320=CARTESIAN_POINT('Ctrl Pts',(7.67514864245731,-3.67592994186105E-15,
-30.0162458630552));
#38321=CARTESIAN_POINT('Ctrl Pts',(7.67514864245731,30.0162458630552,-30.0162458630552));
#38322=CARTESIAN_POINT('Ctrl Pts',(7.67514864245731,30.0162458630552,-3.67592994186105E-15));
#38323=CARTESIAN_POINT('Ctrl Pts',(7.67514864245731,30.0162458630552,30.0162458630552));
#38324=CARTESIAN_POINT('Ctrl Pts',(7.67514864245731,3.67592994186105E-15,
30.0162458630552));
#38325=CARTESIAN_POINT('Ctrl Pts',(7.67514864245731,-28.7060131294556,30.0162458630552));
#38326=CARTESIAN_POINT('Ctrl Pts',(7.67514864245731,-29.9863740491064,1.33880061938141));
#38327=CARTESIAN_POINT('Ctrl Pts',(7.15799654185577,-29.9753522996976,1.33830853171149));
#38328=CARTESIAN_POINT('Ctrl Pts',(7.15799654185577,-30.0052131340045,0.669487398838306));
#38329=CARTESIAN_POINT('Ctrl Pts',(7.15799654185577,-30.0052131340045,3.67457882222928E-15));
#38330=CARTESIAN_POINT('Ctrl Pts',(7.15799654185577,-30.0052131340045,-30.0052131340045));
#38331=CARTESIAN_POINT('Ctrl Pts',(7.15799654185577,-3.67457882222928E-15,
-30.0052131340045));
#38332=CARTESIAN_POINT('Ctrl Pts',(7.15799654185577,30.0052131340045,-30.0052131340045));
#38333=CARTESIAN_POINT('Ctrl Pts',(7.15799654185577,30.0052131340045,-3.67457882222928E-15));
#38334=CARTESIAN_POINT('Ctrl Pts',(7.15799654185577,30.0052131340045,30.0052131340045));
#38335=CARTESIAN_POINT('Ctrl Pts',(7.15799654185577,3.67457882222928E-15,
30.0052131340045));
#38336=CARTESIAN_POINT('Ctrl Pts',(7.15799654185577,-28.695461987703,30.0052131340045));
#38337=CARTESIAN_POINT('Ctrl Pts',(7.15799654185577,-29.9753522996976,1.33830853171149));
#38338=CARTESIAN_POINT('Ctrl Pts',(6.9,-29.9701443537426,1.33807601272607));
#38339=CARTESIAN_POINT('Ctrl Pts',(6.9,-30.,0.669371081466758));
#38340=CARTESIAN_POINT('Ctrl Pts',(6.9,-30.,3.67394039744206E-15));
#38341=CARTESIAN_POINT('Ctrl Pts',(6.9,-30.,-30.));
#38342=CARTESIAN_POINT('Ctrl Pts',(6.9,-3.67394039744206E-15,-30.));
#38343=CARTESIAN_POINT('Ctrl Pts',(6.9,30.,-30.));
#38344=CARTESIAN_POINT('Ctrl Pts',(6.9,30.,-3.67394039744206E-15));
#38345=CARTESIAN_POINT('Ctrl Pts',(6.9,30.,30.));
#38346=CARTESIAN_POINT('Ctrl Pts',(6.9,3.67394039744206E-15,30.));
#38347=CARTESIAN_POINT('Ctrl Pts',(6.9,-28.6904764110968,30.));
#38348=CARTESIAN_POINT('Ctrl Pts',(6.9,-29.9701443537426,1.33807601272607));
#38349=CARTESIAN_POINT('Ctrl Pts',(6.9,-20.5775906479515,-21.8303175223207));
#38350=CARTESIAN_POINT('Ctrl Pts',(7.85773098116326,-22.0288565043892,-20.4889265372405));
#38351=CARTESIAN_POINT('Ctrl Pts',(8.88781981167334,-23.3171626725998,-19.0414114324084));
#38352=CARTESIAN_POINT('Ctrl Pts',(10.5914578196776,-25.1150390010341,-16.6247285680552));
#38353=CARTESIAN_POINT('Ctrl Pts',(11.2365058953701,-25.7254166302984,-15.703976734769));
#38354=CARTESIAN_POINT('Ctrl Pts',(12.0558885382926,-26.3926147460599,-14.5853792872662));
#38355=CARTESIAN_POINT('Ctrl Pts',(12.1875764958397,-26.4963665374952,-14.4076425286694));
#38356=CARTESIAN_POINT('Ctrl Pts',(13.194901830313,-27.2691057169114,-13.0552778456719));
#38357=CARTESIAN_POINT('Ctrl Pts',(14.2258982134098,-27.991732600527,-11.6381637544796));
#38358=CARTESIAN_POINT('Ctrl Pts',(18.2616480823244,-29.9350198014187,-6.95587410790868));
#38359=CARTESIAN_POINT('Ctrl Pts',(21.0496416709525,-30.7693084982877,-4.29983295736293));
#38360=CARTESIAN_POINT('Ctrl Pts',(25.8000196361138,-32.8040277065106,-1.93741001991749));
#38361=CARTESIAN_POINT('Ctrl Pts',(26.8976561124457,-33.3305524688301,-1.74039351523169));
#38362=CARTESIAN_POINT('Ctrl Pts',(28.0045908801237,-33.8378020212277,-1.58669630450145));
#38363=CARTESIAN_POINT('Ctrl Pts',(28.5235971652406,-34.0754855762016,-1.54532623843658));
#38364=CARTESIAN_POINT('Ctrl Pts',(29.0834839543824,-34.3307100593381,-1.4982885487127));
#38365=CARTESIAN_POINT('Ctrl Pts',(29.1146288039499,-34.3449058451715,-1.49562082188434));
#38366=CARTESIAN_POINT('Ctrl Pts',(29.5949306848436,-34.5637016811193,-1.45589225448014));
#38367=CARTESIAN_POINT('Ctrl Pts',(30.0492939924726,-34.7685410859787,-1.44682754698748));
#38368=CARTESIAN_POINT('Ctrl Pts',(30.5,-34.9699609326822,-1.44976976333441));
#38369=CARTESIAN_POINT('Ctrl Pts',(6.45331003273164,-6.83943894028999,-8.65286216739172));
#38370=CARTESIAN_POINT('Ctrl Pts',(7.20830533428676,-7.28712780725476,-8.29622318255582));
#38371=CARTESIAN_POINT('Ctrl Pts',(7.99924796920644,-7.69991572864563,-7.91909532230128));
#38372=CARTESIAN_POINT('Ctrl Pts',(9.76163642871394,-8.50127829248443,-7.0702837202071));
#38373=CARTESIAN_POINT('Ctrl Pts',(10.7316626231511,-8.8793528128254,-6.57783879792861));
#38374=CARTESIAN_POINT('Ctrl Pts',(12.6608237755523,-9.49392179513702,-5.67260683532432));
#38375=CARTESIAN_POINT('Ctrl Pts',(13.6376935580087,-9.74868549844379,-5.20677839827646));
#38376=CARTESIAN_POINT('Ctrl Pts',(14.8683081444882,-10.0072371758851,-4.68571756497415));
#38377=CARTESIAN_POINT('Ctrl Pts',(15.814981546047,-10.1933420307132,-4.28615487511135));
#38378=CARTESIAN_POINT('Ctrl Pts',(16.7774761024725,-10.3417484740057,-3.90183726466219));
#38379=CARTESIAN_POINT('Ctrl Pts',(18.4438470226175,-10.5575964922699,-3.30966453460613));
#38380=CARTESIAN_POINT('Ctrl Pts',(19.4166260537867,-10.6478897990578,-2.98271399009539));
#38381=CARTESIAN_POINT('Ctrl Pts',(20.8624415465507,-10.7552000633454,-2.5875063027773));
#38382=CARTESIAN_POINT('Ctrl Pts',(21.8144010701944,-10.8125125199159,-2.34040933534244));
#38383=CARTESIAN_POINT('Ctrl Pts',(22.7817704456175,-10.8543372932887,-2.13286375196528));
#38384=CARTESIAN_POINT('Ctrl Pts',(23.3296603631195,-10.8753724962822,-2.03163991938108));
#38385=CARTESIAN_POINT('Ctrl Pts',(23.4469280425869,-10.8796667005723,-2.01025391532517));
#38386=CARTESIAN_POINT('Ctrl Pts',(23.6810288813553,-10.8878000542956,-1.96865773783264));
#38387=CARTESIAN_POINT('Ctrl Pts',(24.0941214149603,-10.9009272596696,-1.89824222375216));
#38388=CARTESIAN_POINT('Ctrl Pts',(24.6899984645715,-10.9167861221079,-1.80575737992305));
#38389=CARTESIAN_POINT('Ctrl Pts',(25.4117472347965,-10.9320835607493,-1.71023812556292));
#38390=CARTESIAN_POINT('Ctrl Pts',(25.8944359856997,-10.9403877892627,-1.65861072075244));
#38391=CARTESIAN_POINT('Ctrl Pts',(26.3669426319602,-10.9478841337461,-1.61476081138877));
#38392=CARTESIAN_POINT('Ctrl Pts',(27.2927605647398,-10.9593568588012,-1.54499465236548));
#38393=CARTESIAN_POINT('Ctrl Pts',(28.2852623623168,-10.9616475307267,-1.51981821556059));
#38394=CARTESIAN_POINT('Ctrl Pts',(29.2044123671999,-10.9652006081482,-1.49506529955051));
#38395=CARTESIAN_POINT('Ctrl Pts',(29.5205491106405,-10.9661656603817,-1.48868169066078));
#38396=CARTESIAN_POINT('Ctrl Pts',(30.1691034959588,-10.9670510696507,-1.48263221141176));
#38397=CARTESIAN_POINT('Ctrl Pts',(31.3134334344234,-10.9664912432219,-1.4864605825931));
#38398=CARTESIAN_POINT('Ctrl Pts',(32.3203424123247,-10.9645690748214,-1.49997009105206));
#38399=CARTESIAN_POINT('Ctrl Pts',(33.1675465322482,-10.9645713457497,-1.49998069520818));
#38400=CARTESIAN_POINT('Ctrl Pts',(33.4947519346945,-10.9645717110255,-1.49998093738942));
#38401=CARTESIAN_POINT('Ctrl Pts',(34.1540738134336,-10.9645721532421,-1.49998231763443));
#38402=CARTESIAN_POINT('Ctrl Pts',(34.81145110075,-10.9645737361772,-1.499985805429));
#38403=CARTESIAN_POINT('Ctrl Pts',(35.7991041415374,-10.9645740230236,-1.49998654292927));
#38404=CARTESIAN_POINT('Ctrl Pts',(37.7734954411133,-10.9645758157224,-1.49999064614178));
#38405=CARTESIAN_POINT('Ctrl Pts',(39.5833333333333,-10.9645797934319,-1.5));
#38406=CARTESIAN_POINT('Ctrl Pts',(40.9,-10.9645797934319,-1.5));
#38407=CARTESIAN_POINT('Ctrl Pts',(6.63336813585096,-9.34202246898051,-11.0008793183436));
#38408=CARTESIAN_POINT('Ctrl Pts',(7.389696336477,-9.9106502389341,-10.5126404716241));
#38409=CARTESIAN_POINT('Ctrl Pts',(8.18028889045472,-10.4323217834721,-10.0000669136624));
#38410=CARTESIAN_POINT('Ctrl Pts',(9.94159575574686,-11.439192222287,-8.85353468669098));
#38411=CARTESIAN_POINT('Ctrl Pts',(10.9109419422818,-11.9102705993651,-8.19201021037899));
#38412=CARTESIAN_POINT('Ctrl Pts',(12.8335218625484,-12.6683977976686,-6.98387303125937));
#38413=CARTESIAN_POINT('Ctrl Pts',(13.8091851210584,-12.9798296118147,-6.36343771133683));
#38414=CARTESIAN_POINT('Ctrl Pts',(15.0310774900381,-13.2915570052696,-5.67481209887734));
#38415=CARTESIAN_POINT('Ctrl Pts',(15.9749773134882,-13.5160612446606,-5.14536755152679));
#38416=CARTESIAN_POINT('Ctrl Pts',(16.930312943506,-13.6911692618857,-4.63930769376668));
#38417=CARTESIAN_POINT('Ctrl Pts',(18.5806860927912,-13.9445588072223,-3.86175938608204));
#38418=CARTESIAN_POINT('Ctrl Pts',(19.548719041905,-14.047648520923,-3.43185831734755));
#38419=CARTESIAN_POINT('Ctrl Pts',(20.9744115808253,-14.1690991173097,-2.91639691217872));
#38420=CARTESIAN_POINT('Ctrl Pts',(21.9189583606346,-14.2328177454448,-2.59280390983887));
#38421=CARTESIAN_POINT('Ctrl Pts',(22.8721113115929,-14.2778669302766,-2.32284159836073));
#38422=CARTESIAN_POINT('Ctrl Pts',(23.4111206282029,-14.300719458499,-2.1913240624154));
#38423=CARTESIAN_POINT('Ctrl Pts',(23.5272640974129,-14.3053783578071,-2.16340494095905));
#38424=CARTESIAN_POINT('Ctrl Pts',(23.7586042074435,-14.3141392731538,-2.10919630050476));
#38425=CARTESIAN_POINT('Ctrl Pts',(24.1668594457504,-14.3281409258012,-2.01743796447889));
#38426=CARTESIAN_POINT('Ctrl Pts',(24.7549510427126,-14.3447231768686,-1.89707890772754));
#38427=CARTESIAN_POINT('Ctrl Pts',(25.4661619742724,-14.3604369110458,-1.77296928480105));
#38428=CARTESIAN_POINT('Ctrl Pts',(25.940793652308,-14.3689791856741,-1.7060154102986));
#38429=CARTESIAN_POINT('Ctrl Pts',(26.4047985025956,-14.3768131131953,-1.64920950338615));
#38430=CARTESIAN_POINT('Ctrl Pts',(27.3109130873601,-14.3886741790609,-1.55899536298034));
#38431=CARTESIAN_POINT('Ctrl Pts',(28.2968127703991,-14.3906288624532,-1.52586579774316));
#38432=CARTESIAN_POINT('Ctrl Pts',(29.216365869052,-14.3942351181099,-1.49337715415662));
#38433=CARTESIAN_POINT('Ctrl Pts',(29.5273677411776,-14.3952146919186,-1.48510498656914));
#38434=CARTESIAN_POINT('Ctrl Pts',(30.1704748351474,-14.3961140069303,-1.47720108681953));
#38435=CARTESIAN_POINT('Ctrl Pts',(31.3076822233502,-14.3955480332033,-1.48219673215098));
#38436=CARTESIAN_POINT('Ctrl Pts',(32.3162781940781,-14.3936026936296,-1.49994928257769));
#38437=CARTESIAN_POINT('Ctrl Pts',(33.1684720644413,-14.3936066618446,-1.49996698297726));
#38438=CARTESIAN_POINT('Ctrl Pts',(33.4950641584122,-14.3936073001223,-1.49996744488463));
#38439=CARTESIAN_POINT('Ctrl Pts',(34.1546952525893,-14.3936080728485,-1.49996977575843));
#38440=CARTESIAN_POINT('Ctrl Pts',(34.811773768313,-14.3936108388537,-1.49997575137036));
#38441=CARTESIAN_POINT('Ctrl Pts',(35.7994747102212,-14.3936113400865,-1.49997700611746));
#38442=CARTESIAN_POINT('Ctrl Pts',(37.7736758948774,-14.3936144726314,-1.499984023326));
#38443=CARTESIAN_POINT('Ctrl Pts',(39.5833333333333,-14.3936214232436,-1.5));
#38444=CARTESIAN_POINT('Ctrl Pts',(40.9,-14.3936214232436,-1.5));
#38445=CARTESIAN_POINT('Ctrl Pts',(6.84643360079894,-15.1545575883324,-16.506001665025));
#38446=CARTESIAN_POINT('Ctrl Pts',(7.61273218496772,-16.0159127642118,-15.7040687667121));
#38447=CARTESIAN_POINT('Ctrl Pts',(8.4126771054426,-16.7980113101253,-14.8690272591124));
#38448=CARTESIAN_POINT('Ctrl Pts',(10.1879439641556,-18.2945580567154,-13.0164926384401));
#38449=CARTESIAN_POINT('Ctrl Pts',(11.1642689802371,-18.9856854823124,-11.9550510602025));
#38450=CARTESIAN_POINT('Ctrl Pts',(13.1036036726265,-20.0861315198186,-10.022452207883));
#38451=CARTESIAN_POINT('Ctrl Pts',(14.0826172183607,-20.5290484396469,-9.03879487952599));
#38452=CARTESIAN_POINT('Ctrl Pts',(15.3089235211201,-20.9656035967448,-7.95158583831005));
#38453=CARTESIAN_POINT('Ctrl Pts',(16.2536562498252,-21.279069264144,-7.11690983506512));
#38454=CARTESIAN_POINT('Ctrl Pts',(17.2094234535123,-21.5156901422925,-6.32372298857519));
#38455=CARTESIAN_POINT('Ctrl Pts',(18.8492103514785,-21.8541559656567,-5.11428176787038));
#38456=CARTESIAN_POINT('Ctrl Pts',(19.8132789859546,-21.9855288021884,-4.44555314736778));
#38457=CARTESIAN_POINT('Ctrl Pts',(21.2105274130183,-22.1378650260475,-3.65671370764623));
#38458=CARTESIAN_POINT('Ctrl Pts',(22.1435262947165,-22.2155499994866,-3.15760868632205));
#38459=CARTESIAN_POINT('Ctrl Pts',(23.0712019161591,-22.2672966100825,-2.74759983583376));
#38460=CARTESIAN_POINT('Ctrl Pts',(23.5926643019347,-22.2940508574536,-2.54861011877026));
#38461=CARTESIAN_POINT('Ctrl Pts',(23.7065967589747,-22.2995097248263,-2.50584172092975));
#38462=CARTESIAN_POINT('Ctrl Pts',(23.9324349207315,-22.3096292230893,-2.42316535684894));
#38463=CARTESIAN_POINT('Ctrl Pts',(24.3308966188196,-22.3255066595418,-2.28324508302851));
#38464=CARTESIAN_POINT('Ctrl Pts',(24.9027307486989,-22.3435822260678,-2.10031694390082));
#38465=CARTESIAN_POINT('Ctrl Pts',(25.5912058020402,-22.3601136597686,-1.91242242103885));
#38466=CARTESIAN_POINT('Ctrl Pts',(26.0479116166522,-22.3691489781576,-1.81155274261716));
#38467=CARTESIAN_POINT('Ctrl Pts',(26.4927766852066,-22.3777261422415,-1.72621142470537));
#38468=CARTESIAN_POINT('Ctrl Pts',(27.3538144829414,-22.3904445374985,-1.59133675559696));
#38469=CARTESIAN_POINT('Ctrl Pts',(28.3239440765631,-22.3916143651133,-1.5395372712982));
#38470=CARTESIAN_POINT('Ctrl Pts',(29.2444087331683,-22.3953365265065,-1.48903537353034));
#38471=CARTESIAN_POINT('Ctrl Pts',(29.5434413064006,-22.3963491807022,-1.4765958448865));
#38472=CARTESIAN_POINT('Ctrl Pts',(30.1738228526165,-22.3972793088217,-1.46445321166482));
#38473=CARTESIAN_POINT('Ctrl Pts',(31.2943937060125,-22.3966964278384,-1.47211763918551));
#38474=CARTESIAN_POINT('Ctrl Pts',(32.3068807810285,-22.394691709999,-1.49983279134388));
#38475=CARTESIAN_POINT('Ctrl Pts',(33.1706991860564,-22.3946974029307,-1.49988437406509));
#38476=CARTESIAN_POINT('Ctrl Pts',(33.495857312607,-22.3946983171245,-1.49988713027318));
#38477=CARTESIAN_POINT('Ctrl Pts',(34.1562063695874,-22.394699425001,-1.49989458266054));
#38478=CARTESIAN_POINT('Ctrl Pts',(34.8125750960603,-22.3947033892012,-1.49991575825724));
#38479=CARTESIAN_POINT('Ctrl Pts',(35.8003855127833,-22.3947041076693,-1.49991999484082));
#38480=CARTESIAN_POINT('Ctrl Pts',(37.7741287617181,-22.394708597346,-1.49994455667285));
#38481=CARTESIAN_POINT('Ctrl Pts',(39.5833333333333,-22.394718559471,-1.5));
#38482=CARTESIAN_POINT('Ctrl Pts',(40.9,-22.394718559471,-1.5));
#38483=CARTESIAN_POINT('Ctrl Pts',(6.90857970435319,-20.8698550272217,-22.1068727166734));
#38484=CARTESIAN_POINT('Ctrl Pts',(7.67983757144493,-22.0336104135999,-20.991774688754));
#38485=CARTESIAN_POINT('Ctrl Pts',(8.48444928201916,-23.0860770683301,-19.8332461961107));
#38486=CARTESIAN_POINT('Ctrl Pts',(10.2687663769551,-25.0905346149111,-17.2709888357559));
#38487=CARTESIAN_POINT('Ctrl Pts',(11.2490111943913,-26.0108786577409,-15.8072894822424));
#38488=CARTESIAN_POINT('Ctrl Pts',(13.2067599054631,-27.4745835397,-13.1283892637642));
#38489=CARTESIAN_POINT('Ctrl Pts',(14.1887708824687,-28.0545611646472,-11.7775873547894));
#38490=CARTESIAN_POINT('Ctrl Pts',(15.4301927253883,-28.6258871350548,-10.2708149751555));
#38491=CARTESIAN_POINT('Ctrl Pts',(16.3793034376203,-29.0320485193235,-9.12509880827948));
#38492=CARTESIAN_POINT('Ctrl Pts',(17.3459407209746,-29.335531334809,-8.0290538541365));
#38493=CARTESIAN_POINT('Ctrl Pts',(19.0016786397101,-29.764530122403,-6.36442803225958));
#38494=CARTESIAN_POINT('Ctrl Pts',(19.9708024570658,-29.9249381814107,-5.44984750618438));
#38495=CARTESIAN_POINT('Ctrl Pts',(21.3726541621532,-30.1088343166975,-4.37628680649797));
#38496=CARTESIAN_POINT('Ctrl Pts',(22.305997327355,-30.2002109026539,-3.69883691082954));
#38497=CARTESIAN_POINT('Ctrl Pts',(23.2278577930096,-30.2581794306256,-3.14826448808768));
#38498=CARTESIAN_POINT('Ctrl Pts',(23.7415516356673,-30.2885183156943,-2.88362049576681));
#38499=CARTESIAN_POINT('Ctrl Pts',(23.8544946510481,-30.2947200062415,-2.82623659223923));
#38500=CARTESIAN_POINT('Ctrl Pts',(24.0777274663499,-30.3060802342181,-2.71573667925153));
#38501=CARTESIAN_POINT('Ctrl Pts',(24.4711727956187,-30.32363513723,-2.52895535356898));
#38502=CARTESIAN_POINT('Ctrl Pts',(25.0334457271175,-30.3429441514165,-2.28601411482693));
#38503=CARTESIAN_POINT('Ctrl Pts',(25.706214488466,-30.3600503901637,-2.03835403030808));
#38504=CARTESIAN_POINT('Ctrl Pts',(26.1486936133439,-30.3694723684124,-1.90670660027133));
#38505=CARTESIAN_POINT('Ctrl Pts',(26.5774366289031,-30.3787139799022,-1.79594947825408));
#38506=CARTESIAN_POINT('Ctrl Pts',(27.3975110717084,-30.392198133447,-1.62272694197858));
#38507=CARTESIAN_POINT('Ctrl Pts',(28.3508259392473,-30.3926064111246,-1.55227638555955));
#38508=CARTESIAN_POINT('Ctrl Pts',(29.2723062856311,-30.3964396342324,-1.48380439950634));
#38509=CARTESIAN_POINT('Ctrl Pts',(29.5594622066961,-30.3974855836748,-1.46775103384065));
#38510=CARTESIAN_POINT('Ctrl Pts',(30.1771168569175,-30.3984465770315,-1.45157152773897));
#38511=CARTESIAN_POINT('Ctrl Pts',(31.281071177308,-30.3978463334884,-1.46177125475314));
#38512=CARTESIAN_POINT('Ctrl Pts',(32.297455993961,-30.3957818406259,-1.49958178095819));
#38513=CARTESIAN_POINT('Ctrl Pts',(33.1729044426911,-30.395789026338,-1.49970257782127));
#38514=CARTESIAN_POINT('Ctrl Pts',(33.4966295876142,-30.3957901777219,-1.4997109685702));
#38515=CARTESIAN_POINT('Ctrl Pts',(34.1576977268014,-30.3957915749198,-1.49972932651149));
#38516=CARTESIAN_POINT('Ctrl Pts',(34.813360769929,-30.3957965718591,-1.4997840805116));
#38517=CARTESIAN_POINT('Ctrl Pts',(35.8012813983216,-30.3957974776821,-1.49979479816102));
#38518=CARTESIAN_POINT('Ctrl Pts',(37.7745713511015,-30.395803137258,-1.49985796376524));
#38519=CARTESIAN_POINT('Ctrl Pts',(39.5833333333333,-30.3958156956984,-1.5));
#38520=CARTESIAN_POINT('Ctrl Pts',(40.9,-30.3958156956984,-1.5));
#38521=CARTESIAN_POINT('Ctrl Pts',(6.93528330520032,-24.1234099037007,-25.3195110382618));
#38522=CARTESIAN_POINT('Ctrl Pts',(7.70864561497005,-25.4600205488393,-24.0266258397084));
#38523=CARTESIAN_POINT('Ctrl Pts',(8.51531156164573,-26.6675788409114,-22.6840056101462));
#38524=CARTESIAN_POINT('Ctrl Pts',(10.3033767345502,-28.9634999585434,-19.7178334181139));
#38525=CARTESIAN_POINT('Ctrl Pts',(11.2853975328499,-30.0157138764656,-18.024966824446));
#38526=CARTESIAN_POINT('Ctrl Pts',(13.2504656206425,-31.6887121402305,-14.920608256729));
#38527=CARTESIAN_POINT('Ctrl Pts',(14.2338911783743,-32.3479754973602,-13.360326515741));
#38528=CARTESIAN_POINT('Ctrl Pts',(15.4814489736579,-32.9977120049688,-11.6128587845954));
#38529=CARTESIAN_POINT('Ctrl Pts',(16.4323633322631,-33.457701559807,-10.2891584164032));
#38530=CARTESIAN_POINT('Ctrl Pts',(17.4036580739675,-33.8004278805126,-9.0188416170732));
#38531=CARTESIAN_POINT('Ctrl Pts',(19.0672887678302,-34.2828730898379,-7.09001985912387));
#38532=CARTESIAN_POINT('Ctrl Pts',(20.0391149919151,-34.4604737318843,-6.03348815316117));
#38533=CARTESIAN_POINT('Ctrl Pts',(21.4462778487112,-34.6632929668281,-4.79159535501523));
#38534=CARTESIAN_POINT('Ctrl Pts',(22.3811728101678,-34.7627792680187,-4.01020122074909));
#38535=CARTESIAN_POINT('Ctrl Pts',(23.3032595484893,-34.8244923190156,-3.37635643636738));
#38536=CARTESIAN_POINT('Ctrl Pts',(23.8149974822583,-34.8569118346709,-3.07312481135076));
#38537=CARTESIAN_POINT('Ctrl Pts',(23.9276845297173,-34.8635414236987,-3.00725282827683));
#38538=CARTESIAN_POINT('Ctrl Pts',(24.1501932465709,-34.8756163196444,-2.88055633977638));
#38539=CARTESIAN_POINT('Ctrl Pts',(24.5421106234083,-34.8941314993696,-2.66656979475214));
#38540=CARTESIAN_POINT('Ctrl Pts',(25.1010166003946,-34.9141289755492,-2.38896069563579));
#38541=CARTESIAN_POINT('Ctrl Pts',(25.7673676623321,-34.9315307898229,-2.10719515267299));
#38542=CARTESIAN_POINT('Ctrl Pts',(26.2032614590243,-34.9411502230501,-1.95837832513291));
#38543=CARTESIAN_POINT('Ctrl Pts',(26.6241220770206,-34.9507523611205,-1.83365744353249));
#38544=CARTESIAN_POINT('Ctrl Pts',(27.4227877709103,-34.9646463474546,-1.64008822157604));
#38545=CARTESIAN_POINT('Ctrl Pts',(28.3660425122777,-34.9646178111257,-1.55920845841384));
#38546=CARTESIAN_POINT('Ctrl Pts',(29.288154079426,-34.9685099768711,-1.48047877405357));
#38547=CARTESIAN_POINT('Ctrl Pts',(29.5685743108623,-34.9695745039167,-1.46254110097229));
#38548=CARTESIAN_POINT('Ctrl Pts',(30.1789566228709,-34.9705522790041,-1.44412472938078));
#38549=CARTESIAN_POINT('Ctrl Pts',(31.273428633048,-34.9699406754865,-1.45573528147979));
#38550=CARTESIAN_POINT('Ctrl Pts',(32.2920480078111,-34.9678391394653,-1.49937027232428));
#38551=CARTESIAN_POINT('Ctrl Pts',(33.1741467941405,-34.9678459524317,-1.4995472544355));
#38552=CARTESIAN_POINT('Ctrl Pts',(33.4970538821705,-34.9678470414555,-1.49956078207587));
#38553=CARTESIAN_POINT('Ctrl Pts',(34.1585338443542,-34.9678483649439,-1.49958825610693));
#38554=CARTESIAN_POINT('Ctrl Pts',(34.8137969787743,-34.9678530956496,-1.49967176946748));
#38555=CARTESIAN_POINT('Ctrl Pts',(35.8017811867034,-34.9678539534013,-1.49968797974803));
#38556=CARTESIAN_POINT('Ctrl Pts',(37.7748158892396,-34.9678593117153,-1.49978412416472));
#38557=CARTESIAN_POINT('Ctrl Pts',(39.5833333333333,-34.967871202114,-1.5));
#38558=CARTESIAN_POINT('Ctrl Pts',(40.9,-34.967871202114,-1.5));
#38559=CARTESIAN_POINT('Origin',(6.9,-25.9807621135332,15.));
#38560=CARTESIAN_POINT('',(6.9,-28.7358750109634,-8.61681422303452));
#38561=CARTESIAN_POINT('Ctrl Pts',(6.9,-10.3676856018661,-3.76156693666918));
#38562=CARTESIAN_POINT('Ctrl Pts',(6.9,-14.103554168739,-4.66834435251375));
#38563=CARTESIAN_POINT('Ctrl Pts',(6.90000000166257,-18.0191477848531,-5.7030525211077));
#38564=CARTESIAN_POINT('Ctrl Pts',(6.90000000166257,-23.666490663791,-7.22296038005705));
#38565=CARTESIAN_POINT('Ctrl Pts',(6.9,-26.2182182108371,-7.92134750786925));
#38566=CARTESIAN_POINT('Ctrl Pts',(6.9,-28.7358750109634,-8.61681422303452));
#38567=CARTESIAN_POINT('Origin',(6.9,0.,0.));
#38568=CARTESIAN_POINT('Origin',(40.9,-7.79422863405995,4.5));
#38569=CARTESIAN_POINT('Ctrl Pts',(40.9,-30.5996231131986,15.9346498339374));
#38570=CARTESIAN_POINT('Ctrl Pts',(40.9,-30.1661818974695,15.6844024313584));
#38571=CARTESIAN_POINT('Ctrl Pts',(40.9,-29.7327406817405,15.4341550287793));
#38572=CARTESIAN_POINT('Ctrl Pts',(40.9,-29.2992994660114,15.1839076262003));
#38573=CARTESIAN_POINT('Ctrl Pts',(30.5,-29.5001797522422,18.8345266621011));
#38574=CARTESIAN_POINT('Ctrl Pts',(30.5,-29.9204226682664,18.176307754627));
#38575=CARTESIAN_POINT('Ctrl Pts',(30.5,-30.3108891324553,17.5));
#38576=CARTESIAN_POINT('Ctrl Pts',(30.5,-47.8108891324553,-12.8108891324553));
#38577=CARTESIAN_POINT('Ctrl Pts',(30.5,-17.5,-30.3108891324553));
#38578=CARTESIAN_POINT('Ctrl Pts',(30.5,12.8108891324553,-47.8108891324553));
#38579=CARTESIAN_POINT('Ctrl Pts',(30.5,30.3108891324553,-17.5));
#38580=CARTESIAN_POINT('Ctrl Pts',(30.5,47.8108891324553,12.8108891324553));
#38581=CARTESIAN_POINT('Ctrl Pts',(30.5,17.5,30.3108891324553));
#38582=CARTESIAN_POINT('Ctrl Pts',(30.5,-11.4877949884694,47.0470003722618));
#38583=CARTESIAN_POINT('Ctrl Pts',(30.5,-29.5001797522422,18.8345266621011));
#38584=CARTESIAN_POINT('Ctrl Pts',(30.3311478274255,-29.4365936489566,18.7939298193791));
#38585=CARTESIAN_POINT('Ctrl Pts',(30.3311478274255,-29.8559307532302,18.1371296685291));
#38586=CARTESIAN_POINT('Ctrl Pts',(30.3311478274255,-30.245555587262,17.4622796600955));
#38587=CARTESIAN_POINT('Ctrl Pts',(30.3311478274255,-47.7078352473574,-12.7832759271665));
#38588=CARTESIAN_POINT('Ctrl Pts',(30.3311478274255,-17.4622796600955,-30.245555587262));
#38589=CARTESIAN_POINT('Ctrl Pts',(30.3311478274255,12.7832759271665,-47.7078352473574));
#38590=CARTESIAN_POINT('Ctrl Pts',(30.3311478274255,30.245555587262,-17.4622796600955));
#38591=CARTESIAN_POINT('Ctrl Pts',(30.3311478274255,47.7078352473574,12.7832759271665));
#38592=CARTESIAN_POINT('Ctrl Pts',(30.3311478274255,17.4622796600955,30.245555587262));
#38593=CARTESIAN_POINT('Ctrl Pts',(30.3311478274255,-11.4630336437997,46.9455930096601));
#38594=CARTESIAN_POINT('Ctrl Pts',(30.3311478274255,-29.4365936489566,18.7939298193791));
#38595=CARTESIAN_POINT('Ctrl Pts',(29.9897712690917,-29.3077924996107,18.7116961278613));
#38596=CARTESIAN_POINT('Ctrl Pts',(29.9897712690917,-29.7252947753835,18.0577698358324));
#38597=CARTESIAN_POINT('Ctrl Pts',(29.9897712690917,-30.1132147882992,17.3858726641896));
#38598=CARTESIAN_POINT('Ctrl Pts',(29.9897712690917,-47.4990874524888,-12.7273421241096));
#38599=CARTESIAN_POINT('Ctrl Pts',(29.9897712690917,-17.3858726641896,-30.1132147882992));
#38600=CARTESIAN_POINT('Ctrl Pts',(29.9897712690917,12.7273421241096,-47.4990874524888));
#38601=CARTESIAN_POINT('Ctrl Pts',(29.9897712690917,30.1132147882992,-17.3858726641896));
#38602=CARTESIAN_POINT('Ctrl Pts',(29.9897712690917,47.4990874524888,12.7273421241096));
#38603=CARTESIAN_POINT('Ctrl Pts',(29.9897712690917,17.3858726641896,30.1132147882992));
#38604=CARTESIAN_POINT('Ctrl Pts',(29.9897712690917,-11.4128766206768,46.7401804402414));
#38605=CARTESIAN_POINT('Ctrl Pts',(29.9897712690917,-29.3077924996107,18.7116961278613));
#38606=CARTESIAN_POINT('Ctrl Pts',(29.4666899049319,-29.1097034403905,18.5852252487451));
#38607=CARTESIAN_POINT('Ctrl Pts',(29.4666899049319,-29.5243838511923,17.935718792976));
#38608=CARTESIAN_POINT('Ctrl Pts',(29.4666899049319,-29.9096819433198,17.2683629213518));
#38609=CARTESIAN_POINT('Ctrl Pts',(29.4666899049319,-47.1780448646716,-12.641319021968));
#38610=CARTESIAN_POINT('Ctrl Pts',(29.4666899049319,-17.2683629213518,-29.9096819433198));
#38611=CARTESIAN_POINT('Ctrl Pts',(29.4666899049319,12.641319021968,-47.1780448646716));
#38612=CARTESIAN_POINT('Ctrl Pts',(29.4666899049319,29.9096819433198,-17.2683629213518));
#38613=CARTESIAN_POINT('Ctrl Pts',(29.4666899049319,47.1780448646716,12.641319021968));
#38614=CARTESIAN_POINT('Ctrl Pts',(29.4666899049319,17.2683629213518,29.9096819433198));
#38615=CARTESIAN_POINT('Ctrl Pts',(29.4666899049319,-11.3357378872557,46.4242672450966));
#38616=CARTESIAN_POINT('Ctrl Pts',(29.4666899049319,-29.1097034403905,18.5852252487451));
#38617=CARTESIAN_POINT('Ctrl Pts',(28.7471241621752,-28.8357745030392,18.4103340474916));
#38618=CARTESIAN_POINT('Ctrl Pts',(28.7471241621752,-29.246552676757,17.7669395953572));
#38619=CARTESIAN_POINT('Ctrl Pts',(28.7471241621752,-29.6282250261092,17.105863694435));
#38620=CARTESIAN_POINT('Ctrl Pts',(28.7471241621752,-46.7340887205442,-12.5223613316742));
#38621=CARTESIAN_POINT('Ctrl Pts',(28.7471241621752,-17.105863694435,-29.6282250261092));
#38622=CARTESIAN_POINT('Ctrl Pts',(28.7471241621752,12.5223613316742,-46.7340887205442));
#38623=CARTESIAN_POINT('Ctrl Pts',(28.7471241621752,29.6282250261092,-17.105863694435));
#38624=CARTESIAN_POINT('Ctrl Pts',(28.7471241621752,46.7340887205442,12.5223613316742));
#38625=CARTESIAN_POINT('Ctrl Pts',(28.7471241621752,17.105863694435,29.6282250261092));
#38626=CARTESIAN_POINT('Ctrl Pts',(28.7471241621752,-11.2290660127069,45.9874043199967));
#38627=CARTESIAN_POINT('Ctrl Pts',(28.7471241621752,-28.8357745030392,18.4103340474916));
#38628=CARTESIAN_POINT('Ctrl Pts',(27.8100958442934,-28.4776836217162,18.1817092625453));
#38629=CARTESIAN_POINT('Ctrl Pts',(27.8100958442934,-28.8833606347823,17.5463046664274));
#38630=CARTESIAN_POINT('Ctrl Pts',(27.8100958442934,-29.2602932679205,16.8934381948013));
#38631=CARTESIAN_POINT('Ctrl Pts',(27.8100958442934,-46.1537314627218,-12.3668550731192));
#38632=CARTESIAN_POINT('Ctrl Pts',(27.8100958442934,-16.8934381948013,-29.2602932679205));
#38633=CARTESIAN_POINT('Ctrl Pts',(27.8100958442934,12.3668550731192,-46.1537314627218));
#38634=CARTESIAN_POINT('Ctrl Pts',(27.8100958442934,29.2602932679205,-16.8934381948013));
#38635=CARTESIAN_POINT('Ctrl Pts',(27.8100958442934,46.1537314627218,12.3668550731192));
#38636=CARTESIAN_POINT('Ctrl Pts',(27.8100958442934,16.8934381948013,29.2602932679205));
#38637=CARTESIAN_POINT('Ctrl Pts',(27.8100958442934,-11.0896202647003,45.4163196022628));
#38638=CARTESIAN_POINT('Ctrl Pts',(27.8100958442934,-28.4776836217162,18.1817092625453));
#38639=CARTESIAN_POINT('Ctrl Pts',(26.8343111708818,-28.1064299010669,17.9446806017473));
#38640=CARTESIAN_POINT('Ctrl Pts',(26.8343111708818,-28.5068182430991,17.3175595557791));
#38641=CARTESIAN_POINT('Ctrl Pts',(26.8343111708818,-28.8788369357517,16.6732042787396));
#38642=CARTESIAN_POINT('Ctrl Pts',(26.8343111708818,-45.5520412144912,-12.2056326570121));
#38643=CARTESIAN_POINT('Ctrl Pts',(26.8343111708818,-16.6732042787396,-28.8788369357517));
#38644=CARTESIAN_POINT('Ctrl Pts',(26.8343111708818,12.2056326570121,-45.5520412144912));
#38645=CARTESIAN_POINT('Ctrl Pts',(26.8343111708818,28.8788369357517,-16.6732042787396));
#38646=CARTESIAN_POINT('Ctrl Pts',(26.8343111708818,45.5520412144912,12.2056326570121));
#38647=CARTESIAN_POINT('Ctrl Pts',(26.8343111708818,16.6732042787396,28.8788369357517));
#38648=CARTESIAN_POINT('Ctrl Pts',(26.8343111708818,-10.9450487174303,44.8242427376375));
#38649=CARTESIAN_POINT('Ctrl Pts',(26.8343111708818,-28.1064299010669,17.9446806017473));
#38650=CARTESIAN_POINT('Ctrl Pts',(25.8181479469611,-27.7272550606068,17.7025946652472));
#38651=CARTESIAN_POINT('Ctrl Pts',(25.8181479469611,-28.1222418918016,17.0839339083798));
#38652=CARTESIAN_POINT('Ctrl Pts',(25.8181479469611,-28.4892417994668,16.4482714219305));
#38653=CARTESIAN_POINT('Ctrl Pts',(25.8181479469611,-44.9375132213974,-12.0409703775363));
#38654=CARTESIAN_POINT('Ctrl Pts',(25.8181479469611,-16.4482714219305,-28.4892417994668));
#38655=CARTESIAN_POINT('Ctrl Pts',(25.8181479469611,12.0409703775363,-44.9375132213974));
#38656=CARTESIAN_POINT('Ctrl Pts',(25.8181479469611,28.4892417994668,-16.4482714219305));
#38657=CARTESIAN_POINT('Ctrl Pts',(25.8181479469611,44.9375132213974,12.0409703775363));
#38658=CARTESIAN_POINT('Ctrl Pts',(25.8181479469611,16.4482714219305,28.4892417994668));
#38659=CARTESIAN_POINT('Ctrl Pts',(25.8181479469611,-10.7973925719907,44.2195332406074));
#38660=CARTESIAN_POINT('Ctrl Pts',(25.8181479469611,-27.7272550606068,17.7025946652472));
#38661=CARTESIAN_POINT('Ctrl Pts',(24.7595197917227,-27.3496265541183,17.4614959928472));
#38662=CARTESIAN_POINT('Ctrl Pts',(24.7595197917227,-27.739233902677,16.8512610227058));
#38663=CARTESIAN_POINT('Ctrl Pts',(24.7595197917227,-28.1012354927406,16.2242558762949));
#38664=CARTESIAN_POINT('Ctrl Pts',(24.7595197917227,-44.3254913690355,-11.8769796164457));
#38665=CARTESIAN_POINT('Ctrl Pts',(24.7595197917227,-16.2242558762949,-28.1012354927406));
#38666=CARTESIAN_POINT('Ctrl Pts',(24.7595197917227,11.8769796164457,-44.3254913690355));
#38667=CARTESIAN_POINT('Ctrl Pts',(24.7595197917227,28.1012354927406,-16.2242558762949));
#38668=CARTESIAN_POINT('Ctrl Pts',(24.7595197917227,44.3254913690355,11.8769796164457));
#38669=CARTESIAN_POINT('Ctrl Pts',(24.7595197917227,16.2242558762949,28.1012354927406));
#38670=CARTESIAN_POINT('Ctrl Pts',(24.7595197917227,-10.6503385912768,43.6172898429552));
#38671=CARTESIAN_POINT('Ctrl Pts',(24.7595197917227,-27.3496265541183,17.4614959928472));
#38672=CARTESIAN_POINT('Ctrl Pts',(23.6563574780851,-26.9860278023044,17.229354682426));
#38673=CARTESIAN_POINT('Ctrl Pts',(23.6563574780851,-27.370455528196,16.627232461942));
#38674=CARTESIAN_POINT('Ctrl Pts',(23.6563574780851,-27.7276444994825,16.0085630157705));
#38675=CARTESIAN_POINT('Ctrl Pts',(23.6563574780851,-43.736207515253,-11.719081483712));
#38676=CARTESIAN_POINT('Ctrl Pts',(23.6563574780851,-16.0085630157705,-27.7276444994825));
#38677=CARTESIAN_POINT('Ctrl Pts',(23.6563574780851,11.719081483712,-43.736207515253));
#38678=CARTESIAN_POINT('Ctrl Pts',(23.6563574780851,27.7276444994825,-16.0085630157705));
#38679=CARTESIAN_POINT('Ctrl Pts',(23.6563574780851,43.736207515253,11.719081483712));
#38680=CARTESIAN_POINT('Ctrl Pts',(23.6563574780851,16.0085630157705,27.7276444994825));
#38681=CARTESIAN_POINT('Ctrl Pts',(23.6563574780851,-10.5087479991522,43.0374211521332));
#38682=CARTESIAN_POINT('Ctrl Pts',(23.6563574780851,-26.9860278023044,17.229354682426));
#38683=CARTESIAN_POINT('Ctrl Pts',(22.5073180101405,-26.649565639321,17.0145388530744));
#38684=CARTESIAN_POINT('Ctrl Pts',(22.5073180101405,-27.029200315079,16.419923900654));
#38685=CARTESIAN_POINT('Ctrl Pts',(22.5073180101405,-27.3819358493961,15.8089680335819));
#38686=CARTESIAN_POINT('Ctrl Pts',(22.5073180101405,-43.190903882978,-11.5729678158142));
#38687=CARTESIAN_POINT('Ctrl Pts',(22.5073180101405,-15.8089680335819,-27.3819358493961));
#38688=CARTESIAN_POINT('Ctrl Pts',(22.5073180101405,11.5729678158142,-43.190903882978));
#38689=CARTESIAN_POINT('Ctrl Pts',(22.5073180101405,27.3819358493961,-15.8089680335819));
#38690=CARTESIAN_POINT('Ctrl Pts',(22.5073180101405,43.190903882978,11.5729678158142));
#38691=CARTESIAN_POINT('Ctrl Pts',(22.5073180101405,15.8089680335819,27.3819358493961));
#38692=CARTESIAN_POINT('Ctrl Pts',(22.5073180101405,-10.3777247856603,42.5008299977716));
#38693=CARTESIAN_POINT('Ctrl Pts',(22.5073180101405,-26.649565639321,17.0145388530744));
#38694=CARTESIAN_POINT('Ctrl Pts',(21.3125219557939,-26.3518679613905,16.8244723890963));
#38695=CARTESIAN_POINT('Ctrl Pts',(21.3125219557939,-26.727261803997,16.2364997772301));
#38696=CARTESIAN_POINT('Ctrl Pts',(21.3125219557939,-27.0760569908086,15.632368792237));
#38697=CARTESIAN_POINT('Ctrl Pts',(21.3125219557939,-42.7084257830456,-11.4436881985716));
#38698=CARTESIAN_POINT('Ctrl Pts',(21.3125219557939,-15.632368792237,-27.0760569908086));
#38699=CARTESIAN_POINT('Ctrl Pts',(21.3125219557939,11.4436881985716,-42.7084257830456));
#38700=CARTESIAN_POINT('Ctrl Pts',(21.3125219557939,27.0760569908086,-15.632368792237));
#38701=CARTESIAN_POINT('Ctrl Pts',(21.3125219557939,42.7084257830456,11.4436881985716));
#38702=CARTESIAN_POINT('Ctrl Pts',(21.3125219557939,15.632368792237,27.0760569908086));
#38703=CARTESIAN_POINT('Ctrl Pts',(21.3125219557939,-10.2617970211066,42.0260605935833));
#38704=CARTESIAN_POINT('Ctrl Pts',(21.3125219557939,-26.3518679613905,16.8244723890963));
#38705=CARTESIAN_POINT('Ctrl Pts',(20.0742472323676,-26.1010282252799,16.6643225955232));
#38706=CARTESIAN_POINT('Ctrl Pts',(20.0742472323676,-26.4728487465358,16.0819468125049));
#38707=CARTESIAN_POINT('Ctrl Pts',(20.0742472323676,-26.8183238008715,15.4835664656478));
#38708=CARTESIAN_POINT('Ctrl Pts',(20.0742472323676,-42.3018902665193,-11.3347573352238));
#38709=CARTESIAN_POINT('Ctrl Pts',(20.0742472323676,-15.4835664656478,-26.8183238008715));
#38710=CARTESIAN_POINT('Ctrl Pts',(20.0742472323676,11.3347573352238,-42.3018902665193));
#38711=CARTESIAN_POINT('Ctrl Pts',(20.0742472323676,26.8183238008715,-15.4835664656478));
#38712=CARTESIAN_POINT('Ctrl Pts',(20.0742472323676,42.3018902665193,11.3347573352238));
#38713=CARTESIAN_POINT('Ctrl Pts',(20.0742472323676,15.4835664656478,26.8183238008715));
#38714=CARTESIAN_POINT('Ctrl Pts',(20.0742472323676,-10.1641164141543,41.6260204156154));
#38715=CARTESIAN_POINT('Ctrl Pts',(20.0742472323676,-26.1010282252799,16.6643225955232));
#38716=CARTESIAN_POINT('Ctrl Pts',(18.7979917002302,-25.8989065200918,16.5352770548748));
#38717=CARTESIAN_POINT('Ctrl Pts',(18.7979917002302,-26.2678477295776,15.9574110860028));
#38718=CARTESIAN_POINT('Ctrl Pts',(18.7979917002302,-26.6106474867381,15.3636644897785));
#38719=CARTESIAN_POINT('Ctrl Pts',(18.7979917002302,-41.9743119765166,-11.2469829969596));
#38720=CARTESIAN_POINT('Ctrl Pts',(18.7979917002302,-15.3636644897785,-26.6106474867381));
#38721=CARTESIAN_POINT('Ctrl Pts',(18.7979917002302,11.2469829969596,-41.9743119765166));
#38722=CARTESIAN_POINT('Ctrl Pts',(18.7979917002302,26.6106474867381,-15.3636644897785));
#38723=CARTESIAN_POINT('Ctrl Pts',(18.7979917002302,41.9743119765166,11.2469829969596));
#38724=CARTESIAN_POINT('Ctrl Pts',(18.7979917002302,15.3636644897785,26.6106474867381));
#38725=CARTESIAN_POINT('Ctrl Pts',(18.7979917002302,-10.0854073102973,41.303675941138));
#38726=CARTESIAN_POINT('Ctrl Pts',(18.7979917002302,-25.8989065200918,16.5352770548748));
#38727=CARTESIAN_POINT('Ctrl Pts',(17.4917404060759,-25.7420647185138,16.4351406788133));
#38728=CARTESIAN_POINT('Ctrl Pts',(17.4917404060759,-26.1087716481884,15.8607742221527));
#38729=CARTESIAN_POINT('Ctrl Pts',(17.4917404060759,-26.4494954361781,15.2706233100072));
#38730=CARTESIAN_POINT('Ctrl Pts',(17.4917404060759,-41.7201187461852,-11.1788721261709));
#38731=CARTESIAN_POINT('Ctrl Pts',(17.4917404060759,-15.2706233100072,-26.4494954361781));
#38732=CARTESIAN_POINT('Ctrl Pts',(17.4917404060759,11.1788721261709,-41.7201187461852));
#38733=CARTESIAN_POINT('Ctrl Pts',(17.4917404060759,26.4494954361781,-15.2706233100072));
#38734=CARTESIAN_POINT('Ctrl Pts',(17.4917404060759,41.7201187461852,11.1788721261709));
#38735=CARTESIAN_POINT('Ctrl Pts',(17.4917404060759,15.2706233100072,26.4494954361781));
#38736=CARTESIAN_POINT('Ctrl Pts',(17.4917404060759,-10.0243308532288,41.0535440314616));
#38737=CARTESIAN_POINT('Ctrl Pts',(17.4917404060759,-25.7420647185138,16.4351406788133));
#38738=CARTESIAN_POINT('Ctrl Pts',(16.1647270995715,-25.6237637373094,16.3596108683728));
#38739=CARTESIAN_POINT('Ctrl Pts',(16.1647270995715,-25.988785417954,15.7878839869031));
#38740=CARTESIAN_POINT('Ctrl Pts',(16.1647270995715,-26.3279433657953,15.2004451894512));
#38741=CARTESIAN_POINT('Ctrl Pts',(16.1647270995715,-41.5283885552464,-11.1274981763441));
#38742=CARTESIAN_POINT('Ctrl Pts',(16.1647270995715,-15.2004451894512,-26.3279433657953));
#38743=CARTESIAN_POINT('Ctrl Pts',(16.1647270995715,11.1274981763441,-41.5283885552464));
#38744=CARTESIAN_POINT('Ctrl Pts',(16.1647270995715,26.3279433657953,-15.2004451894512));
#38745=CARTESIAN_POINT('Ctrl Pts',(16.1647270995715,41.5283885552464,11.1274981763441));
#38746=CARTESIAN_POINT('Ctrl Pts',(16.1647270995715,15.2004451894512,26.3279433657953));
#38747=CARTESIAN_POINT('Ctrl Pts',(16.1647270995715,-9.97826274685029,40.8648771706659));
#38748=CARTESIAN_POINT('Ctrl Pts',(16.1647270995715,-25.6237637373094,16.3596108683728));
#38749=CARTESIAN_POINT('Ctrl Pts',(14.8263876417415,-25.5355400760542,16.3032840624315));
#38750=CARTESIAN_POINT('Ctrl Pts',(14.8263876417415,-25.8993049721986,15.7335256598799));
#38751=CARTESIAN_POINT('Ctrl Pts',(14.8263876417415,-26.2372951854241,15.1481094381123));
#38752=CARTESIAN_POINT('Ctrl Pts',(14.8263876417415,-41.3854046235364,-11.0891857473118));
#38753=CARTESIAN_POINT('Ctrl Pts',(14.8263876417415,-15.1481094381123,-26.2372951854241));
#38754=CARTESIAN_POINT('Ctrl Pts',(14.8263876417415,11.0891857473118,-41.3854046235364));
#38755=CARTESIAN_POINT('Ctrl Pts',(14.8263876417415,26.2372951854241,-15.1481094381123));
#38756=CARTESIAN_POINT('Ctrl Pts',(14.8263876417415,41.3854046235364,11.0891857473118));
#38757=CARTESIAN_POINT('Ctrl Pts',(14.8263876417415,15.1481094381123,26.2372951854241));
#38758=CARTESIAN_POINT('Ctrl Pts',(14.8263876417415,-9.94390718216752,40.7241777356532));
#38759=CARTESIAN_POINT('Ctrl Pts',(14.8263876417415,-25.5355400760542,16.3032840624315));
#38760=CARTESIAN_POINT('Ctrl Pts',(13.4853470903953,-25.4687774591536,16.260659159851));
#38761=CARTESIAN_POINT('Ctrl Pts',(13.4853470903953,-25.8315912927267,15.6923903894687));
#38762=CARTESIAN_POINT('Ctrl Pts',(13.4853470903953,-26.1686978312363,15.1085047372063));
#38763=CARTESIAN_POINT('Ctrl Pts',(13.4853470903953,-41.2772025684426,-11.06019309403));
#38764=CARTESIAN_POINT('Ctrl Pts',(13.4853470903953,-15.1085047372063,-26.1686978312363));
#38765=CARTESIAN_POINT('Ctrl Pts',(13.4853470903953,11.06019309403,-41.2772025684426));
#38766=CARTESIAN_POINT('Ctrl Pts',(13.4853470903953,26.1686978312363,-15.1085047372063));
#38767=CARTESIAN_POINT('Ctrl Pts',(13.4853470903953,41.2772025684426,11.06019309403));
#38768=CARTESIAN_POINT('Ctrl Pts',(13.4853470903953,15.1085047372063,26.1686978312363));
#38769=CARTESIAN_POINT('Ctrl Pts',(13.4853470903953,-9.91790885733393,40.617704456895));
#38770=CARTESIAN_POINT('Ctrl Pts',(13.4853470903953,-25.4687774591536,16.260659159851));
#38771=CARTESIAN_POINT('Ctrl Pts',(12.1482076787549,-25.4164718226475,16.2272643834928));
#38772=CARTESIAN_POINT('Ctrl Pts',(12.1482076787549,-25.778540539635,15.660162675793));
#38773=CARTESIAN_POINT('Ctrl Pts',(12.1482076787549,-26.1149547570431,15.0774761588537));
#38774=CARTESIAN_POINT('Ctrl Pts',(12.1482076787549,-41.1924309158968,-11.0374785981893));
#38775=CARTESIAN_POINT('Ctrl Pts',(12.1482076787549,-15.0774761588537,-26.1149547570431));
#38776=CARTESIAN_POINT('Ctrl Pts',(12.1482076787549,11.0374785981893,-41.1924309158968));
#38777=CARTESIAN_POINT('Ctrl Pts',(12.1482076787549,26.1149547570431,-15.0774761588537));
#38778=CARTESIAN_POINT('Ctrl Pts',(12.1482076787549,41.1924309158968,11.0374785981893));
#38779=CARTESIAN_POINT('Ctrl Pts',(12.1482076787549,15.0774761588537,26.1149547570431));
#38780=CARTESIAN_POINT('Ctrl Pts',(12.1482076787549,-9.89754028893977,40.534287226192));
#38781=CARTESIAN_POINT('Ctrl Pts',(12.1482076787549,-25.4164718226475,16.2272643834928));
#38782=CARTESIAN_POINT('Ctrl Pts',(10.8190675759626,-25.3740740708084,16.200195342079));
#38783=CARTESIAN_POINT('Ctrl Pts',(10.8190675759626,-25.7355388133451,15.6340396286792));
#38784=CARTESIAN_POINT('Ctrl Pts',(10.8190675759626,-26.0713918511132,15.0523251033885));
#38785=CARTESIAN_POINT('Ctrl Pts',(10.8190675759626,-41.1237169545017,-11.0190667477248));
#38786=CARTESIAN_POINT('Ctrl Pts',(10.8190675759626,-15.0523251033885,-26.0713918511132));
#38787=CARTESIAN_POINT('Ctrl Pts',(10.8190675759626,11.0190667477248,-41.1237169545017));
#38788=CARTESIAN_POINT('Ctrl Pts',(10.8190675759626,26.0713918511132,-15.0523251033885));
#38789=CARTESIAN_POINT('Ctrl Pts',(10.8190675759626,41.1237169545017,11.0190667477248));
#38790=CARTESIAN_POINT('Ctrl Pts',(10.8190675759626,15.0523251033885,26.0713918511132));
#38791=CARTESIAN_POINT('Ctrl Pts',(10.8190675759626,-9.88102999357242,40.4666711281441));
#38792=CARTESIAN_POINT('Ctrl Pts',(10.8190675759626,-25.3740740708084,16.200195342079));
#38793=CARTESIAN_POINT('Ctrl Pts',(9.50027713254189,-25.3387651379321,16.1776521900286));
#38794=CARTESIAN_POINT('Ctrl Pts',(9.50027713254189,-25.6997268893332,15.6122843025816));
#38795=CARTESIAN_POINT('Ctrl Pts',(9.50027713254189,-26.0351125755702,15.0313792538877));
#38796=CARTESIAN_POINT('Ctrl Pts',(9.50027713254189,-41.0664918294579,-11.0037333216825));
#38797=CARTESIAN_POINT('Ctrl Pts',(9.50027713254189,-15.0313792538877,-26.0351125755702));
#38798=CARTESIAN_POINT('Ctrl Pts',(9.5002771325419,11.0037333216825,-41.0664918294579));
#38799=CARTESIAN_POINT('Ctrl Pts',(9.5002771325419,26.0351125755702,-15.0313792538877));
#38800=CARTESIAN_POINT('Ctrl Pts',(9.5002771325419,41.0664918294579,11.0037333216825));
#38801=CARTESIAN_POINT('Ctrl Pts',(9.50027713254189,15.0313792538877,26.0351125755702));
#38802=CARTESIAN_POINT('Ctrl Pts',(9.50027713254189,-9.8672801864339,40.4103603059007));
#38803=CARTESIAN_POINT('Ctrl Pts',(9.50027713254189,-25.3387651379321,16.1776521900286));
#38804=CARTESIAN_POINT('Ctrl Pts',(8.45435372222587,-25.3150436214797,16.1625070777669));
#38805=CARTESIAN_POINT('Ctrl Pts',(8.45435372222587,-25.6756674495416,15.5976684735573));
#38806=CARTESIAN_POINT('Ctrl Pts',(8.45435372222587,-26.0107391561104,15.0173072536015));
#38807=CARTESIAN_POINT('Ctrl Pts',(8.45435372222587,-41.0280464097118,-10.9934319025089));
#38808=CARTESIAN_POINT('Ctrl Pts',(8.45435372222587,-15.0173072536015,-26.0107391561104));
#38809=CARTESIAN_POINT('Ctrl Pts',(8.45435372222587,10.9934319025089,-41.0280464097118));
#38810=CARTESIAN_POINT('Ctrl Pts',(8.45435372222587,26.0107391561104,-15.0173072536015));
#38811=CARTESIAN_POINT('Ctrl Pts',(8.45435372222587,41.0280464097118,10.9934319025089));
#38812=CARTESIAN_POINT('Ctrl Pts',(8.45435372222587,15.0173072536015,26.0107391561104));
#38813=CARTESIAN_POINT('Ctrl Pts',(8.45435372222587,-9.85804268618443,40.3725291400319));
#38814=CARTESIAN_POINT('Ctrl Pts',(8.45435372222587,-25.3150436214797,16.1625070777669));
#38815=CARTESIAN_POINT('Ctrl Pts',(7.67514864245731,-25.2995613842179,16.1526223715399));
#38816=CARTESIAN_POINT('Ctrl Pts',(7.67514864245731,-25.6599646610633,15.5881292127269));
#38817=CARTESIAN_POINT('Ctrl Pts',(7.67514864245731,-25.9948314436454,15.0081229315276));
#38818=CARTESIAN_POINT('Ctrl Pts',(7.67514864245731,-41.0029543751729,-10.9867085121177));
#38819=CARTESIAN_POINT('Ctrl Pts',(7.67514864245731,-15.0081229315276,-25.9948314436454));
#38820=CARTESIAN_POINT('Ctrl Pts',(7.67514864245731,10.9867085121177,-41.0029543751729));
#38821=CARTESIAN_POINT('Ctrl Pts',(7.67514864245731,25.9948314436454,-15.0081229315276));
#38822=CARTESIAN_POINT('Ctrl Pts',(7.67514864245731,41.0029543751729,10.9867085121177));
#38823=CARTESIAN_POINT('Ctrl Pts',(7.67514864245731,15.0081229315276,25.9948314436454));
#38824=CARTESIAN_POINT('Ctrl Pts',(7.67514864245731,-9.85201367995056,40.3478380083732));
#38825=CARTESIAN_POINT('Ctrl Pts',(7.67514864245731,-25.2995613842179,16.1526223715399));
#38826=CARTESIAN_POINT('Ctrl Pts',(7.15799654185577,-25.2902623130707,16.1466853364124));
#38827=CARTESIAN_POINT('Ctrl Pts',(7.15799654185577,-25.6505331205953,15.5823996619098));
#38828=CARTESIAN_POINT('Ctrl Pts',(7.15799654185577,-25.9852768200144,15.0026065670023));
#38829=CARTESIAN_POINT('Ctrl Pts',(7.15799654185577,-40.9878833870167,-10.9826702530121));
#38830=CARTESIAN_POINT('Ctrl Pts',(7.15799654185577,-15.0026065670023,-25.9852768200144));
#38831=CARTESIAN_POINT('Ctrl Pts',(7.15799654185577,10.9826702530121,-40.9878833870167));
#38832=CARTESIAN_POINT('Ctrl Pts',(7.15799654185577,25.9852768200144,-15.0026065670023));
#38833=CARTESIAN_POINT('Ctrl Pts',(7.15799654185577,40.9878833870167,10.9826702530121));
#38834=CARTESIAN_POINT('Ctrl Pts',(7.15799654185577,15.0026065670023,25.9852768200144));
#38835=CARTESIAN_POINT('Ctrl Pts',(7.15799654185577,-9.84839248767922,40.3330078138659));
#38836=CARTESIAN_POINT('Ctrl Pts',(7.15799654185577,-25.2902623130707,16.1466853364124));
#38837=CARTESIAN_POINT('Ctrl Pts',(6.9,-25.2858683590648,16.1438799960867));
#38838=CARTESIAN_POINT('Ctrl Pts',(6.9,-25.6460765727998,15.5796923611089));
#38839=CARTESIAN_POINT('Ctrl Pts',(6.9,-25.9807621135332,15.));
#38840=CARTESIAN_POINT('Ctrl Pts',(6.9,-40.9807621135332,-10.9807621135331));
#38841=CARTESIAN_POINT('Ctrl Pts',(6.9,-15.,-25.9807621135332));
#38842=CARTESIAN_POINT('Ctrl Pts',(6.9,10.9807621135331,-40.9807621135332));
#38843=CARTESIAN_POINT('Ctrl Pts',(6.9,25.9807621135332,-15.));
#38844=CARTESIAN_POINT('Ctrl Pts',(6.9,40.9807621135332,10.9807621135331));
#38845=CARTESIAN_POINT('Ctrl Pts',(6.9,15.,25.9807621135332));
#38846=CARTESIAN_POINT('Ctrl Pts',(6.9,-9.84668141868803,40.3260003190816));
#38847=CARTESIAN_POINT('Ctrl Pts',(6.9,-25.2858683590648,16.1438799960867));
#38848=CARTESIAN_POINT('Ctrl Pts',(6.9,-28.7358750109634,-8.61681422303452));
#38849=CARTESIAN_POINT('Ctrl Pts',(7.85773098116326,-29.3220126177434,-6.72950262532883));
#38850=CARTESIAN_POINT('Ctrl Pts',(8.88781981167334,-29.7139609348499,-4.83176468807716));
#38851=CARTESIAN_POINT('Ctrl Pts',(10.5914578196776,-30.0626260759601,-1.83991777043967));
#38852=CARTESIAN_POINT('Ctrl Pts',(11.2365058953701,-30.1308526921615,-0.737334477600522));
#38853=CARTESIAN_POINT('Ctrl Pts',(12.0558885382926,-30.1493644860168,0.56499838642607));
#38854=CARTESIAN_POINT('Ctrl Pts',(12.1875764958397,-30.1503477937894,0.770798830274837));
#38855=CARTESIAN_POINT('Ctrl Pts',(13.194901830313,-30.1433772121647,2.3283505906396));
#38856=CARTESIAN_POINT('Ctrl Pts',(14.2258982134098,-30.0606334052373,3.91692083548089));
#38857=CARTESIAN_POINT('Ctrl Pts',(18.2616480823244,-29.4024246647732,8.94354621773404));
#38858=CARTESIAN_POINT('Ctrl Pts',(21.0496416709525,-28.796919295079,11.660889676038));
#38859=CARTESIAN_POINT('Ctrl Pts',(25.8000196361138,-29.3778263502455,14.7241675584603));
#38860=CARTESIAN_POINT('Ctrl Pts',(26.8976561124457,-29.7353019177929,15.1580512376427));
#38861=CARTESIAN_POINT('Ctrl Pts',(28.0045908801237,-30.0977443108623,15.5447817028247));
#38862=CARTESIAN_POINT('Ctrl Pts',(28.5235971652406,-30.2828992744991,15.6994510084801));
#38863=CARTESIAN_POINT('Ctrl Pts',(29.0834839543824,-30.4804113157012,15.8677990842846));
#38864=CARTESIAN_POINT('Ctrl Pts',(29.1146288039499,-30.4913713634453,15.877207296405));
#38865=CARTESIAN_POINT('Ctrl Pts',(29.5949306848436,-30.6609898319163,16.0210111630069));
#38866=CARTESIAN_POINT('Ctrl Pts',(30.0492939924726,-30.8338536064743,16.1312811324031));
#38867=CARTESIAN_POINT('Ctrl Pts',(30.5,-31.0097594187194,16.229443021655));
#38868=CARTESIAN_POINT('Ctrl Pts',(6.45331003273164,-10.2495589536195,-4.07387898226151));
#38869=CARTESIAN_POINT('Ctrl Pts',(7.20830533428676,-10.4589493929845,-3.54117612793134));
#38870=CARTESIAN_POINT('Ctrl Pts',(7.99943720515023,-10.6278530262204,-3.00808536723907));
#38871=CARTESIAN_POINT('Ctrl Pts',(9.76195392812149,-10.8974188156737,-1.87226624217412));
#38872=CARTESIAN_POINT('Ctrl Pts',(10.7319699357145,-10.978614804603,-1.2567580486118));
#38873=CARTESIAN_POINT('Ctrl Pts',(12.6618070777417,-11.0581512103982,-0.165209663835397));
#38874=CARTESIAN_POINT('Ctrl Pts',(13.6366888866736,-11.0460663569154,0.364704064273057));
#38875=CARTESIAN_POINT('Ctrl Pts',(15.55636942495,-10.9884970038505,1.27025231764748));
#38876=CARTESIAN_POINT('Ctrl Pts',(16.5294822240035,-10.9232664847119,1.69980161462952));
#38877=CARTESIAN_POINT('Ctrl Pts',(18.4405353898674,-10.79829507883,2.41132585012623));
#38878=CARTESIAN_POINT('Ctrl Pts',(19.4148048972757,-10.7128845485964,2.74047342809725));
#38879=CARTESIAN_POINT('Ctrl Pts',(20.6320159197514,-10.6248232626626,3.07372863623311));
#38880=CARTESIAN_POINT('Ctrl Pts',(21.1045081958651,-10.5890632628362,3.19855905527616));
#38881=CARTESIAN_POINT('Ctrl Pts',(22.0534615877,-10.517515820459,3.42883778652053));
#38882=CARTESIAN_POINT('Ctrl Pts',(22.7823820470183,-10.4664588970829,3.58029681662344));
#38883=CARTESIAN_POINT('Ctrl Pts',(23.3297776630268,-10.4341170945838,3.67835397010646));
#38884=CARTESIAN_POINT('Ctrl Pts',(23.4470599317459,-10.4271412460568,3.69902619132828));
#38885=CARTESIAN_POINT('Ctrl Pts',(23.6811266122301,-10.4133903945396,3.73910834650872));
#38886=CARTESIAN_POINT('Ctrl Pts',(24.094173095085,-10.3895545652129,3.80664723977494));
#38887=CARTESIAN_POINT('Ctrl Pts',(24.6899146335616,-10.3570603924452,3.8946407511));
#38888=CARTESIAN_POINT('Ctrl Pts',(25.2912361170961,-10.3283061836388,3.96994444386569));
#38889=CARTESIAN_POINT('Ctrl Pts',(25.7735285180352,-10.3085973054881,4.02162740546583));
#38890=CARTESIAN_POINT('Ctrl Pts',(26.0148283477101,-10.3000025859218,4.04448759176681));
#38891=CARTESIAN_POINT('Ctrl Pts',(26.5981242438445,-10.2809495486037,4.09600397233593));
#38892=CARTESIAN_POINT('Ctrl Pts',(27.5413774795631,-10.2607319091994,4.14752077886532));
#38893=CARTESIAN_POINT('Ctrl Pts',(28.5384263877915,-10.2503835882544,4.17105255246829));
#38894=CARTESIAN_POINT('Ctrl Pts',(29.123550305837,-10.2444533826691,4.18584784382928));
#38895=CARTESIAN_POINT('Ctrl Pts',(29.2812719873802,-10.2430815653884,4.18934848102512));
#38896=CARTESIAN_POINT('Ctrl Pts',(29.6033573831701,-10.2409825864506,4.19465178436656));
#38897=CARTESIAN_POINT('Ctrl Pts',(30.1682075695061,-10.2390432854401,4.19956029863434));
#38898=CARTESIAN_POINT('Ctrl Pts',(31.3151152846709,-10.2404426493562,4.19601580459667));
#38899=CARTESIAN_POINT('Ctrl Pts',(32.3203773995797,-10.2455622764132,4.18330340731803));
#38900=CARTESIAN_POINT('Ctrl Pts',(33.1677006908683,-10.245571342205,4.18329188254759));
#38901=CARTESIAN_POINT('Ctrl Pts',(33.4949132850991,-10.2455724350351,4.18329063364476));
#38902=CARTESIAN_POINT('Ctrl Pts',(34.1541785734607,-10.2455743198855,4.18328832445807));
#38903=CARTESIAN_POINT('Ctrl Pts',(34.976129104799,-10.2455804319184,4.18328098024987));
#38904=CARTESIAN_POINT('Ctrl Pts',(35.9637295000903,-10.2455829874647,4.18327789132127));
#38905=CARTESIAN_POINT('Ctrl Pts',(37.938359040684,-10.2455864680815,4.1832737025367));
#38906=CARTESIAN_POINT('Ctrl Pts',(39.5833333333333,-10.2456046429336,4.18325179103929));
#38907=CARTESIAN_POINT('Ctrl Pts',(40.9,-10.2456046429336,4.18325179103929));
#38908=CARTESIAN_POINT('Ctrl Pts',(6.63336813585096,-13.590868440034,-4.85602971916216));
#38909=CARTESIAN_POINT('Ctrl Pts',(7.389696336477,-13.8391951107513,-4.14888858981181));
#38910=CARTESIAN_POINT('Ctrl Pts',(8.18053946683774,-14.0346488726453,-3.44401143686367));
#38911=CARTESIAN_POINT('Ctrl Pts',(9.94201947683641,-14.3333081335907,-1.94757748540838));
#38912=CARTESIAN_POINT('Ctrl Pts',(10.9113717350149,-14.4104989873604,-1.13915583855168));
#38913=CARTESIAN_POINT('Ctrl Pts',(12.8347397322171,-14.4628660834127,0.286629408466327));
#38914=CARTESIAN_POINT('Ctrl Pts',(13.808142871698,-14.4226409916871,0.978270473832921));
#38915=CARTESIAN_POINT('Ctrl Pts',(15.7151185916567,-14.3061107665235,2.15221389622412));
#38916=CARTESIAN_POINT('Ctrl Pts',(16.6852254797785,-14.2015789338064,2.70962741922244));
#38917=CARTESIAN_POINT('Ctrl Pts',(18.5768226767694,-14.0076819635675,3.62608620812781));
#38918=CARTESIAN_POINT('Ctrl Pts',(19.5464729449597,-13.8818273075211,4.05120533415429));
#38919=CARTESIAN_POINT('Ctrl Pts',(20.7463406818481,-13.7535017581768,4.47793026920172));
#38920=CARTESIAN_POINT('Ctrl Pts',(21.2156214332097,-13.7015810566901,4.63869318435445));
#38921=CARTESIAN_POINT('Ctrl Pts',(22.1537708528638,-13.5988388255709,4.9339087652619));
#38922=CARTESIAN_POINT('Ctrl Pts',(22.8728508922897,-13.5262523639447,5.12767073297799));
#38923=CARTESIAN_POINT('Ctrl Pts',(23.4112391022538,-13.48036797944,5.25280074041754));
#38924=CARTESIAN_POINT('Ctrl Pts',(23.5274006995054,-13.4704404449522,5.27931561824266));
#38925=CARTESIAN_POINT('Ctrl Pts',(23.75869759757,-13.4509289072634,5.3306297071107));
#38926=CARTESIAN_POINT('Ctrl Pts',(24.1668938536999,-13.4171810922989,5.41708560365397));
#38927=CARTESIAN_POINT('Ctrl Pts',(24.7548128660958,-13.3713845002052,5.52956305821883));
#38928=CARTESIAN_POINT('Ctrl Pts',(25.3473131502197,-13.3310219589392,5.62567073595883));
#38929=CARTESIAN_POINT('Ctrl Pts',(25.8218041556281,-13.3034028562425,5.69154378511353));
#38930=CARTESIAN_POINT('Ctrl Pts',(26.0589587666352,-13.2913640661324,5.72065900880548));
#38931=CARTESIAN_POINT('Ctrl Pts',(26.6316948383761,-13.2646759506016,5.78623492045644));
#38932=CARTESIAN_POINT('Ctrl Pts',(27.5576851463966,-13.236440987388,5.85186367837989));
#38933=CARTESIAN_POINT('Ctrl Pts',(28.5507795710394,-13.2219159498841,5.88219883517421));
#38934=CARTESIAN_POINT('Ctrl Pts',(29.1361849357887,-13.2135466774645,5.90128718803104));
#38935=CARTESIAN_POINT('Ctrl Pts',(29.2912521292177,-13.211632738116,5.90574282943922));
#38936=CARTESIAN_POINT('Ctrl Pts',(29.6100275770339,-13.2086893874642,5.91253309751288));
#38937=CARTESIAN_POINT('Ctrl Pts',(30.1692894984413,-13.2059721234291,5.91881362945886));
#38938=CARTESIAN_POINT('Ctrl Pts',(31.3098805820073,-13.2079309635128,5.91428725204102));
#38939=CARTESIAN_POINT('Ctrl Pts',(32.3163182251692,-13.215170536538,5.89785677449482));
#38940=CARTESIAN_POINT('Ctrl Pts',(33.1686695899412,-13.2151857432769,5.89783797451692));
#38941=CARTESIAN_POINT('Ctrl Pts',(33.4952713010558,-13.2151875891279,5.89783593918779));
#38942=CARTESIAN_POINT('Ctrl Pts',(34.1548283685118,-13.2151907586342,5.8978321735044));
#38943=CARTESIAN_POINT('Ctrl Pts',(34.9764778638342,-13.2152010495211,5.89782019909883));
#38944=CARTESIAN_POINT('Ctrl Pts',(35.9641101124161,-13.2152053506642,5.89781516246843));
#38945=CARTESIAN_POINT('Ctrl Pts',(37.9386244259607,-13.2152112104218,5.89780833274506));
#38946=CARTESIAN_POINT('Ctrl Pts',(39.5833333333333,-13.2152418049849,5.89777260594516));
#38947=CARTESIAN_POINT('Ctrl Pts',(40.9,-13.2152418049849,5.89777260594516));
#38948=CARTESIAN_POINT('Ctrl Pts',(6.84649785567288,-21.377211306072,-6.71741536412573));
#38949=CARTESIAN_POINT('Ctrl Pts',(7.61279643984166,-21.7222003209083,-5.59224351411651));
#38950=CARTESIAN_POINT('Ctrl Pts',(8.41290239278216,-21.9819683115275,-4.4778139915129));
#38951=CARTESIAN_POINT('Ctrl Pts',(10.1883118359637,-22.351694214315,-2.12504829883047));
#38952=CARTESIAN_POINT('Ctrl Pts',(11.1645908932198,-22.4195115822635,-0.860235293933496));
#38953=CARTESIAN_POINT('Ctrl Pts',(13.104616539894,-22.4060524143024,1.36442582505286));
#38954=CARTESIAN_POINT('Ctrl Pts',(14.0814329274866,-22.2982732069865,2.43568052201622));
#38955=CARTESIAN_POINT('Ctrl Pts',(15.9946796213894,-22.0394507048972,4.24582169215594));
#38956=CARTESIAN_POINT('Ctrl Pts',(16.9653275559585,-21.84127820419,5.10151618176833));
#38957=CARTESIAN_POINT('Ctrl Pts',(18.8448710605557,-21.4842569534398,6.49486940232067));
#38958=CARTESIAN_POINT('Ctrl Pts',(19.8101236302159,-21.2634255374822,7.14150804350577));
#38959=CARTESIAN_POINT('Ctrl Pts',(20.9856903475787,-21.0426589820635,7.78021164720302));
#38960=CARTESIAN_POINT('Ctrl Pts',(21.4500377829479,-20.9532273635236,8.0234729107848));
#38961=CARTESIAN_POINT('Ctrl Pts',(22.3710393802638,-20.7788884454096,8.46623345546781));
#38962=CARTESIAN_POINT('Ctrl Pts',(23.0719693188992,-20.6575298272077,8.75491470148121));
#38963=CARTESIAN_POINT('Ctrl Pts',(23.5926347936586,-20.5813719818061,8.94023465873173));
#38964=CARTESIAN_POINT('Ctrl Pts',(23.7065892332644,-20.5647099449239,8.98001571960571));
#38965=CARTESIAN_POINT('Ctrl Pts',(23.9323706520527,-20.5321468576875,9.0566499549595));
#38966=CARTESIAN_POINT('Ctrl Pts',(24.3307466212143,-20.4759485784751,9.1857404907663));
#38967=CARTESIAN_POINT('Ctrl Pts',(24.9023508233185,-20.4001844372317,9.35309964749801));
#38968=CARTESIAN_POINT('Ctrl Pts',(25.4757972573111,-20.3338472412531,9.49555868076779));
#38969=CARTESIAN_POINT('Ctrl Pts',(25.9330914993694,-20.28864648982,9.59288697707771));
#38970=CARTESIAN_POINT('Ctrl Pts',(26.1609781823311,-20.2689918009898,9.63581705245677));
#38971=CARTESIAN_POINT('Ctrl Pts',(26.709932241435,-20.2254900271807,9.73235004955936));
#38972=CARTESIAN_POINT('Ctrl Pts',(27.5959509089719,-20.1795241403997,9.82915847887795));
#38973=CARTESIAN_POINT('Ctrl Pts',(28.579749560637,-20.155272253243,9.87532060641945));
#38974=CARTESIAN_POINT('Ctrl Pts',(29.1657855350677,-20.1412111689925,9.90441669946595));
#38975=CARTESIAN_POINT('Ctrl Pts',(29.3146731630637,-20.1381027603739,9.91097811975321));
#38976=CARTESIAN_POINT('Ctrl Pts',(29.6257300067643,-20.1332492263269,9.92113271524804));
#38977=CARTESIAN_POINT('Ctrl Pts',(30.1719452394076,-20.1287785103479,9.93050366138696));
#38978=CARTESIAN_POINT('Ctrl Pts',(31.2977811219682,-20.1319916124711,9.92376874726301));
#38979=CARTESIAN_POINT('Ctrl Pts',(32.306925911767,-20.1442225454146,9.8985708956696));
#38980=CARTESIAN_POINT('Ctrl Pts',(33.1709940314752,-20.1442592438603,9.89851679451552));
#38981=CARTESIAN_POINT('Ctrl Pts',(33.4961680489761,-20.1442637388651,9.89851046735387));
#38982=CARTESIAN_POINT('Ctrl Pts',(34.1564024558335,-20.1442714128624,9.89849933968833));
#38983=CARTESIAN_POINT('Ctrl Pts',(34.9773378017947,-20.1442963704308,9.89846345509219));
#38984=CARTESIAN_POINT('Ctrl Pts',(35.9650395265661,-20.1443067963913,9.89844842592582));
#38985=CARTESIAN_POINT('Ctrl Pts',(37.9392783163648,-20.1443210056784,9.8984279817608));
#38986=CARTESIAN_POINT('Ctrl Pts',(39.5833333333333,-20.1443951831047,9.89832117405885));
#38987=CARTESIAN_POINT('Ctrl Pts',(40.9,-20.1443951831047,9.89832117405885));
#38988=CARTESIAN_POINT('Ctrl Pts',(6.90857970435319,-29.1272609852091,-8.7101858572574));
#38989=CARTESIAN_POINT('Ctrl Pts',(7.67983757144493,-29.5775536996439,-7.16260494418019));
#38990=CARTESIAN_POINT('Ctrl Pts',(8.48457055999567,-29.9097225030882,-5.63283520142948));
#38991=CARTESIAN_POINT('Ctrl Pts',(10.2689932185249,-30.3644487697131,-2.41146069737717));
#38992=CARTESIAN_POINT('Ctrl Pts',(11.2491988139072,-30.4296414097155,-0.683672158318401));
#38993=CARTESIAN_POINT('Ctrl Pts',(13.2074449203971,-30.3576235761244,2.36894751212039));
#38994=CARTESIAN_POINT('Ctrl Pts',(14.1878085217557,-30.184965998838,3.82665309566743));
#38995=CARTESIAN_POINT('Ctrl Pts',(16.1228140255812,-29.7814752498472,6.30658851121945));
#38996=CARTESIAN_POINT('Ctrl Pts',(17.0983171044692,-29.4886591763938,7.46839135174002));
#38997=CARTESIAN_POINT('Ctrl Pts',(18.9977376700381,-28.960082872958,9.36704911481261));
#38998=CARTESIAN_POINT('Ctrl Pts',(19.9674462816337,-28.6415548808293,10.2409515663328));
#38999=CARTESIAN_POINT('Ctrl Pts',(21.1471060032309,-28.3239820751165,11.1004135437216));
#39000=CARTESIAN_POINT('Ctrl Pts',(21.6116736136674,-28.1962714220824,11.4272945418467));
#39001=CARTESIAN_POINT('Ctrl Pts',(22.5321107331754,-27.9485409607959,12.020283834991));
#39002=CARTESIAN_POINT('Ctrl Pts',(23.2282372947769,-27.7781185470828,12.4035528917693));
#39003=CARTESIAN_POINT('Ctrl Pts',(23.7411423015336,-27.6723004799183,12.6473785079706));
#39004=CARTESIAN_POINT('Ctrl Pts',(23.8541050059083,-27.6489722597556,12.7001926206312));
#39005=CARTESIAN_POINT('Ctrl Pts',(24.0772792343329,-27.603576753781,12.8015323632731));
#39006=CARTESIAN_POINT('Ctrl Pts',(24.4706231308706,-27.5254067801747,12.9720321690745));
#39007=CARTESIAN_POINT('Ctrl Pts',(25.0326506601034,-27.4207276483819,13.1919318242548));
#39008=CARTESIAN_POINT('Ctrl Pts',(25.5929166162092,-27.3299203180183,13.3777331675809));
#39009=CARTESIAN_POINT('Ctrl Pts',(26.036986986334,-27.2685418388,13.5038445845534));
#39010=CARTESIAN_POINT('Ctrl Pts',(26.257289284528,-27.2420133361897,13.5592118403736));
#39011=CARTESIAN_POINT('Ctrl Pts',(26.7861809172635,-27.1835476308027,13.6833062419416));
#39012=CARTESIAN_POINT('Ctrl Pts',(27.6340630276978,-27.1220525704358,13.8074117592232));
#39013=CARTESIAN_POINT('Ctrl Pts',(28.6084466264574,-27.0881176443602,13.8693290201703));
#39014=CARTESIAN_POINT('Ctrl Pts',(29.1951297895239,-27.0683644245336,13.908430904103));
#39015=CARTESIAN_POINT('Ctrl Pts',(29.3379067795074,-27.0642236253566,13.9168171018367));
#39016=CARTESIAN_POINT('Ctrl Pts',(29.6412852452592,-27.0575993546201,13.9300946799831));
#39017=CARTESIAN_POINT('Ctrl Pts',(30.1744790744102,-27.0515191755617,13.9423073235085));
#39018=CARTESIAN_POINT('Ctrl Pts',(31.285567721335,-27.0558675796336,13.933569334585));
#39019=CARTESIAN_POINT('Ctrl Pts',(32.2974599236722,-27.0731946134563,13.8994232817537));
#39020=CARTESIAN_POINT('Ctrl Pts',(33.1732579076352,-27.0732696672436,13.8993047075201));
#39021=CARTESIAN_POINT('Ctrl Pts',(33.4970065888605,-27.0732789151667,13.8992904506871));
#39022=CARTESIAN_POINT('Ctrl Pts',(34.1579215418455,-27.0732946436725,13.8992658208367));
#39023=CARTESIAN_POINT('Ctrl Pts',(34.9781539333149,-27.0733458523266,13.8991859907804));
#39024=CARTESIAN_POINT('Ctrl Pts',(35.9659297143336,-27.0733672375489,13.8991526077107));
#39025=CARTESIAN_POINT('Ctrl Pts',(37.9398993196362,-27.0733963900547,13.8991071452309));
#39026=CARTESIAN_POINT('Ctrl Pts',(39.5833333333333,-27.0735485612246,13.8988697421725));
#39027=CARTESIAN_POINT('Ctrl Pts',(40.9,-27.0735485612246,13.8988697421725));
#39028=CARTESIAN_POINT('Ctrl Pts',(6.93528330520032,-33.5512413216408,-9.86563481868489));
#39029=CARTESIAN_POINT('Ctrl Pts',(7.70864561497005,-34.0623374960229,-8.07765806999139));
#39030=CARTESIAN_POINT('Ctrl Pts',(8.51541871352369,-34.4367698578613,-6.31093086144101));
#39031=CARTESIAN_POINT('Ctrl Pts',(10.3035747340621,-34.941954951338,-2.59403255178488));
#39032=CARTESIAN_POINT('Ctrl Pts',(11.2855474597114,-35.0067705115655,-0.601863607331424));
#39033=CARTESIAN_POINT('Ctrl Pts',(13.2510271399958,-34.9032893217431,2.92382891559037));
#39034=CARTESIAN_POINT('Ctrl Pts',(14.2329608248363,-34.6945593989858,4.60257161238985));
#39035=CARTESIAN_POINT('Ctrl Pts',(16.1768697182175,-34.2095752766376,7.46747574760142));
#39036=CARTESIAN_POINT('Ctrl Pts',(17.1545233971705,-33.863251175018,8.80499374792142));
#39037=CARTESIAN_POINT('Ctrl Pts',(19.0635787323924,-33.2359528227277,10.9976618314205));
#39038=CARTESIAN_POINT('Ctrl Pts',(20.0357940514507,-32.8613840028834,12.0029926013879));
#39039=CARTESIAN_POINT('Ctrl Pts',(21.2200273744511,-32.4867165469276,12.9932317593815));
#39040=CARTESIAN_POINT('Ctrl Pts',(21.6852779128344,-32.3368305207217,13.3687144259959));
#39041=CARTESIAN_POINT('Ctrl Pts',(22.6074094382987,-32.0460468583651,14.0501505350056));
#39042=CARTESIAN_POINT('Ctrl Pts',(23.303404556016,-31.8467199720656,14.4891819334101));
#39043=CARTESIAN_POINT('Ctrl Pts',(23.8143672767891,-31.7234333079366,14.7674149360666));
#39044=CARTESIAN_POINT('Ctrl Pts',(23.9270724954075,-31.6962311639846,14.8277950271988));
#39045=CARTESIAN_POINT('Ctrl Pts',(24.1495225469484,-31.6433583861176,14.9435144746797));
#39046=CARTESIAN_POINT('Ctrl Pts',(24.5413305977736,-31.5524212197087,15.1380475804187));
#39047=CARTESIAN_POINT('Ctrl Pts',(25.0999889357199,-31.4310156375917,15.3882930140602));
#39048=CARTESIAN_POINT('Ctrl Pts',(25.6548568854792,-31.3262265443364,15.5988027583032));
#39049=CARTESIAN_POINT('Ctrl Pts',(26.0929602492094,-31.2557376661541,15.741087693316));
#39050=CARTESIAN_POINT('Ctrl Pts',(26.3096479269533,-31.2253935968531,15.8033473177939));
#39051=CARTESIAN_POINT('Ctrl Pts',(26.8287121638341,-31.1587088311854,15.9425694431084));
#39052=CARTESIAN_POINT('Ctrl Pts',(27.6557884297532,-31.0890012981156,16.0810926132799));
#39053=CARTESIAN_POINT('Ctrl Pts',(28.624709126668,-31.0495586097517,16.1519656805034));
#39054=CARTESIAN_POINT('Ctrl Pts',(29.2117706203409,-31.0265558099781,16.1967753671696));
#39055=CARTESIAN_POINT('Ctrl Pts',(29.351092195488,-31.021876437373,16.2061151113191));
#39056=CARTESIAN_POINT('Ctrl Pts',(29.6501043905816,-31.014285796168,16.2210980111665));
#39057=CARTESIAN_POINT('Ctrl Pts',(30.175870201979,-31.0073340046886,16.2348498398373));
#39058=CARTESIAN_POINT('Ctrl Pts',(31.278535210342,-31.0122942956317,16.2250286703999));
#39059=CARTESIAN_POINT('Ctrl Pts',(32.2920164760145,-31.0325718136052,16.1856975481828));
#39060=CARTESIAN_POINT('Ctrl Pts',(33.174523274163,-31.0326760798738,16.1855272745483));
#39061=CARTESIAN_POINT('Ctrl Pts',(33.4974585875216,-31.0326890056742,16.1855064782319));
#39062=CARTESIAN_POINT('Ctrl Pts',(34.158763915549,-31.0327109045834,16.1854709093049));
#39063=CARTESIAN_POINT('Ctrl Pts',(34.9785998474407,-31.0327822824583,16.1853552918984));
#39064=CARTESIAN_POINT('Ctrl Pts',(35.9664200829455,-31.0328120805002,16.1853069853609));
#39065=CARTESIAN_POINT('Ctrl Pts',(37.9402388284556,-31.0328527115371,16.185241157271));
#39066=CARTESIAN_POINT('Ctrl Pts',(39.5833333333333,-31.033064777293,16.1848974953804));
#39067=CARTESIAN_POINT('Ctrl Pts',(40.9,-31.033064777293,16.1848974953804));
#39068=CARTESIAN_POINT('Origin',(6.9,-15.,25.9807621135332));
#39069=CARTESIAN_POINT('',(6.9,-29.194404870986,6.90555748864273));
#39070=CARTESIAN_POINT('Ctrl Pts',(6.9,-10.8594625780008,1.92623027574191));
#39071=CARTESIAN_POINT('Ctrl Pts',(6.9,-14.5482083700348,3.00887228147899));
#39072=CARTESIAN_POINT('Ctrl Pts',(6.90000000166257,-18.4565659967827,4.07058553003038));
#39073=CARTESIAN_POINT('Ctrl Pts',(6.90000000166257,-24.1072623232988,5.57797815223758));
#39074=CARTESIAN_POINT('Ctrl Pts',(6.9,-26.6663167664834,6.24902093139924));
#39075=CARTESIAN_POINT('Ctrl Pts',(6.9,-29.194404870986,6.90555748864272));
#39076=CARTESIAN_POINT('Origin',(6.9,0.,0.));
#39077=CARTESIAN_POINT('Origin',(40.9,-4.5,7.79422863405995));
#39078=CARTESIAN_POINT('Ctrl Pts',(40.9,-18.5327260452907,29.0996231131986));
#39079=CARTESIAN_POINT('Ctrl Pts',(40.9,-18.2824786427117,28.6661818974695));
#39080=CARTESIAN_POINT('Ctrl Pts',(40.9,-18.0322312401326,28.2327406817405));
#39081=CARTESIAN_POINT('Ctrl Pts',(40.9,-17.7819838375536,27.7992994660114));
#39082=CARTESIAN_POINT('Ctrl Pts',(30.5,-16.1306417505986,31.061268433756));
#39083=CARTESIAN_POINT('Ctrl Pts',(30.5,-16.823692245373,30.7013555966443));
#39084=CARTESIAN_POINT('Ctrl Pts',(30.5,-17.5,30.3108891324554));
#39085=CARTESIAN_POINT('Ctrl Pts',(30.5,-47.8108891324553,12.8108891324554));
#39086=CARTESIAN_POINT('Ctrl Pts',(30.5,-30.3108891324554,-17.5));
#39087=CARTESIAN_POINT('Ctrl Pts',(30.5,-12.8108891324554,-47.8108891324553));
#39088=CARTESIAN_POINT('Ctrl Pts',(30.5,17.5,-30.3108891324554));
#39089=CARTESIAN_POINT('Ctrl Pts',(30.5,47.8108891324553,-12.8108891324554));
#39090=CARTESIAN_POINT('Ctrl Pts',(30.5,30.3108891324554,17.5));
#39091=CARTESIAN_POINT('Ctrl Pts',(30.5,13.5747778926489,46.4877949884694));
#39092=CARTESIAN_POINT('Ctrl Pts',(30.5,-16.1306417505986,31.061268433756));
#39093=CARTESIAN_POINT('Ctrl Pts',(30.3311478274255,-16.0958729911865,30.9943174850025));
#39094=CARTESIAN_POINT('Ctrl Pts',(30.3311478274255,-16.7874296516619,30.6351804212937));
#39095=CARTESIAN_POINT('Ctrl Pts',(30.3311478274255,-17.4622796600955,30.245555587262));
#39096=CARTESIAN_POINT('Ctrl Pts',(30.3311478274255,-47.7078352473574,12.7832759271665));
#39097=CARTESIAN_POINT('Ctrl Pts',(30.3311478274255,-30.245555587262,-17.4622796600955));
#39098=CARTESIAN_POINT('Ctrl Pts',(30.3311478274255,-12.7832759271665,-47.7078352473574));
#39099=CARTESIAN_POINT('Ctrl Pts',(30.3311478274255,17.4622796600955,-30.245555587262));
#39100=CARTESIAN_POINT('Ctrl Pts',(30.3311478274255,47.7078352473574,-12.7832759271665));
#39101=CARTESIAN_POINT('Ctrl Pts',(30.3311478274255,30.245555587262,17.4622796600955));
#39102=CARTESIAN_POINT('Ctrl Pts',(30.3311478274255,13.5455181648638,46.3875929639907));
#39103=CARTESIAN_POINT('Ctrl Pts',(30.3311478274255,-16.0958729911865,30.9943174850025));
#39104=CARTESIAN_POINT('Ctrl Pts',(29.9897712690917,-16.0254447695752,30.8587004444282));
#39105=CARTESIAN_POINT('Ctrl Pts',(29.9897712690917,-16.7139754925468,30.501134801215));
#39106=CARTESIAN_POINT('Ctrl Pts',(29.9897712690917,-17.3858726641896,30.1132147882992));
#39107=CARTESIAN_POINT('Ctrl Pts',(29.9897712690917,-47.4990874524888,12.7273421241097));
#39108=CARTESIAN_POINT('Ctrl Pts',(29.9897712690917,-30.1132147882992,-17.3858726641896));
#39109=CARTESIAN_POINT('Ctrl Pts',(29.9897712690917,-12.7273421241097,-47.4990874524888));
#39110=CARTESIAN_POINT('Ctrl Pts',(29.9897712690917,17.3858726641896,-30.1132147882992));
#39111=CARTESIAN_POINT('Ctrl Pts',(29.9897712690917,47.4990874524888,-12.7273421241097));
#39112=CARTESIAN_POINT('Ctrl Pts',(29.9897712690917,30.1132147882992,17.3858726641896));
#39113=CARTESIAN_POINT('Ctrl Pts',(29.9897712690917,13.4862491363571,46.1846219490559));
#39114=CARTESIAN_POINT('Ctrl Pts',(29.9897712690917,-16.0254447695752,30.8587004444282));
#39115=CARTESIAN_POINT('Ctrl Pts',(29.4666899049319,-15.9171300516369,30.6501289206644));
#39116=CARTESIAN_POINT('Ctrl Pts',(29.4666899049319,-16.6010070497276,30.2949800354474));
#39117=CARTESIAN_POINT('Ctrl Pts',(29.4666899049319,-17.2683629213518,29.9096819433198));
#39118=CARTESIAN_POINT('Ctrl Pts',(29.4666899049319,-47.1780448646716,12.6413190219681));
#39119=CARTESIAN_POINT('Ctrl Pts',(29.4666899049319,-29.9096819433198,-17.2683629213518));
#39120=CARTESIAN_POINT('Ctrl Pts',(29.4666899049319,-12.6413190219681,-47.1780448646716));
#39121=CARTESIAN_POINT('Ctrl Pts',(29.4666899049319,17.2683629213518,-29.9096819433198));
#39122=CARTESIAN_POINT('Ctrl Pts',(29.4666899049319,47.1780448646716,-12.6413190219681));
#39123=CARTESIAN_POINT('Ctrl Pts',(29.4666899049319,29.9096819433198,17.2683629213518));
#39124=CARTESIAN_POINT('Ctrl Pts',(29.4666899049319,13.3950966415431,45.8724637299593));
#39125=CARTESIAN_POINT('Ctrl Pts',(29.4666899049319,-15.9171300516369,30.6501289206644));
#39126=CARTESIAN_POINT('Ctrl Pts',(28.7471241621752,-15.7673462336858,30.3617042288049));
#39127=CARTESIAN_POINT('Ctrl Pts',(28.7471241621752,-16.4447877935127,30.0098973754615));
#39128=CARTESIAN_POINT('Ctrl Pts',(28.7471241621752,-17.105863694435,29.6282250261092));
#39129=CARTESIAN_POINT('Ctrl Pts',(28.7471241621752,-46.7340887205442,12.5223613316743));
#39130=CARTESIAN_POINT('Ctrl Pts',(28.7471241621752,-29.6282250261092,-17.105863694435));
#39131=CARTESIAN_POINT('Ctrl Pts',(28.7471241621752,-12.5223613316743,-46.7340887205442));
#39132=CARTESIAN_POINT('Ctrl Pts',(28.7471241621752,17.105863694435,-29.6282250261092));
#39133=CARTESIAN_POINT('Ctrl Pts',(28.7471241621752,46.7340887205442,-12.5223613316743));
#39134=CARTESIAN_POINT('Ctrl Pts',(28.7471241621752,29.6282250261092,17.105863694435));
#39135=CARTESIAN_POINT('Ctrl Pts',(28.7471241621752,13.2690457322218,45.4407934015768));
#39136=CARTESIAN_POINT('Ctrl Pts',(28.7471241621752,-15.7673462336858,30.3617042288049));
#39137=CARTESIAN_POINT('Ctrl Pts',(27.8100958442934,-15.5715428260696,29.9846639164451));
#39138=CARTESIAN_POINT('Ctrl Pts',(27.8100958442934,-16.2405717231752,29.6372259010587));
#39139=CARTESIAN_POINT('Ctrl Pts',(27.8100958442934,-16.8934381948013,29.2602932679205));
#39140=CARTESIAN_POINT('Ctrl Pts',(27.8100958442934,-46.1537314627218,12.3668550731192));
#39141=CARTESIAN_POINT('Ctrl Pts',(27.8100958442934,-29.2602932679205,-16.8934381948013));
#39142=CARTESIAN_POINT('Ctrl Pts',(27.8100958442934,-12.3668550731192,-46.1537314627218));
#39143=CARTESIAN_POINT('Ctrl Pts',(27.8100958442934,16.8934381948013,-29.2602932679205));
#39144=CARTESIAN_POINT('Ctrl Pts',(27.8100958442934,46.1537314627218,-12.3668550731192));
#39145=CARTESIAN_POINT('Ctrl Pts',(27.8100958442934,29.2602932679205,16.8934381948013));
#39146=CARTESIAN_POINT('Ctrl Pts',(27.8100958442934,13.1042669335782,44.8764966543029));
#39147=CARTESIAN_POINT('Ctrl Pts',(27.8100958442934,-15.5715428260696,29.9846639164451));
#39148=CARTESIAN_POINT('Ctrl Pts',(26.8343111708818,-15.3685420031368,29.5937642144445));
#39149=CARTESIAN_POINT('Ctrl Pts',(26.8343111708818,-16.0288490017,29.2508556284042));
#39150=CARTESIAN_POINT('Ctrl Pts',(26.8343111708818,-16.6732042787395,28.8788369357517));
#39151=CARTESIAN_POINT('Ctrl Pts',(26.8343111708818,-45.5520412144912,12.2056326570122));
#39152=CARTESIAN_POINT('Ctrl Pts',(26.8343111708818,-28.8788369357517,-16.6732042787395));
#39153=CARTESIAN_POINT('Ctrl Pts',(26.8343111708818,-12.2056326570122,-45.5520412144912));
#39154=CARTESIAN_POINT('Ctrl Pts',(26.8343111708818,16.6732042787395,-28.8788369357517));
#39155=CARTESIAN_POINT('Ctrl Pts',(26.8343111708818,45.5520412144912,-12.2056326570122));
#39156=CARTESIAN_POINT('Ctrl Pts',(26.8343111708818,28.8788369357517,16.6732042787395));
#39157=CARTESIAN_POINT('Ctrl Pts',(26.8343111708818,12.9334311338658,44.2914572749094));
#39158=CARTESIAN_POINT('Ctrl Pts',(26.8343111708818,-15.3685420031368,29.5937642144445));
#39159=CARTESIAN_POINT('Ctrl Pts',(25.8181479469611,-15.1612099270726,29.1945242233064));
#39160=CARTESIAN_POINT('Ctrl Pts',(25.8181479469611,-15.8126089354813,28.8562417071321));
#39161=CARTESIAN_POINT('Ctrl Pts',(25.8181479469611,-16.4482714219305,28.4892417994669));
#39162=CARTESIAN_POINT('Ctrl Pts',(25.8181479469611,-44.9375132213974,12.0409703775363));
#39163=CARTESIAN_POINT('Ctrl Pts',(25.8181479469611,-28.4892417994669,-16.4482714219305));
#39164=CARTESIAN_POINT('Ctrl Pts',(25.8181479469611,-12.0409703775363,-44.9375132213974));
#39165=CARTESIAN_POINT('Ctrl Pts',(25.8181479469611,16.4482714219305,-28.4892417994669));
#39166=CARTESIAN_POINT('Ctrl Pts',(25.8181479469611,44.9375132213974,-12.0409703775363));
#39167=CARTESIAN_POINT('Ctrl Pts',(25.8181479469611,28.4892417994669,16.4482714219305));
#39168=CARTESIAN_POINT('Ctrl Pts',(25.8181479469611,12.7589503583263,43.6939354158518));
#39169=CARTESIAN_POINT('Ctrl Pts',(25.8181479469611,-15.1612099270726,29.1945242233064));
#39170=CARTESIAN_POINT('Ctrl Pts',(24.7595197917227,-14.9547233834603,28.796912394945));
#39171=CARTESIAN_POINT('Ctrl Pts',(24.7595197917227,-15.5972507298839,28.4632370828042));
#39172=CARTESIAN_POINT('Ctrl Pts',(24.7595197917227,-16.2242558762949,28.1012354927406));
#39173=CARTESIAN_POINT('Ctrl Pts',(24.7595197917227,-44.3254913690355,11.8769796164458));
#39174=CARTESIAN_POINT('Ctrl Pts',(24.7595197917227,-28.1012354927406,-16.2242558762949));
#39175=CARTESIAN_POINT('Ctrl Pts',(24.7595197917227,-11.8769796164458,-44.3254913690355));
#39176=CARTESIAN_POINT('Ctrl Pts',(24.7595197917227,16.2242558762949,-28.1012354927406));
#39177=CARTESIAN_POINT('Ctrl Pts',(24.7595197917227,44.3254913690355,-11.8769796164458));
#39178=CARTESIAN_POINT('Ctrl Pts',(24.7595197917227,28.1012354927406,16.2242558762949));
#39179=CARTESIAN_POINT('Ctrl Pts',(24.7595197917227,12.5851811425261,43.0988503438666));
#39180=CARTESIAN_POINT('Ctrl Pts',(24.7595197917227,-14.9547233834603,28.796912394945));
#39181=CARTESIAN_POINT('Ctrl Pts',(23.6563574780851,-14.7559082828157,28.4140727469455));
#39182=CARTESIAN_POINT('Ctrl Pts',(23.6563574780851,-15.389893569599,28.084833470769));
#39183=CARTESIAN_POINT('Ctrl Pts',(23.6563574780851,-16.0085630157705,27.7276444994825));
#39184=CARTESIAN_POINT('Ctrl Pts',(23.6563574780851,-43.736207515253,11.7190814837121));
#39185=CARTESIAN_POINT('Ctrl Pts',(23.6563574780851,-27.7276444994825,-16.0085630157705));
#39186=CARTESIAN_POINT('Ctrl Pts',(23.6563574780851,-11.7190814837121,-43.736207515253));
#39187=CARTESIAN_POINT('Ctrl Pts',(23.6563574780851,16.0085630157705,-27.7276444994825));
#39188=CARTESIAN_POINT('Ctrl Pts',(23.6563574780851,43.736207515253,-11.7190814837121));
#39189=CARTESIAN_POINT('Ctrl Pts',(23.6563574780851,27.7276444994825,16.0085630157705));
#39190=CARTESIAN_POINT('Ctrl Pts',(23.6563574780851,12.4178678468319,42.5258740306932));
#39191=CARTESIAN_POINT('Ctrl Pts',(23.6563574780851,-14.7559082828157,28.4140727469455));
#39192=CARTESIAN_POINT('Ctrl Pts',(22.5073180101405,-14.5719314169357,28.0598057001003));
#39193=CARTESIAN_POINT('Ctrl Pts',(22.5073180101405,-15.1980121665098,27.7346713837132));
#39194=CARTESIAN_POINT('Ctrl Pts',(22.5073180101405,-15.8089680335819,27.3819358493961));
#39195=CARTESIAN_POINT('Ctrl Pts',(22.5073180101405,-43.190903882978,11.5729678158142));
#39196=CARTESIAN_POINT('Ctrl Pts',(22.5073180101405,-27.3819358493961,-15.8089680335819));
#39197=CARTESIAN_POINT('Ctrl Pts',(22.5073180101405,-11.5729678158142,-43.190903882978));
#39198=CARTESIAN_POINT('Ctrl Pts',(22.5073180101405,15.8089680335819,-27.3819358493961));
#39199=CARTESIAN_POINT('Ctrl Pts',(22.5073180101405,43.190903882978,-11.5729678158142));
#39200=CARTESIAN_POINT('Ctrl Pts',(22.5073180101405,27.3819358493961,15.8089680335819));
#39201=CARTESIAN_POINT('Ctrl Pts',(22.5073180101405,12.2630417010206,41.9956608528241));
#39202=CARTESIAN_POINT('Ctrl Pts',(22.5073180101405,-14.5719314169357,28.0598057001003));
#39203=CARTESIAN_POINT('Ctrl Pts',(21.3125219557939,-14.4091508971893,27.7463544749225));
#39204=CARTESIAN_POINT('Ctrl Pts',(21.3125219557939,-15.0282378072439,27.4248521776202));
#39205=CARTESIAN_POINT('Ctrl Pts',(21.3125219557939,-15.632368792237,27.0760569908086));
#39206=CARTESIAN_POINT('Ctrl Pts',(21.3125219557939,-42.7084257830456,11.4436881985716));
#39207=CARTESIAN_POINT('Ctrl Pts',(21.3125219557939,-27.0760569908086,-15.632368792237));
#39208=CARTESIAN_POINT('Ctrl Pts',(21.3125219557939,-11.4436881985716,-42.7084257830456));
#39209=CARTESIAN_POINT('Ctrl Pts',(21.3125219557939,15.632368792237,-27.0760569908086));
#39210=CARTESIAN_POINT('Ctrl Pts',(21.3125219557939,42.7084257830456,-11.4436881985716));
#39211=CARTESIAN_POINT('Ctrl Pts',(21.3125219557939,27.0760569908086,15.632368792237));
#39212=CARTESIAN_POINT('Ctrl Pts',(21.3125219557939,12.1260533880339,41.5265346055806));
#39213=CARTESIAN_POINT('Ctrl Pts',(21.3125219557939,-14.4091508971893,27.7463544749225));
#39214=CARTESIAN_POINT('Ctrl Pts',(20.0742472323676,-14.2719922102254,27.4822408172221));
#39215=CARTESIAN_POINT('Ctrl Pts',(20.0742472323676,-14.8851861187906,27.1637988552073));
#39216=CARTESIAN_POINT('Ctrl Pts',(20.0742472323676,-15.4835664656477,26.8183238008716));
#39217=CARTESIAN_POINT('Ctrl Pts',(20.0742472323676,-42.3018902665193,11.3347573352238));
#39218=CARTESIAN_POINT('Ctrl Pts',(20.0742472323676,-26.8183238008716,-15.4835664656477));
#39219=CARTESIAN_POINT('Ctrl Pts',(20.0742472323676,-11.3347573352238,-42.3018902665193));
#39220=CARTESIAN_POINT('Ctrl Pts',(20.0742472323676,15.4835664656477,-26.8183238008716));
#39221=CARTESIAN_POINT('Ctrl Pts',(20.0742472323676,42.3018902665193,-11.3347573352238));
#39222=CARTESIAN_POINT('Ctrl Pts',(20.0742472323676,26.8183238008716,15.4835664656477));
#39223=CARTESIAN_POINT('Ctrl Pts',(20.0742472323676,12.0106271861277,41.1312493454498));
#39224=CARTESIAN_POINT('Ctrl Pts',(20.0742472323676,-14.2719922102254,27.4822408172221));
#39225=CARTESIAN_POINT('Ctrl Pts',(18.7979917002302,-14.1614724492006,27.2694232481814));
#39226=CARTESIAN_POINT('Ctrl Pts',(18.7979917002302,-14.7699178935542,26.9534472438987));
#39227=CARTESIAN_POINT('Ctrl Pts',(18.7979917002302,-15.3636644897785,26.6106474867381));
#39228=CARTESIAN_POINT('Ctrl Pts',(18.7979917002302,-41.9743119765166,11.2469829969596));
#39229=CARTESIAN_POINT('Ctrl Pts',(18.7979917002302,-26.6106474867381,-15.3636644897785));
#39230=CARTESIAN_POINT('Ctrl Pts',(18.7979917002302,-11.2469829969596,-41.9743119765166));
#39231=CARTESIAN_POINT('Ctrl Pts',(18.7979917002302,15.3636644897785,-26.6106474867381));
#39232=CARTESIAN_POINT('Ctrl Pts',(18.7979917002302,41.9743119765166,-11.2469829969596));
#39233=CARTESIAN_POINT('Ctrl Pts',(18.7979917002302,26.6106474867381,15.3636644897785));
#39234=CARTESIAN_POINT('Ctrl Pts',(18.7979917002302,11.9176190323383,40.8127362898543));
#39235=CARTESIAN_POINT('Ctrl Pts',(18.7979917002302,-14.1614724492006,27.2694232481814));
#39236=CARTESIAN_POINT('Ctrl Pts',(17.4917404060759,-14.0757116526895,27.1042817018803));
#39237=CARTESIAN_POINT('Ctrl Pts',(17.4917404060759,-14.6804723978617,26.7902192241678));
#39238=CARTESIAN_POINT('Ctrl Pts',(17.4917404060759,-15.2706233100072,26.4494954361781));
#39239=CARTESIAN_POINT('Ctrl Pts',(17.4917404060759,-41.7201187461852,11.1788721261709));
#39240=CARTESIAN_POINT('Ctrl Pts',(17.4917404060759,-26.4494954361781,-15.2706233100072));
#39241=CARTESIAN_POINT('Ctrl Pts',(17.4917404060759,-11.1788721261709,-41.7201187461852));
#39242=CARTESIAN_POINT('Ctrl Pts',(17.4917404060759,15.2706233100072,-26.4494954361781));
#39243=CARTESIAN_POINT('Ctrl Pts',(17.4917404060759,41.7201187461852,-11.1788721261709));
#39244=CARTESIAN_POINT('Ctrl Pts',(17.4917404060759,26.4494954361781,15.2706233100072));
#39245=CARTESIAN_POINT('Ctrl Pts',(17.4917404060759,11.8454468408945,40.5655774732432));
#39246=CARTESIAN_POINT('Ctrl Pts',(17.4917404060759,-14.0757116526895,27.1042817018803));
#39247=CARTESIAN_POINT('Ctrl Pts',(16.1647270995715,-14.011024902894,26.9797204766935));
#39248=CARTESIAN_POINT('Ctrl Pts',(16.1647270995715,-14.6130063919992,26.6671013136366));
#39249=CARTESIAN_POINT('Ctrl Pts',(16.1647270995715,-15.2004451894511,26.3279433657953));
#39250=CARTESIAN_POINT('Ctrl Pts',(16.1647270995715,-41.5283885552464,11.1274981763442));
#39251=CARTESIAN_POINT('Ctrl Pts',(16.1647270995715,-26.3279433657953,-15.2004451894511));
#39252=CARTESIAN_POINT('Ctrl Pts',(16.1647270995715,-11.1274981763442,-41.5283885552464));
#39253=CARTESIAN_POINT('Ctrl Pts',(16.1647270995715,15.2004451894511,-26.3279433657953));
#39254=CARTESIAN_POINT('Ctrl Pts',(16.1647270995715,41.5283885552464,-11.1274981763442));
#39255=CARTESIAN_POINT('Ctrl Pts',(16.1647270995715,26.3279433657953,15.2004451894511));
#39256=CARTESIAN_POINT('Ctrl Pts',(16.1647270995715,11.7910095609247,40.3791531257526));
#39257=CARTESIAN_POINT('Ctrl Pts',(16.1647270995715,-14.011024902894,26.9797204766935));
#39258=CARTESIAN_POINT('Ctrl Pts',(14.8263876417415,-13.9627843740029,26.8868282012068));
#39259=CARTESIAN_POINT('Ctrl Pts',(14.8263876417415,-14.5626932163446,26.5752853986496));
#39260=CARTESIAN_POINT('Ctrl Pts',(14.8263876417415,-15.1481094381123,26.2372951854241));
#39261=CARTESIAN_POINT('Ctrl Pts',(14.8263876417415,-41.3854046235364,11.0891857473118));
#39262=CARTESIAN_POINT('Ctrl Pts',(14.8263876417415,-26.2372951854241,-15.1481094381123));
#39263=CARTESIAN_POINT('Ctrl Pts',(14.8263876417415,-11.0891857473118,-41.3854046235364));
#39264=CARTESIAN_POINT('Ctrl Pts',(14.8263876417415,15.1481094381123,-26.2372951854241));
#39265=CARTESIAN_POINT('Ctrl Pts',(14.8263876417415,41.3854046235364,-11.0891857473118));
#39266=CARTESIAN_POINT('Ctrl Pts',(14.8263876417415,26.2372951854241,15.1481094381123));
#39267=CARTESIAN_POINT('Ctrl Pts',(14.8263876417415,11.750412635195,40.2401260583921));
#39268=CARTESIAN_POINT('Ctrl Pts',(14.8263876417415,-13.9627843740029,26.8868282012068));
#39269=CARTESIAN_POINT('Ctrl Pts',(13.4853470903953,-13.926278703034,26.8165326442879));
#39270=CARTESIAN_POINT('Ctrl Pts',(13.4853470903953,-14.5246190849439,26.505804369746));
#39271=CARTESIAN_POINT('Ctrl Pts',(13.4853470903953,-15.1085047372063,26.1686978312363));
#39272=CARTESIAN_POINT('Ctrl Pts',(13.4853470903953,-41.2772025684426,11.0601930940301));
#39273=CARTESIAN_POINT('Ctrl Pts',(13.4853470903953,-26.1686978312363,-15.1085047372063));
#39274=CARTESIAN_POINT('Ctrl Pts',(13.4853470903953,-11.0601930940301,-41.2772025684426));
#39275=CARTESIAN_POINT('Ctrl Pts',(13.4853470903953,15.1085047372063,-26.1686978312363));
#39276=CARTESIAN_POINT('Ctrl Pts',(13.4853470903953,41.2772025684426,-11.0601930940301));
#39277=CARTESIAN_POINT('Ctrl Pts',(13.4853470903953,26.1686978312363,15.1085047372063));
#39278=CARTESIAN_POINT('Ctrl Pts',(13.4853470903953,11.7196912055776,40.1349183317465));
#39279=CARTESIAN_POINT('Ctrl Pts',(13.4853470903953,-13.926278703034,26.8165326442879));
#39280=CARTESIAN_POINT('Ctrl Pts',(12.1482076787549,-13.8976780812377,26.7614591013549));
#39281=CARTESIAN_POINT('Ctrl Pts',(12.1482076787549,-14.4947896419145,26.4513689744511));
#39282=CARTESIAN_POINT('Ctrl Pts',(12.1482076787549,-15.0774761588537,26.1149547570431));
#39283=CARTESIAN_POINT('Ctrl Pts',(12.1482076787549,-41.1924309158968,11.0374785981894));
#39284=CARTESIAN_POINT('Ctrl Pts',(12.1482076787549,-26.1149547570431,-15.0774761588537));
#39285=CARTESIAN_POINT('Ctrl Pts',(12.1482076787549,-11.0374785981894,-41.1924309158968));
#39286=CARTESIAN_POINT('Ctrl Pts',(12.1482076787549,15.0774761588537,-26.1149547570431));
#39287=CARTESIAN_POINT('Ctrl Pts',(12.1482076787549,41.1924309158968,-11.0374785981894));
#39288=CARTESIAN_POINT('Ctrl Pts',(12.1482076787549,26.1149547570431,15.0774761588537));
#39289=CARTESIAN_POINT('Ctrl Pts',(12.1482076787549,11.6956222878942,40.0524926066472));
#39290=CARTESIAN_POINT('Ctrl Pts',(12.1482076787549,-13.8976780812377,26.7614591013549));
#39291=CARTESIAN_POINT('Ctrl Pts',(10.8190675759626,-13.8744950717886,26.716817747915));
#39292=CARTESIAN_POINT('Ctrl Pts',(10.8190675759626,-14.4706105780977,26.4072448888814));
#39293=CARTESIAN_POINT('Ctrl Pts',(10.8190675759626,-15.0523251033884,26.0713918511132));
#39294=CARTESIAN_POINT('Ctrl Pts',(10.8190675759626,-41.1237169545017,11.0190667477248));
#39295=CARTESIAN_POINT('Ctrl Pts',(10.8190675759626,-26.0713918511132,-15.0523251033884));
#39296=CARTESIAN_POINT('Ctrl Pts',(10.8190675759626,-11.0190667477248,-41.1237169545017));
#39297=CARTESIAN_POINT('Ctrl Pts',(10.8190675759626,15.0523251033884,-26.0713918511132));
#39298=CARTESIAN_POINT('Ctrl Pts',(10.8190675759626,41.1237169545017,-11.0190667477248));
#39299=CARTESIAN_POINT('Ctrl Pts',(10.8190675759626,26.0713918511132,15.0523251033884));
#39300=CARTESIAN_POINT('Ctrl Pts',(10.8190675759626,11.6761125740823,39.9856802003493));
#39301=CARTESIAN_POINT('Ctrl Pts',(10.8190675759626,-13.8744950717886,26.716817747915));
#39302=CARTESIAN_POINT('Ctrl Pts',(9.50027713254189,-13.8551882149624,26.6796403391198));
#39303=CARTESIAN_POINT('Ctrl Pts',(9.50027713254189,-14.4504742051937,26.3704982618073));
#39304=CARTESIAN_POINT('Ctrl Pts',(9.50027713254189,-15.0313792538877,26.0351125755702));
#39305=CARTESIAN_POINT('Ctrl Pts',(9.50027713254189,-41.0664918294579,11.0037333216825));
#39306=CARTESIAN_POINT('Ctrl Pts',(9.50027713254189,-26.0351125755702,-15.0313792538877));
#39307=CARTESIAN_POINT('Ctrl Pts',(9.5002771325419,-11.0037333216825,-41.0664918294579));
#39308=CARTESIAN_POINT('Ctrl Pts',(9.5002771325419,15.0313792538877,-26.0351125755702));
#39309=CARTESIAN_POINT('Ctrl Pts',(9.5002771325419,41.0664918294579,-11.0037333216825));
#39310=CARTESIAN_POINT('Ctrl Pts',(9.50027713254189,26.0351125755702,15.0313792538877));
#39311=CARTESIAN_POINT('Ctrl Pts',(9.50027713254189,11.6598648452397,39.9300386942093));
#39312=CARTESIAN_POINT('Ctrl Pts',(9.50027713254189,-13.8551882149624,26.6796403391198));
#39313=CARTESIAN_POINT('Ctrl Pts',(8.45435372222587,-13.8422173352292,26.6546635289318));
#39314=CARTESIAN_POINT('Ctrl Pts',(8.45435372222587,-14.4369460336456,26.3458108626791));
#39315=CARTESIAN_POINT('Ctrl Pts',(8.45435372222587,-15.0173072536015,26.0107391561104));
#39316=CARTESIAN_POINT('Ctrl Pts',(8.45435372222587,-41.0280464097118,10.9934319025089));
#39317=CARTESIAN_POINT('Ctrl Pts',(8.45435372222587,-26.0107391561104,-15.0173072536015));
#39318=CARTESIAN_POINT('Ctrl Pts',(8.45435372222587,-10.9934319025089,-41.0280464097118));
#39319=CARTESIAN_POINT('Ctrl Pts',(8.45435372222587,15.0173072536015,-26.0107391561104));
#39320=CARTESIAN_POINT('Ctrl Pts',(8.45435372222587,41.0280464097118,-10.9934319025089));
#39321=CARTESIAN_POINT('Ctrl Pts',(8.45435372222587,26.0107391561104,15.0173072536015));
#39322=CARTESIAN_POINT('Ctrl Pts',(8.45435372222587,11.6489491721888,39.8926571933874));
#39323=CARTESIAN_POINT('Ctrl Pts',(8.45435372222587,-13.8422173352292,26.6546635289318));
#39324=CARTESIAN_POINT('Ctrl Pts',(7.67514864245731,-13.8337516775666,26.6383620035993));
#39325=CARTESIAN_POINT('Ctrl Pts',(7.67514864245731,-14.4281166503283,26.3296982262274));
#39326=CARTESIAN_POINT('Ctrl Pts',(7.67514864245731,-15.0081229315276,25.9948314436454));
#39327=CARTESIAN_POINT('Ctrl Pts',(7.67514864245731,-41.0029543751729,10.9867085121178));
#39328=CARTESIAN_POINT('Ctrl Pts',(7.67514864245731,-25.9948314436454,-15.0081229315276));
#39329=CARTESIAN_POINT('Ctrl Pts',(7.67514864245731,-10.9867085121178,-41.0029543751729));
#39330=CARTESIAN_POINT('Ctrl Pts',(7.67514864245731,15.0081229315276,-25.9948314436454));
#39331=CARTESIAN_POINT('Ctrl Pts',(7.67514864245731,41.0029543751729,-10.9867085121178));
#39332=CARTESIAN_POINT('Ctrl Pts',(7.67514864245731,25.9948314436454,15.0081229315276));
#39333=CARTESIAN_POINT('Ctrl Pts',(7.67514864245731,11.6418248789176,39.8682595430058));
#39334=CARTESIAN_POINT('Ctrl Pts',(7.67514864245731,-13.8337516775666,26.6383620035993));
#39335=CARTESIAN_POINT('Ctrl Pts',(7.15799654185577,-13.8286669632852,26.6285708447822));
#39336=CARTESIAN_POINT('Ctrl Pts',(7.15799654185577,-14.4228134720947,26.3200205194336));
#39337=CARTESIAN_POINT('Ctrl Pts',(7.15799654185577,-15.0026065670023,25.9852768200144));
#39338=CARTESIAN_POINT('Ctrl Pts',(7.15799654185577,-40.9878833870167,10.9826702530122));
#39339=CARTESIAN_POINT('Ctrl Pts',(7.15799654185577,-25.9852768200144,-15.0026065670023));
#39340=CARTESIAN_POINT('Ctrl Pts',(7.15799654185577,-10.9826702530122,-40.9878833870167));
#39341=CARTESIAN_POINT('Ctrl Pts',(7.15799654185577,15.0026065670023,-25.9852768200144));
#39342=CARTESIAN_POINT('Ctrl Pts',(7.15799654185577,40.9878833870167,-10.9826702530122));
#39343=CARTESIAN_POINT('Ctrl Pts',(7.15799654185577,25.9852768200144,15.0026065670023));
#39344=CARTESIAN_POINT('Ctrl Pts',(7.15799654185577,11.6375458261629,39.8536056216838));
#39345=CARTESIAN_POINT('Ctrl Pts',(7.15799654185577,-13.8286669632852,26.6285708447822));
#39346=CARTESIAN_POINT('Ctrl Pts',(6.9,-13.8262643576559,26.6239443717909));
#39347=CARTESIAN_POINT('Ctrl Pts',(6.9,-14.4203076388911,26.3154476542665));
#39348=CARTESIAN_POINT('Ctrl Pts',(6.9,-15.,25.9807621135332));
#39349=CARTESIAN_POINT('Ctrl Pts',(6.9,-40.9807621135331,10.9807621135332));
#39350=CARTESIAN_POINT('Ctrl Pts',(6.9,-25.9807621135332,-15.));
#39351=CARTESIAN_POINT('Ctrl Pts',(6.9,-10.9807621135332,-40.9807621135331));
#39352=CARTESIAN_POINT('Ctrl Pts',(6.9,15.,-25.9807621135332));
#39353=CARTESIAN_POINT('Ctrl Pts',(6.9,40.9807621135331,-10.9807621135332));
#39354=CARTESIAN_POINT('Ctrl Pts',(6.9,25.9807621135332,15.));
#39355=CARTESIAN_POINT('Ctrl Pts',(6.9,11.6355239079847,39.846681418688));
#39356=CARTESIAN_POINT('Ctrl Pts',(6.9,-13.8262643576559,26.6239443717909));
#39357=CARTESIAN_POINT('Ctrl Pts',(6.9,-29.194404870986,6.90555748864273));
#39358=CARTESIAN_POINT('Ctrl Pts',(7.85773098116326,-28.7583591297181,8.83308608050287));
#39359=CARTESIAN_POINT('Ctrl Pts',(8.88781981167334,-28.148927360677,10.6725495024415));
#39360=CARTESIAN_POINT('Ctrl Pts',(10.5914578196776,-26.9549567714738,13.4378975079049));
#39361=CARTESIAN_POINT('Ctrl Pts',(11.2365058953701,-26.4627511078989,14.4268759573926));
#39362=CARTESIAN_POINT('Ctrl Pts',(12.0558885382926,-25.8276163596339,15.5639851987506));
#39363=CARTESIAN_POINT('Ctrl Pts',(12.1875764958397,-25.7255677072203,15.7427052651201));
#39364=CARTESIAN_POINT('Ctrl Pts',(13.194901830313,-24.9407551262718,17.0880993664927));
#39365=CARTESIAN_POINT('Ctrl Pts',(14.2258982134098,-24.0748117650462,18.4224696507577));
#39366=CARTESIAN_POINT('Ctrl Pts',(18.2616480823244,-20.9914735836847,22.4465505568645));
#39367=CARTESIAN_POINT('Ctrl Pts',(21.0496416709525,-19.1084188222497,24.4970863377161));
#39368=CARTESIAN_POINT('Ctrl Pts',(25.8000196361138,-18.0798601480504,27.440416330328));
#39369=CARTESIAN_POINT('Ctrl Pts',(26.8976561124457,-18.1725012311874,27.9949084025612));
#39370=CARTESIAN_POINT('Ctrl Pts',(28.0045908801237,-18.293020318403,28.5110480063609));
#39371=CARTESIAN_POINT('Ctrl Pts',(28.5235971652406,-18.3760345677215,28.7375730360626));
#39372=CARTESIAN_POINT('Ctrl Pts',(29.0834839543824,-18.4629109750536,28.9821227669885));
#39373=CARTESIAN_POINT('Ctrl Pts',(29.1146288039499,-18.4676985487665,28.995750541561));
#39374=CARTESIAN_POINT('Ctrl Pts',(29.5949306848436,-18.5426905181125,29.2050975774362));
#39375=CARTESIAN_POINT('Ctrl Pts',(30.0492939924726,-18.6372599535756,29.3870260594868));
#39376=CARTESIAN_POINT('Ctrl Pts',(30.5,-18.7405179110273,29.559989655385));
#39377=CARTESIAN_POINT('Ctrl Pts',(6.45331003273164,-10.9133179225515,1.59669678622779));
#39378=CARTESIAN_POINT('Ctrl Pts',(7.20830533428676,-10.8283039351861,2.1627262104287));
#39379=CARTESIAN_POINT('Ctrl Pts',(7.99928962140321,-10.7080816105349,2.70879554626307));
#39380=CARTESIAN_POINT('Ctrl Pts',(9.76164489174099,-10.3736775708918,3.82718122480732));
#39381=CARTESIAN_POINT('Ctrl Pts',(10.7316587814816,-10.1362456656108,4.40082635509405));
#39382=CARTESIAN_POINT('Ctrl Pts',(12.6606926111663,-9.65961205419967,5.38563263712135));
#39383=CARTESIAN_POINT('Ctrl Pts',(13.6374431259542,-9.38360450626092,5.83915384029438));
#39384=CARTESIAN_POINT('Ctrl Pts',(14.8679539417017,-9.06165302613707,6.32358226998235));
#39385=CARTESIAN_POINT('Ctrl Pts',(15.8146186835336,-8.8086769516328,6.68453209751778));
#39386=CARTESIAN_POINT('Ctrl Pts',(16.7768279789013,-8.55011854625632,7.00516941257112));
#39387=CARTESIAN_POINT('Ctrl Pts',(18.442654946101,-8.14533972931256,7.48808598435168));
#39388=CARTESIAN_POINT('Ctrl Pts',(19.4151948753429,-7.90738588441827,7.72973898022675));
#39389=CARTESIAN_POINT('Ctrl Pts',(20.6328868119185,-7.66437297695775,7.97443640583065));
#39390=CARTESIAN_POINT('Ctrl Pts',(21.1054260060188,-7.57098863237667,8.06465516157011));
#39391=CARTESIAN_POINT('Ctrl Pts',(22.0544239964409,-7.39387592479574,8.22831938421076));
#39392=CARTESIAN_POINT('Ctrl Pts',(22.7836594350115,-7.27389266543028,8.33397294082328));
#39393=CARTESIAN_POINT('Ctrl Pts',(23.5025637456207,-7.17270583388463,8.42426711082611));
#39394=CARTESIAN_POINT('Ctrl Pts',(23.9756232708732,-7.10861034193446,8.47952646912231));
#39395=CARTESIAN_POINT('Ctrl Pts',(24.5702383273715,-7.03666681503315,8.53935462310099));
#39396=CARTESIAN_POINT('Ctrl Pts',(25.0506812637285,-6.98463603831072,8.58189400875859));
#39397=CARTESIAN_POINT('Ctrl Pts',(25.4117237717371,-6.94891133994711,8.61093616318075));
#39398=CARTESIAN_POINT('Ctrl Pts',(25.7132331301515,-6.92207219011225,8.63276690479109));
#39399=CARTESIAN_POINT('Ctrl Pts',(25.9243500189544,-6.90499555217227,8.64675417662557));
#39400=CARTESIAN_POINT('Ctrl Pts',(26.0449825351311,-6.895741659732,8.65437719289245));
#39401=CARTESIAN_POINT('Ctrl Pts',(26.1053107047437,-6.89128602190977,8.65806460962823));
#39402=CARTESIAN_POINT('Ctrl Pts',(26.5982868813563,-6.85557010312607,8.68771831234652));
#39403=CARTESIAN_POINT('Ctrl Pts',(27.5414448539119,-6.81230249083092,8.7222238682219));
#39404=CARTESIAN_POINT('Ctrl Pts',(28.5384718269748,-6.79157348079209,8.73742874004852));
#39405=CARTESIAN_POINT('Ctrl Pts',(29.1235718011012,-6.77903979219494,8.74727658763325));
#39406=CARTESIAN_POINT('Ctrl Pts',(29.281292582401,-6.77610142826291,8.74962231400058));
#39407=CARTESIAN_POINT('Ctrl Pts',(29.6033746665999,-6.77163194910168,8.75316560056408));
#39408=CARTESIAN_POINT('Ctrl Pts',(30.1682156581428,-6.76749797708627,8.75644680260451));
#39409=CARTESIAN_POINT('Ctrl Pts',(31.3151120085301,-6.77048174742394,8.75407681716344));
#39410=CARTESIAN_POINT('Ctrl Pts',(32.3203490755541,-6.78127046660758,8.7456273326708));
#39411=CARTESIAN_POINT('Ctrl Pts',(33.1676615322708,-6.78128357449781,8.7456218694399));
#39412=CARTESIAN_POINT('Ctrl Pts',(33.4948723279895,-6.78128505761796,8.74562133595171));
#39413=CARTESIAN_POINT('Ctrl Pts',(34.1541357431677,-6.78128770533522,8.74562028433969));
#39414=CARTESIAN_POINT('Ctrl Pts',(34.9760826079904,-6.78129612595841,8.7456170279898));
#39415=CARTESIAN_POINT('Ctrl Pts',(35.9636845487692,-6.78129958330353,8.74561567977431));
#39416=CARTESIAN_POINT('Ctrl Pts',(37.9383132355672,-6.7813043592495,8.745613828852));
#39417=CARTESIAN_POINT('Ctrl Pts',(39.5833333333333,-6.7813280023926,8.74560464293355));
#39418=CARTESIAN_POINT('Ctrl Pts',(40.9,-6.7813280023926,8.74560464293355));
#39419=CARTESIAN_POINT('Ctrl Pts',(6.63336813585096,-14.1980521881427,2.58998912169033));
#39420=CARTESIAN_POINT('Ctrl Pts',(7.389696336477,-14.0595388287459,3.32655463912721));
#39421=CARTESIAN_POINT('Ctrl Pts',(8.18035160561763,-13.8764440634215,4.03465273479121));
#39422=CARTESIAN_POINT('Ctrl Pts',(9.94163143861871,-13.3869575789582,5.47986851886094));
#39423=CARTESIAN_POINT('Ctrl Pts',(10.9109664605569,-13.0495988183286,6.21859686207519));
#39424=CARTESIAN_POINT('Ctrl Pts',(12.8334013836927,-12.3824387994051,7.47915893423736));
#39425=CARTESIAN_POINT('Ctrl Pts',(13.8089179831182,-12.0008911509523,8.05904353786122));
#39426=CARTESIAN_POINT('Ctrl Pts',(15.0306778911273,-11.5604290689694,8.67329495695322));
#39427=CARTESIAN_POINT('Ctrl Pts',(15.9745670647922,-11.2141745075895,9.13243737556315));
#39428=CARTESIAN_POINT('Ctrl Pts',(16.929544084173,-10.8635736365946,9.53704617981306));
#39429=CARTESIAN_POINT('Ctrl Pts',(18.5792362231986,-10.3171018918725,10.1451076803253));
#39430=CARTESIAN_POINT('Ctrl Pts',(19.5469773926758,-9.99640408637921,10.4493242965117));
#39431=CARTESIAN_POINT('Ctrl Pts',(20.7474295734277,-9.67172058444866,10.7549000186161));
#39432=CARTESIAN_POINT('Ctrl Pts',(21.2167794172895,-9.54637190554481,10.8681544802447));
#39433=CARTESIAN_POINT('Ctrl Pts',(22.1549843938465,-9.30976886072822,11.0724642143303));
#39434=CARTESIAN_POINT('Ctrl Pts',(22.8744776078269,-9.14996578827694,11.2039970972495));
#39435=CARTESIAN_POINT('Ctrl Pts',(23.5816077902765,-9.01558422395426,11.316201946695));
#39436=CARTESIAN_POINT('Ctrl Pts',(24.0500749276267,-8.9300835935144,11.3851612528795));
#39437=CARTESIAN_POINT('Ctrl Pts',(24.6365533946129,-8.83449183240035,11.4594652258085));
#39438=CARTESIAN_POINT('Ctrl Pts',(25.1102835291691,-8.76539275960638,11.5122699159732));
#39439=CARTESIAN_POINT('Ctrl Pts',(25.4658322439333,-8.71801358900149,11.5482688417074));
#39440=CARTESIAN_POINT('Ctrl Pts',(25.7624874136689,-8.6824463850995,11.5753180370235));
#39441=CARTESIAN_POINT('Ctrl Pts',(25.9700349923415,-8.65983585467444,11.592640163876));
#39442=CARTESIAN_POINT('Ctrl Pts',(26.0885791323133,-8.64758737376065,11.6020803597254));
#39443=CARTESIAN_POINT('Ctrl Pts',(26.1478525996408,-8.64169115913871,11.6066467500382));
#39444=CARTESIAN_POINT('Ctrl Pts',(26.6319130667266,-8.59444428954226,11.6433645250357));
#39445=CARTESIAN_POINT('Ctrl Pts',(27.5577774489369,-8.53717709311587,11.6860824768893));
#39446=CARTESIAN_POINT('Ctrl Pts',(28.5508423746858,-8.50942828058727,11.7050908260002));
#39447=CARTESIAN_POINT('Ctrl Pts',(29.1362159539423,-8.49263545125894,11.7174369518246));
#39448=CARTESIAN_POINT('Ctrl Pts',(29.2912819508841,-8.48875007883417,11.7203386713976));
#39449=CARTESIAN_POINT('Ctrl Pts',(29.610052998187,-8.48280581727731,11.7247475094471));
#39450=CARTESIAN_POINT('Ctrl Pts',(30.1693026775047,-8.47731190452096,11.728827902791));
#39451=CARTESIAN_POINT('Ctrl Pts',(31.3098786008463,-8.48127083805332,11.7258872894481));
#39452=CARTESIAN_POINT('Ctrl Pts',(32.3162827048883,-8.49575357359989,11.7152777874899));
#39453=CARTESIAN_POINT('Ctrl Pts',(33.1686195735697,-8.49577523975603,11.715269078277));
#39454=CARTESIAN_POINT('Ctrl Pts',(33.4952188807558,-8.49577770055114,11.7152682401723));
#39455=CARTESIAN_POINT('Ctrl Pts',(34.1547734244042,-8.49578208271197,11.7152665713231));
#39456=CARTESIAN_POINT('Ctrl Pts',(34.9764178792931,-8.49579602915746,11.7152614171757));
#39457=CARTESIAN_POINT('Ctrl Pts',(35.9640520550922,-8.49580175406157,11.7152592814565));
#39458=CARTESIAN_POINT('Ctrl Pts',(37.9385651163988,-8.49580966366,11.7152563511877));
#39459=CARTESIAN_POINT('Ctrl Pts',(39.5833333333333,-8.49584881729847,11.7152418049849));
#39460=CARTESIAN_POINT('Ctrl Pts',(40.9,-8.49584881729847,11.7152418049849));
#39461=CARTESIAN_POINT('Ctrl Pts',(6.84648239176542,-21.8719108775553,4.8711720049463));
#39462=CARTESIAN_POINT('Ctrl Pts',(7.61278097593421,-21.6080942034255,6.01809391809558));
#39463=CARTESIAN_POINT('Ctrl Pts',(8.41274152921387,-21.2759544371052,7.1129769401534));
#39464=CARTESIAN_POINT('Ctrl Pts',(10.1879716557546,-20.4198986989574,9.33526598964861));
#39465=CARTESIAN_POINT('Ctrl Pts',(11.1642573475929,-19.8462357742843,10.4645258845954));
#39466=CARTESIAN_POINT('Ctrl Pts',(13.1034321172788,-18.7228640453274,12.3837514736036));
#39467=CARTESIAN_POINT('Ctrl Pts',(14.0822646095709,-18.0925354910949,13.259092905625));
#39468=CARTESIAN_POINT('Ctrl Pts',(15.3084001581867,-17.369341405527,14.1807147676625));
#39469=CARTESIAN_POINT('Ctrl Pts',(16.2531227144981,-16.8032299545452,14.8695159890908));
#39470=CARTESIAN_POINT('Ctrl Pts',(17.2084375604977,-16.2348330754283,15.4708786153412));
#39471=CARTESIAN_POINT('Ctrl Pts',(18.8473961588579,-15.3570672461537,16.3684102669437));
#39472=CARTESIAN_POINT('Ctrl Pts',(19.8110405035782,-14.8437940564497,16.8164458459158));
#39473=CARTESIAN_POINT('Ctrl Pts',(20.9872655006161,-14.3329359049567,17.2594998647324));
#39474=CARTESIAN_POINT('Ctrl Pts',(21.4517346237735,-14.1338378277512,17.4254488483262));
#39475=CARTESIAN_POINT('Ctrl Pts',(22.3727984841465,-13.7614448137588,17.72174912934));
#39476=CARTESIAN_POINT('Ctrl Pts',(23.0743543377562,-13.5118529399622,17.9111527143536));
#39477=CARTESIAN_POINT('Ctrl Pts',(23.7582742987066,-13.3034745440381,18.0719640430563));
#39478=CARTESIAN_POINT('Ctrl Pts',(24.2174386855896,-13.1693266480668,18.1719103336479));
#39479=CARTESIAN_POINT('Ctrl Pts',(24.787021394359,-13.0207037868382,18.278521814341));
#39480=CARTESIAN_POINT('Ctrl Pts',(25.2463470121637,-12.9133861579984,18.3542161979474));
#39481=CARTESIAN_POINT('Ctrl Pts',(25.5899787396422,-12.840037267054,18.4056632423989));
#39482=CARTESIAN_POINT('Ctrl Pts',(25.8759048428227,-12.7850917865306,18.4442660174723));
#39483=CARTESIAN_POINT('Ctrl Pts',(26.0755068065032,-12.7502361709815,18.4689567859643));
#39484=CARTESIAN_POINT('Ctrl Pts',(26.1893780149132,-12.7313725692329,18.4824083304414));
#39485=CARTESIAN_POINT('Ctrl Pts',(26.2462863876023,-12.7222969574596,18.4889145361422));
#39486=CARTESIAN_POINT('Ctrl Pts',(26.7102722067275,-12.6496548741739,18.5411896593431));
#39487=CARTESIAN_POINT('Ctrl Pts',(27.5960905386888,-12.5614420302556,18.6020458648122));
#39488=CARTESIAN_POINT('Ctrl Pts',(28.5798438027286,-12.5173520665108,18.629899960324));
#39489=CARTESIAN_POINT('Ctrl Pts',(29.1658297917577,-12.4906249890439,18.6480680632814));
#39490=CARTESIAN_POINT('Ctrl Pts',(29.3147155528138,-12.4846522276656,18.6521962493032));
#39491=CARTESIAN_POINT('Ctrl Pts',(29.6257654938391,-12.4753713397182,18.6585637397073));
#39492=CARTESIAN_POINT('Ctrl Pts',(30.1719616098277,-12.4668129248999,18.6644443298454));
#39493=CARTESIAN_POINT('Ctrl Pts',(31.2977738410334,-12.472961188488,18.6602190141086));
#39494=CARTESIAN_POINT('Ctrl Pts',(32.3068669150108,-12.4961463862897,18.6445149503826));
#39495=CARTESIAN_POINT('Ctrl Pts',(33.1709127040733,-12.4962026881972,18.6444874715366));
#39496=CARTESIAN_POINT('Ctrl Pts',(33.4960830255434,-12.4962093123004,18.644484418038));
#39497=CARTESIAN_POINT('Ctrl Pts',(34.1563135822162,-12.4962208405724,18.6444789016084));
#39498=CARTESIAN_POINT('Ctrl Pts',(34.9772414248899,-12.4962577684095,18.6444614154564));
#39499=CARTESIAN_POINT('Ctrl Pts',(35.964946372113,-12.496272896639,18.6444542286038));
#39500=CARTESIAN_POINT('Ctrl Pts',(37.9391834323222,-12.4962938290757,18.6444443083029));
#39501=CARTESIAN_POINT('Ctrl Pts',(39.5833333333333,-12.4963973854122,18.6443951831047));
#39502=CARTESIAN_POINT('Ctrl Pts',(40.9,-12.4963973854122,18.6443951831047));
#39503=CARTESIAN_POINT('Ctrl Pts',(6.90857970435318,-29.5800408844791,7.02038826853569));
#39504=CARTESIAN_POINT('Ctrl Pts',(7.67983757144493,-29.1962153577801,8.58577901088989));
#39505=CARTESIAN_POINT('Ctrl Pts',(8.4844629659692,-28.7191114013952,10.0765485557758));
#39506=CARTESIAN_POINT('Ctrl Pts',(10.2687526859613,-27.5023711977385,13.0935628879538));
#39507=CARTESIAN_POINT('Ctrl Pts',(11.2489627292759,-26.6949552438923,14.6224501564806));
#39508=CARTESIAN_POINT('Ctrl Pts',(13.2065810728343,-25.1069038454383,17.2294066625499));
#39509=CARTESIAN_POINT('Ctrl Pts',(14.188432579866,-24.2271697832519,18.4069952853951));
#39510=CARTESIAN_POINT('Ctrl Pts',(15.4296983589676,-23.2080338536349,19.6550892131211));
#39511=CARTESIAN_POINT('Ctrl Pts',(16.3788042670987,-22.4189011948389,20.5796860932724));
#39512=CARTESIAN_POINT('Ctrl Pts',(17.3450159165718,-21.6217224592711,21.3903231452907));
#39513=CARTESIAN_POINT('Ctrl Pts',(18.9999962645463,-20.3951481814249,22.5937460627635));
#39514=CARTESIAN_POINT('Ctrl Pts',(19.9686658165166,-19.6835411202359,23.189805412739));
#39515=CARTESIAN_POINT('Ctrl Pts',(21.1489437168842,-18.9783964629487,23.775691048575));
#39516=CARTESIAN_POINT('Ctrl Pts',(21.6136662410168,-18.7043064424586,23.9949385633154));
#39517=CARTESIAN_POINT('Ctrl Pts',(22.5341605437883,-18.1932305660767,24.3846521737584));
#39518=CARTESIAN_POINT('Ctrl Pts',(23.2310352415765,-17.8537326154788,24.6315178872712));
#39519=CARTESIAN_POINT('Ctrl Pts',(23.9047680627613,-17.5731511638353,24.839431592137));
#39520=CARTESIAN_POINT('Ctrl Pts',(24.3593217251596,-17.3912549800692,24.9695871891304));
#39521=CARTESIAN_POINT('Ctrl Pts',(24.9191284505011,-17.1917285847409,25.1069751863361));
#39522=CARTESIAN_POINT('Ctrl Pts',(25.3687829483029,-17.0482631873595,25.2041659752938));
#39523=CARTESIAN_POINT('Ctrl Pts',(25.7038809466243,-16.9507036504245,25.2699171894924));
#39524=CARTESIAN_POINT('Ctrl Pts',(25.9815275275383,-16.8779731233106,25.3190677310926));
#39525=CARTESIAN_POINT('Ctrl Pts',(26.1747255747312,-16.8320233777013,25.3504124116981));
#39526=CARTESIAN_POINT('Ctrl Pts',(26.2847430019944,-16.8072090098455,25.367466019553));
#39527=CARTESIAN_POINT('Ctrl Pts',(26.3396756125256,-16.7952849898387,25.3757090167857));
#39528=CARTESIAN_POINT('Ctrl Pts',(26.7867185605552,-16.7000344271699,25.4418392909477));
#39529=CARTESIAN_POINT('Ctrl Pts',(27.6343089133552,-16.5847364280864,25.5185659559044));
#39530=CARTESIAN_POINT('Ctrl Pts',(28.6086204191332,-16.5243820587324,25.5552242576155));
#39531=CARTESIAN_POINT('Ctrl Pts',(29.1952293795949,-16.4877244301025,25.5792110357046));
#39532=CARTESIAN_POINT('Ctrl Pts',(29.3380035933319,-16.4799452423709,25.584403327273));
#39533=CARTESIAN_POINT('Ctrl Pts',(29.6413717635321,-16.4675695714433,25.5925899885791));
#39534=CARTESIAN_POINT('Ctrl Pts',(30.174536806517,-16.4561967872262,25.6001268754995));
#39535=CARTESIAN_POINT('Ctrl Pts',(31.2855894033322,-16.464330041984,25.5947346655064));
#39536=CARTESIAN_POINT('Ctrl Pts',(32.2974015084455,-16.4964013295029,25.5738307704501));
#39537=CARTESIAN_POINT('Ctrl Pts',(33.1731651112183,-16.4965224425527,25.5737672879574));
#39538=CARTESIAN_POINT('Ctrl Pts',(33.4969081472872,-16.4965369996129,25.5737598716201));
#39539=CARTESIAN_POINT('Ctrl Pts',(34.157816939104,-16.4965619872359,25.5737469053195));
#39540=CARTESIAN_POINT('Ctrl Pts',(34.9780359591179,-16.496642344611,25.5737054251287));
#39541=CARTESIAN_POINT('Ctrl Pts',(35.9658147840134,-16.4966752246753,25.5736884251096));
#39542=CARTESIAN_POINT('Ctrl Pts',(37.9397802282712,-16.4967207607426,25.5736649097449));
#39543=CARTESIAN_POINT('Ctrl Pts',(39.5833333333333,-16.4969459535258,25.5735485612246));
#39544=CARTESIAN_POINT('Ctrl Pts',(40.9,-16.4969459535258,25.5735485612246));
#39545=CARTESIAN_POINT('Ctrl Pts',(6.93528330520032,-33.9890447223856,8.231730283379));
#39546=CARTESIAN_POINT('Ctrl Pts',(7.70864561497005,-33.5376786188307,10.0357116563145));
#39547=CARTESIAN_POINT('Ctrl Pts',(8.51532719250786,-32.9786927413523,11.7528338486872));
#39548=CARTESIAN_POINT('Ctrl Pts',(10.3033707684643,-31.5578840442132,15.2242195800702));
#39549=CARTESIAN_POINT('Ctrl Pts',(11.285359425586,-30.6179424293772,16.9818886494149));
#39550=CARTESIAN_POINT('Ctrl Pts',(13.2503075123955,-28.7660858779662,19.9828238609275));
#39551=CARTESIAN_POINT('Ctrl Pts',(14.2335802328307,-27.744590382611,21.333808720003));
#39552=CARTESIAN_POINT('Ctrl Pts',(15.4809874764708,-26.5562215055806,22.7701484639684));
#39553=CARTESIAN_POINT('Ctrl Pts',(16.4318967140333,-25.6398645222148,23.8303538982284));
#39554=CARTESIAN_POINT('Ctrl Pts',(17.4027860882062,-24.7114068344531,24.7620955812504));
#39555=CARTESIAN_POINT('Ctrl Pts',(19.0657008739464,-23.2827894621994,26.1438767914272));
#39556=CARTESIAN_POINT('Ctrl Pts',(20.0370987955264,-22.4568785783625,26.8257745442828));
#39557=CARTESIAN_POINT('Ctrl Pts',(21.221937368182,-21.6368752952082,27.4963832022123));
#39558=CARTESIAN_POINT('Ctrl Pts',(21.6873545199149,-21.319265575768,27.7466423667128));
#39559=CARTESIAN_POINT('Ctrl Pts',(22.6095407883917,-20.7266792263567,28.1914275999319));
#39560=CARTESIAN_POINT('Ctrl Pts',(23.3063195468722,-20.3342063552501,28.4721721598035));
#39561=CARTESIAN_POINT('Ctrl Pts',(23.9774915837903,-20.0111563083467,28.7077527668382));
#39562=CARTESIAN_POINT('Ctrl Pts',(24.4307021142577,-19.8016082531844,28.8553793495039));
#39563=CARTESIAN_POINT('Ctrl Pts',(24.9871188326864,-19.5726095610121,29.010562613784));
#39564=CARTESIAN_POINT('Ctrl Pts',(25.4329141726817,-19.4084486444525,29.1200357132468));
#39565=CARTESIAN_POINT('Ctrl Pts',(25.76439505547,-19.2971155191109,29.1939083663027));
#39566=CARTESIAN_POINT('Ctrl Pts',(26.0382972138579,-19.2143910494176,29.2489718106942));
#39567=CARTESIAN_POINT('Ctrl Pts',(26.2284820979137,-19.1622606931672,29.284017210513));
#39568=CARTESIAN_POINT('Ctrl Pts',(26.3366494455064,-19.1341507449288,29.3030632173398));
#39569=CARTESIAN_POINT('Ctrl Pts',(26.3906225284368,-19.1206543727099,29.3122642693068));
#39570=CARTESIAN_POINT('Ctrl Pts',(26.8293654116034,-19.0129885834593,29.3859982106892));
#39571=CARTESIAN_POINT('Ctrl Pts',(27.6560988760145,-18.8833816200194,29.4710985842867));
#39572=CARTESIAN_POINT('Ctrl Pts',(28.6249317030318,-18.8137794716616,29.5127595133998));
#39573=CARTESIAN_POINT('Ctrl Pts',(29.2119052185273,-18.7714558506415,29.5400636810177));
#39574=CARTESIAN_POINT('Ctrl Pts',(29.351223493954,-18.7627335234215,29.5458124634024));
#39575=CARTESIAN_POINT('Ctrl Pts',(29.6502234545151,-18.7486685476099,29.5549926880432));
#39576=CARTESIAN_POINT('Ctrl Pts',(30.1759548990665,-18.7357718416967,29.5634265890421));
#39577=CARTESIAN_POINT('Ctrl Pts',(31.2785766862301,-18.7449771625331,29.5574021311857));
#39578=CARTESIAN_POINT('Ctrl Pts',(32.2919610610309,-18.7821959068194,29.5334837411524));
#39579=CARTESIAN_POINT('Ctrl Pts',(33.1744263360525,-18.7823679845324,29.533390407254));
#39580=CARTESIAN_POINT('Ctrl Pts',(33.4973548461808,-18.7823889294252,29.5333792377699));
#39581=CARTESIAN_POINT('Ctrl Pts',(34.1586526208335,-18.7824245927187,29.5333600113094));
#39582=CARTESIAN_POINT('Ctrl Pts',(34.978471543808,-18.7825395490483,29.5332982308031));
#39583=CARTESIAN_POINT('Ctrl Pts',(35.9662945600334,-18.7825865524221,29.5332729456428));
#39584=CARTESIAN_POINT('Ctrl Pts',(37.9401075800399,-18.7826516826344,29.533237934286));
#39585=CARTESIAN_POINT('Ctrl Pts',(39.5833333333333,-18.7829737067337,29.533064777293));
#39586=CARTESIAN_POINT('Ctrl Pts',(40.9,-18.7829737067337,29.533064777293));
#39587=CARTESIAN_POINT('Origin',(6.9,1.83697019872103E-15,30.));
#39588=CARTESIAN_POINT('',(6.9,-21.8303175223207,20.5775906479515));
#39589=CARTESIAN_POINT('Ctrl Pts',(6.9,-8.44145532612415,7.09789564133157));
#39590=CARTESIAN_POINT('Ctrl Pts',(6.9,-11.09468188726,9.87986401752105));
#39591=CARTESIAN_POINT('Ctrl Pts',(6.90000000166257,-13.9485622548227,12.753513475675));
#39592=CARTESIAN_POINT('Ctrl Pts',(6.90000000166257,-18.0885125115534,16.8843019432417));
#39593=CARTESIAN_POINT('Ctrl Pts',(6.9,-19.9691972794379,18.7449692586141));
#39594=CARTESIAN_POINT('Ctrl Pts',(6.9,-21.8303175223207,20.5775906479515));
#39595=CARTESIAN_POINT('Origin',(6.9,0.,0.));
#39596=CARTESIAN_POINT('Origin',(40.9,5.51091059616309E-16,9.));
#39597=CARTESIAN_POINT('Ctrl Pts',(40.9,-1.5,34.4673758792282));
#39598=CARTESIAN_POINT('Ctrl Pts',(40.9,-1.5,33.9668810740701));
#39599=CARTESIAN_POINT('Ctrl Pts',(40.9,-1.5,33.466386268912));
#39600=CARTESIAN_POINT('Ctrl Pts',(40.9,-1.5,32.9658914637539));
#39601=CARTESIAN_POINT('Ctrl Pts',(30.5,1.56108868151375,34.9651684126997));
#39602=CARTESIAN_POINT('Ctrl Pts',(30.5,0.780932928377882,35.));
#39603=CARTESIAN_POINT('Ctrl Pts',(30.5,2.14313189850787E-15,35.));
#39604=CARTESIAN_POINT('Ctrl Pts',(30.5,-35.,35.));
#39605=CARTESIAN_POINT('Ctrl Pts',(30.5,-35.,2.14313189850787E-15));
#39606=CARTESIAN_POINT('Ctrl Pts',(30.5,-35.,-35.));
#39607=CARTESIAN_POINT('Ctrl Pts',(30.5,-2.14313189850787E-15,-35.));
#39608=CARTESIAN_POINT('Ctrl Pts',(30.5,35.,-35.));
#39609=CARTESIAN_POINT('Ctrl Pts',(30.5,35.,-2.14313189850787E-15));
#39610=CARTESIAN_POINT('Ctrl Pts',(30.5,35.,33.472222479613));
#39611=CARTESIAN_POINT('Ctrl Pts',(30.5,1.56108868151375,34.9651684126997));
#39612=CARTESIAN_POINT('Ctrl Pts',(30.3311478274255,1.55772383604587,34.8898028105656));
#39613=CARTESIAN_POINT('Ctrl Pts',(30.3311478274255,0.779249668063536,34.924559320191));
#39614=CARTESIAN_POINT('Ctrl Pts',(30.3311478274255,2.13851248915519E-15,
34.924559320191));
#39615=CARTESIAN_POINT('Ctrl Pts',(30.3311478274255,-34.924559320191,34.924559320191));
#39616=CARTESIAN_POINT('Ctrl Pts',(30.3311478274255,-34.924559320191,2.13851248915519E-15));
#39617=CARTESIAN_POINT('Ctrl Pts',(30.3311478274255,-34.924559320191,-34.924559320191));
#39618=CARTESIAN_POINT('Ctrl Pts',(30.3311478274255,-2.13851248915519E-15,
-34.924559320191));
#39619=CARTESIAN_POINT('Ctrl Pts',(30.3311478274255,34.924559320191,-34.924559320191));
#39620=CARTESIAN_POINT('Ctrl Pts',(30.3311478274255,34.924559320191,-2.13851248915519E-15));
#39621=CARTESIAN_POINT('Ctrl Pts',(30.3311478274255,34.924559320191,33.4000748447964));
#39622=CARTESIAN_POINT('Ctrl Pts',(30.3311478274255,1.55772383604587,34.8898028105656));
#39623=CARTESIAN_POINT('Ctrl Pts',(29.9897712690917,1.55090794481747,34.7371408974366));
#39624=CARTESIAN_POINT('Ctrl Pts',(29.9897712690917,0.775840025831459,34.7717453283792));
#39625=CARTESIAN_POINT('Ctrl Pts',(29.9897712690917,2.12915533085832E-15,
34.7717453283792));
#39626=CARTESIAN_POINT('Ctrl Pts',(29.9897712690917,-34.7717453283791,34.7717453283791));
#39627=CARTESIAN_POINT('Ctrl Pts',(29.9897712690917,-34.7717453283792,2.12915533085832E-15));
#39628=CARTESIAN_POINT('Ctrl Pts',(29.9897712690917,-34.7717453283791,-34.7717453283791));
#39629=CARTESIAN_POINT('Ctrl Pts',(29.9897712690917,-2.12915533085832E-15,
-34.7717453283792));
#39630=CARTESIAN_POINT('Ctrl Pts',(29.9897712690917,34.7717453283791,-34.7717453283791));
#39631=CARTESIAN_POINT('Ctrl Pts',(29.9897712690917,34.7717453283792,-2.12915533085832E-15));
#39632=CARTESIAN_POINT('Ctrl Pts',(29.9897712690917,34.7717453283791,33.2539313038843));
#39633=CARTESIAN_POINT('Ctrl Pts',(29.9897712690917,1.55090794481747,34.7371408974366));
#39634=CARTESIAN_POINT('Ctrl Pts',(29.4666899049319,1.54042548027394,34.5023553003819));
#39635=CARTESIAN_POINT('Ctrl Pts',(29.4666899049319,0.770596184255045,34.5367258427036));
#39636=CARTESIAN_POINT('Ctrl Pts',(29.4666899049319,2.11476453781483E-15,
34.5367258427036));
#39637=CARTESIAN_POINT('Ctrl Pts',(29.4666899049319,-34.5367258427036,34.5367258427036));
#39638=CARTESIAN_POINT('Ctrl Pts',(29.4666899049319,-34.5367258427036,2.11476453781483E-15));
#39639=CARTESIAN_POINT('Ctrl Pts',(29.4666899049319,-34.5367258427036,-34.5367258427036));
#39640=CARTESIAN_POINT('Ctrl Pts',(29.4666899049319,-2.11476453781483E-15,
-34.5367258427036));
#39641=CARTESIAN_POINT('Ctrl Pts',(29.4666899049319,34.5367258427036,-34.5367258427036));
#39642=CARTESIAN_POINT('Ctrl Pts',(29.4666899049319,34.5367258427036,-2.11476453781483E-15));
#39643=CARTESIAN_POINT('Ctrl Pts',(29.4666899049319,34.5367258427036,33.0291706035535));
#39644=CARTESIAN_POINT('Ctrl Pts',(29.4666899049319,1.54042548027394,34.5023553003819));
#39645=CARTESIAN_POINT('Ctrl Pts',(28.7471241621752,1.52592972576568,34.1776802811774));
#39646=CARTESIAN_POINT('Ctrl Pts',(28.7471241621752,0.763344698704457,34.21172738887));
#39647=CARTESIAN_POINT('Ctrl Pts',(28.7471241621752,2.09486412200407E-15,
34.21172738887));
#39648=CARTESIAN_POINT('Ctrl Pts',(28.7471241621752,-34.2117273888699,34.2117273888699));
#39649=CARTESIAN_POINT('Ctrl Pts',(28.7471241621752,-34.21172738887,2.09486412200407E-15));
#39650=CARTESIAN_POINT('Ctrl Pts',(28.7471241621752,-34.2117273888699,-34.2117273888699));
#39651=CARTESIAN_POINT('Ctrl Pts',(28.7471241621752,-2.09486412200407E-15,
-34.21172738887));
#39652=CARTESIAN_POINT('Ctrl Pts',(28.7471241621752,34.2117273888699,-34.2117273888699));
#39653=CARTESIAN_POINT('Ctrl Pts',(28.7471241621752,34.21172738887,-2.09486412200407E-15));
#39654=CARTESIAN_POINT('Ctrl Pts',(28.7471241621752,34.2117273888699,32.718358587775));
#39655=CARTESIAN_POINT('Ctrl Pts',(28.7471241621752,1.52592972576568,34.1776802811774));
#39656=CARTESIAN_POINT('Ctrl Pts',(27.8100958442934,1.50698029472894,33.7532520886149));
#39657=CARTESIAN_POINT('Ctrl Pts',(27.8100958442934,0.753865266276396,33.7868763896026));
#39658=CARTESIAN_POINT('Ctrl Pts',(27.8100958442934,2.06884950118571E-15,
33.7868763896026));
#39659=CARTESIAN_POINT('Ctrl Pts',(27.8100958442934,-33.7868763896026,33.7868763896026));
#39660=CARTESIAN_POINT('Ctrl Pts',(27.8100958442934,-33.7868763896026,2.06884950118571E-15));
#39661=CARTESIAN_POINT('Ctrl Pts',(27.8100958442934,-33.7868763896026,-33.7868763896026));
#39662=CARTESIAN_POINT('Ctrl Pts',(27.8100958442934,-2.06884950118571E-15,
-33.7868763896026));
#39663=CARTESIAN_POINT('Ctrl Pts',(27.8100958442934,33.7868763896026,-33.7868763896026));
#39664=CARTESIAN_POINT('Ctrl Pts',(27.8100958442934,33.7868763896026,-2.06884950118571E-15));
#39665=CARTESIAN_POINT('Ctrl Pts',(27.8100958442934,33.7868763896026,32.3120526686846));
#39666=CARTESIAN_POINT('Ctrl Pts',(27.8100958442934,1.50698029472894,33.7532520886149));
#39667=CARTESIAN_POINT('Ctrl Pts',(26.8343111708818,1.48733431337754,33.3132226048841));
#39668=CARTESIAN_POINT('Ctrl Pts',(26.8343111708818,0.744037385305068,33.3464085574791));
#39669=CARTESIAN_POINT('Ctrl Pts',(26.8343111708818,2.04187862514883E-15,
33.3464085574791));
#39670=CARTESIAN_POINT('Ctrl Pts',(26.8343111708818,-33.3464085574791,33.3464085574791));
#39671=CARTESIAN_POINT('Ctrl Pts',(26.8343111708818,-33.3464085574791,2.04187862514883E-15));
#39672=CARTESIAN_POINT('Ctrl Pts',(26.8343111708818,-33.3464085574791,-33.3464085574791));
#39673=CARTESIAN_POINT('Ctrl Pts',(26.8343111708818,-2.04187862514883E-15,
-33.3464085574791));
#39674=CARTESIAN_POINT('Ctrl Pts',(26.8343111708818,33.3464085574791,-33.3464085574791));
#39675=CARTESIAN_POINT('Ctrl Pts',(26.8343111708818,33.3464085574791,-2.04187862514883E-15));
#39676=CARTESIAN_POINT('Ctrl Pts',(26.8343111708818,33.3464085574791,31.8908116037717));
#39677=CARTESIAN_POINT('Ctrl Pts',(26.8343111708818,1.48733431337754,33.3132226048841));
#39678=CARTESIAN_POINT('Ctrl Pts',(25.8181479469611,1.46726916269953,32.8638045923198));
#39679=CARTESIAN_POINT('Ctrl Pts',(25.8181479469611,0.733999815330425,32.8965428438611));
#39680=CARTESIAN_POINT('Ctrl Pts',(25.8181479469611,2.01433229483741E-15,
32.8965428438611));
#39681=CARTESIAN_POINT('Ctrl Pts',(25.8181479469611,-32.896542843861,32.896542843861));
#39682=CARTESIAN_POINT('Ctrl Pts',(25.8181479469611,-32.8965428438611,2.01433229483741E-15));
#39683=CARTESIAN_POINT('Ctrl Pts',(25.8181479469611,-32.896542843861,-32.896542843861));
#39684=CARTESIAN_POINT('Ctrl Pts',(25.8181479469611,-2.01433229483741E-15,
-32.8965428438611));
#39685=CARTESIAN_POINT('Ctrl Pts',(25.8181479469611,32.896542843861,-32.896542843861));
#39686=CARTESIAN_POINT('Ctrl Pts',(25.8181479469611,32.8965428438611,-2.01433229483741E-15));
#39687=CARTESIAN_POINT('Ctrl Pts',(25.8181479469611,32.896542843861,31.4605828822811));
#39688=CARTESIAN_POINT('Ctrl Pts',(25.8181479469611,1.46726916269953,32.8638045923198));
#39689=CARTESIAN_POINT('Ctrl Pts',(24.7595197917227,1.44728584082668,32.4162193763075));
#39690=CARTESIAN_POINT('Ctrl Pts',(24.7595197917227,0.724003180127257,32.4485117525897));
#39691=CARTESIAN_POINT('Ctrl Pts',(24.7595197917227,1.98689830274521E-15,
32.4485117525897));
#39692=CARTESIAN_POINT('Ctrl Pts',(24.7595197917227,-32.4485117525897,32.4485117525897));
#39693=CARTESIAN_POINT('Ctrl Pts',(24.7595197917227,-32.4485117525897,1.98689830274521E-15));
#39694=CARTESIAN_POINT('Ctrl Pts',(24.7595197917227,-32.4485117525897,-32.4485117525897));
#39695=CARTESIAN_POINT('Ctrl Pts',(24.7595197917227,-1.98689830274521E-15,
-32.4485117525897));
#39696=CARTESIAN_POINT('Ctrl Pts',(24.7595197917227,32.4485117525897,-32.4485117525897));
#39697=CARTESIAN_POINT('Ctrl Pts',(24.7595197917227,32.4485117525897,-1.98689830274521E-15));
#39698=CARTESIAN_POINT('Ctrl Pts',(24.7595197917227,32.4485117525897,31.0321087004291));
#39699=CARTESIAN_POINT('Ctrl Pts',(24.7595197917227,1.44728584082668,32.4162193763075));
#39700=CARTESIAN_POINT('Ctrl Pts',(23.6563574780851,1.42804494464108,31.9852629652417));
#39701=CARTESIAN_POINT('Ctrl Pts',(23.6563574780851,0.714377942573,32.017126031541));
#39702=CARTESIAN_POINT('Ctrl Pts',(23.6563574780851,1.9604835456212E-15,
32.017126031541));
#39703=CARTESIAN_POINT('Ctrl Pts',(23.6563574780851,-32.017126031541,32.017126031541));
#39704=CARTESIAN_POINT('Ctrl Pts',(23.6563574780851,-32.017126031541,1.9604835456212E-15));
#39705=CARTESIAN_POINT('Ctrl Pts',(23.6563574780851,-32.017126031541,-32.017126031541));
#39706=CARTESIAN_POINT('Ctrl Pts',(23.6563574780851,-1.9604835456212E-15,
-32.017126031541));
#39707=CARTESIAN_POINT('Ctrl Pts',(23.6563574780851,32.017126031541,-32.017126031541));
#39708=CARTESIAN_POINT('Ctrl Pts',(23.6563574780851,32.017126031541,-1.9604835456212E-15));
#39709=CARTESIAN_POINT('Ctrl Pts',(23.6563574780851,32.017126031541,30.6195533053014));
#39710=CARTESIAN_POINT('Ctrl Pts',(23.6563574780851,1.42804494464108,31.9852629652417));
#39711=CARTESIAN_POINT('Ctrl Pts',(22.5073180101405,1.41024006077928,31.5864702700101));
#39712=CARTESIAN_POINT('Ctrl Pts',(22.5073180101405,0.70547106863414,31.6179360671638));
#39713=CARTESIAN_POINT('Ctrl Pts',(22.5073180101405,1.93604021001489E-15,
31.6179360671638));
#39714=CARTESIAN_POINT('Ctrl Pts',(22.5073180101405,-31.6179360671638,31.6179360671638));
#39715=CARTESIAN_POINT('Ctrl Pts',(22.5073180101405,-31.6179360671638,1.93604021001489E-15));
#39716=CARTESIAN_POINT('Ctrl Pts',(22.5073180101405,-31.6179360671638,-31.6179360671638));
#39717=CARTESIAN_POINT('Ctrl Pts',(22.5073180101405,-1.93604021001489E-15,
-31.6179360671638));
#39718=CARTESIAN_POINT('Ctrl Pts',(22.5073180101405,31.6179360671638,-31.6179360671638));
#39719=CARTESIAN_POINT('Ctrl Pts',(22.5073180101405,31.6179360671638,-1.93604021001489E-15));
#39720=CARTESIAN_POINT('Ctrl Pts',(22.5073180101405,31.6179360671638,30.237788296751));
#39721=CARTESIAN_POINT('Ctrl Pts',(22.5073180101405,1.41024006077928,31.5864702700101));
#39722=CARTESIAN_POINT('Ctrl Pts',(21.3125219557939,1.394486513532,31.2336232862855));
#39723=CARTESIAN_POINT('Ctrl Pts',(21.3125219557939,0.697590373623123,31.264737584474));
#39724=CARTESIAN_POINT('Ctrl Pts',(21.3125219557939,1.9144130404504E-15,
31.264737584474));
#39725=CARTESIAN_POINT('Ctrl Pts',(21.3125219557939,-31.264737584474,31.264737584474));
#39726=CARTESIAN_POINT('Ctrl Pts',(21.3125219557939,-31.264737584474,1.9144130404504E-15));
#39727=CARTESIAN_POINT('Ctrl Pts',(21.3125219557939,-31.264737584474,-31.264737584474));
#39728=CARTESIAN_POINT('Ctrl Pts',(21.3125219557939,-1.9144130404504E-15,
-31.264737584474));
#39729=CARTESIAN_POINT('Ctrl Pts',(21.3125219557939,31.264737584474,-31.264737584474));
#39730=CARTESIAN_POINT('Ctrl Pts',(21.3125219557939,31.264737584474,-1.9144130404504E-15));
#39731=CARTESIAN_POINT('Ctrl Pts',(21.3125219557939,31.264737584474,29.9000072055494));
#39732=CARTESIAN_POINT('Ctrl Pts',(21.3125219557939,1.394486513532,31.2336232862855));
#39733=CARTESIAN_POINT('Ctrl Pts',(20.0742472323676,1.3812125919422,30.9363148057487));
#39734=CARTESIAN_POINT('Ctrl Pts',(20.0742472323676,0.690950108671535,30.9671329312955));
#39735=CARTESIAN_POINT('Ctrl Pts',(20.0742472323676,1.89619001115408E-15,
30.9671329312955));
#39736=CARTESIAN_POINT('Ctrl Pts',(20.0742472323676,-30.9671329312955,30.9671329312955));
#39737=CARTESIAN_POINT('Ctrl Pts',(20.0742472323676,-30.9671329312955,1.89619001115408E-15));
#39738=CARTESIAN_POINT('Ctrl Pts',(20.0742472323676,-30.9671329312955,-30.9671329312955));
#39739=CARTESIAN_POINT('Ctrl Pts',(20.0742472323676,-1.89619001115408E-15,
-30.9671329312955));
#39740=CARTESIAN_POINT('Ctrl Pts',(20.0742472323676,30.9671329312955,-30.9671329312955));
#39741=CARTESIAN_POINT('Ctrl Pts',(20.0742472323676,30.9671329312955,-1.89619001115408E-15));
#39742=CARTESIAN_POINT('Ctrl Pts',(20.0742472323676,30.9671329312955,29.6153932294878));
#39743=CARTESIAN_POINT('Ctrl Pts',(20.0742472323676,1.3812125919422,30.9363148057487));
#39744=CARTESIAN_POINT('Ctrl Pts',(18.7979917002302,1.3705167280896,30.6967495040754));
#39745=CARTESIAN_POINT('Ctrl Pts',(18.7979917002302,0.685599514321029,30.727328979557));
#39746=CARTESIAN_POINT('Ctrl Pts',(18.7979917002302,1.88150625405811E-15,
30.727328979557));
#39747=CARTESIAN_POINT('Ctrl Pts',(18.7979917002302,-30.727328979557,30.727328979557));
#39748=CARTESIAN_POINT('Ctrl Pts',(18.7979917002302,-30.727328979557,1.88150625405811E-15));
#39749=CARTESIAN_POINT('Ctrl Pts',(18.7979917002302,-30.727328979557,-30.727328979557));
#39750=CARTESIAN_POINT('Ctrl Pts',(18.7979917002302,-1.88150625405811E-15,
-30.727328979557));
#39751=CARTESIAN_POINT('Ctrl Pts',(18.7979917002302,30.727328979557,-30.727328979557));
#39752=CARTESIAN_POINT('Ctrl Pts',(18.7979917002302,30.727328979557,-1.88150625405811E-15));
#39753=CARTESIAN_POINT('Ctrl Pts',(18.7979917002302,30.727328979557,29.3860569087997));
#39754=CARTESIAN_POINT('Ctrl Pts',(18.7979917002302,1.3705167280896,30.6967495040754));
#39755=CARTESIAN_POINT('Ctrl Pts',(17.4917404060759,1.36221698336641,30.5108523315028));
#39756=CARTESIAN_POINT('Ctrl Pts',(17.4917404060759,0.681447575979397,30.5412466200144));
#39757=CARTESIAN_POINT('Ctrl Pts',(17.4917404060759,1.87011199575853E-15,
30.5412466200144));
#39758=CARTESIAN_POINT('Ctrl Pts',(17.4917404060759,-30.5412466200144,30.5412466200144));
#39759=CARTESIAN_POINT('Ctrl Pts',(17.4917404060759,-30.5412466200144,1.87011199575853E-15));
#39760=CARTESIAN_POINT('Ctrl Pts',(17.4917404060759,-30.5412466200144,-30.5412466200144));
#39761=CARTESIAN_POINT('Ctrl Pts',(17.4917404060759,-1.87011199575853E-15,
-30.5412466200144));
#39762=CARTESIAN_POINT('Ctrl Pts',(17.4917404060759,30.5412466200144,-30.5412466200144));
#39763=CARTESIAN_POINT('Ctrl Pts',(17.4917404060759,30.5412466200144,-1.87011199575853E-15));
#39764=CARTESIAN_POINT('Ctrl Pts',(17.4917404060759,30.5412466200144,29.2080971905671));
#39765=CARTESIAN_POINT('Ctrl Pts',(17.4917404060759,1.36221698336641,30.5108523315028));
#39766=CARTESIAN_POINT('Ctrl Pts',(16.1647270995715,1.35595673938413,30.3706357712668));
#39767=CARTESIAN_POINT('Ctrl Pts',(16.1647270995715,0.678315895682604,30.4008903789023));
#39768=CARTESIAN_POINT('Ctrl Pts',(16.1647270995715,1.86151765468761E-15,
30.4008903789023));
#39769=CARTESIAN_POINT('Ctrl Pts',(16.1647270995715,-30.4008903789023,30.4008903789023));
#39770=CARTESIAN_POINT('Ctrl Pts',(16.1647270995715,-30.4008903789023,1.86151765468761E-15));
#39771=CARTESIAN_POINT('Ctrl Pts',(16.1647270995715,-30.4008903789023,-30.4008903789023));
#39772=CARTESIAN_POINT('Ctrl Pts',(16.1647270995715,-1.86151765468761E-15,
-30.4008903789023));
#39773=CARTESIAN_POINT('Ctrl Pts',(16.1647270995715,30.4008903789023,-30.4008903789023));
#39774=CARTESIAN_POINT('Ctrl Pts',(16.1647270995715,30.4008903789023,-1.86151765468761E-15));
#39775=CARTESIAN_POINT('Ctrl Pts',(16.1647270995715,30.4008903789023,29.0738676097412));
#39776=CARTESIAN_POINT('Ctrl Pts',(16.1647270995715,1.35595673938413,30.3706357712668));
#39777=CARTESIAN_POINT('Ctrl Pts',(14.8263876417415,1.3512881251525,30.2660684364343));
#39778=CARTESIAN_POINT('Ctrl Pts',(14.8263876417415,0.675980426451066,30.2962188762246));
#39779=CARTESIAN_POINT('Ctrl Pts',(14.8263876417415,1.8551083736518E-15,
30.2962188762246));
#39780=CARTESIAN_POINT('Ctrl Pts',(14.8263876417415,-30.2962188762245,30.2962188762245));
#39781=CARTESIAN_POINT('Ctrl Pts',(14.8263876417415,-30.2962188762246,1.8551083736518E-15));
#39782=CARTESIAN_POINT('Ctrl Pts',(14.8263876417415,-30.2962188762245,-30.2962188762245));
#39783=CARTESIAN_POINT('Ctrl Pts',(14.8263876417415,-1.8551083736518E-15,
-30.2962188762246));
#39784=CARTESIAN_POINT('Ctrl Pts',(14.8263876417415,30.2962188762245,-30.2962188762245));
#39785=CARTESIAN_POINT('Ctrl Pts',(14.8263876417415,30.2962188762246,-1.8551083736518E-15));
#39786=CARTESIAN_POINT('Ctrl Pts',(14.8263876417415,30.2962188762245,28.9737651004582));
#39787=CARTESIAN_POINT('Ctrl Pts',(14.8263876417415,1.3512881251525,30.2660684364343));
#39788=CARTESIAN_POINT('Ctrl Pts',(13.4853470903953,1.34775518513426,30.186937862885));
#39789=CARTESIAN_POINT('Ctrl Pts',(13.4853470903953,0.674213077019291,30.2170094744125));
#39790=CARTESIAN_POINT('Ctrl Pts',(13.4853470903953,1.85025819663223E-15,
30.2170094744125));
#39791=CARTESIAN_POINT('Ctrl Pts',(13.4853470903953,-30.2170094744125,30.2170094744125));
#39792=CARTESIAN_POINT('Ctrl Pts',(13.4853470903953,-30.2170094744125,1.85025819663223E-15));
#39793=CARTESIAN_POINT('Ctrl Pts',(13.4853470903953,-30.2170094744125,-30.2170094744125));
#39794=CARTESIAN_POINT('Ctrl Pts',(13.4853470903953,-1.85025819663223E-15,
-30.2170094744125));
#39795=CARTESIAN_POINT('Ctrl Pts',(13.4853470903953,30.2170094744125,-30.2170094744125));
#39796=CARTESIAN_POINT('Ctrl Pts',(13.4853470903953,30.2170094744125,-1.85025819663223E-15));
#39797=CARTESIAN_POINT('Ctrl Pts',(13.4853470903953,30.2170094744125,28.8980132513174));
#39798=CARTESIAN_POINT('Ctrl Pts',(13.4853470903953,1.34775518513426,30.186937862885));
#39799=CARTESIAN_POINT('Ctrl Pts',(12.1482076787549,1.34498727870742,30.1249424647305));
#39800=CARTESIAN_POINT('Ctrl Pts',(12.1482076787549,0.672828434816076,30.1549523177074));
#39801=CARTESIAN_POINT('Ctrl Pts',(12.1482076787549,1.84645829171607E-15,
30.1549523177074));
#39802=CARTESIAN_POINT('Ctrl Pts',(12.1482076787549,-30.1549523177074,30.1549523177074));
#39803=CARTESIAN_POINT('Ctrl Pts',(12.1482076787549,-30.1549523177074,1.84645829171607E-15));
#39804=CARTESIAN_POINT('Ctrl Pts',(12.1482076787549,-30.1549523177074,-30.1549523177074));
#39805=CARTESIAN_POINT('Ctrl Pts',(12.1482076787549,-1.84645829171607E-15,
-30.1549523177074));
#39806=CARTESIAN_POINT('Ctrl Pts',(12.1482076787549,30.1549523177074,-30.1549523177074));
#39807=CARTESIAN_POINT('Ctrl Pts',(12.1482076787549,30.1549523177074,-1.84645829171607E-15));
#39808=CARTESIAN_POINT('Ctrl Pts',(12.1482076787549,30.1549523177074,28.8386649382978));
#39809=CARTESIAN_POINT('Ctrl Pts',(12.1482076787549,1.34498727870742,30.1249424647305));
#39810=CARTESIAN_POINT('Ctrl Pts',(10.8190675759626,1.34274367710657,30.0746904138676));
#39811=CARTESIAN_POINT('Ctrl Pts',(10.8190675759626,0.671706075536288,30.1046502067769));
#39812=CARTESIAN_POINT('Ctrl Pts',(10.8190675759626,1.843378175759E-15,
30.1046502067769));
#39813=CARTESIAN_POINT('Ctrl Pts',(10.8190675759626,-30.1046502067769,30.1046502067769));
#39814=CARTESIAN_POINT('Ctrl Pts',(10.8190675759626,-30.1046502067769,1.843378175759E-15));
#39815=CARTESIAN_POINT('Ctrl Pts',(10.8190675759626,-30.1046502067769,-30.1046502067769));
#39816=CARTESIAN_POINT('Ctrl Pts',(10.8190675759626,-1.843378175759E-15,
-30.1046502067769));
#39817=CARTESIAN_POINT('Ctrl Pts',(10.8190675759626,30.1046502067769,-30.1046502067769));
#39818=CARTESIAN_POINT('Ctrl Pts',(10.8190675759626,30.1046502067769,-1.843378175759E-15));
#39819=CARTESIAN_POINT('Ctrl Pts',(10.8190675759626,30.1046502067769,28.7905585540618));
#39820=CARTESIAN_POINT('Ctrl Pts',(10.8190675759626,1.34274367710657,30.0746904138676));
#39821=CARTESIAN_POINT('Ctrl Pts',(9.50027713254189,1.34087520118769,30.032840404991));
#39822=CARTESIAN_POINT('Ctrl Pts',(9.50027713254189,0.670771372474117,30.0627585077754));
#39823=CARTESIAN_POINT('Ctrl Pts',(9.50027713254189,1.84081304900435E-15,
30.0627585077754));
#39824=CARTESIAN_POINT('Ctrl Pts',(9.50027713254189,-30.0627585077753,30.0627585077753));
#39825=CARTESIAN_POINT('Ctrl Pts',(9.50027713254189,-30.0627585077754,1.84081304900435E-15));
#39826=CARTESIAN_POINT('Ctrl Pts',(9.5002771325419,-30.0627585077753,-30.0627585077753));
#39827=CARTESIAN_POINT('Ctrl Pts',(9.5002771325419,-1.84081304900435E-15,
-30.0627585077754));
#39828=CARTESIAN_POINT('Ctrl Pts',(9.5002771325419,30.0627585077753,-30.0627585077753));
#39829=CARTESIAN_POINT('Ctrl Pts',(9.50027713254189,30.0627585077754,-1.84081304900435E-15));
#39830=CARTESIAN_POINT('Ctrl Pts',(9.50027713254189,30.0627585077753,28.750495460661));
#39831=CARTESIAN_POINT('Ctrl Pts',(9.50027713254189,1.34087520118769,30.032840404991));
#39832=CARTESIAN_POINT('Ctrl Pts',(8.45435372222587,1.33961990745209,30.0047244129961));
#39833=CARTESIAN_POINT('Ctrl Pts',(8.45435372222587,0.670143413137451,30.0346145072029));
#39834=CARTESIAN_POINT('Ctrl Pts',(8.45435372222587,1.83908972599354E-15,
30.0346145072029));
#39835=CARTESIAN_POINT('Ctrl Pts',(8.45435372222587,-30.0346145072029,30.0346145072029));
#39836=CARTESIAN_POINT('Ctrl Pts',(8.45435372222587,-30.0346145072029,1.83908972599354E-15));
#39837=CARTESIAN_POINT('Ctrl Pts',(8.45435372222587,-30.0346145072029,-30.0346145072029));
#39838=CARTESIAN_POINT('Ctrl Pts',(8.45435372222587,-1.83908972599354E-15,
-30.0346145072029));
#39839=CARTESIAN_POINT('Ctrl Pts',(8.45435372222587,30.0346145072029,-30.0346145072029));
#39840=CARTESIAN_POINT('Ctrl Pts',(8.45435372222587,30.0346145072029,-1.83908972599354E-15));
#39841=CARTESIAN_POINT('Ctrl Pts',(8.45435372222587,30.0346145072029,28.7235799678431));
#39842=CARTESIAN_POINT('Ctrl Pts',(8.45435372222587,1.33961990745209,30.0047244129961));
#39843=CARTESIAN_POINT('Ctrl Pts',(7.67514864245731,1.33880061938141,29.9863740491064));
#39844=CARTESIAN_POINT('Ctrl Pts',(7.67514864245731,0.669733565164176,30.0162458630552));
#39845=CARTESIAN_POINT('Ctrl Pts',(7.67514864245731,1.83796497093053E-15,
30.0162458630552));
#39846=CARTESIAN_POINT('Ctrl Pts',(7.67514864245731,-30.0162458630552,30.0162458630552));
#39847=CARTESIAN_POINT('Ctrl Pts',(7.67514864245731,-30.0162458630552,1.83796497093053E-15));
#39848=CARTESIAN_POINT('Ctrl Pts',(7.67514864245731,-30.0162458630552,-30.0162458630552));
#39849=CARTESIAN_POINT('Ctrl Pts',(7.67514864245731,-1.83796497093053E-15,
-30.0162458630552));
#39850=CARTESIAN_POINT('Ctrl Pts',(7.67514864245731,30.0162458630552,-30.0162458630552));
#39851=CARTESIAN_POINT('Ctrl Pts',(7.67514864245731,30.0162458630552,-1.83796497093053E-15));
#39852=CARTESIAN_POINT('Ctrl Pts',(7.67514864245731,30.0162458630552,28.7060131294556));
#39853=CARTESIAN_POINT('Ctrl Pts',(7.67514864245731,1.33880061938141,29.9863740491064));
#39854=CARTESIAN_POINT('Ctrl Pts',(7.15799654185577,1.33830853171149,29.9753522996976));
#39855=CARTESIAN_POINT('Ctrl Pts',(7.15799654185577,0.669487398838304,30.0052131340045));
#39856=CARTESIAN_POINT('Ctrl Pts',(7.15799654185577,1.83728941111464E-15,
30.0052131340045));
#39857=CARTESIAN_POINT('Ctrl Pts',(7.15799654185577,-30.0052131340045,30.0052131340045));
#39858=CARTESIAN_POINT('Ctrl Pts',(7.15799654185577,-30.0052131340045,1.83728941111464E-15));
#39859=CARTESIAN_POINT('Ctrl Pts',(7.15799654185577,-30.0052131340045,-30.0052131340045));
#39860=CARTESIAN_POINT('Ctrl Pts',(7.15799654185577,-1.83728941111464E-15,
-30.0052131340045));
#39861=CARTESIAN_POINT('Ctrl Pts',(7.15799654185577,30.0052131340045,-30.0052131340045));
#39862=CARTESIAN_POINT('Ctrl Pts',(7.15799654185577,30.0052131340045,-1.83728941111464E-15));
#39863=CARTESIAN_POINT('Ctrl Pts',(7.15799654185577,30.0052131340045,28.695461987703));
#39864=CARTESIAN_POINT('Ctrl Pts',(7.15799654185577,1.33830853171149,29.9753522996976));
#39865=CARTESIAN_POINT('Ctrl Pts',(6.9,1.33807601272607,29.9701443537426));
#39866=CARTESIAN_POINT('Ctrl Pts',(6.9,0.669371081466756,30.));
#39867=CARTESIAN_POINT('Ctrl Pts',(6.9,1.83697019872103E-15,30.));
#39868=CARTESIAN_POINT('Ctrl Pts',(6.9,-30.,30.));
#39869=CARTESIAN_POINT('Ctrl Pts',(6.9,-30.,1.83697019872103E-15));
#39870=CARTESIAN_POINT('Ctrl Pts',(6.9,-30.,-30.));
#39871=CARTESIAN_POINT('Ctrl Pts',(6.9,-1.83697019872103E-15,-30.));
#39872=CARTESIAN_POINT('Ctrl Pts',(6.9,30.,-30.));
#39873=CARTESIAN_POINT('Ctrl Pts',(6.9,30.,-1.83697019872103E-15));
#39874=CARTESIAN_POINT('Ctrl Pts',(6.9,30.,28.6904764110968));
#39875=CARTESIAN_POINT('Ctrl Pts',(6.9,1.33807601272607,29.9701443537426));
#39876=CARTESIAN_POINT('Ctrl Pts',(6.9,-21.8303175223207,20.5775906479515));
#39877=CARTESIAN_POINT('Ctrl Pts',(7.85773098116326,-20.4889265372406,22.0288565043892));
#39878=CARTESIAN_POINT('Ctrl Pts',(8.88781981167334,-19.0414114324084,23.3171626725998));
#39879=CARTESIAN_POINT('Ctrl Pts',(10.5914578196776,-16.6247285680552,25.1150390010341));
#39880=CARTESIAN_POINT('Ctrl Pts',(11.2365058953701,-15.703976734769,25.7254166302984));
#39881=CARTESIAN_POINT('Ctrl Pts',(12.0558885382926,-14.5853792872662,26.3926147460599));
#39882=CARTESIAN_POINT('Ctrl Pts',(12.1875764958397,-14.4076425286694,26.4963665374952));
#39883=CARTESIAN_POINT('Ctrl Pts',(13.194901830313,-13.0552778456719,27.2691057169114));
#39884=CARTESIAN_POINT('Ctrl Pts',(14.2258982134098,-11.6381637544796,27.991732600527));
#39885=CARTESIAN_POINT('Ctrl Pts',(18.2616480823244,-6.95587410790868,29.9350198014187));
#39886=CARTESIAN_POINT('Ctrl Pts',(21.0496416709525,-4.29983295736294,30.7693084982877));
#39887=CARTESIAN_POINT('Ctrl Pts',(25.8000196361138,-1.93741001991749,32.8040277065106));
#39888=CARTESIAN_POINT('Ctrl Pts',(26.8976561124457,-1.74039351523169,33.3305524688301));
#39889=CARTESIAN_POINT('Ctrl Pts',(28.0045908801237,-1.58669630450145,33.8378020212277));
#39890=CARTESIAN_POINT('Ctrl Pts',(28.5235971652406,-1.54532623843658,34.0754855762016));
#39891=CARTESIAN_POINT('Ctrl Pts',(29.0834839543824,-1.4982885487127,34.3307100593381));
#39892=CARTESIAN_POINT('Ctrl Pts',(29.1146288039499,-1.49562082188434,34.3449058451715));
#39893=CARTESIAN_POINT('Ctrl Pts',(29.5949306848436,-1.45589225448014,34.5637016811193));
#39894=CARTESIAN_POINT('Ctrl Pts',(30.0492939924726,-1.44682754698748,34.7685410859787));
#39895=CARTESIAN_POINT('Ctrl Pts',(30.5,-1.44976976333441,34.9699609326822));
#39896=CARTESIAN_POINT('Ctrl Pts',(6.45331003273164,-8.65286216739172,6.83943894028999));
#39897=CARTESIAN_POINT('Ctrl Pts',(7.20830533428676,-8.29622318255582,7.28712780725476));
#39898=CARTESIAN_POINT('Ctrl Pts',(7.99995511878976,-7.91871702121326,7.7001428520779));
#39899=CARTESIAN_POINT('Ctrl Pts',(9.52825943498397,-7.18271304249705,8.39510948814989));
#39900=CARTESIAN_POINT('Ctrl Pts',(10.4940807594721,-6.69830435523696,8.7864108718328));
#39901=CARTESIAN_POINT('Ctrl Pts',(11.4876274938915,-6.22320820014201,9.12017193389638));
#39902=CARTESIAN_POINT('Ctrl Pts',(12.4303878001112,-5.78075775962483,9.42058964158202));
#39903=CARTESIAN_POINT('Ctrl Pts',(13.3997261751211,-5.32007492151067,9.68640068655135));
#39904=CARTESIAN_POINT('Ctrl Pts',(14.3872053777042,-4.88962379427552,9.90607181050111));
#39905=CARTESIAN_POINT('Ctrl Pts',(15.556163132278,-4.3942725212231,10.1514774675698));
#39906=CARTESIAN_POINT('Ctrl Pts',(16.5289171701813,-3.99001252407697,10.309499502888));
#39907=CARTESIAN_POINT('Ctrl Pts',(18.441690792892,-3.31066676205255,10.5572419303421));
#39908=CARTESIAN_POINT('Ctrl Pts',(19.4166449194874,-2.9827440568927,10.6478584846087));
#39909=CARTESIAN_POINT('Ctrl Pts',(20.8623232387078,-2.58759893430878,10.7551557591785));
#39910=CARTESIAN_POINT('Ctrl Pts',(21.8144303959787,-2.34043714010253,10.8124914939577));
#39911=CARTESIAN_POINT('Ctrl Pts',(22.7818406100989,-2.13287731493684,10.8543222400653));
#39912=CARTESIAN_POINT('Ctrl Pts',(23.3297671905071,-2.0316389093207,10.8753628160501));
#39913=CARTESIAN_POINT('Ctrl Pts',(23.4470348316276,-2.01025275957826,10.8796570477425));
#39914=CARTESIAN_POINT('Ctrl Pts',(23.6811400295324,-1.96865550184816,10.8877908591686));
#39915=CARTESIAN_POINT('Ctrl Pts',(24.094239596771,-1.89823453468209,10.9009196003301));
#39916=CARTESIAN_POINT('Ctrl Pts',(24.6901429177709,-1.80574893003815,10.9167796594793));
#39917=CARTESIAN_POINT('Ctrl Pts',(25.2916165705408,-1.72612415763836,10.9295334868831));
#39918=CARTESIAN_POINT('Ctrl Pts',(25.7739565747927,-1.67150491651973,10.9383070002314));
#39919=CARTESIAN_POINT('Ctrl Pts',(26.0152863105174,-1.64740058814794,10.9422949598257));
#39920=CARTESIAN_POINT('Ctrl Pts',(26.3672928498145,-1.61473834547487,10.94787874029));
#39921=CARTESIAN_POINT('Ctrl Pts',(27.2930496194305,-1.54497298618683,10.9593530234768));
#39922=CARTESIAN_POINT('Ctrl Pts',(28.2854511951053,-1.51980459192319,10.9616448439048));
#39923=CARTESIAN_POINT('Ctrl Pts',(29.2045434923158,-1.49505480423355,10.965198770667));
#39924=CARTESIAN_POINT('Ctrl Pts',(29.5206711976023,-1.48867173691355,10.9661639337506));
#39925=CARTESIAN_POINT('Ctrl Pts',(30.1692097404134,-1.48262317876973,10.9670495493201));
#39926=CARTESIAN_POINT('Ctrl Pts',(31.3135190714371,-1.4864528553831,10.96649000528));
#39927=CARTESIAN_POINT('Ctrl Pts',(32.3203822393921,-1.49996522881633,10.9645683677272));
#39928=CARTESIAN_POINT('Ctrl Pts',(33.1675664922,-1.49997704079034,10.9645708546322));
#39929=CARTESIAN_POINT('Ctrl Pts',(33.4947686467078,-1.49997747170577,10.9645712531308));
#39930=CARTESIAN_POINT('Ctrl Pts',(34.1540868645893,-1.49997908112576,10.9645717353852));
#39931=CARTESIAN_POINT('Ctrl Pts',(34.8114534640785,-1.49998335379094,10.9645734486355));
#39932=CARTESIAN_POINT('Ctrl Pts',(35.7991052695187,-1.49998422299017,10.9645737550385));
#39933=CARTESIAN_POINT('Ctrl Pts',(37.7734889032248,-1.49998916111724,10.9645756745653));
#39934=CARTESIAN_POINT('Ctrl Pts',(39.5833333333333,-1.5,10.9645797934319));
#39935=CARTESIAN_POINT('Ctrl Pts',(40.9,-1.5,10.9645797934319));
#39936=CARTESIAN_POINT('Ctrl Pts',(6.6933875035574,-11.7835517019943,10.176216978544));
#39937=CARTESIAN_POINT('Ctrl Pts',(7.45057679732275,-11.2512208468221,10.7852657388529));
#39938=CARTESIAN_POINT('Ctrl Pts',(8.2413121575229,-10.6930046754631,11.3436596611095));
#39939=CARTESIAN_POINT('Ctrl Pts',(9.76826989623895,-9.61265036078123,12.2763196346049));
#39940=CARTESIAN_POINT('Ctrl Pts',(10.7329606123233,-8.90528802461967,12.797808932554));
#39941=CARTESIAN_POINT('Ctrl Pts',(11.7232269898393,-8.21708628846332,13.2363397818143));
#39942=CARTESIAN_POINT('Ctrl Pts',(12.6618589495312,-7.57719783124145,13.6303705734608));
#39943=CARTESIAN_POINT('Ctrl Pts',(13.62938101007,-6.91168434311037,13.9766495525684));
#39944=CARTESIAN_POINT('Ctrl Pts',(14.6088313783793,-6.29602822290691,14.2570519664642));
#39945=CARTESIAN_POINT('Ctrl Pts',(15.7681704150403,-5.5877427072411,14.570157055854));
#39946=CARTESIAN_POINT('Ctrl Pts',(16.7369555416689,-5.00954692132628,14.767994500732));
#39947=CARTESIAN_POINT('Ctrl Pts',(18.6242750358685,-4.04747101384392,15.072833876247));
#39948=CARTESIAN_POINT('Ctrl Pts',(19.5932251737343,-3.58155807753862,15.1807788814753));
#39949=CARTESIAN_POINT('Ctrl Pts',(21.0118923342793,-3.02625583363473,15.3069309857053));
#39950=CARTESIAN_POINT('Ctrl Pts',(21.9540630652681,-2.67707795507692,15.3728356386159));
#39951=CARTESIAN_POINT('Ctrl Pts',(22.9024384113963,-2.38630901256787,15.4189810434881));
#39952=CARTESIAN_POINT('Ctrl Pts',(23.4384834214784,-2.24465775851538,15.4424563702175));
#39953=CARTESIAN_POINT('Ctrl Pts',(23.5542447038724,-2.2145633523891,15.4472367652768));
#39954=CARTESIAN_POINT('Ctrl Pts',(23.78465432169,-2.15615095063381,15.4562082859198));
#39955=CARTESIAN_POINT('Ctrl Pts',(24.1912813672913,-2.0572689135757,15.4705057473596));
#39956=CARTESIAN_POINT('Ctrl Pts',(24.7767883762699,-1.92760629035867,15.487334852315));
#39957=CARTESIAN_POINT('Ctrl Pts',(25.36654130234,-1.81617759528126,15.5005605148525));
#39958=CARTESIAN_POINT('Ctrl Pts',(25.8384861976413,-1.73988825246362,15.5096611552857));
#39959=CARTESIAN_POINT('Ctrl Pts',(26.0742971451332,-1.70625267454512,15.5138439934012));
#39960=CARTESIAN_POINT('Ctrl Pts',(26.4178590548908,-1.66071842408642,15.5197632302621));
#39961=CARTESIAN_POINT('Ctrl Pts',(27.3173215852521,-1.563674416307,15.5317592244184));
#39962=CARTESIAN_POINT('Ctrl Pts',(28.3008974271582,-1.52789332168387,15.5336084019203));
#39963=CARTESIAN_POINT('Ctrl Pts',(29.2205106969984,-1.49282313901989,15.5372361675902));
#39964=CARTESIAN_POINT('Ctrl Pts',(29.5297893441341,-1.48392111804966,15.5382211183205));
#39965=CARTESIAN_POINT('Ctrl Pts',(30.1710603648191,-1.47539843727042,15.5391260510599));
#39966=CARTESIAN_POINT('Ctrl Pts',(31.3058674630461,-1.48078221272374,15.5385594105444));
#39967=CARTESIAN_POINT('Ctrl Pts',(32.3149674119483,-1.49994719631519,15.5366091538308));
#39968=CARTESIAN_POINT('Ctrl Pts',(33.1687991060451,-1.49996649944875,15.5366148440523));
#39969=CARTESIAN_POINT('Ctrl Pts',(33.4951825987405,-1.49996690229146,15.5366157560837));
#39970=CARTESIAN_POINT('Ctrl Pts',(34.1549121057911,-1.49996939198939,15.5366168596277));
#39971=CARTESIAN_POINT('Ctrl Pts',(34.8118777623806,-1.49997557765831,15.5366207802977));
#39972=CARTESIAN_POINT('Ctrl Pts',(35.7995932556016,-1.49997687727485,15.5366214814653));
#39973=CARTESIAN_POINT('Ctrl Pts',(37.7737223043124,-1.49998408565139,15.536625874162));
#39974=CARTESIAN_POINT('Ctrl Pts',(39.5833333333333,-1.5,15.5366352998475));
#39975=CARTESIAN_POINT('Ctrl Pts',(40.9,-1.5,15.5366352998475));
#39976=CARTESIAN_POINT('Ctrl Pts',(6.84856199327287,-17.3015601300326,15.9756656267856));
#39977=CARTESIAN_POINT('Ctrl Pts',(7.6163426075982,-16.4542577625343,16.880477206766));
#39978=CARTESIAN_POINT('Ctrl Pts',(8.41867777462062,-15.5717695685564,17.7014911506025));
#39979=CARTESIAN_POINT('Ctrl Pts',(9.96113195955868,-13.8764580517237,19.0620073137526));
#39980=CARTESIAN_POINT('Ctrl Pts',(10.9332800166621,-12.7736673235567,19.815224791801));
#39981=CARTESIAN_POINT('Ctrl Pts',(11.9367963602557,-11.6987467748375,20.4447687021717));
#39982=CARTESIAN_POINT('Ctrl Pts',(12.8867814792929,-10.7022950266451,21.0075672609871));
#39983=CARTESIAN_POINT('Ctrl Pts',(13.8590496672151,-9.67539612019949,21.4943962460795));
#39984=CARTESIAN_POINT('Ctrl Pts',(14.8485921349356,-8.72431608662546,21.884054887486));
#39985=CARTESIAN_POINT('Ctrl Pts',(16.0163007294256,-7.63455433184466,22.3166578360873));
#39986=CARTESIAN_POINT('Ctrl Pts',(16.9884569437496,-6.75057879345238,22.5821364755291));
#39987=CARTESIAN_POINT('Ctrl Pts',(18.8739644427958,-5.29110974776816,22.9841384147108));
#39988=CARTESIAN_POINT('Ctrl Pts',(19.8410528812574,-4.58570965781586,23.1201648771934));
#39989=CARTESIAN_POINT('Ctrl Pts',(21.2381152642979,-3.75822630090649,23.2766545601846));
#39990=CARTESIAN_POINT('Ctrl Pts',(22.1709482299956,-3.23413242036785,23.3562489404792));
#39991=CARTESIAN_POINT('Ctrl Pts',(23.0969226589074,-2.80482604568844,23.4088332599271));
#39992=CARTESIAN_POINT('Ctrl Pts',(23.6167257768698,-2.59669919378737,23.436097008432));
#39993=CARTESIAN_POINT('Ctrl Pts',(23.7304440861555,-2.55187487879195,23.4416610185368));
#39994=CARTESIAN_POINT('Ctrl Pts',(23.9557382879883,-2.46529344501871,23.4519564031388));
#39995=CARTESIAN_POINT('Ctrl Pts',(24.3531769354774,-2.3187667506293,23.4680750466195));
#39996=CARTESIAN_POINT('Ctrl Pts',(24.9232265691605,-2.12735895816067,23.4863293251813));
#39997=CARTESIAN_POINT('Ctrl Pts',(25.4945991725924,-1.96359000545671,23.5001927499934));
#39998=CARTESIAN_POINT('Ctrl Pts',(25.9497700202409,-1.8518994638432,23.5097714589304));
#39999=CARTESIAN_POINT('Ctrl Pts',(26.176473840736,-1.80278336268422,23.5142578389004));
#40000=CARTESIAN_POINT('Ctrl Pts',(26.5059907605108,-1.73643358900275,23.5207181203645));
#40001=CARTESIAN_POINT('Ctrl Pts',(27.3606430706766,-1.59579143734496,23.5335529917322));
#40002=CARTESIAN_POINT('Ctrl Pts',(28.328238250736,-1.54133580528123,23.5346127004849));
#40003=CARTESIAN_POINT('Ctrl Pts',(29.2487071190625,-1.48828577636564,23.5383515936462));
#40004=CARTESIAN_POINT('Ctrl Pts',(29.5460132431354,-1.47529943899978,23.5393690406291));
#40005=CARTESIAN_POINT('Ctrl Pts',(30.1745409675272,-1.46257298770338,23.5403036706459));
#40006=CARTESIAN_POINT('Ctrl Pts',(31.2926891957807,-1.47061513008709,23.5397184432942));
#40007=CARTESIAN_POINT('Ctrl Pts',(32.3056292653037,-1.49977993503654,23.5377052457532));
#40008=CARTESIAN_POINT('Ctrl Pts',(33.171063928526,-1.49984576464778,23.53771116989));
#40009=CARTESIAN_POINT('Ctrl Pts',(33.4960099678507,-1.49985013662889,23.5377121171257));
#40010=CARTESIAN_POINT('Ctrl Pts',(34.1564534126615,-1.49986002424299,23.5377132649686));
#40011=CARTESIAN_POINT('Ctrl Pts',(34.8126967694548,-1.4998890457023,23.5377173407623));
#40012=CARTESIAN_POINT('Ctrl Pts',(35.8005200217607,-1.49989467989925,23.5377180698364));
#40013=CARTESIAN_POINT('Ctrl Pts',(37.7741804086525,-1.4999278336931,23.5377226365692));
#40014=CARTESIAN_POINT('Ctrl Pts',(39.5833333333333,-1.5,23.5377324360749));
#40015=CARTESIAN_POINT('Ctrl Pts',(40.9,-1.5,23.5377324360749));
#40016=CARTESIAN_POINT('Ctrl Pts',(6.91525560456497,-22.9100322970705,21.6832437463415));
#40017=CARTESIAN_POINT('Ctrl Pts',(7.68680828807946,-21.7506407559596,22.8901115475878));
#40018=CARTESIAN_POINT('Ctrl Pts',(8.49254333196796,-20.5454520608109,23.9817021083909));
#40019=CARTESIAN_POINT('Ctrl Pts',(10.0410868869421,-18.2355476030532,25.783436835301));
#40020=CARTESIAN_POINT('Ctrl Pts',(11.0156330688494,-16.7381286127845,26.7761285175838));
#40021=CARTESIAN_POINT('Ctrl Pts',(12.0267774787436,-15.2694195930957,27.6065335630864));
#40022=CARTESIAN_POINT('Ctrl Pts',(12.9837665933316,-13.9090077888112,28.3472037410707));
#40023=CARTESIAN_POINT('Ctrl Pts',(13.9582748251365,-12.5185550738456,28.9806054990946));
#40024=CARTESIAN_POINT('Ctrl Pts',(14.9579439087574,-11.2181255435619,29.4879275336708));
#40025=CARTESIAN_POINT('Ctrl Pts',(16.1360231813382,-9.73182073292782,30.0486109782393));
#40026=CARTESIAN_POINT('Ctrl Pts',(17.1125926236779,-8.53469955955227,30.3858860137637));
#40027=CARTESIAN_POINT('Ctrl Pts',(19.0161910165423,-6.54807207599635,30.893375381823));
#40028=CARTESIAN_POINT('Ctrl Pts',(19.9877676407317,-5.59579046139741,31.0588212358041));
#40029=CARTESIAN_POINT('Ctrl Pts',(21.3909461476618,-4.48020211813739,31.2474019180858));
#40030=CARTESIAN_POINT('Ctrl Pts',(22.3248563284891,-3.77659408112775,31.3408522311969));
#40031=CARTESIAN_POINT('Ctrl Pts',(23.2468923217639,-3.20514337922215,31.3997620359148));
#40032=CARTESIAN_POINT('Ctrl Pts',(23.7601739654543,-2.93082137010623,31.430627683656));
#40033=CARTESIAN_POINT('Ctrl Pts',(23.8730573072336,-2.87131241748073,31.4369365823338));
#40034=CARTESIAN_POINT('Ctrl Pts',(24.0961287002213,-2.75675829411561,31.4484760107116));
#40035=CARTESIAN_POINT('Ctrl Pts',(24.4892033184452,-2.56315742515059,31.4662740955766));
#40036=CARTESIAN_POINT('Ctrl Pts',(25.0507326849357,-2.31155892021077,31.4857535994475));
#40037=CARTESIAN_POINT('Ctrl Pts',(25.6099642666879,-2.09799811072266,31.5000858680305));
#40038=CARTESIAN_POINT('Ctrl Pts',(26.0526717556216,-1.95341986226856,31.5100364612848));
#40039=CARTESIAN_POINT('Ctrl Pts',(26.2721174193034,-1.89019302484359,31.5147848140591));
#40040=CARTESIAN_POINT('Ctrl Pts',(26.5900938789433,-1.80510164023555,31.5217327388238));
#40041=CARTESIAN_POINT('Ctrl Pts',(27.4046313185694,-1.62683363158072,31.5353204657088));
#40042=CARTESIAN_POINT('Ctrl Pts',(28.3551551181953,-1.55385623211788,31.5356158769573));
#40043=CARTESIAN_POINT('Ctrl Pts',(29.2766284588593,-1.48285998465491,31.5394629693118));
#40044=CARTESIAN_POINT('Ctrl Pts',(29.5620749777487,-1.46634178597095,31.5405133739895));
#40045=CARTESIAN_POINT('Ctrl Pts',(30.1778667116529,-1.44961397315314,31.5414782418285));
#40046=CARTESIAN_POINT('Ctrl Pts',(31.2793924730891,-1.46018163281271,31.5408746533112));
#40047=CARTESIAN_POINT('Ctrl Pts',(32.2962077526077,-1.49947992165247,31.5387996004541));
#40048=CARTESIAN_POINT('Ctrl Pts',(33.1732631913448,-1.49962796113082,31.5388061398229));
#40049=CARTESIAN_POINT('Ctrl Pts',(33.4967747473349,-1.49963968162193,31.538807182264));
#40050=CARTESIAN_POINT('Ctrl Pts',(34.1579356372808,-1.49966279717681,31.5388084478368));
#40051=CARTESIAN_POINT('Ctrl Pts',(34.813469269944,-1.49973305460827,31.5388129385369));
#40052=CARTESIAN_POINT('Ctrl Pts',(35.8014025220136,-1.49974648220053,31.5388137420569));
#40053=CARTESIAN_POINT('Ctrl Pts',(37.7746083248076,-1.49982643859215,31.5388187740001));
#40054=CARTESIAN_POINT('Ctrl Pts',(39.5833333333333,-1.5,31.5388295723023));
#40055=CARTESIAN_POINT('Ctrl Pts',(40.9,-1.5,31.5388295723023));
#40056=CARTESIAN_POINT('Ctrl Pts',(6.93528330520032,-25.3195110382618,24.1234099037007));
#40057=CARTESIAN_POINT('Ctrl Pts',(7.70864561497005,-24.0266258397084,25.4600205488393));
#40058=CARTESIAN_POINT('Ctrl Pts',(8.51562113079159,-22.683454927525,26.6679288641754));
#40059=CARTESIAN_POINT('Ctrl Pts',(10.0666374697795,-20.1106380333435,28.6593492285767));
#40060=CARTESIAN_POINT('Ctrl Pts',(11.042032006318,-18.4443560472,29.7550958483524));
#40061=CARTESIAN_POINT('Ctrl Pts',(12.0563101934605,-16.8071578945887,30.6719165802071));
#40062=CARTESIAN_POINT('Ctrl Pts',(13.0160460695303,-15.29096142786,31.4891825490877));
#40063=CARTESIAN_POINT('Ctrl Pts',(13.9913179180522,-13.7448072814026,32.1858307461017));
#40064=CARTESIAN_POINT('Ctrl Pts',(14.9948977569346,-12.2946331064003,32.7439647444974));
#40065=CARTESIAN_POINT('Ctrl Pts',(16.1769113040285,-10.6381684618929,33.3600488616169));
#40066=CARTESIAN_POINT('Ctrl Pts',(17.1550702558646,-9.30667068355118,33.7285091938727));
#40067=CARTESIAN_POINT('Ctrl Pts',(19.0659094948408,-7.09221287605646,34.2820742196266));
#40068=CARTESIAN_POINT('Ctrl Pts',(20.0392998042888,-6.03343331328744,34.4604355518963));
#40069=CARTESIAN_POINT('Ctrl Pts',(21.4463900864313,-4.79170617358831,34.6632094821159));
#40070=CARTESIAN_POINT('Ctrl Pts',(22.3814014849328,-4.01016373038329,34.7627470812904));
#40071=CARTESIAN_POINT('Ctrl Pts',(23.3035439511912,-3.37628406315923,34.8244714644531));
#40072=CARTESIAN_POINT('Ctrl Pts',(23.8153199893244,-3.07301749249811,34.8569024326816));
#40073=CARTESIAN_POINT('Ctrl Pts',(23.9280059115487,-3.00714498962961,34.8635321227254));
#40074=CARTESIAN_POINT('Ctrl Pts',(24.1505233346922,-2.88044612076907,34.8756078808959));
#40075=CARTESIAN_POINT('Ctrl Pts',(24.5424299687223,-2.66644368612956,34.8941271156085));
#40076=CARTESIAN_POINT('Ctrl Pts',(25.1014254054398,-2.38883635621612,34.914125424837));
#40077=CARTESIAN_POINT('Ctrl Pts',(25.6566063651091,-2.1539516173883,34.9286453169304));
#40078=CARTESIAN_POINT('Ctrl Pts',(26.0948392448068,-1.99544031319315,34.938744218721));
#40079=CARTESIAN_POINT('Ctrl Pts',(26.3115689572165,-1.92629671309846,34.9435997527764));
#40080=CARTESIAN_POINT('Ctrl Pts',(26.6251471538059,-1.83339663912719,34.9507497717891));
#40081=CARTESIAN_POINT('Ctrl Pts',(27.4236115182935,-1.63986518992209,34.9646466630656));
#40082=CARTESIAN_POINT('Ctrl Pts',(28.3665836197148,-1.55906444107099,34.9646176398389));
#40083=CARTESIAN_POINT('Ctrl Pts',(29.2885219356023,-1.48037458462995,34.9685105141258));
#40084=CARTESIAN_POINT('Ctrl Pts',(29.5689154366503,-1.46244305203796,34.9695750902676));
#40085=CARTESIAN_POINT('Ctrl Pts',(30.1792507153713,-1.44403741340358,34.9705529766509));
#40086=CARTESIAN_POINT('Ctrl Pts',(31.2736623104601,-1.45566276263915,34.9699414890844));
#40087=CARTESIAN_POINT('Ctrl Pts',(32.2921477181609,-1.49932800272566,34.9678399885732));
#40088=CARTESIAN_POINT('Ctrl Pts',(33.1741882479305,-1.499517595871,34.9678468028527));
#40089=CARTESIAN_POINT('Ctrl Pts',(33.4970858163865,-1.49953305131999,34.967847887745));
#40090=CARTESIAN_POINT('Ctrl Pts',(34.1585551188942,-1.49956286264318,34.9678492058823));
#40091=CARTESIAN_POINT('Ctrl Pts',(34.813787937747,-1.49965401758262,34.9678538817401));
#40092=CARTESIAN_POINT('Ctrl Pts',(35.8017689303045,-1.49967139266818,34.9678547184894));
#40093=CARTESIAN_POINT('Ctrl Pts',(37.7747836658544,-1.49977506469251,34.9678599580489));
#40094=CARTESIAN_POINT('Ctrl Pts',(39.5833333333333,-1.5,34.967871202114));
#40095=CARTESIAN_POINT('Ctrl Pts',(40.9,-1.5,34.967871202114));
#40096=CARTESIAN_POINT('Origin',(6.9,15.,25.9807621135332));
#40097=CARTESIAN_POINT('',(6.9,-8.61681422303453,28.7358750109634));
#40098=CARTESIAN_POINT('Ctrl Pts',(6.9,-3.76156693666918,10.3676856018661));
#40099=CARTESIAN_POINT('Ctrl Pts',(6.9,-4.66834435251376,14.103554168739));
#40100=CARTESIAN_POINT('Ctrl Pts',(6.90000000166257,-5.7030525211077,18.0191477848531));
#40101=CARTESIAN_POINT('Ctrl Pts',(6.90000000166257,-7.22296038005706,23.666490663791));
#40102=CARTESIAN_POINT('Ctrl Pts',(6.9,-7.92134750786926,26.2182182108371));
#40103=CARTESIAN_POINT('Ctrl Pts',(6.9,-8.61681422303453,28.7358750109634));
#40104=CARTESIAN_POINT('Origin',(6.9,0.,0.));
#40105=CARTESIAN_POINT('Origin',(40.9,4.5,7.79422863405995));
#40106=CARTESIAN_POINT('Ctrl Pts',(40.9,15.9346498339374,30.5996231131986));
#40107=CARTESIAN_POINT('Ctrl Pts',(40.9,15.6844024313584,30.1661818974695));
#40108=CARTESIAN_POINT('Ctrl Pts',(40.9,15.4341550287793,29.7327406817405));
#40109=CARTESIAN_POINT('Ctrl Pts',(40.9,15.1839076262003,29.2992994660114));
#40110=CARTESIAN_POINT('Ctrl Pts',(30.5,18.8345266621011,29.5001797522422));
#40111=CARTESIAN_POINT('Ctrl Pts',(30.5,18.176307754627,29.9204226682664));
#40112=CARTESIAN_POINT('Ctrl Pts',(30.5,17.5,30.3108891324554));
#40113=CARTESIAN_POINT('Ctrl Pts',(30.5,-12.8108891324553,47.8108891324553));
#40114=CARTESIAN_POINT('Ctrl Pts',(30.5,-30.3108891324554,17.5));
#40115=CARTESIAN_POINT('Ctrl Pts',(30.5,-47.8108891324553,-12.8108891324553));
#40116=CARTESIAN_POINT('Ctrl Pts',(30.5,-17.5,-30.3108891324554));
#40117=CARTESIAN_POINT('Ctrl Pts',(30.5,12.8108891324553,-47.8108891324553));
#40118=CARTESIAN_POINT('Ctrl Pts',(30.5,30.3108891324554,-17.5));
#40119=CARTESIAN_POINT('Ctrl Pts',(30.5,47.0470003722618,11.4877949884694));
#40120=CARTESIAN_POINT('Ctrl Pts',(30.5,18.8345266621011,29.5001797522422));
#40121=CARTESIAN_POINT('Ctrl Pts',(30.3311478274255,18.7939298193791,29.4365936489566));
#40122=CARTESIAN_POINT('Ctrl Pts',(30.3311478274255,18.1371296685291,29.8559307532302));
#40123=CARTESIAN_POINT('Ctrl Pts',(30.3311478274255,17.4622796600955,30.245555587262));
#40124=CARTESIAN_POINT('Ctrl Pts',(30.3311478274255,-12.7832759271665,47.7078352473574));
#40125=CARTESIAN_POINT('Ctrl Pts',(30.3311478274255,-30.245555587262,17.4622796600955));
#40126=CARTESIAN_POINT('Ctrl Pts',(30.3311478274255,-47.7078352473574,-12.7832759271665));
#40127=CARTESIAN_POINT('Ctrl Pts',(30.3311478274255,-17.4622796600955,-30.245555587262));
#40128=CARTESIAN_POINT('Ctrl Pts',(30.3311478274255,12.7832759271665,-47.7078352473574));
#40129=CARTESIAN_POINT('Ctrl Pts',(30.3311478274255,30.245555587262,-17.4622796600955));
#40130=CARTESIAN_POINT('Ctrl Pts',(30.3311478274255,46.9455930096601,11.4630336437998));
#40131=CARTESIAN_POINT('Ctrl Pts',(30.3311478274255,18.7939298193791,29.4365936489566));
#40132=CARTESIAN_POINT('Ctrl Pts',(29.9897712690917,18.7116961278613,29.3077924996107));
#40133=CARTESIAN_POINT('Ctrl Pts',(29.9897712690917,18.0577698358324,29.7252947753835));
#40134=CARTESIAN_POINT('Ctrl Pts',(29.9897712690917,17.3858726641896,30.1132147882992));
#40135=CARTESIAN_POINT('Ctrl Pts',(29.9897712690917,-12.7273421241096,47.4990874524888));
#40136=CARTESIAN_POINT('Ctrl Pts',(29.9897712690917,-30.1132147882992,17.3858726641896));
#40137=CARTESIAN_POINT('Ctrl Pts',(29.9897712690917,-47.4990874524888,-12.7273421241096));
#40138=CARTESIAN_POINT('Ctrl Pts',(29.9897712690917,-17.3858726641896,-30.1132147882992));
#40139=CARTESIAN_POINT('Ctrl Pts',(29.9897712690917,12.7273421241096,-47.4990874524888));
#40140=CARTESIAN_POINT('Ctrl Pts',(29.9897712690917,30.1132147882992,-17.3858726641896));
#40141=CARTESIAN_POINT('Ctrl Pts',(29.9897712690917,46.7401804402414,11.4128766206768));
#40142=CARTESIAN_POINT('Ctrl Pts',(29.9897712690917,18.7116961278613,29.3077924996107));
#40143=CARTESIAN_POINT('Ctrl Pts',(29.4666899049319,18.5852252487451,29.1097034403905));
#40144=CARTESIAN_POINT('Ctrl Pts',(29.4666899049319,17.935718792976,29.5243838511923));
#40145=CARTESIAN_POINT('Ctrl Pts',(29.4666899049319,17.2683629213518,29.9096819433198));
#40146=CARTESIAN_POINT('Ctrl Pts',(29.4666899049319,-12.641319021968,47.1780448646716));
#40147=CARTESIAN_POINT('Ctrl Pts',(29.4666899049319,-29.9096819433198,17.2683629213518));
#40148=CARTESIAN_POINT('Ctrl Pts',(29.4666899049319,-47.1780448646716,-12.641319021968));
#40149=CARTESIAN_POINT('Ctrl Pts',(29.4666899049319,-17.2683629213518,-29.9096819433198));
#40150=CARTESIAN_POINT('Ctrl Pts',(29.4666899049319,12.641319021968,-47.1780448646716));
#40151=CARTESIAN_POINT('Ctrl Pts',(29.4666899049319,29.9096819433198,-17.2683629213518));
#40152=CARTESIAN_POINT('Ctrl Pts',(29.4666899049319,46.4242672450966,11.3357378872558));
#40153=CARTESIAN_POINT('Ctrl Pts',(29.4666899049319,18.5852252487451,29.1097034403905));
#40154=CARTESIAN_POINT('Ctrl Pts',(28.7471241621752,18.4103340474916,28.8357745030392));
#40155=CARTESIAN_POINT('Ctrl Pts',(28.7471241621752,17.7669395953572,29.246552676757));
#40156=CARTESIAN_POINT('Ctrl Pts',(28.7471241621752,17.105863694435,29.6282250261092));
#40157=CARTESIAN_POINT('Ctrl Pts',(28.7471241621752,-12.5223613316743,46.7340887205442));
#40158=CARTESIAN_POINT('Ctrl Pts',(28.7471241621752,-29.6282250261092,17.105863694435));
#40159=CARTESIAN_POINT('Ctrl Pts',(28.7471241621752,-46.7340887205442,-12.5223613316743));
#40160=CARTESIAN_POINT('Ctrl Pts',(28.7471241621752,-17.105863694435,-29.6282250261092));
#40161=CARTESIAN_POINT('Ctrl Pts',(28.7471241621752,12.5223613316743,-46.7340887205442));
#40162=CARTESIAN_POINT('Ctrl Pts',(28.7471241621752,29.6282250261092,-17.105863694435));
#40163=CARTESIAN_POINT('Ctrl Pts',(28.7471241621752,45.9874043199967,11.2290660127069));
#40164=CARTESIAN_POINT('Ctrl Pts',(28.7471241621752,18.4103340474916,28.8357745030392));
#40165=CARTESIAN_POINT('Ctrl Pts',(27.8100958442934,18.1817092625453,28.4776836217162));
#40166=CARTESIAN_POINT('Ctrl Pts',(27.8100958442934,17.5463046664274,28.8833606347823));
#40167=CARTESIAN_POINT('Ctrl Pts',(27.8100958442934,16.8934381948013,29.2602932679205));
#40168=CARTESIAN_POINT('Ctrl Pts',(27.8100958442934,-12.3668550731192,46.1537314627218));
#40169=CARTESIAN_POINT('Ctrl Pts',(27.8100958442934,-29.2602932679205,16.8934381948013));
#40170=CARTESIAN_POINT('Ctrl Pts',(27.8100958442934,-46.1537314627218,-12.3668550731192));
#40171=CARTESIAN_POINT('Ctrl Pts',(27.8100958442934,-16.8934381948013,-29.2602932679205));
#40172=CARTESIAN_POINT('Ctrl Pts',(27.8100958442934,12.3668550731192,-46.1537314627218));
#40173=CARTESIAN_POINT('Ctrl Pts',(27.8100958442934,29.2602932679205,-16.8934381948013));
#40174=CARTESIAN_POINT('Ctrl Pts',(27.8100958442934,45.4163196022628,11.0896202647003));
#40175=CARTESIAN_POINT('Ctrl Pts',(27.8100958442934,18.1817092625453,28.4776836217162));
#40176=CARTESIAN_POINT('Ctrl Pts',(26.8343111708818,17.9446806017473,28.1064299010669));
#40177=CARTESIAN_POINT('Ctrl Pts',(26.8343111708818,17.3175595557791,28.5068182430991));
#40178=CARTESIAN_POINT('Ctrl Pts',(26.8343111708818,16.6732042787395,28.8788369357517));
#40179=CARTESIAN_POINT('Ctrl Pts',(26.8343111708818,-12.2056326570121,45.5520412144912));
#40180=CARTESIAN_POINT('Ctrl Pts',(26.8343111708818,-28.8788369357517,16.6732042787395));
#40181=CARTESIAN_POINT('Ctrl Pts',(26.8343111708818,-45.5520412144912,-12.2056326570121));
#40182=CARTESIAN_POINT('Ctrl Pts',(26.8343111708818,-16.6732042787395,-28.8788369357517));
#40183=CARTESIAN_POINT('Ctrl Pts',(26.8343111708818,12.2056326570121,-45.5520412144912));
#40184=CARTESIAN_POINT('Ctrl Pts',(26.8343111708818,28.8788369357517,-16.6732042787395));
#40185=CARTESIAN_POINT('Ctrl Pts',(26.8343111708818,44.8242427376375,10.9450487174303));
#40186=CARTESIAN_POINT('Ctrl Pts',(26.8343111708818,17.9446806017473,28.1064299010669));
#40187=CARTESIAN_POINT('Ctrl Pts',(25.8181479469611,17.7025946652472,27.7272550606068));
#40188=CARTESIAN_POINT('Ctrl Pts',(25.8181479469611,17.0839339083798,28.1222418918016));
#40189=CARTESIAN_POINT('Ctrl Pts',(25.8181479469611,16.4482714219305,28.4892417994669));
#40190=CARTESIAN_POINT('Ctrl Pts',(25.8181479469611,-12.0409703775363,44.9375132213974));
#40191=CARTESIAN_POINT('Ctrl Pts',(25.8181479469611,-28.4892417994669,16.4482714219305));
#40192=CARTESIAN_POINT('Ctrl Pts',(25.8181479469611,-44.9375132213974,-12.0409703775363));
#40193=CARTESIAN_POINT('Ctrl Pts',(25.8181479469611,-16.4482714219305,-28.4892417994669));
#40194=CARTESIAN_POINT('Ctrl Pts',(25.8181479469611,12.0409703775363,-44.9375132213974));
#40195=CARTESIAN_POINT('Ctrl Pts',(25.8181479469611,28.4892417994669,-16.4482714219305));
#40196=CARTESIAN_POINT('Ctrl Pts',(25.8181479469611,44.2195332406074,10.7973925719907));
#40197=CARTESIAN_POINT('Ctrl Pts',(25.8181479469611,17.7025946652472,27.7272550606068));
#40198=CARTESIAN_POINT('Ctrl Pts',(24.7595197917227,17.4614959928472,27.3496265541183));
#40199=CARTESIAN_POINT('Ctrl Pts',(24.7595197917227,16.8512610227058,27.739233902677));
#40200=CARTESIAN_POINT('Ctrl Pts',(24.7595197917227,16.2242558762949,28.1012354927406));
#40201=CARTESIAN_POINT('Ctrl Pts',(24.7595197917227,-11.8769796164457,44.3254913690355));
#40202=CARTESIAN_POINT('Ctrl Pts',(24.7595197917227,-28.1012354927406,16.2242558762949));
#40203=CARTESIAN_POINT('Ctrl Pts',(24.7595197917227,-44.3254913690355,-11.8769796164457));
#40204=CARTESIAN_POINT('Ctrl Pts',(24.7595197917227,-16.2242558762949,-28.1012354927406));
#40205=CARTESIAN_POINT('Ctrl Pts',(24.7595197917227,11.8769796164457,-44.3254913690355));
#40206=CARTESIAN_POINT('Ctrl Pts',(24.7595197917227,28.1012354927406,-16.2242558762949));
#40207=CARTESIAN_POINT('Ctrl Pts',(24.7595197917227,43.6172898429552,10.6503385912769));
#40208=CARTESIAN_POINT('Ctrl Pts',(24.7595197917227,17.4614959928472,27.3496265541183));
#40209=CARTESIAN_POINT('Ctrl Pts',(23.6563574780851,17.229354682426,26.9860278023044));
#40210=CARTESIAN_POINT('Ctrl Pts',(23.6563574780851,16.627232461942,27.370455528196));
#40211=CARTESIAN_POINT('Ctrl Pts',(23.6563574780851,16.0085630157705,27.7276444994825));
#40212=CARTESIAN_POINT('Ctrl Pts',(23.6563574780851,-11.719081483712,43.736207515253));
#40213=CARTESIAN_POINT('Ctrl Pts',(23.6563574780851,-27.7276444994825,16.0085630157705));
#40214=CARTESIAN_POINT('Ctrl Pts',(23.6563574780851,-43.736207515253,-11.719081483712));
#40215=CARTESIAN_POINT('Ctrl Pts',(23.6563574780851,-16.0085630157705,-27.7276444994825));
#40216=CARTESIAN_POINT('Ctrl Pts',(23.6563574780851,11.719081483712,-43.736207515253));
#40217=CARTESIAN_POINT('Ctrl Pts',(23.6563574780851,27.7276444994825,-16.0085630157705));
#40218=CARTESIAN_POINT('Ctrl Pts',(23.6563574780851,43.0374211521332,10.5087479991523));
#40219=CARTESIAN_POINT('Ctrl Pts',(23.6563574780851,17.229354682426,26.9860278023044));
#40220=CARTESIAN_POINT('Ctrl Pts',(22.5073180101405,17.0145388530744,26.649565639321));
#40221=CARTESIAN_POINT('Ctrl Pts',(22.5073180101405,16.419923900654,27.0292003150791));
#40222=CARTESIAN_POINT('Ctrl Pts',(22.5073180101405,15.8089680335819,27.3819358493961));
#40223=CARTESIAN_POINT('Ctrl Pts',(22.5073180101405,-11.5729678158142,43.190903882978));
#40224=CARTESIAN_POINT('Ctrl Pts',(22.5073180101405,-27.3819358493961,15.8089680335819));
#40225=CARTESIAN_POINT('Ctrl Pts',(22.5073180101405,-43.190903882978,-11.5729678158142));
#40226=CARTESIAN_POINT('Ctrl Pts',(22.5073180101405,-15.8089680335819,-27.3819358493961));
#40227=CARTESIAN_POINT('Ctrl Pts',(22.5073180101405,11.5729678158142,-43.190903882978));
#40228=CARTESIAN_POINT('Ctrl Pts',(22.5073180101405,27.3819358493961,-15.8089680335819));
#40229=CARTESIAN_POINT('Ctrl Pts',(22.5073180101405,42.5008299977716,10.3777247856603));
#40230=CARTESIAN_POINT('Ctrl Pts',(22.5073180101405,17.0145388530744,26.649565639321));
#40231=CARTESIAN_POINT('Ctrl Pts',(21.3125219557939,16.8244723890963,26.3518679613905));
#40232=CARTESIAN_POINT('Ctrl Pts',(21.3125219557939,16.2364997772301,26.727261803997));
#40233=CARTESIAN_POINT('Ctrl Pts',(21.3125219557939,15.632368792237,27.0760569908086));
#40234=CARTESIAN_POINT('Ctrl Pts',(21.3125219557939,-11.4436881985716,42.7084257830456));
#40235=CARTESIAN_POINT('Ctrl Pts',(21.3125219557939,-27.0760569908086,15.632368792237));
#40236=CARTESIAN_POINT('Ctrl Pts',(21.3125219557939,-42.7084257830456,-11.4436881985716));
#40237=CARTESIAN_POINT('Ctrl Pts',(21.3125219557939,-15.632368792237,-27.0760569908086));
#40238=CARTESIAN_POINT('Ctrl Pts',(21.3125219557939,11.4436881985716,-42.7084257830456));
#40239=CARTESIAN_POINT('Ctrl Pts',(21.3125219557939,27.0760569908086,-15.632368792237));
#40240=CARTESIAN_POINT('Ctrl Pts',(21.3125219557939,42.0260605935833,10.2617970211066));
#40241=CARTESIAN_POINT('Ctrl Pts',(21.3125219557939,16.8244723890963,26.3518679613905));
#40242=CARTESIAN_POINT('Ctrl Pts',(20.0742472323676,16.6643225955232,26.1010282252799));
#40243=CARTESIAN_POINT('Ctrl Pts',(20.0742472323676,16.0819468125049,26.4728487465358));
#40244=CARTESIAN_POINT('Ctrl Pts',(20.0742472323676,15.4835664656477,26.8183238008716));
#40245=CARTESIAN_POINT('Ctrl Pts',(20.0742472323676,-11.3347573352238,42.3018902665193));
#40246=CARTESIAN_POINT('Ctrl Pts',(20.0742472323676,-26.8183238008716,15.4835664656477));
#40247=CARTESIAN_POINT('Ctrl Pts',(20.0742472323676,-42.3018902665193,-11.3347573352238));
#40248=CARTESIAN_POINT('Ctrl Pts',(20.0742472323676,-15.4835664656477,-26.8183238008716));
#40249=CARTESIAN_POINT('Ctrl Pts',(20.0742472323676,11.3347573352238,-42.3018902665193));
#40250=CARTESIAN_POINT('Ctrl Pts',(20.0742472323676,26.8183238008716,-15.4835664656477));
#40251=CARTESIAN_POINT('Ctrl Pts',(20.0742472323676,41.6260204156154,10.1641164141543));
#40252=CARTESIAN_POINT('Ctrl Pts',(20.0742472323676,16.6643225955232,26.1010282252799));
#40253=CARTESIAN_POINT('Ctrl Pts',(18.7979917002302,16.5352770548748,25.8989065200918));
#40254=CARTESIAN_POINT('Ctrl Pts',(18.7979917002302,15.9574110860028,26.2678477295776));
#40255=CARTESIAN_POINT('Ctrl Pts',(18.7979917002302,15.3636644897785,26.6106474867381));
#40256=CARTESIAN_POINT('Ctrl Pts',(18.7979917002302,-11.2469829969596,41.9743119765166));
#40257=CARTESIAN_POINT('Ctrl Pts',(18.7979917002302,-26.6106474867381,15.3636644897785));
#40258=CARTESIAN_POINT('Ctrl Pts',(18.7979917002302,-41.9743119765166,-11.2469829969596));
#40259=CARTESIAN_POINT('Ctrl Pts',(18.7979917002302,-15.3636644897785,-26.6106474867381));
#40260=CARTESIAN_POINT('Ctrl Pts',(18.7979917002302,11.2469829969596,-41.9743119765166));
#40261=CARTESIAN_POINT('Ctrl Pts',(18.7979917002302,26.6106474867381,-15.3636644897785));
#40262=CARTESIAN_POINT('Ctrl Pts',(18.7979917002302,41.303675941138,10.0854073102973));
#40263=CARTESIAN_POINT('Ctrl Pts',(18.7979917002302,16.5352770548748,25.8989065200918));
#40264=CARTESIAN_POINT('Ctrl Pts',(17.4917404060759,16.4351406788133,25.7420647185138));
#40265=CARTESIAN_POINT('Ctrl Pts',(17.4917404060759,15.8607742221527,26.1087716481884));
#40266=CARTESIAN_POINT('Ctrl Pts',(17.4917404060759,15.2706233100072,26.4494954361781));
#40267=CARTESIAN_POINT('Ctrl Pts',(17.4917404060759,-11.1788721261709,41.7201187461852));
#40268=CARTESIAN_POINT('Ctrl Pts',(17.4917404060759,-26.4494954361781,15.2706233100072));
#40269=CARTESIAN_POINT('Ctrl Pts',(17.4917404060759,-41.7201187461852,-11.1788721261709));
#40270=CARTESIAN_POINT('Ctrl Pts',(17.4917404060759,-15.2706233100072,-26.4494954361781));
#40271=CARTESIAN_POINT('Ctrl Pts',(17.4917404060759,11.1788721261709,-41.7201187461852));
#40272=CARTESIAN_POINT('Ctrl Pts',(17.4917404060759,26.4494954361781,-15.2706233100072));
#40273=CARTESIAN_POINT('Ctrl Pts',(17.4917404060759,41.0535440314616,10.0243308532288));
#40274=CARTESIAN_POINT('Ctrl Pts',(17.4917404060759,16.4351406788133,25.7420647185138));
#40275=CARTESIAN_POINT('Ctrl Pts',(16.1647270995715,16.3596108683728,25.6237637373094));
#40276=CARTESIAN_POINT('Ctrl Pts',(16.1647270995715,15.7878839869031,25.988785417954));
#40277=CARTESIAN_POINT('Ctrl Pts',(16.1647270995715,15.2004451894511,26.3279433657953));
#40278=CARTESIAN_POINT('Ctrl Pts',(16.1647270995715,-11.1274981763442,41.5283885552464));
#40279=CARTESIAN_POINT('Ctrl Pts',(16.1647270995715,-26.3279433657953,15.2004451894511));
#40280=CARTESIAN_POINT('Ctrl Pts',(16.1647270995715,-41.5283885552464,-11.1274981763442));
#40281=CARTESIAN_POINT('Ctrl Pts',(16.1647270995715,-15.2004451894511,-26.3279433657953));
#40282=CARTESIAN_POINT('Ctrl Pts',(16.1647270995715,11.1274981763442,-41.5283885552464));
#40283=CARTESIAN_POINT('Ctrl Pts',(16.1647270995715,26.3279433657953,-15.2004451894511));
#40284=CARTESIAN_POINT('Ctrl Pts',(16.1647270995715,40.8648771706659,9.9782627468503));
#40285=CARTESIAN_POINT('Ctrl Pts',(16.1647270995715,16.3596108683728,25.6237637373094));
#40286=CARTESIAN_POINT('Ctrl Pts',(14.8263876417415,16.3032840624315,25.5355400760543));
#40287=CARTESIAN_POINT('Ctrl Pts',(14.8263876417415,15.7335256598799,25.8993049721986));
#40288=CARTESIAN_POINT('Ctrl Pts',(14.8263876417415,15.1481094381123,26.2372951854241));
#40289=CARTESIAN_POINT('Ctrl Pts',(14.8263876417415,-11.0891857473118,41.3854046235364));
#40290=CARTESIAN_POINT('Ctrl Pts',(14.8263876417415,-26.2372951854241,15.1481094381123));
#40291=CARTESIAN_POINT('Ctrl Pts',(14.8263876417415,-41.3854046235364,-11.0891857473118));
#40292=CARTESIAN_POINT('Ctrl Pts',(14.8263876417415,-15.1481094381123,-26.2372951854241));
#40293=CARTESIAN_POINT('Ctrl Pts',(14.8263876417415,11.0891857473118,-41.3854046235364));
#40294=CARTESIAN_POINT('Ctrl Pts',(14.8263876417415,26.2372951854241,-15.1481094381123));
#40295=CARTESIAN_POINT('Ctrl Pts',(14.8263876417415,40.7241777356532,9.94390718216753));
#40296=CARTESIAN_POINT('Ctrl Pts',(14.8263876417415,16.3032840624315,25.5355400760543));
#40297=CARTESIAN_POINT('Ctrl Pts',(13.4853470903953,16.260659159851,25.4687774591536));
#40298=CARTESIAN_POINT('Ctrl Pts',(13.4853470903953,15.6923903894686,25.8315912927267));
#40299=CARTESIAN_POINT('Ctrl Pts',(13.4853470903953,15.1085047372063,26.1686978312363));
#40300=CARTESIAN_POINT('Ctrl Pts',(13.4853470903953,-11.06019309403,41.2772025684426));
#40301=CARTESIAN_POINT('Ctrl Pts',(13.4853470903953,-26.1686978312363,15.1085047372063));
#40302=CARTESIAN_POINT('Ctrl Pts',(13.4853470903953,-41.2772025684426,-11.06019309403));
#40303=CARTESIAN_POINT('Ctrl Pts',(13.4853470903953,-15.1085047372063,-26.1686978312363));
#40304=CARTESIAN_POINT('Ctrl Pts',(13.4853470903953,11.06019309403,-41.2772025684426));
#40305=CARTESIAN_POINT('Ctrl Pts',(13.4853470903953,26.1686978312363,-15.1085047372063));
#40306=CARTESIAN_POINT('Ctrl Pts',(13.4853470903953,40.617704456895,9.91790885733394));
#40307=CARTESIAN_POINT('Ctrl Pts',(13.4853470903953,16.260659159851,25.4687774591536));
#40308=CARTESIAN_POINT('Ctrl Pts',(12.1482076787549,16.2272643834928,25.4164718226475));
#40309=CARTESIAN_POINT('Ctrl Pts',(12.1482076787549,15.660162675793,25.778540539635));
#40310=CARTESIAN_POINT('Ctrl Pts',(12.1482076787549,15.0774761588537,26.1149547570431));
#40311=CARTESIAN_POINT('Ctrl Pts',(12.1482076787549,-11.0374785981893,41.1924309158968));
#40312=CARTESIAN_POINT('Ctrl Pts',(12.1482076787549,-26.1149547570431,15.0774761588537));
#40313=CARTESIAN_POINT('Ctrl Pts',(12.1482076787549,-41.1924309158968,-11.0374785981893));
#40314=CARTESIAN_POINT('Ctrl Pts',(12.1482076787549,-15.0774761588537,-26.1149547570431));
#40315=CARTESIAN_POINT('Ctrl Pts',(12.1482076787549,11.0374785981893,-41.1924309158968));
#40316=CARTESIAN_POINT('Ctrl Pts',(12.1482076787549,26.1149547570431,-15.0774761588537));
#40317=CARTESIAN_POINT('Ctrl Pts',(12.1482076787549,40.5342872261919,9.89754028893978));
#40318=CARTESIAN_POINT('Ctrl Pts',(12.1482076787549,16.2272643834928,25.4164718226475));
#40319=CARTESIAN_POINT('Ctrl Pts',(10.8190675759626,16.200195342079,25.3740740708084));
#40320=CARTESIAN_POINT('Ctrl Pts',(10.8190675759626,15.6340396286792,25.7355388133451));
#40321=CARTESIAN_POINT('Ctrl Pts',(10.8190675759626,15.0523251033884,26.0713918511132));
#40322=CARTESIAN_POINT('Ctrl Pts',(10.8190675759626,-11.0190667477248,41.1237169545017));
#40323=CARTESIAN_POINT('Ctrl Pts',(10.8190675759626,-26.0713918511132,15.0523251033884));
#40324=CARTESIAN_POINT('Ctrl Pts',(10.8190675759626,-41.1237169545017,-11.0190667477248));
#40325=CARTESIAN_POINT('Ctrl Pts',(10.8190675759626,-15.0523251033884,-26.0713918511132));
#40326=CARTESIAN_POINT('Ctrl Pts',(10.8190675759626,11.0190667477248,-41.1237169545017));
#40327=CARTESIAN_POINT('Ctrl Pts',(10.8190675759626,26.0713918511132,-15.0523251033884));
#40328=CARTESIAN_POINT('Ctrl Pts',(10.8190675759626,40.4666711281441,9.88102999357243));
#40329=CARTESIAN_POINT('Ctrl Pts',(10.8190675759626,16.200195342079,25.3740740708084));
#40330=CARTESIAN_POINT('Ctrl Pts',(9.50027713254189,16.1776521900286,25.3387651379321));
#40331=CARTESIAN_POINT('Ctrl Pts',(9.50027713254189,15.6122843025816,25.6997268893332));
#40332=CARTESIAN_POINT('Ctrl Pts',(9.50027713254189,15.0313792538877,26.0351125755702));
#40333=CARTESIAN_POINT('Ctrl Pts',(9.50027713254189,-11.0037333216825,41.0664918294579));
#40334=CARTESIAN_POINT('Ctrl Pts',(9.50027713254189,-26.0351125755702,15.0313792538877));
#40335=CARTESIAN_POINT('Ctrl Pts',(9.5002771325419,-41.0664918294579,-11.0037333216825));
#40336=CARTESIAN_POINT('Ctrl Pts',(9.5002771325419,-15.0313792538877,-26.0351125755702));
#40337=CARTESIAN_POINT('Ctrl Pts',(9.5002771325419,11.0037333216825,-41.0664918294579));
#40338=CARTESIAN_POINT('Ctrl Pts',(9.50027713254189,26.0351125755702,-15.0313792538877));
#40339=CARTESIAN_POINT('Ctrl Pts',(9.50027713254189,40.4103603059007,9.86728018643391));
#40340=CARTESIAN_POINT('Ctrl Pts',(9.50027713254189,16.1776521900286,25.3387651379321));
#40341=CARTESIAN_POINT('Ctrl Pts',(8.45435372222587,16.1625070777669,25.3150436214797));
#40342=CARTESIAN_POINT('Ctrl Pts',(8.45435372222587,15.5976684735573,25.6756674495416));
#40343=CARTESIAN_POINT('Ctrl Pts',(8.45435372222587,15.0173072536015,26.0107391561104));
#40344=CARTESIAN_POINT('Ctrl Pts',(8.45435372222587,-10.9934319025089,41.0280464097118));
#40345=CARTESIAN_POINT('Ctrl Pts',(8.45435372222587,-26.0107391561104,15.0173072536015));
#40346=CARTESIAN_POINT('Ctrl Pts',(8.45435372222587,-41.0280464097118,-10.9934319025089));
#40347=CARTESIAN_POINT('Ctrl Pts',(8.45435372222587,-15.0173072536015,-26.0107391561104));
#40348=CARTESIAN_POINT('Ctrl Pts',(8.45435372222587,10.9934319025089,-41.0280464097118));
#40349=CARTESIAN_POINT('Ctrl Pts',(8.45435372222587,26.0107391561104,-15.0173072536015));
#40350=CARTESIAN_POINT('Ctrl Pts',(8.45435372222587,40.3725291400319,9.85804268618444));
#40351=CARTESIAN_POINT('Ctrl Pts',(8.45435372222587,16.1625070777669,25.3150436214797));
#40352=CARTESIAN_POINT('Ctrl Pts',(7.67514864245731,16.1526223715398,25.2995613842179));
#40353=CARTESIAN_POINT('Ctrl Pts',(7.67514864245731,15.5881292127269,25.6599646610633));
#40354=CARTESIAN_POINT('Ctrl Pts',(7.67514864245731,15.0081229315276,25.9948314436454));
#40355=CARTESIAN_POINT('Ctrl Pts',(7.67514864245731,-10.9867085121178,41.0029543751729));
#40356=CARTESIAN_POINT('Ctrl Pts',(7.67514864245731,-25.9948314436454,15.0081229315276));
#40357=CARTESIAN_POINT('Ctrl Pts',(7.67514864245731,-41.0029543751729,-10.9867085121178));
#40358=CARTESIAN_POINT('Ctrl Pts',(7.67514864245731,-15.0081229315276,-25.9948314436454));
#40359=CARTESIAN_POINT('Ctrl Pts',(7.67514864245731,10.9867085121178,-41.0029543751729));
#40360=CARTESIAN_POINT('Ctrl Pts',(7.67514864245731,25.9948314436454,-15.0081229315276));
#40361=CARTESIAN_POINT('Ctrl Pts',(7.67514864245731,40.3478380083732,9.85201367995058));
#40362=CARTESIAN_POINT('Ctrl Pts',(7.67514864245731,16.1526223715398,25.2995613842179));
#40363=CARTESIAN_POINT('Ctrl Pts',(7.15799654185577,16.1466853364124,25.2902623130707));
#40364=CARTESIAN_POINT('Ctrl Pts',(7.15799654185577,15.5823996619098,25.6505331205953));
#40365=CARTESIAN_POINT('Ctrl Pts',(7.15799654185577,15.0026065670023,25.9852768200144));
#40366=CARTESIAN_POINT('Ctrl Pts',(7.15799654185577,-10.9826702530121,40.9878833870167));
#40367=CARTESIAN_POINT('Ctrl Pts',(7.15799654185577,-25.9852768200144,15.0026065670023));
#40368=CARTESIAN_POINT('Ctrl Pts',(7.15799654185577,-40.9878833870167,-10.9826702530121));
#40369=CARTESIAN_POINT('Ctrl Pts',(7.15799654185577,-15.0026065670023,-25.9852768200144));
#40370=CARTESIAN_POINT('Ctrl Pts',(7.15799654185577,10.9826702530121,-40.9878833870167));
#40371=CARTESIAN_POINT('Ctrl Pts',(7.15799654185577,25.9852768200144,-15.0026065670023));
#40372=CARTESIAN_POINT('Ctrl Pts',(7.15799654185577,40.3330078138659,9.84839248767923));
#40373=CARTESIAN_POINT('Ctrl Pts',(7.15799654185577,16.1466853364124,25.2902623130707));
#40374=CARTESIAN_POINT('Ctrl Pts',(6.9,16.1438799960866,25.2858683590648));
#40375=CARTESIAN_POINT('Ctrl Pts',(6.9,15.5796923611089,25.6460765727998));
#40376=CARTESIAN_POINT('Ctrl Pts',(6.9,15.,25.9807621135332));
#40377=CARTESIAN_POINT('Ctrl Pts',(6.9,-10.9807621135332,40.9807621135332));
#40378=CARTESIAN_POINT('Ctrl Pts',(6.9,-25.9807621135332,15.));
#40379=CARTESIAN_POINT('Ctrl Pts',(6.9,-40.9807621135332,-10.9807621135332));
#40380=CARTESIAN_POINT('Ctrl Pts',(6.9,-15.,-25.9807621135332));
#40381=CARTESIAN_POINT('Ctrl Pts',(6.9,10.9807621135332,-40.9807621135332));
#40382=CARTESIAN_POINT('Ctrl Pts',(6.9,25.9807621135332,-15.));
#40383=CARTESIAN_POINT('Ctrl Pts',(6.9,40.3260003190816,9.84668141868804));
#40384=CARTESIAN_POINT('Ctrl Pts',(6.9,16.1438799960866,25.2858683590648));
#40385=CARTESIAN_POINT('Ctrl Pts',(6.9,-8.61681422303453,28.7358750109634));
#40386=CARTESIAN_POINT('Ctrl Pts',(7.85773098116326,-6.72950262532883,29.3220126177434));
#40387=CARTESIAN_POINT('Ctrl Pts',(8.88781981167334,-4.83176468807716,29.7139609348499));
#40388=CARTESIAN_POINT('Ctrl Pts',(10.5914578196776,-1.83991777043967,30.0626260759601));
#40389=CARTESIAN_POINT('Ctrl Pts',(11.2365058953701,-0.737334477600529,
30.1308526921615));
#40390=CARTESIAN_POINT('Ctrl Pts',(12.0558885382926,0.564998386426061,30.1493644860168));
#40391=CARTESIAN_POINT('Ctrl Pts',(12.1875764958397,0.77079883027483,30.1503477937894));
#40392=CARTESIAN_POINT('Ctrl Pts',(13.194901830313,2.32835059063959,30.1433772121647));
#40393=CARTESIAN_POINT('Ctrl Pts',(14.2258982134098,3.91692083548088,30.0606334052373));
#40394=CARTESIAN_POINT('Ctrl Pts',(18.2616480823244,8.94354621773403,29.4024246647732));
#40395=CARTESIAN_POINT('Ctrl Pts',(21.0496416709525,11.660889676038,28.796919295079));
#40396=CARTESIAN_POINT('Ctrl Pts',(25.8000196361138,14.7241675584603,29.3778263502455));
#40397=CARTESIAN_POINT('Ctrl Pts',(26.8976561124457,15.1580512376427,29.7353019177929));
#40398=CARTESIAN_POINT('Ctrl Pts',(28.0045908801237,15.5447817028247,30.0977443108623));
#40399=CARTESIAN_POINT('Ctrl Pts',(28.5235971652406,15.6994510084801,30.2828992744991));
#40400=CARTESIAN_POINT('Ctrl Pts',(29.0834839543824,15.8677990842846,30.4804113157012));
#40401=CARTESIAN_POINT('Ctrl Pts',(29.1146288039499,15.877207296405,30.4913713634453));
#40402=CARTESIAN_POINT('Ctrl Pts',(29.5949306848436,16.0210111630069,30.6609898319163));
#40403=CARTESIAN_POINT('Ctrl Pts',(30.0492939924726,16.1312811324031,30.8338536064743));
#40404=CARTESIAN_POINT('Ctrl Pts',(30.5,16.229443021655,31.0097594187194));
#40405=CARTESIAN_POINT('Ctrl Pts',(6.45331003273164,-4.07387898226151,10.2495589536195));
#40406=CARTESIAN_POINT('Ctrl Pts',(7.20830533428676,-3.54117612793135,10.4589493929845));
#40407=CARTESIAN_POINT('Ctrl Pts',(7.99943720515023,-3.00808536723907,10.6278530262205));
#40408=CARTESIAN_POINT('Ctrl Pts',(9.76195392812149,-1.87226624217412,10.8974188156737));
#40409=CARTESIAN_POINT('Ctrl Pts',(10.7319699357145,-1.2567580486118,10.978614804603));
#40410=CARTESIAN_POINT('Ctrl Pts',(12.6618070777417,-0.165209663835399,
11.0581512103982));
#40411=CARTESIAN_POINT('Ctrl Pts',(13.6366888866736,0.364704064273056,11.0460663569154));
#40412=CARTESIAN_POINT('Ctrl Pts',(15.5563694249501,1.27025231764748,10.9884970038505));
#40413=CARTESIAN_POINT('Ctrl Pts',(16.5294822240035,1.69980161462952,10.9232664847119));
#40414=CARTESIAN_POINT('Ctrl Pts',(18.4405353898675,2.41132585012623,10.79829507883));
#40415=CARTESIAN_POINT('Ctrl Pts',(19.4148048972757,2.74047342809725,10.7128845485964));
#40416=CARTESIAN_POINT('Ctrl Pts',(20.6320159197514,3.07372863623311,10.6248232626626));
#40417=CARTESIAN_POINT('Ctrl Pts',(21.1045081958651,3.19855905527616,10.5890632628362));
#40418=CARTESIAN_POINT('Ctrl Pts',(22.0534615877,3.42883778652053,10.517515820459));
#40419=CARTESIAN_POINT('Ctrl Pts',(22.7823820470183,3.58029681662344,10.4664588970829));
#40420=CARTESIAN_POINT('Ctrl Pts',(23.3297776630268,3.67835397010647,10.4341170945839));
#40421=CARTESIAN_POINT('Ctrl Pts',(23.447059931746,3.69902619132828,10.4271412460568));
#40422=CARTESIAN_POINT('Ctrl Pts',(23.6811266122301,3.73910834650872,10.4133903945396));
#40423=CARTESIAN_POINT('Ctrl Pts',(24.094173095085,3.80664723977494,10.3895545652129));
#40424=CARTESIAN_POINT('Ctrl Pts',(24.6899146335616,3.8946407511,10.3570603924452));
#40425=CARTESIAN_POINT('Ctrl Pts',(25.2912361170961,3.96994444386569,10.3283061836388));
#40426=CARTESIAN_POINT('Ctrl Pts',(25.7735285180352,4.02162740546583,10.3085973054881));
#40427=CARTESIAN_POINT('Ctrl Pts',(26.0148283477101,4.04448759176681,10.3000025859218));
#40428=CARTESIAN_POINT('Ctrl Pts',(26.5981242438445,4.09600397233593,10.2809495486037));
#40429=CARTESIAN_POINT('Ctrl Pts',(27.5413774795631,4.14752077886532,10.2607319091994));
#40430=CARTESIAN_POINT('Ctrl Pts',(28.5384263877915,4.17105255246829,10.2503835882544));
#40431=CARTESIAN_POINT('Ctrl Pts',(29.123550305837,4.18584784382927,10.2444533826691));
#40432=CARTESIAN_POINT('Ctrl Pts',(29.2812719873802,4.18934848102512,10.2430815653884));
#40433=CARTESIAN_POINT('Ctrl Pts',(29.60335738317,4.19465178436656,10.2409825864506));
#40434=CARTESIAN_POINT('Ctrl Pts',(30.1682075695061,4.19956029863434,10.2390432854401));
#40435=CARTESIAN_POINT('Ctrl Pts',(31.3151152846709,4.19601580459666,10.2404426493562));
#40436=CARTESIAN_POINT('Ctrl Pts',(32.3203773995798,4.18330340731804,10.2455622764132));
#40437=CARTESIAN_POINT('Ctrl Pts',(33.1677006908683,4.18329188254759,10.245571342205));
#40438=CARTESIAN_POINT('Ctrl Pts',(33.4949132850991,4.18329063364476,10.2455724350351));
#40439=CARTESIAN_POINT('Ctrl Pts',(34.1541785734608,4.18328832445807,10.2455743198855));
#40440=CARTESIAN_POINT('Ctrl Pts',(34.976129104799,4.18328098024987,10.2455804319184));
#40441=CARTESIAN_POINT('Ctrl Pts',(35.9637295000904,4.18327789132127,10.2455829874647));
#40442=CARTESIAN_POINT('Ctrl Pts',(37.938359040684,4.1832737025367,10.2455864680815));
#40443=CARTESIAN_POINT('Ctrl Pts',(39.5833333333333,4.18325179103929,10.2456046429336));
#40444=CARTESIAN_POINT('Ctrl Pts',(40.9,4.18325179103929,10.2456046429336));
#40445=CARTESIAN_POINT('Ctrl Pts',(6.63336813585096,-4.85602971916217,13.590868440034));
#40446=CARTESIAN_POINT('Ctrl Pts',(7.389696336477,-4.14888858981181,13.8391951107513));
#40447=CARTESIAN_POINT('Ctrl Pts',(8.18053946683774,-3.44401143686368,14.0346488726453));
#40448=CARTESIAN_POINT('Ctrl Pts',(9.94201947683641,-1.94757748540838,14.3333081335907));
#40449=CARTESIAN_POINT('Ctrl Pts',(10.9113717350149,-1.13915583855168,14.4104989873604));
#40450=CARTESIAN_POINT('Ctrl Pts',(12.8347397322171,0.286629408466322,14.4628660834127));
#40451=CARTESIAN_POINT('Ctrl Pts',(13.808142871698,0.978270473832916,14.4226409916871));
#40452=CARTESIAN_POINT('Ctrl Pts',(15.7151185916567,2.15221389622412,14.3061107665235));
#40453=CARTESIAN_POINT('Ctrl Pts',(16.6852254797785,2.70962741922244,14.2015789338064));
#40454=CARTESIAN_POINT('Ctrl Pts',(18.5768226767695,3.62608620812782,14.0076819635675));
#40455=CARTESIAN_POINT('Ctrl Pts',(19.5464729449597,4.0512053341543,13.8818273075212));
#40456=CARTESIAN_POINT('Ctrl Pts',(20.7463406818482,4.47793026920173,13.7535017581769));
#40457=CARTESIAN_POINT('Ctrl Pts',(21.2156214332097,4.63869318435446,13.7015810566902));
#40458=CARTESIAN_POINT('Ctrl Pts',(22.1537708528639,4.93390876526191,13.5988388255709));
#40459=CARTESIAN_POINT('Ctrl Pts',(22.8728508922898,5.127670732978,13.5262523639447));
#40460=CARTESIAN_POINT('Ctrl Pts',(23.4112391022538,5.25280074041755,13.48036797944));
#40461=CARTESIAN_POINT('Ctrl Pts',(23.5274006995055,5.27931561824267,13.4704404449522));
#40462=CARTESIAN_POINT('Ctrl Pts',(23.7586975975701,5.3306297071107,13.4509289072634));
#40463=CARTESIAN_POINT('Ctrl Pts',(24.1668938536999,5.41708560365398,13.417181092299));
#40464=CARTESIAN_POINT('Ctrl Pts',(24.7548128660958,5.52956305821884,13.3713845002052));
#40465=CARTESIAN_POINT('Ctrl Pts',(25.3473131502197,5.62567073595883,13.3310219589392));
#40466=CARTESIAN_POINT('Ctrl Pts',(25.8218041556281,5.69154378511353,13.3034028562425));
#40467=CARTESIAN_POINT('Ctrl Pts',(26.0589587666352,5.72065900880548,13.2913640661324));
#40468=CARTESIAN_POINT('Ctrl Pts',(26.6316948383761,5.78623492045643,13.2646759506016));
#40469=CARTESIAN_POINT('Ctrl Pts',(27.5576851463966,5.85186367837989,13.236440987388));
#40470=CARTESIAN_POINT('Ctrl Pts',(28.5507795710394,5.88219883517421,13.2219159498841));
#40471=CARTESIAN_POINT('Ctrl Pts',(29.1361849357887,5.90128718803103,13.2135466774645));
#40472=CARTESIAN_POINT('Ctrl Pts',(29.2912521292177,5.90574282943922,13.211632738116));
#40473=CARTESIAN_POINT('Ctrl Pts',(29.6100275770339,5.91253309751288,13.2086893874642));
#40474=CARTESIAN_POINT('Ctrl Pts',(30.1692894984413,5.91881362945886,13.2059721234291));
#40475=CARTESIAN_POINT('Ctrl Pts',(31.3098805820073,5.91428725204102,13.2079309635128));
#40476=CARTESIAN_POINT('Ctrl Pts',(32.3163182251692,5.89785677449483,13.215170536538));
#40477=CARTESIAN_POINT('Ctrl Pts',(33.1686695899412,5.89783797451692,13.215185743277));
#40478=CARTESIAN_POINT('Ctrl Pts',(33.4952713010558,5.89783593918779,13.2151875891279));
#40479=CARTESIAN_POINT('Ctrl Pts',(34.1548283685118,5.8978321735044,13.2151907586342));
#40480=CARTESIAN_POINT('Ctrl Pts',(34.9764778638342,5.89782019909884,13.2152010495212));
#40481=CARTESIAN_POINT('Ctrl Pts',(35.9641101124161,5.89781516246843,13.2152053506642));
#40482=CARTESIAN_POINT('Ctrl Pts',(37.9386244259607,5.89780833274506,13.2152112104218));
#40483=CARTESIAN_POINT('Ctrl Pts',(39.5833333333333,5.89777260594516,13.2152418049849));
#40484=CARTESIAN_POINT('Ctrl Pts',(40.9,5.89777260594516,13.2152418049849));
#40485=CARTESIAN_POINT('Ctrl Pts',(6.84649785567288,-6.71741536412573,21.377211306072));
#40486=CARTESIAN_POINT('Ctrl Pts',(7.61279643984166,-5.59224351411651,21.7222003209083));
#40487=CARTESIAN_POINT('Ctrl Pts',(8.41290239278216,-4.4778139915129,21.9819683115275));
#40488=CARTESIAN_POINT('Ctrl Pts',(10.1883118359637,-2.12504829883048,22.351694214315));
#40489=CARTESIAN_POINT('Ctrl Pts',(11.1645908932198,-0.860235293933499,
22.4195115822635));
#40490=CARTESIAN_POINT('Ctrl Pts',(13.104616539894,1.36442582505286,22.4060524143024));
#40491=CARTESIAN_POINT('Ctrl Pts',(14.0814329274866,2.43568052201622,22.2982732069865));
#40492=CARTESIAN_POINT('Ctrl Pts',(15.9946796213894,4.24582169215595,22.0394507048973));
#40493=CARTESIAN_POINT('Ctrl Pts',(16.9653275559585,5.10151618176833,21.8412782041901));
#40494=CARTESIAN_POINT('Ctrl Pts',(18.8448710605557,6.49486940232068,21.4842569534398));
#40495=CARTESIAN_POINT('Ctrl Pts',(19.810123630216,7.14150804350578,21.2634255374822));
#40496=CARTESIAN_POINT('Ctrl Pts',(20.9856903475788,7.78021164720303,21.0426589820636));
#40497=CARTESIAN_POINT('Ctrl Pts',(21.450037782948,8.0234729107848,20.9532273635236));
#40498=CARTESIAN_POINT('Ctrl Pts',(22.3710393802638,8.46623345546782,20.7788884454097));
#40499=CARTESIAN_POINT('Ctrl Pts',(23.0719693188992,8.75491470148122,20.6575298272077));
#40500=CARTESIAN_POINT('Ctrl Pts',(23.5926347936587,8.94023465873174,20.5813719818061));
#40501=CARTESIAN_POINT('Ctrl Pts',(23.7065892332644,8.98001571960572,20.5647099449239));
#40502=CARTESIAN_POINT('Ctrl Pts',(23.9323706520528,9.05664995495951,20.5321468576875));
#40503=CARTESIAN_POINT('Ctrl Pts',(24.3307466212144,9.18574049076631,20.4759485784751));
#40504=CARTESIAN_POINT('Ctrl Pts',(24.9023508233185,9.35309964749801,20.4001844372317));
#40505=CARTESIAN_POINT('Ctrl Pts',(25.4757972573111,9.49555868076778,20.3338472412532));
#40506=CARTESIAN_POINT('Ctrl Pts',(25.9330914993694,9.5928869770777,20.28864648982));
#40507=CARTESIAN_POINT('Ctrl Pts',(26.1609781823312,9.63581705245677,20.2689918009898));
#40508=CARTESIAN_POINT('Ctrl Pts',(26.709932241435,9.73235004955936,20.2254900271808));
#40509=CARTESIAN_POINT('Ctrl Pts',(27.5959509089719,9.82915847887794,20.1795241403997));
#40510=CARTESIAN_POINT('Ctrl Pts',(28.579749560637,9.87532060641944,20.155272253243));
#40511=CARTESIAN_POINT('Ctrl Pts',(29.1657855350677,9.90441669946594,20.1412111689925));
#40512=CARTESIAN_POINT('Ctrl Pts',(29.3146731630637,9.9109781197532,20.1381027603739));
#40513=CARTESIAN_POINT('Ctrl Pts',(29.6257300067643,9.92113271524803,20.1332492263269));
#40514=CARTESIAN_POINT('Ctrl Pts',(30.1719452394076,9.93050366138696,20.1287785103479));
#40515=CARTESIAN_POINT('Ctrl Pts',(31.2977811219682,9.923768747263,20.1319916124711));
#40516=CARTESIAN_POINT('Ctrl Pts',(32.3069259117671,9.8985708956696,20.1442225454147));
#40517=CARTESIAN_POINT('Ctrl Pts',(33.1709940314752,9.89851679451553,20.1442592438603));
#40518=CARTESIAN_POINT('Ctrl Pts',(33.4961680489761,9.89851046735387,20.1442637388652));
#40519=CARTESIAN_POINT('Ctrl Pts',(34.1564024558335,9.89849933968833,20.1442714128625));
#40520=CARTESIAN_POINT('Ctrl Pts',(34.9773378017947,9.8984634550922,20.1442963704308));
#40521=CARTESIAN_POINT('Ctrl Pts',(35.9650395265661,9.89844842592581,20.1443067963913));
#40522=CARTESIAN_POINT('Ctrl Pts',(37.9392783163648,9.8984279817608,20.1443210056784));
#40523=CARTESIAN_POINT('Ctrl Pts',(39.5833333333333,9.89832117405885,20.1443951831047));
#40524=CARTESIAN_POINT('Ctrl Pts',(40.9,9.89832117405885,20.1443951831047));
#40525=CARTESIAN_POINT('Ctrl Pts',(6.90857970435318,-8.71018585725741,29.1272609852091));
#40526=CARTESIAN_POINT('Ctrl Pts',(7.67983757144493,-7.1626049441802,29.5775536996439));
#40527=CARTESIAN_POINT('Ctrl Pts',(8.48457055999567,-5.63283520142949,29.9097225030882));
#40528=CARTESIAN_POINT('Ctrl Pts',(10.2689932185249,-2.41146069737718,30.3644487697131));
#40529=CARTESIAN_POINT('Ctrl Pts',(11.2491988139072,-0.683672158318406,
30.4296414097155));
#40530=CARTESIAN_POINT('Ctrl Pts',(13.2074449203971,2.36894751212038,30.3576235761245));
#40531=CARTESIAN_POINT('Ctrl Pts',(14.1878085217557,3.82665309566742,30.184965998838));
#40532=CARTESIAN_POINT('Ctrl Pts',(16.1228140255812,6.30658851121944,29.7814752498472));
#40533=CARTESIAN_POINT('Ctrl Pts',(17.0983171044692,7.46839135174002,29.4886591763939));
#40534=CARTESIAN_POINT('Ctrl Pts',(18.9977376700381,9.36704911481261,28.960082872958));
#40535=CARTESIAN_POINT('Ctrl Pts',(19.9674462816337,10.2409515663328,28.6415548808294));
#40536=CARTESIAN_POINT('Ctrl Pts',(21.147106003231,11.1004135437216,28.3239820751166));
#40537=CARTESIAN_POINT('Ctrl Pts',(21.6116736136675,11.4272945418467,28.1962714220824));
#40538=CARTESIAN_POINT('Ctrl Pts',(22.5321107331755,12.0202838349911,27.948540960796));
#40539=CARTESIAN_POINT('Ctrl Pts',(23.2282372947769,12.4035528917693,27.7781185470828));
#40540=CARTESIAN_POINT('Ctrl Pts',(23.7411423015336,12.6473785079706,27.6723004799184));
#40541=CARTESIAN_POINT('Ctrl Pts',(23.8541050059083,12.7001926206312,27.6489722597557));
#40542=CARTESIAN_POINT('Ctrl Pts',(24.0772792343329,12.8015323632731,27.6035767537811));
#40543=CARTESIAN_POINT('Ctrl Pts',(24.4706231308706,12.9720321690745,27.5254067801747));
#40544=CARTESIAN_POINT('Ctrl Pts',(25.0326506601034,13.1919318242548,27.4207276483819));
#40545=CARTESIAN_POINT('Ctrl Pts',(25.5929166162092,13.3777331675808,27.3299203180183));
#40546=CARTESIAN_POINT('Ctrl Pts',(26.036986986334,13.5038445845534,27.2685418388));
#40547=CARTESIAN_POINT('Ctrl Pts',(26.257289284528,13.5592118403736,27.2420133361897));
#40548=CARTESIAN_POINT('Ctrl Pts',(26.7861809172635,13.6833062419416,27.1835476308027));
#40549=CARTESIAN_POINT('Ctrl Pts',(27.6340630276978,13.8074117592232,27.1220525704358));
#40550=CARTESIAN_POINT('Ctrl Pts',(28.6084466264574,13.8693290201703,27.0881176443602));
#40551=CARTESIAN_POINT('Ctrl Pts',(29.1951297895239,13.908430904103,27.0683644245336));
#40552=CARTESIAN_POINT('Ctrl Pts',(29.3379067795074,13.9168171018367,27.0642236253566));
#40553=CARTESIAN_POINT('Ctrl Pts',(29.6412852452592,13.9300946799831,27.0575993546201));
#40554=CARTESIAN_POINT('Ctrl Pts',(30.1744790744103,13.9423073235084,27.0515191755617));
#40555=CARTESIAN_POINT('Ctrl Pts',(31.285567721335,13.933569334585,27.0558675796336));
#40556=CARTESIAN_POINT('Ctrl Pts',(32.2974599236722,13.8994232817537,27.0731946134563));
#40557=CARTESIAN_POINT('Ctrl Pts',(33.1732579076352,13.8993047075201,27.0732696672437));
#40558=CARTESIAN_POINT('Ctrl Pts',(33.4970065888605,13.8992904506871,27.0732789151668));
#40559=CARTESIAN_POINT('Ctrl Pts',(34.1579215418456,13.8992658208367,27.0732946436726));
#40560=CARTESIAN_POINT('Ctrl Pts',(34.9781539333149,13.8991859907804,27.0733458523267));
#40561=CARTESIAN_POINT('Ctrl Pts',(35.9659297143336,13.8991526077107,27.0733672375489));
#40562=CARTESIAN_POINT('Ctrl Pts',(37.9398993196362,13.8991071452309,27.0733963900547));
#40563=CARTESIAN_POINT('Ctrl Pts',(39.5833333333333,13.8988697421725,27.0735485612246));
#40564=CARTESIAN_POINT('Ctrl Pts',(40.9,13.8988697421725,27.0735485612246));
#40565=CARTESIAN_POINT('Ctrl Pts',(6.93528330520032,-9.8656348186849,33.5512413216408));
#40566=CARTESIAN_POINT('Ctrl Pts',(7.70864561497005,-8.0776580699914,34.0623374960229));
#40567=CARTESIAN_POINT('Ctrl Pts',(8.5154187135237,-6.31093086144102,34.4367698578614));
#40568=CARTESIAN_POINT('Ctrl Pts',(10.3035747340622,-2.59403255178489,34.941954951338));
#40569=CARTESIAN_POINT('Ctrl Pts',(11.2855474597114,-0.60186360733143,35.0067705115655));
#40570=CARTESIAN_POINT('Ctrl Pts',(13.2510271399958,2.92382891559037,34.9032893217431));
#40571=CARTESIAN_POINT('Ctrl Pts',(14.2329608248363,4.60257161238984,34.6945593989859));
#40572=CARTESIAN_POINT('Ctrl Pts',(16.1768697182175,7.46747574760142,34.2095752766377));
#40573=CARTESIAN_POINT('Ctrl Pts',(17.1545233971705,8.80499374792143,33.8632511750181));
#40574=CARTESIAN_POINT('Ctrl Pts',(19.0635787323925,10.9976618314205,33.2359528227277));
#40575=CARTESIAN_POINT('Ctrl Pts',(20.0357940514507,12.0029926013879,32.8613840028835));
#40576=CARTESIAN_POINT('Ctrl Pts',(21.2200273744511,12.9932317593816,32.4867165469277));
#40577=CARTESIAN_POINT('Ctrl Pts',(21.6852779128345,13.3687144259959,32.3368305207218));
#40578=CARTESIAN_POINT('Ctrl Pts',(22.6074094382988,14.0501505350056,32.0460468583652));
#40579=CARTESIAN_POINT('Ctrl Pts',(23.303404556016,14.4891819334101,31.8467199720656));
#40580=CARTESIAN_POINT('Ctrl Pts',(23.8143672767891,14.7674149360666,31.7234333079367));
#40581=CARTESIAN_POINT('Ctrl Pts',(23.9270724954075,14.8277950271988,31.6962311639846));
#40582=CARTESIAN_POINT('Ctrl Pts',(24.1495225469485,14.9435144746797,31.6433583861176));
#40583=CARTESIAN_POINT('Ctrl Pts',(24.5413305977737,15.1380475804188,31.5524212197088));
#40584=CARTESIAN_POINT('Ctrl Pts',(25.09998893572,15.3882930140603,31.4310156375918));
#40585=CARTESIAN_POINT('Ctrl Pts',(25.6548568854792,15.5988027583032,31.3262265443364));
#40586=CARTESIAN_POINT('Ctrl Pts',(26.0929602492094,15.741087693316,31.2557376661541));
#40587=CARTESIAN_POINT('Ctrl Pts',(26.3096479269533,15.8033473177939,31.2253935968531));
#40588=CARTESIAN_POINT('Ctrl Pts',(26.8287121638341,15.9425694431084,31.1587088311854));
#40589=CARTESIAN_POINT('Ctrl Pts',(27.6557884297532,16.0810926132799,31.0890012981156));
#40590=CARTESIAN_POINT('Ctrl Pts',(28.624709126668,16.1519656805034,31.0495586097517));
#40591=CARTESIAN_POINT('Ctrl Pts',(29.2117706203409,16.1967753671696,31.0265558099781));
#40592=CARTESIAN_POINT('Ctrl Pts',(29.351092195488,16.206115111319,31.021876437373));
#40593=CARTESIAN_POINT('Ctrl Pts',(29.6501043905815,16.2210980111665,31.014285796168));
#40594=CARTESIAN_POINT('Ctrl Pts',(30.175870201979,16.2348498398373,31.0073340046886));
#40595=CARTESIAN_POINT('Ctrl Pts',(31.278535210342,16.2250286703999,31.0122942956317));
#40596=CARTESIAN_POINT('Ctrl Pts',(32.2920164760146,16.1856975481828,31.0325718136053));
#40597=CARTESIAN_POINT('Ctrl Pts',(33.1745232741631,16.1855272745483,31.0326760798738));
#40598=CARTESIAN_POINT('Ctrl Pts',(33.4974585875216,16.1855064782319,31.0326890056743));
#40599=CARTESIAN_POINT('Ctrl Pts',(34.1587639155491,16.1854709093049,31.0327109045834));
#40600=CARTESIAN_POINT('Ctrl Pts',(34.9785998474407,16.1853552918985,31.0327822824583));
#40601=CARTESIAN_POINT('Ctrl Pts',(35.9664200829455,16.1853069853609,31.0328120805002));
#40602=CARTESIAN_POINT('Ctrl Pts',(37.9402388284556,16.185241157271,31.0328527115372));
#40603=CARTESIAN_POINT('Ctrl Pts',(39.5833333333333,16.1848974953804,31.033064777293));
#40604=CARTESIAN_POINT('Ctrl Pts',(40.9,16.1848974953804,31.033064777293));
#40605=CARTESIAN_POINT('Origin',(6.9,25.9807621135332,15.));
#40606=CARTESIAN_POINT('',(6.9,6.90555748864272,29.194404870986));
#40607=CARTESIAN_POINT('Ctrl Pts',(6.9,1.9262302757419,10.8594625780008));
#40608=CARTESIAN_POINT('Ctrl Pts',(6.9,3.00887228147899,14.5482083700348));
#40609=CARTESIAN_POINT('Ctrl Pts',(6.90000000166257,4.07058553003038,18.4565659967827));
#40610=CARTESIAN_POINT('Ctrl Pts',(6.90000000166257,5.57797815223758,24.1072623232988));
#40611=CARTESIAN_POINT('Ctrl Pts',(6.9,6.24902093139924,26.6663167664834));
#40612=CARTESIAN_POINT('Ctrl Pts',(6.9,6.90555748864272,29.194404870986));
#40613=CARTESIAN_POINT('Origin',(6.9,0.,0.));
#40614=CARTESIAN_POINT('Origin',(40.9,7.79422863405995,4.5));
#40615=CARTESIAN_POINT('Ctrl Pts',(40.9,29.0996231131986,18.5327260452907));
#40616=CARTESIAN_POINT('Ctrl Pts',(40.9,28.6661818974695,18.2824786427117));
#40617=CARTESIAN_POINT('Ctrl Pts',(40.9,28.2327406817405,18.0322312401326));
#40618=CARTESIAN_POINT('Ctrl Pts',(40.9,27.7992994660114,17.7819838375536));
#40619=CARTESIAN_POINT('Ctrl Pts',(30.5,31.061268433756,16.1306417505986));
#40620=CARTESIAN_POINT('Ctrl Pts',(30.5,30.7013555966443,16.823692245373));
#40621=CARTESIAN_POINT('Ctrl Pts',(30.5,30.3108891324554,17.5));
#40622=CARTESIAN_POINT('Ctrl Pts',(30.5,12.8108891324554,47.8108891324553));
#40623=CARTESIAN_POINT('Ctrl Pts',(30.5,-17.5,30.3108891324554));
#40624=CARTESIAN_POINT('Ctrl Pts',(30.5,-47.8108891324553,12.8108891324554));
#40625=CARTESIAN_POINT('Ctrl Pts',(30.5,-30.3108891324554,-17.5));
#40626=CARTESIAN_POINT('Ctrl Pts',(30.5,-12.8108891324554,-47.8108891324553));
#40627=CARTESIAN_POINT('Ctrl Pts',(30.5,17.5,-30.3108891324554));
#40628=CARTESIAN_POINT('Ctrl Pts',(30.5,46.4877949884694,-13.5747778926489));
#40629=CARTESIAN_POINT('Ctrl Pts',(30.5,31.061268433756,16.1306417505986));
#40630=CARTESIAN_POINT('Ctrl Pts',(30.3311478274255,30.9943174850025,16.0958729911865));
#40631=CARTESIAN_POINT('Ctrl Pts',(30.3311478274255,30.6351804212937,16.7874296516619));
#40632=CARTESIAN_POINT('Ctrl Pts',(30.3311478274255,30.245555587262,17.4622796600955));
#40633=CARTESIAN_POINT('Ctrl Pts',(30.3311478274255,12.7832759271665,47.7078352473574));
#40634=CARTESIAN_POINT('Ctrl Pts',(30.3311478274255,-17.4622796600955,30.245555587262));
#40635=CARTESIAN_POINT('Ctrl Pts',(30.3311478274255,-47.7078352473574,12.7832759271665));
#40636=CARTESIAN_POINT('Ctrl Pts',(30.3311478274255,-30.245555587262,-17.4622796600955));
#40637=CARTESIAN_POINT('Ctrl Pts',(30.3311478274255,-12.7832759271665,-47.7078352473574));
#40638=CARTESIAN_POINT('Ctrl Pts',(30.3311478274255,17.4622796600955,-30.245555587262));
#40639=CARTESIAN_POINT('Ctrl Pts',(30.3311478274255,46.3875929639907,-13.5455181648638));
#40640=CARTESIAN_POINT('Ctrl Pts',(30.3311478274255,30.9943174850025,16.0958729911865));
#40641=CARTESIAN_POINT('Ctrl Pts',(29.9897712690917,30.8587004444282,16.0254447695752));
#40642=CARTESIAN_POINT('Ctrl Pts',(29.9897712690917,30.501134801215,16.7139754925468));
#40643=CARTESIAN_POINT('Ctrl Pts',(29.9897712690917,30.1132147882992,17.3858726641896));
#40644=CARTESIAN_POINT('Ctrl Pts',(29.9897712690917,12.7273421241097,47.4990874524888));
#40645=CARTESIAN_POINT('Ctrl Pts',(29.9897712690917,-17.3858726641896,30.1132147882992));
#40646=CARTESIAN_POINT('Ctrl Pts',(29.9897712690917,-47.4990874524888,12.7273421241097));
#40647=CARTESIAN_POINT('Ctrl Pts',(29.9897712690917,-30.1132147882992,-17.3858726641896));
#40648=CARTESIAN_POINT('Ctrl Pts',(29.9897712690917,-12.7273421241097,-47.4990874524888));
#40649=CARTESIAN_POINT('Ctrl Pts',(29.9897712690917,17.3858726641896,-30.1132147882992));
#40650=CARTESIAN_POINT('Ctrl Pts',(29.9897712690917,46.1846219490559,-13.4862491363571));
#40651=CARTESIAN_POINT('Ctrl Pts',(29.9897712690917,30.8587004444282,16.0254447695752));
#40652=CARTESIAN_POINT('Ctrl Pts',(29.4666899049319,30.6501289206644,15.9171300516369));
#40653=CARTESIAN_POINT('Ctrl Pts',(29.4666899049319,30.2949800354474,16.6010070497276));
#40654=CARTESIAN_POINT('Ctrl Pts',(29.4666899049319,29.9096819433198,17.2683629213518));
#40655=CARTESIAN_POINT('Ctrl Pts',(29.4666899049319,12.641319021968,47.1780448646716));
#40656=CARTESIAN_POINT('Ctrl Pts',(29.4666899049319,-17.2683629213518,29.9096819433198));
#40657=CARTESIAN_POINT('Ctrl Pts',(29.4666899049319,-47.1780448646716,12.641319021968));
#40658=CARTESIAN_POINT('Ctrl Pts',(29.4666899049319,-29.9096819433198,-17.2683629213518));
#40659=CARTESIAN_POINT('Ctrl Pts',(29.4666899049319,-12.641319021968,-47.1780448646716));
#40660=CARTESIAN_POINT('Ctrl Pts',(29.4666899049319,17.2683629213518,-29.9096819433198));
#40661=CARTESIAN_POINT('Ctrl Pts',(29.4666899049319,45.8724637299593,-13.3950966415431));
#40662=CARTESIAN_POINT('Ctrl Pts',(29.4666899049319,30.6501289206644,15.9171300516369));
#40663=CARTESIAN_POINT('Ctrl Pts',(28.7471241621752,30.3617042288049,15.7673462336858));
#40664=CARTESIAN_POINT('Ctrl Pts',(28.7471241621752,30.0098973754615,16.4447877935127));
#40665=CARTESIAN_POINT('Ctrl Pts',(28.7471241621752,29.6282250261092,17.105863694435));
#40666=CARTESIAN_POINT('Ctrl Pts',(28.7471241621752,12.5223613316743,46.7340887205442));
#40667=CARTESIAN_POINT('Ctrl Pts',(28.7471241621752,-17.105863694435,29.6282250261092));
#40668=CARTESIAN_POINT('Ctrl Pts',(28.7471241621752,-46.7340887205442,12.5223613316743));
#40669=CARTESIAN_POINT('Ctrl Pts',(28.7471241621752,-29.6282250261092,-17.105863694435));
#40670=CARTESIAN_POINT('Ctrl Pts',(28.7471241621752,-12.5223613316743,-46.7340887205442));
#40671=CARTESIAN_POINT('Ctrl Pts',(28.7471241621752,17.105863694435,-29.6282250261092));
#40672=CARTESIAN_POINT('Ctrl Pts',(28.7471241621752,45.4407934015768,-13.2690457322218));
#40673=CARTESIAN_POINT('Ctrl Pts',(28.7471241621752,30.3617042288049,15.7673462336858));
#40674=CARTESIAN_POINT('Ctrl Pts',(27.8100958442934,29.9846639164451,15.5715428260696));
#40675=CARTESIAN_POINT('Ctrl Pts',(27.8100958442934,29.6372259010587,16.2405717231752));
#40676=CARTESIAN_POINT('Ctrl Pts',(27.8100958442934,29.2602932679205,16.8934381948013));
#40677=CARTESIAN_POINT('Ctrl Pts',(27.8100958442934,12.3668550731192,46.1537314627218));
#40678=CARTESIAN_POINT('Ctrl Pts',(27.8100958442934,-16.8934381948013,29.2602932679205));
#40679=CARTESIAN_POINT('Ctrl Pts',(27.8100958442934,-46.1537314627218,12.3668550731192));
#40680=CARTESIAN_POINT('Ctrl Pts',(27.8100958442934,-29.2602932679205,-16.8934381948013));
#40681=CARTESIAN_POINT('Ctrl Pts',(27.8100958442934,-12.3668550731192,-46.1537314627218));
#40682=CARTESIAN_POINT('Ctrl Pts',(27.8100958442934,16.8934381948013,-29.2602932679205));
#40683=CARTESIAN_POINT('Ctrl Pts',(27.8100958442934,44.8764966543029,-13.1042669335782));
#40684=CARTESIAN_POINT('Ctrl Pts',(27.8100958442934,29.9846639164451,15.5715428260696));
#40685=CARTESIAN_POINT('Ctrl Pts',(26.8343111708818,29.5937642144445,15.3685420031368));
#40686=CARTESIAN_POINT('Ctrl Pts',(26.8343111708818,29.2508556284042,16.0288490017));
#40687=CARTESIAN_POINT('Ctrl Pts',(26.8343111708818,28.8788369357517,16.6732042787395));
#40688=CARTESIAN_POINT('Ctrl Pts',(26.8343111708818,12.2056326570121,45.5520412144912));
#40689=CARTESIAN_POINT('Ctrl Pts',(26.8343111708818,-16.6732042787395,28.8788369357517));
#40690=CARTESIAN_POINT('Ctrl Pts',(26.8343111708818,-45.5520412144912,12.2056326570121));
#40691=CARTESIAN_POINT('Ctrl Pts',(26.8343111708818,-28.8788369357517,-16.6732042787395));
#40692=CARTESIAN_POINT('Ctrl Pts',(26.8343111708818,-12.2056326570121,-45.5520412144912));
#40693=CARTESIAN_POINT('Ctrl Pts',(26.8343111708818,16.6732042787395,-28.8788369357517));
#40694=CARTESIAN_POINT('Ctrl Pts',(26.8343111708818,44.2914572749094,-12.9334311338658));
#40695=CARTESIAN_POINT('Ctrl Pts',(26.8343111708818,29.5937642144445,15.3685420031368));
#40696=CARTESIAN_POINT('Ctrl Pts',(25.8181479469611,29.1945242233064,15.1612099270726));
#40697=CARTESIAN_POINT('Ctrl Pts',(25.8181479469611,28.8562417071321,15.8126089354813));
#40698=CARTESIAN_POINT('Ctrl Pts',(25.8181479469611,28.4892417994669,16.4482714219305));
#40699=CARTESIAN_POINT('Ctrl Pts',(25.8181479469611,12.0409703775363,44.9375132213974));
#40700=CARTESIAN_POINT('Ctrl Pts',(25.8181479469611,-16.4482714219305,28.4892417994669));
#40701=CARTESIAN_POINT('Ctrl Pts',(25.8181479469611,-44.9375132213974,12.0409703775363));
#40702=CARTESIAN_POINT('Ctrl Pts',(25.8181479469611,-28.4892417994669,-16.4482714219305));
#40703=CARTESIAN_POINT('Ctrl Pts',(25.8181479469611,-12.0409703775363,-44.9375132213974));
#40704=CARTESIAN_POINT('Ctrl Pts',(25.8181479469611,16.4482714219305,-28.4892417994669));
#40705=CARTESIAN_POINT('Ctrl Pts',(25.8181479469611,43.6939354158518,-12.7589503583263));
#40706=CARTESIAN_POINT('Ctrl Pts',(25.8181479469611,29.1945242233064,15.1612099270726));
#40707=CARTESIAN_POINT('Ctrl Pts',(24.7595197917227,28.796912394945,14.9547233834603));
#40708=CARTESIAN_POINT('Ctrl Pts',(24.7595197917227,28.4632370828042,15.5972507298839));
#40709=CARTESIAN_POINT('Ctrl Pts',(24.7595197917227,28.1012354927406,16.2242558762949));
#40710=CARTESIAN_POINT('Ctrl Pts',(24.7595197917227,11.8769796164458,44.3254913690355));
#40711=CARTESIAN_POINT('Ctrl Pts',(24.7595197917227,-16.2242558762949,28.1012354927406));
#40712=CARTESIAN_POINT('Ctrl Pts',(24.7595197917227,-44.3254913690355,11.8769796164458));
#40713=CARTESIAN_POINT('Ctrl Pts',(24.7595197917227,-28.1012354927406,-16.2242558762949));
#40714=CARTESIAN_POINT('Ctrl Pts',(24.7595197917227,-11.8769796164458,-44.3254913690355));
#40715=CARTESIAN_POINT('Ctrl Pts',(24.7595197917227,16.2242558762949,-28.1012354927406));
#40716=CARTESIAN_POINT('Ctrl Pts',(24.7595197917227,43.0988503438666,-12.5851811425261));
#40717=CARTESIAN_POINT('Ctrl Pts',(24.7595197917227,28.796912394945,14.9547233834603));
#40718=CARTESIAN_POINT('Ctrl Pts',(23.6563574780851,28.4140727469455,14.7559082828157));
#40719=CARTESIAN_POINT('Ctrl Pts',(23.6563574780851,28.084833470769,15.389893569599));
#40720=CARTESIAN_POINT('Ctrl Pts',(23.6563574780851,27.7276444994825,16.0085630157705));
#40721=CARTESIAN_POINT('Ctrl Pts',(23.6563574780851,11.719081483712,43.736207515253));
#40722=CARTESIAN_POINT('Ctrl Pts',(23.6563574780851,-16.0085630157705,27.7276444994825));
#40723=CARTESIAN_POINT('Ctrl Pts',(23.6563574780851,-43.736207515253,11.719081483712));
#40724=CARTESIAN_POINT('Ctrl Pts',(23.6563574780851,-27.7276444994825,-16.0085630157705));
#40725=CARTESIAN_POINT('Ctrl Pts',(23.6563574780851,-11.719081483712,-43.736207515253));
#40726=CARTESIAN_POINT('Ctrl Pts',(23.6563574780851,16.0085630157705,-27.7276444994825));
#40727=CARTESIAN_POINT('Ctrl Pts',(23.6563574780851,42.5258740306932,-12.4178678468319));
#40728=CARTESIAN_POINT('Ctrl Pts',(23.6563574780851,28.4140727469455,14.7559082828157));
#40729=CARTESIAN_POINT('Ctrl Pts',(22.5073180101405,28.0598057001003,14.5719314169357));
#40730=CARTESIAN_POINT('Ctrl Pts',(22.5073180101405,27.7346713837132,15.1980121665098));
#40731=CARTESIAN_POINT('Ctrl Pts',(22.5073180101405,27.3819358493961,15.8089680335819));
#40732=CARTESIAN_POINT('Ctrl Pts',(22.5073180101405,11.5729678158142,43.190903882978));
#40733=CARTESIAN_POINT('Ctrl Pts',(22.5073180101405,-15.8089680335819,27.3819358493961));
#40734=CARTESIAN_POINT('Ctrl Pts',(22.5073180101405,-43.190903882978,11.5729678158142));
#40735=CARTESIAN_POINT('Ctrl Pts',(22.5073180101405,-27.3819358493961,-15.8089680335819));
#40736=CARTESIAN_POINT('Ctrl Pts',(22.5073180101405,-11.5729678158142,-43.190903882978));
#40737=CARTESIAN_POINT('Ctrl Pts',(22.5073180101405,15.8089680335819,-27.3819358493961));
#40738=CARTESIAN_POINT('Ctrl Pts',(22.5073180101405,41.9956608528241,-12.2630417010206));
#40739=CARTESIAN_POINT('Ctrl Pts',(22.5073180101405,28.0598057001003,14.5719314169357));
#40740=CARTESIAN_POINT('Ctrl Pts',(21.3125219557939,27.7463544749225,14.4091508971893));
#40741=CARTESIAN_POINT('Ctrl Pts',(21.3125219557939,27.4248521776202,15.0282378072439));
#40742=CARTESIAN_POINT('Ctrl Pts',(21.3125219557939,27.0760569908086,15.632368792237));
#40743=CARTESIAN_POINT('Ctrl Pts',(21.3125219557939,11.4436881985716,42.7084257830456));
#40744=CARTESIAN_POINT('Ctrl Pts',(21.3125219557939,-15.632368792237,27.0760569908086));
#40745=CARTESIAN_POINT('Ctrl Pts',(21.3125219557939,-42.7084257830456,11.4436881985716));
#40746=CARTESIAN_POINT('Ctrl Pts',(21.3125219557939,-27.0760569908086,-15.632368792237));
#40747=CARTESIAN_POINT('Ctrl Pts',(21.3125219557939,-11.4436881985716,-42.7084257830456));
#40748=CARTESIAN_POINT('Ctrl Pts',(21.3125219557939,15.632368792237,-27.0760569908086));
#40749=CARTESIAN_POINT('Ctrl Pts',(21.3125219557939,41.5265346055806,-12.1260533880339));
#40750=CARTESIAN_POINT('Ctrl Pts',(21.3125219557939,27.7463544749225,14.4091508971893));
#40751=CARTESIAN_POINT('Ctrl Pts',(20.0742472323676,27.4822408172221,14.2719922102254));
#40752=CARTESIAN_POINT('Ctrl Pts',(20.0742472323676,27.1637988552073,14.8851861187906));
#40753=CARTESIAN_POINT('Ctrl Pts',(20.0742472323676,26.8183238008716,15.4835664656477));
#40754=CARTESIAN_POINT('Ctrl Pts',(20.0742472323676,11.3347573352238,42.3018902665193));
#40755=CARTESIAN_POINT('Ctrl Pts',(20.0742472323676,-15.4835664656477,26.8183238008716));
#40756=CARTESIAN_POINT('Ctrl Pts',(20.0742472323676,-42.3018902665193,11.3347573352238));
#40757=CARTESIAN_POINT('Ctrl Pts',(20.0742472323676,-26.8183238008716,-15.4835664656477));
#40758=CARTESIAN_POINT('Ctrl Pts',(20.0742472323676,-11.3347573352238,-42.3018902665193));
#40759=CARTESIAN_POINT('Ctrl Pts',(20.0742472323676,15.4835664656477,-26.8183238008716));
#40760=CARTESIAN_POINT('Ctrl Pts',(20.0742472323676,41.1312493454498,-12.0106271861277));
#40761=CARTESIAN_POINT('Ctrl Pts',(20.0742472323676,27.4822408172221,14.2719922102254));
#40762=CARTESIAN_POINT('Ctrl Pts',(18.7979917002302,27.2694232481814,14.1614724492006));
#40763=CARTESIAN_POINT('Ctrl Pts',(18.7979917002302,26.9534472438987,14.7699178935542));
#40764=CARTESIAN_POINT('Ctrl Pts',(18.7979917002302,26.6106474867381,15.3636644897785));
#40765=CARTESIAN_POINT('Ctrl Pts',(18.7979917002302,11.2469829969596,41.9743119765166));
#40766=CARTESIAN_POINT('Ctrl Pts',(18.7979917002302,-15.3636644897785,26.6106474867381));
#40767=CARTESIAN_POINT('Ctrl Pts',(18.7979917002302,-41.9743119765166,11.2469829969596));
#40768=CARTESIAN_POINT('Ctrl Pts',(18.7979917002302,-26.6106474867381,-15.3636644897785));
#40769=CARTESIAN_POINT('Ctrl Pts',(18.7979917002302,-11.2469829969596,-41.9743119765166));
#40770=CARTESIAN_POINT('Ctrl Pts',(18.7979917002302,15.3636644897785,-26.6106474867381));
#40771=CARTESIAN_POINT('Ctrl Pts',(18.7979917002302,40.8127362898543,-11.9176190323383));
#40772=CARTESIAN_POINT('Ctrl Pts',(18.7979917002302,27.2694232481814,14.1614724492006));
#40773=CARTESIAN_POINT('Ctrl Pts',(17.4917404060759,27.1042817018803,14.0757116526895));
#40774=CARTESIAN_POINT('Ctrl Pts',(17.4917404060759,26.7902192241678,14.6804723978617));
#40775=CARTESIAN_POINT('Ctrl Pts',(17.4917404060759,26.4494954361781,15.2706233100072));
#40776=CARTESIAN_POINT('Ctrl Pts',(17.4917404060759,11.1788721261709,41.7201187461852));
#40777=CARTESIAN_POINT('Ctrl Pts',(17.4917404060759,-15.2706233100072,26.4494954361781));
#40778=CARTESIAN_POINT('Ctrl Pts',(17.4917404060759,-41.7201187461852,11.1788721261709));
#40779=CARTESIAN_POINT('Ctrl Pts',(17.4917404060759,-26.4494954361781,-15.2706233100072));
#40780=CARTESIAN_POINT('Ctrl Pts',(17.4917404060759,-11.1788721261709,-41.7201187461852));
#40781=CARTESIAN_POINT('Ctrl Pts',(17.4917404060759,15.2706233100072,-26.4494954361781));
#40782=CARTESIAN_POINT('Ctrl Pts',(17.4917404060759,40.5655774732432,-11.8454468408945));
#40783=CARTESIAN_POINT('Ctrl Pts',(17.4917404060759,27.1042817018803,14.0757116526895));
#40784=CARTESIAN_POINT('Ctrl Pts',(16.1647270995715,26.9797204766935,14.011024902894));
#40785=CARTESIAN_POINT('Ctrl Pts',(16.1647270995715,26.6671013136366,14.6130063919992));
#40786=CARTESIAN_POINT('Ctrl Pts',(16.1647270995715,26.3279433657953,15.2004451894511));
#40787=CARTESIAN_POINT('Ctrl Pts',(16.1647270995715,11.1274981763442,41.5283885552464));
#40788=CARTESIAN_POINT('Ctrl Pts',(16.1647270995715,-15.2004451894511,26.3279433657953));
#40789=CARTESIAN_POINT('Ctrl Pts',(16.1647270995715,-41.5283885552464,11.1274981763442));
#40790=CARTESIAN_POINT('Ctrl Pts',(16.1647270995715,-26.3279433657953,-15.2004451894511));
#40791=CARTESIAN_POINT('Ctrl Pts',(16.1647270995715,-11.1274981763442,-41.5283885552464));
#40792=CARTESIAN_POINT('Ctrl Pts',(16.1647270995715,15.2004451894511,-26.3279433657953));
#40793=CARTESIAN_POINT('Ctrl Pts',(16.1647270995715,40.3791531257526,-11.7910095609247));
#40794=CARTESIAN_POINT('Ctrl Pts',(16.1647270995715,26.9797204766935,14.011024902894));
#40795=CARTESIAN_POINT('Ctrl Pts',(14.8263876417415,26.8868282012067,13.9627843740029));
#40796=CARTESIAN_POINT('Ctrl Pts',(14.8263876417415,26.5752853986496,14.5626932163446));
#40797=CARTESIAN_POINT('Ctrl Pts',(14.8263876417415,26.2372951854241,15.1481094381123));
#40798=CARTESIAN_POINT('Ctrl Pts',(14.8263876417415,11.0891857473118,41.3854046235364));
#40799=CARTESIAN_POINT('Ctrl Pts',(14.8263876417415,-15.1481094381123,26.2372951854241));
#40800=CARTESIAN_POINT('Ctrl Pts',(14.8263876417415,-41.3854046235364,11.0891857473118));
#40801=CARTESIAN_POINT('Ctrl Pts',(14.8263876417415,-26.2372951854241,-15.1481094381123));
#40802=CARTESIAN_POINT('Ctrl Pts',(14.8263876417415,-11.0891857473118,-41.3854046235364));
#40803=CARTESIAN_POINT('Ctrl Pts',(14.8263876417415,15.1481094381123,-26.2372951854241));
#40804=CARTESIAN_POINT('Ctrl Pts',(14.8263876417415,40.2401260583921,-11.750412635195));
#40805=CARTESIAN_POINT('Ctrl Pts',(14.8263876417415,26.8868282012067,13.9627843740029));
#40806=CARTESIAN_POINT('Ctrl Pts',(13.4853470903953,26.8165326442879,13.926278703034));
#40807=CARTESIAN_POINT('Ctrl Pts',(13.4853470903953,26.505804369746,14.5246190849439));
#40808=CARTESIAN_POINT('Ctrl Pts',(13.4853470903953,26.1686978312363,15.1085047372063));
#40809=CARTESIAN_POINT('Ctrl Pts',(13.4853470903953,11.0601930940301,41.2772025684426));
#40810=CARTESIAN_POINT('Ctrl Pts',(13.4853470903953,-15.1085047372063,26.1686978312363));
#40811=CARTESIAN_POINT('Ctrl Pts',(13.4853470903953,-41.2772025684426,11.0601930940301));
#40812=CARTESIAN_POINT('Ctrl Pts',(13.4853470903953,-26.1686978312363,-15.1085047372063));
#40813=CARTESIAN_POINT('Ctrl Pts',(13.4853470903953,-11.0601930940301,-41.2772025684426));
#40814=CARTESIAN_POINT('Ctrl Pts',(13.4853470903953,15.1085047372063,-26.1686978312363));
#40815=CARTESIAN_POINT('Ctrl Pts',(13.4853470903953,40.1349183317465,-11.7196912055776));
#40816=CARTESIAN_POINT('Ctrl Pts',(13.4853470903953,26.8165326442879,13.926278703034));
#40817=CARTESIAN_POINT('Ctrl Pts',(12.1482076787549,26.7614591013549,13.8976780812377));
#40818=CARTESIAN_POINT('Ctrl Pts',(12.1482076787549,26.4513689744511,14.4947896419145));
#40819=CARTESIAN_POINT('Ctrl Pts',(12.1482076787549,26.1149547570431,15.0774761588537));
#40820=CARTESIAN_POINT('Ctrl Pts',(12.1482076787549,11.0374785981894,41.1924309158968));
#40821=CARTESIAN_POINT('Ctrl Pts',(12.1482076787549,-15.0774761588537,26.1149547570431));
#40822=CARTESIAN_POINT('Ctrl Pts',(12.1482076787549,-41.1924309158968,11.0374785981894));
#40823=CARTESIAN_POINT('Ctrl Pts',(12.1482076787549,-26.1149547570431,-15.0774761588537));
#40824=CARTESIAN_POINT('Ctrl Pts',(12.1482076787549,-11.0374785981894,-41.1924309158968));
#40825=CARTESIAN_POINT('Ctrl Pts',(12.1482076787549,15.0774761588537,-26.1149547570431));
#40826=CARTESIAN_POINT('Ctrl Pts',(12.1482076787549,40.0524926066472,-11.6956222878942));
#40827=CARTESIAN_POINT('Ctrl Pts',(12.1482076787549,26.7614591013549,13.8976780812377));
#40828=CARTESIAN_POINT('Ctrl Pts',(10.8190675759626,26.716817747915,13.8744950717886));
#40829=CARTESIAN_POINT('Ctrl Pts',(10.8190675759626,26.4072448888814,14.4706105780977));
#40830=CARTESIAN_POINT('Ctrl Pts',(10.8190675759626,26.0713918511132,15.0523251033884));
#40831=CARTESIAN_POINT('Ctrl Pts',(10.8190675759626,11.0190667477248,41.1237169545017));
#40832=CARTESIAN_POINT('Ctrl Pts',(10.8190675759626,-15.0523251033884,26.0713918511132));
#40833=CARTESIAN_POINT('Ctrl Pts',(10.8190675759626,-41.1237169545017,11.0190667477248));
#40834=CARTESIAN_POINT('Ctrl Pts',(10.8190675759626,-26.0713918511132,-15.0523251033884));
#40835=CARTESIAN_POINT('Ctrl Pts',(10.8190675759626,-11.0190667477248,-41.1237169545017));
#40836=CARTESIAN_POINT('Ctrl Pts',(10.8190675759626,15.0523251033884,-26.0713918511132));
#40837=CARTESIAN_POINT('Ctrl Pts',(10.8190675759626,39.9856802003493,-11.6761125740823));
#40838=CARTESIAN_POINT('Ctrl Pts',(10.8190675759626,26.716817747915,13.8744950717886));
#40839=CARTESIAN_POINT('Ctrl Pts',(9.50027713254189,26.6796403391198,13.8551882149624));
#40840=CARTESIAN_POINT('Ctrl Pts',(9.50027713254189,26.3704982618073,14.4504742051937));
#40841=CARTESIAN_POINT('Ctrl Pts',(9.50027713254189,26.0351125755702,15.0313792538877));
#40842=CARTESIAN_POINT('Ctrl Pts',(9.50027713254189,11.0037333216825,41.0664918294579));
#40843=CARTESIAN_POINT('Ctrl Pts',(9.50027713254189,-15.0313792538877,26.0351125755702));
#40844=CARTESIAN_POINT('Ctrl Pts',(9.5002771325419,-41.0664918294579,11.0037333216825));
#40845=CARTESIAN_POINT('Ctrl Pts',(9.5002771325419,-26.0351125755702,-15.0313792538877));
#40846=CARTESIAN_POINT('Ctrl Pts',(9.5002771325419,-11.0037333216825,-41.0664918294579));
#40847=CARTESIAN_POINT('Ctrl Pts',(9.50027713254189,15.0313792538877,-26.0351125755702));
#40848=CARTESIAN_POINT('Ctrl Pts',(9.50027713254189,39.9300386942093,-11.6598648452397));
#40849=CARTESIAN_POINT('Ctrl Pts',(9.50027713254189,26.6796403391198,13.8551882149624));
#40850=CARTESIAN_POINT('Ctrl Pts',(8.45435372222587,26.6546635289318,13.8422173352292));
#40851=CARTESIAN_POINT('Ctrl Pts',(8.45435372222587,26.3458108626791,14.4369460336456));
#40852=CARTESIAN_POINT('Ctrl Pts',(8.45435372222587,26.0107391561104,15.0173072536015));
#40853=CARTESIAN_POINT('Ctrl Pts',(8.45435372222587,10.9934319025089,41.0280464097118));
#40854=CARTESIAN_POINT('Ctrl Pts',(8.45435372222587,-15.0173072536015,26.0107391561104));
#40855=CARTESIAN_POINT('Ctrl Pts',(8.45435372222587,-41.0280464097118,10.9934319025089));
#40856=CARTESIAN_POINT('Ctrl Pts',(8.45435372222587,-26.0107391561104,-15.0173072536015));
#40857=CARTESIAN_POINT('Ctrl Pts',(8.45435372222587,-10.9934319025089,-41.0280464097118));
#40858=CARTESIAN_POINT('Ctrl Pts',(8.45435372222587,15.0173072536015,-26.0107391561104));
#40859=CARTESIAN_POINT('Ctrl Pts',(8.45435372222587,39.8926571933874,-11.6489491721888));
#40860=CARTESIAN_POINT('Ctrl Pts',(8.45435372222587,26.6546635289318,13.8422173352292));
#40861=CARTESIAN_POINT('Ctrl Pts',(7.67514864245731,26.6383620035993,13.8337516775666));
#40862=CARTESIAN_POINT('Ctrl Pts',(7.67514864245731,26.3296982262274,14.4281166503283));
#40863=CARTESIAN_POINT('Ctrl Pts',(7.67514864245731,25.9948314436454,15.0081229315276));
#40864=CARTESIAN_POINT('Ctrl Pts',(7.67514864245731,10.9867085121178,41.0029543751729));
#40865=CARTESIAN_POINT('Ctrl Pts',(7.67514864245731,-15.0081229315276,25.9948314436454));
#40866=CARTESIAN_POINT('Ctrl Pts',(7.67514864245731,-41.0029543751729,10.9867085121178));
#40867=CARTESIAN_POINT('Ctrl Pts',(7.67514864245731,-25.9948314436454,-15.0081229315276));
#40868=CARTESIAN_POINT('Ctrl Pts',(7.67514864245731,-10.9867085121178,-41.0029543751729));
#40869=CARTESIAN_POINT('Ctrl Pts',(7.67514864245731,15.0081229315276,-25.9948314436454));
#40870=CARTESIAN_POINT('Ctrl Pts',(7.67514864245731,39.8682595430058,-11.6418248789176));
#40871=CARTESIAN_POINT('Ctrl Pts',(7.67514864245731,26.6383620035993,13.8337516775666));
#40872=CARTESIAN_POINT('Ctrl Pts',(7.15799654185577,26.6285708447822,13.8286669632852));
#40873=CARTESIAN_POINT('Ctrl Pts',(7.15799654185577,26.3200205194336,14.4228134720947));
#40874=CARTESIAN_POINT('Ctrl Pts',(7.15799654185577,25.9852768200144,15.0026065670023));
#40875=CARTESIAN_POINT('Ctrl Pts',(7.15799654185577,10.9826702530122,40.9878833870167));
#40876=CARTESIAN_POINT('Ctrl Pts',(7.15799654185577,-15.0026065670023,25.9852768200144));
#40877=CARTESIAN_POINT('Ctrl Pts',(7.15799654185577,-40.9878833870167,10.9826702530122));
#40878=CARTESIAN_POINT('Ctrl Pts',(7.15799654185577,-25.9852768200144,-15.0026065670023));
#40879=CARTESIAN_POINT('Ctrl Pts',(7.15799654185577,-10.9826702530122,-40.9878833870167));
#40880=CARTESIAN_POINT('Ctrl Pts',(7.15799654185577,15.0026065670023,-25.9852768200144));
#40881=CARTESIAN_POINT('Ctrl Pts',(7.15799654185577,39.8536056216838,-11.6375458261629));
#40882=CARTESIAN_POINT('Ctrl Pts',(7.15799654185577,26.6285708447822,13.8286669632852));
#40883=CARTESIAN_POINT('Ctrl Pts',(6.9,26.6239443717909,13.8262643576559));
#40884=CARTESIAN_POINT('Ctrl Pts',(6.9,26.3154476542665,14.4203076388911));
#40885=CARTESIAN_POINT('Ctrl Pts',(6.9,25.9807621135332,15.));
#40886=CARTESIAN_POINT('Ctrl Pts',(6.9,10.9807621135332,40.9807621135332));
#40887=CARTESIAN_POINT('Ctrl Pts',(6.9,-15.,25.9807621135332));
#40888=CARTESIAN_POINT('Ctrl Pts',(6.9,-40.9807621135332,10.9807621135332));
#40889=CARTESIAN_POINT('Ctrl Pts',(6.9,-25.9807621135332,-15.));
#40890=CARTESIAN_POINT('Ctrl Pts',(6.9,-10.9807621135332,-40.9807621135332));
#40891=CARTESIAN_POINT('Ctrl Pts',(6.9,15.,-25.9807621135332));
#40892=CARTESIAN_POINT('Ctrl Pts',(6.9,39.846681418688,-11.6355239079847));
#40893=CARTESIAN_POINT('Ctrl Pts',(6.9,26.6239443717909,13.8262643576559));
#40894=CARTESIAN_POINT('Ctrl Pts',(6.9,6.90555748864272,29.194404870986));
#40895=CARTESIAN_POINT('Ctrl Pts',(7.85773098116326,8.83308608050287,28.7583591297181));
#40896=CARTESIAN_POINT('Ctrl Pts',(8.88781981167334,10.6725495024415,28.148927360677));
#40897=CARTESIAN_POINT('Ctrl Pts',(10.5914578196776,13.4378975079049,26.9549567714738));
#40898=CARTESIAN_POINT('Ctrl Pts',(11.2365058953701,14.4268759573926,26.4627511078989));
#40899=CARTESIAN_POINT('Ctrl Pts',(12.0558885382926,15.5639851987506,25.8276163596339));
#40900=CARTESIAN_POINT('Ctrl Pts',(12.1875764958397,15.7427052651201,25.7255677072203));
#40901=CARTESIAN_POINT('Ctrl Pts',(13.194901830313,17.0880993664927,24.9407551262718));
#40902=CARTESIAN_POINT('Ctrl Pts',(14.2258982134098,18.4224696507577,24.0748117650462));
#40903=CARTESIAN_POINT('Ctrl Pts',(18.2616480823244,22.4465505568645,20.9914735836847));
#40904=CARTESIAN_POINT('Ctrl Pts',(21.0496416709525,24.4970863377161,19.1084188222497));
#40905=CARTESIAN_POINT('Ctrl Pts',(25.8000196361138,27.440416330328,18.0798601480504));
#40906=CARTESIAN_POINT('Ctrl Pts',(26.8976561124457,27.9949084025612,18.1725012311874));
#40907=CARTESIAN_POINT('Ctrl Pts',(28.0045908801237,28.5110480063609,18.293020318403));
#40908=CARTESIAN_POINT('Ctrl Pts',(28.5235971652406,28.7375730360626,18.3760345677216));
#40909=CARTESIAN_POINT('Ctrl Pts',(29.0834839543824,28.9821227669884,18.4629109750536));
#40910=CARTESIAN_POINT('Ctrl Pts',(29.1146288039499,28.995750541561,18.4676985487665));
#40911=CARTESIAN_POINT('Ctrl Pts',(29.5949306848436,29.2050975774362,18.5426905181125));
#40912=CARTESIAN_POINT('Ctrl Pts',(30.0492939924726,29.3870260594868,18.6372599535756));
#40913=CARTESIAN_POINT('Ctrl Pts',(30.5,29.559989655385,18.7405179110273));
#40914=CARTESIAN_POINT('Ctrl Pts',(6.45331003273164,1.59669678622779,10.9133179225515));
#40915=CARTESIAN_POINT('Ctrl Pts',(7.20830533428676,2.1627262104287,10.8283039351861));
#40916=CARTESIAN_POINT('Ctrl Pts',(7.9992896214032,2.70879554626307,10.7080816105349));
#40917=CARTESIAN_POINT('Ctrl Pts',(9.76164489174098,3.82718122480732,10.3736775708918));
#40918=CARTESIAN_POINT('Ctrl Pts',(10.7316587814816,4.40082635509404,10.1362456656108));
#40919=CARTESIAN_POINT('Ctrl Pts',(12.6606926111663,5.38563263712134,9.65961205419967));
#40920=CARTESIAN_POINT('Ctrl Pts',(13.6374431259541,5.83915384029437,9.38360450626091));
#40921=CARTESIAN_POINT('Ctrl Pts',(14.8679539417017,6.32358226998234,9.06165302613707));
#40922=CARTESIAN_POINT('Ctrl Pts',(15.8146186835335,6.68453209751777,8.8086769516328));
#40923=CARTESIAN_POINT('Ctrl Pts',(16.7768279789012,7.0051694125711,8.55011854625631));
#40924=CARTESIAN_POINT('Ctrl Pts',(18.4426549461009,7.48808598435166,8.14533972931254));
#40925=CARTESIAN_POINT('Ctrl Pts',(19.4151948753427,7.72973898022671,7.90738588441824));
#40926=CARTESIAN_POINT('Ctrl Pts',(20.6328868119184,7.97443640583059,7.66437297695771));
#40927=CARTESIAN_POINT('Ctrl Pts',(21.1054260060187,8.06465516157005,7.57098863237663));
#40928=CARTESIAN_POINT('Ctrl Pts',(22.0544239964407,8.2283193842107,7.3938759247957));
#40929=CARTESIAN_POINT('Ctrl Pts',(22.7836594350112,8.33397294082319,7.27389266543021));
#40930=CARTESIAN_POINT('Ctrl Pts',(23.5025637456204,8.42426711082601,7.17270583388455));
#40931=CARTESIAN_POINT('Ctrl Pts',(23.9756232708729,8.4795264691222,7.10861034193437));
#40932=CARTESIAN_POINT('Ctrl Pts',(24.5702383273712,8.53935462310087,7.03666681503306));
#40933=CARTESIAN_POINT('Ctrl Pts',(25.0506812637281,8.58189400875846,6.98463603831062));
#40934=CARTESIAN_POINT('Ctrl Pts',(25.4117237717367,8.61093616318062,6.94891133994702));
#40935=CARTESIAN_POINT('Ctrl Pts',(25.713233130151,8.63276690479095,6.92207219011214));
#40936=CARTESIAN_POINT('Ctrl Pts',(25.924350018954,8.64675417662542,6.90499555217216));
#40937=CARTESIAN_POINT('Ctrl Pts',(26.0449825351307,8.65437719289231,6.89574165973189));
#40938=CARTESIAN_POINT('Ctrl Pts',(26.1053107047432,8.65806460962808,6.89128602190966));
#40939=CARTESIAN_POINT('Ctrl Pts',(26.5982868813559,8.68771831234638,6.85557010312596));
#40940=CARTESIAN_POINT('Ctrl Pts',(27.5414448539116,8.7222238682218,6.81230249083085));
#40941=CARTESIAN_POINT('Ctrl Pts',(28.5384718269746,8.73742874004845,6.79157348079204));
#40942=CARTESIAN_POINT('Ctrl Pts',(29.123571801101,8.74727658763319,6.77903979219489));
#40943=CARTESIAN_POINT('Ctrl Pts',(29.2812925824008,8.74962231400052,6.77610142826287));
#40944=CARTESIAN_POINT('Ctrl Pts',(29.6033746665997,8.75316560056402,6.77163194910164));
#40945=CARTESIAN_POINT('Ctrl Pts',(30.1682156581426,8.75644680260445,6.76749797708623));
#40946=CARTESIAN_POINT('Ctrl Pts',(31.31511200853,8.75407681716339,6.7704817474239));
#40947=CARTESIAN_POINT('Ctrl Pts',(32.3203490755539,8.74562733267077,6.78127046660755));
#40948=CARTESIAN_POINT('Ctrl Pts',(33.1676615322707,8.74562186943987,6.78128357449778));
#40949=CARTESIAN_POINT('Ctrl Pts',(33.4948723279894,8.74562133595168,6.78128505761794));
#40950=CARTESIAN_POINT('Ctrl Pts',(34.1541357431676,8.74562028433967,6.7812877053352));
#40951=CARTESIAN_POINT('Ctrl Pts',(34.9760826079903,8.74561702798978,6.78129612595839));
#40952=CARTESIAN_POINT('Ctrl Pts',(35.9636845487691,8.74561567977429,6.78129958330352));
#40953=CARTESIAN_POINT('Ctrl Pts',(37.9383132355672,8.74561382885199,6.78130435924949));
#40954=CARTESIAN_POINT('Ctrl Pts',(39.5833333333333,8.74560464293355,6.7813280023926));
#40955=CARTESIAN_POINT('Ctrl Pts',(40.9,8.74560464293355,6.7813280023926));
#40956=CARTESIAN_POINT('Ctrl Pts',(6.63336813585096,2.58998912169033,14.1980521881427));
#40957=CARTESIAN_POINT('Ctrl Pts',(7.389696336477,3.32655463912721,14.0595388287459));
#40958=CARTESIAN_POINT('Ctrl Pts',(8.18035160561763,4.03465273479121,13.8764440634215));
#40959=CARTESIAN_POINT('Ctrl Pts',(9.9416314386187,5.47986851886093,13.3869575789582));
#40960=CARTESIAN_POINT('Ctrl Pts',(10.9109664605568,6.21859686207518,13.0495988183286));
#40961=CARTESIAN_POINT('Ctrl Pts',(12.8334013836927,7.47915893423736,12.3824387994051));
#40962=CARTESIAN_POINT('Ctrl Pts',(13.8089179831182,8.05904353786121,12.0008911509523));
#40963=CARTESIAN_POINT('Ctrl Pts',(15.0306778911272,8.67329495695321,11.5604290689694));
#40964=CARTESIAN_POINT('Ctrl Pts',(15.9745670647921,9.13243737556314,11.2141745075895));
#40965=CARTESIAN_POINT('Ctrl Pts',(16.9295440841729,9.53704617981304,10.8635736365946));
#40966=CARTESIAN_POINT('Ctrl Pts',(18.5792362231986,10.1451076803253,10.3171018918725));
#40967=CARTESIAN_POINT('Ctrl Pts',(19.5469773926756,10.4493242965117,9.99640408637918));
#40968=CARTESIAN_POINT('Ctrl Pts',(20.7474295734276,10.754900018616,9.67172058444861));
#40969=CARTESIAN_POINT('Ctrl Pts',(21.2167794172893,10.8681544802446,9.54637190554475));
#40970=CARTESIAN_POINT('Ctrl Pts',(22.1549843938463,11.0724642143302,9.30976886072816));
#40971=CARTESIAN_POINT('Ctrl Pts',(22.8744776078266,11.2039970972494,9.14996578827686));
#40972=CARTESIAN_POINT('Ctrl Pts',(23.5816077902761,11.3162019466948,9.01558422395416));
#40973=CARTESIAN_POINT('Ctrl Pts',(24.0500749276264,11.3851612528794,8.93008359351429));
#40974=CARTESIAN_POINT('Ctrl Pts',(24.6365533946125,11.4594652258083,8.83449183240023));
#40975=CARTESIAN_POINT('Ctrl Pts',(25.1102835291687,11.512269915973,8.76539275960626));
#40976=CARTESIAN_POINT('Ctrl Pts',(25.4658322439329,11.5482688417072,8.71801358900137));
#40977=CARTESIAN_POINT('Ctrl Pts',(25.7624874136684,11.5753180370233,8.68244638509936));
#40978=CARTESIAN_POINT('Ctrl Pts',(25.9700349923411,11.5926401638759,8.65983585467431));
#40979=CARTESIAN_POINT('Ctrl Pts',(26.0885791323128,11.6020803597252,8.64758737376051));
#40980=CARTESIAN_POINT('Ctrl Pts',(26.1478525996403,11.606646750038,8.64169115913857));
#40981=CARTESIAN_POINT('Ctrl Pts',(26.6319130667262,11.6433645250355,8.59444428954213));
#40982=CARTESIAN_POINT('Ctrl Pts',(27.5577774489366,11.6860824768892,8.53717709311578));
#40983=CARTESIAN_POINT('Ctrl Pts',(28.5508423746856,11.7050908260001,8.5094282805872));
#40984=CARTESIAN_POINT('Ctrl Pts',(29.1362159539421,11.7174369518245,8.49263545125888));
#40985=CARTESIAN_POINT('Ctrl Pts',(29.291281950884,11.7203386713975,8.48875007883411));
#40986=CARTESIAN_POINT('Ctrl Pts',(29.6100529981868,11.724747509447,8.48280581727725));
#40987=CARTESIAN_POINT('Ctrl Pts',(30.1693026775045,11.7288279027909,8.4773119045209));
#40988=CARTESIAN_POINT('Ctrl Pts',(31.3098786008462,11.725887289448,8.48127083805327));
#40989=CARTESIAN_POINT('Ctrl Pts',(32.3162827048882,11.7152777874898,8.49575357359986));
#40990=CARTESIAN_POINT('Ctrl Pts',(33.1686195735696,11.7152690782769,8.495775239756));
#40991=CARTESIAN_POINT('Ctrl Pts',(33.4952188807557,11.7152682401723,8.49577770055111));
#40992=CARTESIAN_POINT('Ctrl Pts',(34.1547734244041,11.7152665713231,8.49578208271195));
#40993=CARTESIAN_POINT('Ctrl Pts',(34.9764178792931,11.7152614171757,8.49579602915744));
#40994=CARTESIAN_POINT('Ctrl Pts',(35.9640520550921,11.7152592814565,8.49580175406155));
#40995=CARTESIAN_POINT('Ctrl Pts',(37.9385651163987,11.7152563511876,8.49580966365999));
#40996=CARTESIAN_POINT('Ctrl Pts',(39.5833333333333,11.7152418049849,8.49584881729847));
#40997=CARTESIAN_POINT('Ctrl Pts',(40.9,11.7152418049849,8.49584881729847));
#40998=CARTESIAN_POINT('Ctrl Pts',(6.84648239176542,4.8711720049463,21.8719108775553));
#40999=CARTESIAN_POINT('Ctrl Pts',(7.61278097593421,6.01809391809558,21.6080942034255));
#41000=CARTESIAN_POINT('Ctrl Pts',(8.41274152921386,7.11297694015339,21.2759544371052));
#41001=CARTESIAN_POINT('Ctrl Pts',(10.1879716557546,9.3352659896486,20.4198986989574));
#41002=CARTESIAN_POINT('Ctrl Pts',(11.1642573475929,10.4645258845954,19.8462357742843));
#41003=CARTESIAN_POINT('Ctrl Pts',(13.1034321172788,12.3837514736036,18.7228640453274));
#41004=CARTESIAN_POINT('Ctrl Pts',(14.0822646095709,13.259092905625,18.0925354910949));
#41005=CARTESIAN_POINT('Ctrl Pts',(15.3084001581866,14.1807147676624,17.369341405527));
#41006=CARTESIAN_POINT('Ctrl Pts',(16.2531227144981,14.8695159890908,16.8032299545452));
#41007=CARTESIAN_POINT('Ctrl Pts',(17.2084375604977,15.4708786153412,16.2348330754283));
#41008=CARTESIAN_POINT('Ctrl Pts',(18.8473961588578,16.3684102669437,15.3570672461537));
#41009=CARTESIAN_POINT('Ctrl Pts',(19.8110405035781,16.8164458459157,14.8437940564496));
#41010=CARTESIAN_POINT('Ctrl Pts',(20.9872655006159,17.2594998647323,14.3329359049566));
#41011=CARTESIAN_POINT('Ctrl Pts',(21.4517346237734,17.4254488483261,14.1338378277511));
#41012=CARTESIAN_POINT('Ctrl Pts',(22.3727984841463,17.7217491293399,13.7614448137587));
#41013=CARTESIAN_POINT('Ctrl Pts',(23.0743543377559,17.9111527143534,13.5118529399621));
#41014=CARTESIAN_POINT('Ctrl Pts',(23.7582742987063,18.0719640430561,13.3034745440379));
#41015=CARTESIAN_POINT('Ctrl Pts',(24.2174386855893,18.1719103336476,13.1693266480666));
#41016=CARTESIAN_POINT('Ctrl Pts',(24.7870213943586,18.2785218143407,13.020703786838));
#41017=CARTESIAN_POINT('Ctrl Pts',(25.2463470121633,18.3542161979471,12.9133861579982));
#41018=CARTESIAN_POINT('Ctrl Pts',(25.5899787396418,18.4056632423986,12.8400372670538));
#41019=CARTESIAN_POINT('Ctrl Pts',(25.8759048428223,18.4442660174719,12.7850917865304));
#41020=CARTESIAN_POINT('Ctrl Pts',(26.0755068065028,18.468956785964,12.7502361709813));
#41021=CARTESIAN_POINT('Ctrl Pts',(26.1893780149128,18.4824083304411,12.7313725692327));
#41022=CARTESIAN_POINT('Ctrl Pts',(26.2462863876019,18.4889145361418,12.7222969574594));
#41023=CARTESIAN_POINT('Ctrl Pts',(26.7102722067271,18.5411896593428,12.6496548741737));
#41024=CARTESIAN_POINT('Ctrl Pts',(27.5960905386885,18.602045864812,12.5614420302555));
#41025=CARTESIAN_POINT('Ctrl Pts',(28.5798438027284,18.6298999603239,12.5173520665107));
#41026=CARTESIAN_POINT('Ctrl Pts',(29.1658297917575,18.6480680632813,12.4906249890438));
#41027=CARTESIAN_POINT('Ctrl Pts',(29.3147155528136,18.652196249303,12.4846522276655));
#41028=CARTESIAN_POINT('Ctrl Pts',(29.6257654938389,18.6585637397072,12.4753713397181));
#41029=CARTESIAN_POINT('Ctrl Pts',(30.1719616098275,18.6644443298452,12.4668129248998));
#41030=CARTESIAN_POINT('Ctrl Pts',(31.2977738410332,18.6602190141085,12.4729611884879));
#41031=CARTESIAN_POINT('Ctrl Pts',(32.3068669150107,18.6445149503825,12.4961463862896));
#41032=CARTESIAN_POINT('Ctrl Pts',(33.1709127040732,18.6444874715365,12.4962026881972));
#41033=CARTESIAN_POINT('Ctrl Pts',(33.4960830255433,18.644484418038,12.4962093123004));
#41034=CARTESIAN_POINT('Ctrl Pts',(34.1563135822161,18.6444789016083,12.4962208405723));
#41035=CARTESIAN_POINT('Ctrl Pts',(34.9772414248898,18.6444614154563,12.4962577684094));
#41036=CARTESIAN_POINT('Ctrl Pts',(35.9649463721129,18.6444542286038,12.496272896639));
#41037=CARTESIAN_POINT('Ctrl Pts',(37.9391834323222,18.6444443083029,12.4962938290756));
#41038=CARTESIAN_POINT('Ctrl Pts',(39.5833333333333,18.6443951831047,12.4963973854122));
#41039=CARTESIAN_POINT('Ctrl Pts',(40.9,18.6443951831047,12.4963973854122));
#41040=CARTESIAN_POINT('Ctrl Pts',(6.90857970435318,7.02038826853569,29.5800408844791));
#41041=CARTESIAN_POINT('Ctrl Pts',(7.67983757144493,8.58577901088988,29.1962153577801));
#41042=CARTESIAN_POINT('Ctrl Pts',(8.48446296596919,10.0765485557757,28.7191114013952));
#41043=CARTESIAN_POINT('Ctrl Pts',(10.2687526859613,13.0935628879537,27.5023711977385));
#41044=CARTESIAN_POINT('Ctrl Pts',(11.2489627292759,14.6224501564806,26.6949552438923));
#41045=CARTESIAN_POINT('Ctrl Pts',(13.2065810728343,17.2294066625499,25.1069038454383));
#41046=CARTESIAN_POINT('Ctrl Pts',(14.1884325798659,18.406995285395,24.2271697832518));
#41047=CARTESIAN_POINT('Ctrl Pts',(15.4296983589675,19.6550892131211,23.2080338536349));
#41048=CARTESIAN_POINT('Ctrl Pts',(16.3788042670986,20.5796860932724,22.4189011948389));
#41049=CARTESIAN_POINT('Ctrl Pts',(17.3450159165718,21.3903231452906,21.6217224592711));
#41050=CARTESIAN_POINT('Ctrl Pts',(18.9999962645462,22.5937460627634,20.3951481814249));
#41051=CARTESIAN_POINT('Ctrl Pts',(19.9686658165164,23.1898054127388,19.6835411202358));
#41052=CARTESIAN_POINT('Ctrl Pts',(21.148943716884,23.7756910485748,18.9783964629486));
#41053=CARTESIAN_POINT('Ctrl Pts',(21.6136662410167,23.9949385633152,18.7043064424585));
#41054=CARTESIAN_POINT('Ctrl Pts',(22.5341605437881,24.3846521737582,18.1932305660766));
#41055=CARTESIAN_POINT('Ctrl Pts',(23.2310352415762,24.6315178872709,17.8537326154787));
#41056=CARTESIAN_POINT('Ctrl Pts',(23.9047680627609,24.8394315921367,17.5731511638351));
#41057=CARTESIAN_POINT('Ctrl Pts',(24.3593217251592,24.96958718913,17.391254980069));
#41058=CARTESIAN_POINT('Ctrl Pts',(24.9191284505008,25.1069751863358,17.1917285847407));
#41059=CARTESIAN_POINT('Ctrl Pts',(25.3687829483026,25.2041659752934,17.0482631873592));
#41060=CARTESIAN_POINT('Ctrl Pts',(25.7038809466239,25.269917189492,16.9507036504243));
#41061=CARTESIAN_POINT('Ctrl Pts',(25.9815275275379,25.3190677310922,16.8779731233104));
#41062=CARTESIAN_POINT('Ctrl Pts',(26.1747255747307,25.3504124116977,16.832023377701));
#41063=CARTESIAN_POINT('Ctrl Pts',(26.284743001994,25.3674660195526,16.8072090098453));
#41064=CARTESIAN_POINT('Ctrl Pts',(26.3396756125252,25.3757090167853,16.7952849898384));
#41065=CARTESIAN_POINT('Ctrl Pts',(26.7867185605548,25.4418392909473,16.7000344271697));
#41066=CARTESIAN_POINT('Ctrl Pts',(27.6343089133549,25.5185659559041,16.5847364280862));
#41067=CARTESIAN_POINT('Ctrl Pts',(28.608620419133,25.5552242576153,16.5243820587323));
#41068=CARTESIAN_POINT('Ctrl Pts',(29.1952293795947,25.5792110357045,16.4877244301024));
#41069=CARTESIAN_POINT('Ctrl Pts',(29.3380035933317,25.5844033272728,16.4799452423708));
#41070=CARTESIAN_POINT('Ctrl Pts',(29.6413717635319,25.5925899885789,16.4675695714432));
#41071=CARTESIAN_POINT('Ctrl Pts',(30.1745368065168,25.6001268754993,16.4561967872261));
#41072=CARTESIAN_POINT('Ctrl Pts',(31.2855894033321,25.5947346655062,16.464330041984));
#41073=CARTESIAN_POINT('Ctrl Pts',(32.2974015084454,25.57383077045,16.4964013295029));
#41074=CARTESIAN_POINT('Ctrl Pts',(33.1731651112182,25.5737672879573,16.4965224425527));
#41075=CARTESIAN_POINT('Ctrl Pts',(33.4969081472871,25.57375987162,16.4965369996128));
#41076=CARTESIAN_POINT('Ctrl Pts',(34.1578169391039,25.5737469053194,16.4965619872358));
#41077=CARTESIAN_POINT('Ctrl Pts',(34.9780359591179,25.5737054251286,16.496642344611));
#41078=CARTESIAN_POINT('Ctrl Pts',(35.9658147840134,25.5736884251095,16.4966752246752));
#41079=CARTESIAN_POINT('Ctrl Pts',(37.9397802282711,25.5736649097448,16.4967207607426));
#41080=CARTESIAN_POINT('Ctrl Pts',(39.5833333333333,25.5735485612246,16.4969459535258));
#41081=CARTESIAN_POINT('Ctrl Pts',(40.9,25.5735485612246,16.4969459535258));
#41082=CARTESIAN_POINT('Ctrl Pts',(6.93528330520032,8.231730283379,33.9890447223856));
#41083=CARTESIAN_POINT('Ctrl Pts',(7.70864561497005,10.0357116563145,33.5376786188307));
#41084=CARTESIAN_POINT('Ctrl Pts',(8.51532719250786,11.7528338486872,32.9786927413523));
#41085=CARTESIAN_POINT('Ctrl Pts',(10.3033707684643,15.2242195800702,31.5578840442132));
#41086=CARTESIAN_POINT('Ctrl Pts',(11.285359425586,16.9818886494149,30.6179424293771));
#41087=CARTESIAN_POINT('Ctrl Pts',(13.2503075123955,19.9828238609275,28.7660858779662));
#41088=CARTESIAN_POINT('Ctrl Pts',(14.2335802328307,21.333808720003,27.7445903826109));
#41089=CARTESIAN_POINT('Ctrl Pts',(15.4809874764708,22.7701484639683,26.5562215055806));
#41090=CARTESIAN_POINT('Ctrl Pts',(16.4318967140332,23.8303538982284,25.6398645222147));
#41091=CARTESIAN_POINT('Ctrl Pts',(17.4027860882061,24.7620955812504,24.7114068344531));
#41092=CARTESIAN_POINT('Ctrl Pts',(19.0657008739463,26.1438767914272,23.2827894621994));
#41093=CARTESIAN_POINT('Ctrl Pts',(20.0370987955263,26.8257745442827,22.4568785783624));
#41094=CARTESIAN_POINT('Ctrl Pts',(21.2219373681819,27.4963832022122,21.636875295208));
#41095=CARTESIAN_POINT('Ctrl Pts',(21.6873545199147,27.7466423667126,21.3192655757679));
#41096=CARTESIAN_POINT('Ctrl Pts',(22.6095407883915,28.1914275999317,20.7266792263566));
#41097=CARTESIAN_POINT('Ctrl Pts',(23.306319546872,28.4721721598032,20.3342063552499));
#41098=CARTESIAN_POINT('Ctrl Pts',(23.97749158379,28.7077527668379,20.0111563083465));
#41099=CARTESIAN_POINT('Ctrl Pts',(24.4307021142574,28.8553793495036,19.8016082531841));
#41100=CARTESIAN_POINT('Ctrl Pts',(24.9871188326861,29.0105626137835,19.5726095610118));
#41101=CARTESIAN_POINT('Ctrl Pts',(25.4329141726813,29.1200357132463,19.4084486444522));
#41102=CARTESIAN_POINT('Ctrl Pts',(25.7643950554696,29.1939083663022,19.2971155191106));
#41103=CARTESIAN_POINT('Ctrl Pts',(26.0382972138574,29.2489718106937,19.2143910494173));
#41104=CARTESIAN_POINT('Ctrl Pts',(26.2284820979132,29.2840172105126,19.1622606931669));
#41105=CARTESIAN_POINT('Ctrl Pts',(26.336649445506,29.3030632173393,19.1341507449285));
#41106=CARTESIAN_POINT('Ctrl Pts',(26.3906225284363,29.3122642693063,19.1206543727096));
#41107=CARTESIAN_POINT('Ctrl Pts',(26.829365411603,29.3859982106888,19.012988583459));
#41108=CARTESIAN_POINT('Ctrl Pts',(27.6560988760142,29.4710985842864,18.8833816200192));
#41109=CARTESIAN_POINT('Ctrl Pts',(28.6249317030316,29.5127595133995,18.8137794716614));
#41110=CARTESIAN_POINT('Ctrl Pts',(29.2119052185271,29.5400636810175,18.7714558506413));
#41111=CARTESIAN_POINT('Ctrl Pts',(29.3512234939538,29.5458124634022,18.7627335234214));
#41112=CARTESIAN_POINT('Ctrl Pts',(29.6502234545149,29.5549926880431,18.7486685476098));
#41113=CARTESIAN_POINT('Ctrl Pts',(30.1759548990663,29.5634265890419,18.7357718416965));
#41114=CARTESIAN_POINT('Ctrl Pts',(31.2785766862299,29.5574021311856,18.744977162533));
#41115=CARTESIAN_POINT('Ctrl Pts',(32.2919610610308,29.5334837411523,18.7821959068193));
#41116=CARTESIAN_POINT('Ctrl Pts',(33.1744263360524,29.5333904072539,18.7823679845324));
#41117=CARTESIAN_POINT('Ctrl Pts',(33.4973548461807,29.5333792377698,18.7823889294252));
#41118=CARTESIAN_POINT('Ctrl Pts',(34.1586526208335,29.5333600113093,18.7824245927187));
#41119=CARTESIAN_POINT('Ctrl Pts',(34.9784715438079,29.533298230803,18.7825395490483));
#41120=CARTESIAN_POINT('Ctrl Pts',(35.9662945600334,29.5332729456427,18.782586552422));
#41121=CARTESIAN_POINT('Ctrl Pts',(37.9401075800398,29.5332379342859,18.7826516826343));
#41122=CARTESIAN_POINT('Ctrl Pts',(39.5833333333333,29.533064777293,18.7829737067337));
#41123=CARTESIAN_POINT('Ctrl Pts',(40.9,29.533064777293,18.7829737067337));
#41124=CARTESIAN_POINT('Origin',(6.9,30.,0.));
#41125=CARTESIAN_POINT('',(6.9,20.5775906479515,21.8303175223207));
#41126=CARTESIAN_POINT('Ctrl Pts',(6.9,7.09789564133157,8.44145532612415));
#41127=CARTESIAN_POINT('Ctrl Pts',(6.9,9.87986401752105,11.09468188726));
#41128=CARTESIAN_POINT('Ctrl Pts',(6.90000000166257,12.753513475675,13.9485622548227));
#41129=CARTESIAN_POINT('Ctrl Pts',(6.90000000166257,16.8843019432417,18.0885125115534));
#41130=CARTESIAN_POINT('Ctrl Pts',(6.9,18.7449692586141,19.9691972794379));
#41131=CARTESIAN_POINT('Ctrl Pts',(6.9,20.5775906479515,21.8303175223207));
#41132=CARTESIAN_POINT('Origin',(6.9,0.,0.));
#41133=CARTESIAN_POINT('Origin',(40.9,9.,0.));
#41134=CARTESIAN_POINT('Ctrl Pts',(40.9,34.4673758792282,1.5));
#41135=CARTESIAN_POINT('Ctrl Pts',(40.9,33.9668810740701,1.5));
#41136=CARTESIAN_POINT('Ctrl Pts',(40.9,33.466386268912,1.5));
#41137=CARTESIAN_POINT('Ctrl Pts',(40.9,32.9658914637539,1.5));
#41138=CARTESIAN_POINT('Ctrl Pts',(30.5,34.9651684126997,-1.56108868151375));
#41139=CARTESIAN_POINT('Ctrl Pts',(30.5,35.,-0.78093292837788));
#41140=CARTESIAN_POINT('Ctrl Pts',(30.5,35.,0.));
#41141=CARTESIAN_POINT('Ctrl Pts',(30.5,35.,35.));
#41142=CARTESIAN_POINT('Ctrl Pts',(30.5,0.,35.));
#41143=CARTESIAN_POINT('Ctrl Pts',(30.5,-35.,35.));
#41144=CARTESIAN_POINT('Ctrl Pts',(30.5,-35.,0.));
#41145=CARTESIAN_POINT('Ctrl Pts',(30.5,-35.,-35.));
#41146=CARTESIAN_POINT('Ctrl Pts',(30.5,0.,-35.));
#41147=CARTESIAN_POINT('Ctrl Pts',(30.5,33.472222479613,-35.));
#41148=CARTESIAN_POINT('Ctrl Pts',(30.5,34.9651684126997,-1.56108868151375));
#41149=CARTESIAN_POINT('Ctrl Pts',(30.3311478274255,34.8898028105656,-1.55772383604587));
#41150=CARTESIAN_POINT('Ctrl Pts',(30.3311478274255,34.924559320191,-0.779249668063534));
#41151=CARTESIAN_POINT('Ctrl Pts',(30.3311478274255,34.924559320191,0.));
#41152=CARTESIAN_POINT('Ctrl Pts',(30.3311478274255,34.924559320191,34.924559320191));
#41153=CARTESIAN_POINT('Ctrl Pts',(30.3311478274255,0.,34.924559320191));
#41154=CARTESIAN_POINT('Ctrl Pts',(30.3311478274255,-34.924559320191,34.924559320191));
#41155=CARTESIAN_POINT('Ctrl Pts',(30.3311478274255,-34.924559320191,0.));
#41156=CARTESIAN_POINT('Ctrl Pts',(30.3311478274255,-34.924559320191,-34.924559320191));
#41157=CARTESIAN_POINT('Ctrl Pts',(30.3311478274255,0.,-34.924559320191));
#41158=CARTESIAN_POINT('Ctrl Pts',(30.3311478274255,33.4000748447964,-34.924559320191));
#41159=CARTESIAN_POINT('Ctrl Pts',(30.3311478274255,34.8898028105656,-1.55772383604587));
#41160=CARTESIAN_POINT('Ctrl Pts',(29.9897712690917,34.7371408974366,-1.55090794481746));
#41161=CARTESIAN_POINT('Ctrl Pts',(29.9897712690917,34.7717453283792,-0.775840025831457));
#41162=CARTESIAN_POINT('Ctrl Pts',(29.9897712690917,34.7717453283792,0.));
#41163=CARTESIAN_POINT('Ctrl Pts',(29.9897712690917,34.7717453283791,34.7717453283791));
#41164=CARTESIAN_POINT('Ctrl Pts',(29.9897712690917,0.,34.7717453283792));
#41165=CARTESIAN_POINT('Ctrl Pts',(29.9897712690917,-34.7717453283791,34.7717453283791));
#41166=CARTESIAN_POINT('Ctrl Pts',(29.9897712690917,-34.7717453283792,0.));
#41167=CARTESIAN_POINT('Ctrl Pts',(29.9897712690917,-34.7717453283791,-34.7717453283791));
#41168=CARTESIAN_POINT('Ctrl Pts',(29.9897712690917,0.,-34.7717453283792));
#41169=CARTESIAN_POINT('Ctrl Pts',(29.9897712690917,33.2539313038843,-34.7717453283791));
#41170=CARTESIAN_POINT('Ctrl Pts',(29.9897712690917,34.7371408974366,-1.55090794481746));
#41171=CARTESIAN_POINT('Ctrl Pts',(29.4666899049319,34.5023553003819,-1.54042548027394));
#41172=CARTESIAN_POINT('Ctrl Pts',(29.4666899049319,34.5367258427036,-0.770596184255043));
#41173=CARTESIAN_POINT('Ctrl Pts',(29.4666899049319,34.5367258427036,0.));
#41174=CARTESIAN_POINT('Ctrl Pts',(29.4666899049319,34.5367258427036,34.5367258427036));
#41175=CARTESIAN_POINT('Ctrl Pts',(29.4666899049319,0.,34.5367258427036));
#41176=CARTESIAN_POINT('Ctrl Pts',(29.4666899049319,-34.5367258427036,34.5367258427036));
#41177=CARTESIAN_POINT('Ctrl Pts',(29.4666899049319,-34.5367258427036,0.));
#41178=CARTESIAN_POINT('Ctrl Pts',(29.4666899049319,-34.5367258427036,-34.5367258427036));
#41179=CARTESIAN_POINT('Ctrl Pts',(29.4666899049319,0.,-34.5367258427036));
#41180=CARTESIAN_POINT('Ctrl Pts',(29.4666899049319,33.0291706035535,-34.5367258427036));
#41181=CARTESIAN_POINT('Ctrl Pts',(29.4666899049319,34.5023553003819,-1.54042548027394));
#41182=CARTESIAN_POINT('Ctrl Pts',(28.7471241621752,34.1776802811774,-1.52592972576568));
#41183=CARTESIAN_POINT('Ctrl Pts',(28.7471241621752,34.21172738887,-0.763344698704455));
#41184=CARTESIAN_POINT('Ctrl Pts',(28.7471241621752,34.21172738887,0.));
#41185=CARTESIAN_POINT('Ctrl Pts',(28.7471241621752,34.2117273888699,34.2117273888699));
#41186=CARTESIAN_POINT('Ctrl Pts',(28.7471241621752,0.,34.21172738887));
#41187=CARTESIAN_POINT('Ctrl Pts',(28.7471241621752,-34.2117273888699,34.2117273888699));
#41188=CARTESIAN_POINT('Ctrl Pts',(28.7471241621752,-34.21172738887,0.));
#41189=CARTESIAN_POINT('Ctrl Pts',(28.7471241621752,-34.2117273888699,-34.2117273888699));
#41190=CARTESIAN_POINT('Ctrl Pts',(28.7471241621752,0.,-34.21172738887));
#41191=CARTESIAN_POINT('Ctrl Pts',(28.7471241621752,32.718358587775,-34.2117273888699));
#41192=CARTESIAN_POINT('Ctrl Pts',(28.7471241621752,34.1776802811774,-1.52592972576568));
#41193=CARTESIAN_POINT('Ctrl Pts',(27.8100958442934,33.7532520886149,-1.50698029472893));
#41194=CARTESIAN_POINT('Ctrl Pts',(27.8100958442934,33.7868763896026,-0.753865266276394));
#41195=CARTESIAN_POINT('Ctrl Pts',(27.8100958442934,33.7868763896026,0.));
#41196=CARTESIAN_POINT('Ctrl Pts',(27.8100958442934,33.7868763896026,33.7868763896026));
#41197=CARTESIAN_POINT('Ctrl Pts',(27.8100958442934,0.,33.7868763896026));
#41198=CARTESIAN_POINT('Ctrl Pts',(27.8100958442934,-33.7868763896026,33.7868763896026));
#41199=CARTESIAN_POINT('Ctrl Pts',(27.8100958442934,-33.7868763896026,0.));
#41200=CARTESIAN_POINT('Ctrl Pts',(27.8100958442934,-33.7868763896026,-33.7868763896026));
#41201=CARTESIAN_POINT('Ctrl Pts',(27.8100958442934,0.,-33.7868763896026));
#41202=CARTESIAN_POINT('Ctrl Pts',(27.8100958442934,32.3120526686846,-33.7868763896026));
#41203=CARTESIAN_POINT('Ctrl Pts',(27.8100958442934,33.7532520886149,-1.50698029472893));
#41204=CARTESIAN_POINT('Ctrl Pts',(26.8343111708818,33.3132226048841,-1.48733431337754));
#41205=CARTESIAN_POINT('Ctrl Pts',(26.8343111708818,33.3464085574791,-0.744037385305066));
#41206=CARTESIAN_POINT('Ctrl Pts',(26.8343111708818,33.3464085574791,0.));
#41207=CARTESIAN_POINT('Ctrl Pts',(26.8343111708818,33.3464085574791,33.3464085574791));
#41208=CARTESIAN_POINT('Ctrl Pts',(26.8343111708818,0.,33.3464085574791));
#41209=CARTESIAN_POINT('Ctrl Pts',(26.8343111708818,-33.3464085574791,33.3464085574791));
#41210=CARTESIAN_POINT('Ctrl Pts',(26.8343111708818,-33.3464085574791,0.));
#41211=CARTESIAN_POINT('Ctrl Pts',(26.8343111708818,-33.3464085574791,-33.3464085574791));
#41212=CARTESIAN_POINT('Ctrl Pts',(26.8343111708818,0.,-33.3464085574791));
#41213=CARTESIAN_POINT('Ctrl Pts',(26.8343111708818,31.8908116037717,-33.3464085574791));
#41214=CARTESIAN_POINT('Ctrl Pts',(26.8343111708818,33.3132226048841,-1.48733431337754));
#41215=CARTESIAN_POINT('Ctrl Pts',(25.8181479469611,32.8638045923198,-1.46726916269953));
#41216=CARTESIAN_POINT('Ctrl Pts',(25.8181479469611,32.8965428438611,-0.733999815330423));
#41217=CARTESIAN_POINT('Ctrl Pts',(25.8181479469611,32.8965428438611,0.));
#41218=CARTESIAN_POINT('Ctrl Pts',(25.8181479469611,32.896542843861,32.896542843861));
#41219=CARTESIAN_POINT('Ctrl Pts',(25.8181479469611,0.,32.8965428438611));
#41220=CARTESIAN_POINT('Ctrl Pts',(25.8181479469611,-32.896542843861,32.896542843861));
#41221=CARTESIAN_POINT('Ctrl Pts',(25.8181479469611,-32.8965428438611,0.));
#41222=CARTESIAN_POINT('Ctrl Pts',(25.8181479469611,-32.896542843861,-32.896542843861));
#41223=CARTESIAN_POINT('Ctrl Pts',(25.8181479469611,0.,-32.8965428438611));
#41224=CARTESIAN_POINT('Ctrl Pts',(25.8181479469611,31.4605828822811,-32.896542843861));
#41225=CARTESIAN_POINT('Ctrl Pts',(25.8181479469611,32.8638045923198,-1.46726916269953));
#41226=CARTESIAN_POINT('Ctrl Pts',(24.7595197917227,32.4162193763075,-1.44728584082667));
#41227=CARTESIAN_POINT('Ctrl Pts',(24.7595197917227,32.4485117525897,-0.724003180127255));
#41228=CARTESIAN_POINT('Ctrl Pts',(24.7595197917227,32.4485117525897,0.));
#41229=CARTESIAN_POINT('Ctrl Pts',(24.7595197917227,32.4485117525897,32.4485117525897));
#41230=CARTESIAN_POINT('Ctrl Pts',(24.7595197917227,0.,32.4485117525897));
#41231=CARTESIAN_POINT('Ctrl Pts',(24.7595197917227,-32.4485117525897,32.4485117525897));
#41232=CARTESIAN_POINT('Ctrl Pts',(24.7595197917227,-32.4485117525897,0.));
#41233=CARTESIAN_POINT('Ctrl Pts',(24.7595197917227,-32.4485117525897,-32.4485117525897));
#41234=CARTESIAN_POINT('Ctrl Pts',(24.7595197917227,0.,-32.4485117525897));
#41235=CARTESIAN_POINT('Ctrl Pts',(24.7595197917227,31.0321087004291,-32.4485117525897));
#41236=CARTESIAN_POINT('Ctrl Pts',(24.7595197917227,32.4162193763075,-1.44728584082667));
#41237=CARTESIAN_POINT('Ctrl Pts',(23.6563574780851,31.9852629652417,-1.42804494464108));
#41238=CARTESIAN_POINT('Ctrl Pts',(23.6563574780851,32.017126031541,-0.714377942572998));
#41239=CARTESIAN_POINT('Ctrl Pts',(23.6563574780851,32.017126031541,0.));
#41240=CARTESIAN_POINT('Ctrl Pts',(23.6563574780851,32.017126031541,32.017126031541));
#41241=CARTESIAN_POINT('Ctrl Pts',(23.6563574780851,0.,32.017126031541));
#41242=CARTESIAN_POINT('Ctrl Pts',(23.6563574780851,-32.017126031541,32.017126031541));
#41243=CARTESIAN_POINT('Ctrl Pts',(23.6563574780851,-32.017126031541,0.));
#41244=CARTESIAN_POINT('Ctrl Pts',(23.6563574780851,-32.017126031541,-32.017126031541));
#41245=CARTESIAN_POINT('Ctrl Pts',(23.6563574780851,0.,-32.017126031541));
#41246=CARTESIAN_POINT('Ctrl Pts',(23.6563574780851,30.6195533053014,-32.017126031541));
#41247=CARTESIAN_POINT('Ctrl Pts',(23.6563574780851,31.9852629652417,-1.42804494464108));
#41248=CARTESIAN_POINT('Ctrl Pts',(22.5073180101405,31.5864702700101,-1.41024006077928));
#41249=CARTESIAN_POINT('Ctrl Pts',(22.5073180101405,31.6179360671638,-0.705471068634138));
#41250=CARTESIAN_POINT('Ctrl Pts',(22.5073180101405,31.6179360671638,0.));
#41251=CARTESIAN_POINT('Ctrl Pts',(22.5073180101405,31.6179360671638,31.6179360671638));
#41252=CARTESIAN_POINT('Ctrl Pts',(22.5073180101405,0.,31.6179360671638));
#41253=CARTESIAN_POINT('Ctrl Pts',(22.5073180101405,-31.6179360671638,31.6179360671638));
#41254=CARTESIAN_POINT('Ctrl Pts',(22.5073180101405,-31.6179360671638,0.));
#41255=CARTESIAN_POINT('Ctrl Pts',(22.5073180101405,-31.6179360671638,-31.6179360671638));
#41256=CARTESIAN_POINT('Ctrl Pts',(22.5073180101405,0.,-31.6179360671638));
#41257=CARTESIAN_POINT('Ctrl Pts',(22.5073180101405,30.237788296751,-31.6179360671638));
#41258=CARTESIAN_POINT('Ctrl Pts',(22.5073180101405,31.5864702700101,-1.41024006077928));
#41259=CARTESIAN_POINT('Ctrl Pts',(21.3125219557939,31.2336232862855,-1.39448651353199));
#41260=CARTESIAN_POINT('Ctrl Pts',(21.3125219557939,31.264737584474,-0.697590373623121));
#41261=CARTESIAN_POINT('Ctrl Pts',(21.3125219557939,31.264737584474,0.));
#41262=CARTESIAN_POINT('Ctrl Pts',(21.3125219557939,31.264737584474,31.264737584474));
#41263=CARTESIAN_POINT('Ctrl Pts',(21.3125219557939,0.,31.264737584474));
#41264=CARTESIAN_POINT('Ctrl Pts',(21.3125219557939,-31.264737584474,31.264737584474));
#41265=CARTESIAN_POINT('Ctrl Pts',(21.3125219557939,-31.264737584474,0.));
#41266=CARTESIAN_POINT('Ctrl Pts',(21.3125219557939,-31.264737584474,-31.264737584474));
#41267=CARTESIAN_POINT('Ctrl Pts',(21.3125219557939,0.,-31.264737584474));
#41268=CARTESIAN_POINT('Ctrl Pts',(21.3125219557939,29.9000072055494,-31.264737584474));
#41269=CARTESIAN_POINT('Ctrl Pts',(21.3125219557939,31.2336232862855,-1.39448651353199));
#41270=CARTESIAN_POINT('Ctrl Pts',(20.0742472323676,30.9363148057487,-1.3812125919422));
#41271=CARTESIAN_POINT('Ctrl Pts',(20.0742472323676,30.9671329312955,-0.690950108671533));
#41272=CARTESIAN_POINT('Ctrl Pts',(20.0742472323676,30.9671329312955,0.));
#41273=CARTESIAN_POINT('Ctrl Pts',(20.0742472323676,30.9671329312955,30.9671329312955));
#41274=CARTESIAN_POINT('Ctrl Pts',(20.0742472323676,0.,30.9671329312955));
#41275=CARTESIAN_POINT('Ctrl Pts',(20.0742472323676,-30.9671329312955,30.9671329312955));
#41276=CARTESIAN_POINT('Ctrl Pts',(20.0742472323676,-30.9671329312955,0.));
#41277=CARTESIAN_POINT('Ctrl Pts',(20.0742472323676,-30.9671329312955,-30.9671329312955));
#41278=CARTESIAN_POINT('Ctrl Pts',(20.0742472323676,0.,-30.9671329312955));
#41279=CARTESIAN_POINT('Ctrl Pts',(20.0742472323676,29.6153932294878,-30.9671329312955));
#41280=CARTESIAN_POINT('Ctrl Pts',(20.0742472323676,30.9363148057487,-1.3812125919422));
#41281=CARTESIAN_POINT('Ctrl Pts',(18.7979917002302,30.6967495040754,-1.37051672808959));
#41282=CARTESIAN_POINT('Ctrl Pts',(18.7979917002302,30.727328979557,-0.685599514321027));
#41283=CARTESIAN_POINT('Ctrl Pts',(18.7979917002302,30.727328979557,0.));
#41284=CARTESIAN_POINT('Ctrl Pts',(18.7979917002302,30.727328979557,30.727328979557));
#41285=CARTESIAN_POINT('Ctrl Pts',(18.7979917002302,0.,30.727328979557));
#41286=CARTESIAN_POINT('Ctrl Pts',(18.7979917002302,-30.727328979557,30.727328979557));
#41287=CARTESIAN_POINT('Ctrl Pts',(18.7979917002302,-30.727328979557,0.));
#41288=CARTESIAN_POINT('Ctrl Pts',(18.7979917002302,-30.727328979557,-30.727328979557));
#41289=CARTESIAN_POINT('Ctrl Pts',(18.7979917002302,0.,-30.727328979557));
#41290=CARTESIAN_POINT('Ctrl Pts',(18.7979917002302,29.3860569087997,-30.727328979557));
#41291=CARTESIAN_POINT('Ctrl Pts',(18.7979917002302,30.6967495040754,-1.37051672808959));
#41292=CARTESIAN_POINT('Ctrl Pts',(17.4917404060759,30.5108523315028,-1.36221698336641));
#41293=CARTESIAN_POINT('Ctrl Pts',(17.4917404060759,30.5412466200144,-0.681447575979395));
#41294=CARTESIAN_POINT('Ctrl Pts',(17.4917404060759,30.5412466200144,0.));
#41295=CARTESIAN_POINT('Ctrl Pts',(17.4917404060759,30.5412466200144,30.5412466200144));
#41296=CARTESIAN_POINT('Ctrl Pts',(17.4917404060759,0.,30.5412466200144));
#41297=CARTESIAN_POINT('Ctrl Pts',(17.4917404060759,-30.5412466200144,30.5412466200144));
#41298=CARTESIAN_POINT('Ctrl Pts',(17.4917404060759,-30.5412466200144,0.));
#41299=CARTESIAN_POINT('Ctrl Pts',(17.4917404060759,-30.5412466200144,-30.5412466200144));
#41300=CARTESIAN_POINT('Ctrl Pts',(17.4917404060759,0.,-30.5412466200144));
#41301=CARTESIAN_POINT('Ctrl Pts',(17.4917404060759,29.2080971905671,-30.5412466200144));
#41302=CARTESIAN_POINT('Ctrl Pts',(17.4917404060759,30.5108523315028,-1.36221698336641));
#41303=CARTESIAN_POINT('Ctrl Pts',(16.1647270995715,30.3706357712668,-1.35595673938413));
#41304=CARTESIAN_POINT('Ctrl Pts',(16.1647270995715,30.4008903789023,-0.678315895682602));
#41305=CARTESIAN_POINT('Ctrl Pts',(16.1647270995715,30.4008903789023,0.));
#41306=CARTESIAN_POINT('Ctrl Pts',(16.1647270995715,30.4008903789023,30.4008903789023));
#41307=CARTESIAN_POINT('Ctrl Pts',(16.1647270995715,0.,30.4008903789023));
#41308=CARTESIAN_POINT('Ctrl Pts',(16.1647270995715,-30.4008903789023,30.4008903789023));
#41309=CARTESIAN_POINT('Ctrl Pts',(16.1647270995715,-30.4008903789023,0.));
#41310=CARTESIAN_POINT('Ctrl Pts',(16.1647270995715,-30.4008903789023,-30.4008903789023));
#41311=CARTESIAN_POINT('Ctrl Pts',(16.1647270995715,0.,-30.4008903789023));
#41312=CARTESIAN_POINT('Ctrl Pts',(16.1647270995715,29.0738676097412,-30.4008903789023));
#41313=CARTESIAN_POINT('Ctrl Pts',(16.1647270995715,30.3706357712668,-1.35595673938413));
#41314=CARTESIAN_POINT('Ctrl Pts',(14.8263876417415,30.2660684364343,-1.35128812515249));
#41315=CARTESIAN_POINT('Ctrl Pts',(14.8263876417415,30.2962188762246,-0.675980426451064));
#41316=CARTESIAN_POINT('Ctrl Pts',(14.8263876417415,30.2962188762246,0.));
#41317=CARTESIAN_POINT('Ctrl Pts',(14.8263876417415,30.2962188762245,30.2962188762245));
#41318=CARTESIAN_POINT('Ctrl Pts',(14.8263876417415,0.,30.2962188762246));
#41319=CARTESIAN_POINT('Ctrl Pts',(14.8263876417415,-30.2962188762245,30.2962188762245));
#41320=CARTESIAN_POINT('Ctrl Pts',(14.8263876417415,-30.2962188762246,0.));
#41321=CARTESIAN_POINT('Ctrl Pts',(14.8263876417415,-30.2962188762245,-30.2962188762245));
#41322=CARTESIAN_POINT('Ctrl Pts',(14.8263876417415,0.,-30.2962188762246));
#41323=CARTESIAN_POINT('Ctrl Pts',(14.8263876417415,28.9737651004582,-30.2962188762245));
#41324=CARTESIAN_POINT('Ctrl Pts',(14.8263876417415,30.2660684364343,-1.35128812515249));
#41325=CARTESIAN_POINT('Ctrl Pts',(13.4853470903953,30.186937862885,-1.34775518513426));
#41326=CARTESIAN_POINT('Ctrl Pts',(13.4853470903953,30.2170094744125,-0.674213077019289));
#41327=CARTESIAN_POINT('Ctrl Pts',(13.4853470903953,30.2170094744125,0.));
#41328=CARTESIAN_POINT('Ctrl Pts',(13.4853470903953,30.2170094744125,30.2170094744125));
#41329=CARTESIAN_POINT('Ctrl Pts',(13.4853470903953,0.,30.2170094744125));
#41330=CARTESIAN_POINT('Ctrl Pts',(13.4853470903953,-30.2170094744125,30.2170094744125));
#41331=CARTESIAN_POINT('Ctrl Pts',(13.4853470903953,-30.2170094744125,0.));
#41332=CARTESIAN_POINT('Ctrl Pts',(13.4853470903953,-30.2170094744125,-30.2170094744125));
#41333=CARTESIAN_POINT('Ctrl Pts',(13.4853470903953,0.,-30.2170094744125));
#41334=CARTESIAN_POINT('Ctrl Pts',(13.4853470903953,28.8980132513174,-30.2170094744125));
#41335=CARTESIAN_POINT('Ctrl Pts',(13.4853470903953,30.186937862885,-1.34775518513426));
#41336=CARTESIAN_POINT('Ctrl Pts',(12.1482076787549,30.1249424647305,-1.34498727870742));
#41337=CARTESIAN_POINT('Ctrl Pts',(12.1482076787549,30.1549523177074,-0.672828434816074));
#41338=CARTESIAN_POINT('Ctrl Pts',(12.1482076787549,30.1549523177074,0.));
#41339=CARTESIAN_POINT('Ctrl Pts',(12.1482076787549,30.1549523177074,30.1549523177074));
#41340=CARTESIAN_POINT('Ctrl Pts',(12.1482076787549,0.,30.1549523177074));
#41341=CARTESIAN_POINT('Ctrl Pts',(12.1482076787549,-30.1549523177074,30.1549523177074));
#41342=CARTESIAN_POINT('Ctrl Pts',(12.1482076787549,-30.1549523177074,0.));
#41343=CARTESIAN_POINT('Ctrl Pts',(12.1482076787549,-30.1549523177074,-30.1549523177074));
#41344=CARTESIAN_POINT('Ctrl Pts',(12.1482076787549,0.,-30.1549523177074));
#41345=CARTESIAN_POINT('Ctrl Pts',(12.1482076787549,28.8386649382978,-30.1549523177074));
#41346=CARTESIAN_POINT('Ctrl Pts',(12.1482076787549,30.1249424647305,-1.34498727870742));
#41347=CARTESIAN_POINT('Ctrl Pts',(10.8190675759626,30.0746904138676,-1.34274367710657));
#41348=CARTESIAN_POINT('Ctrl Pts',(10.8190675759626,30.1046502067769,-0.671706075536286));
#41349=CARTESIAN_POINT('Ctrl Pts',(10.8190675759626,30.1046502067769,0.));
#41350=CARTESIAN_POINT('Ctrl Pts',(10.8190675759626,30.1046502067769,30.1046502067769));
#41351=CARTESIAN_POINT('Ctrl Pts',(10.8190675759626,0.,30.1046502067769));
#41352=CARTESIAN_POINT('Ctrl Pts',(10.8190675759626,-30.1046502067769,30.1046502067769));
#41353=CARTESIAN_POINT('Ctrl Pts',(10.8190675759626,-30.1046502067769,0.));
#41354=CARTESIAN_POINT('Ctrl Pts',(10.8190675759626,-30.1046502067769,-30.1046502067769));
#41355=CARTESIAN_POINT('Ctrl Pts',(10.8190675759626,0.,-30.1046502067769));
#41356=CARTESIAN_POINT('Ctrl Pts',(10.8190675759626,28.7905585540618,-30.1046502067769));
#41357=CARTESIAN_POINT('Ctrl Pts',(10.8190675759626,30.0746904138676,-1.34274367710657));
#41358=CARTESIAN_POINT('Ctrl Pts',(9.50027713254189,30.032840404991,-1.34087520118769));
#41359=CARTESIAN_POINT('Ctrl Pts',(9.50027713254189,30.0627585077754,-0.670771372474115));
#41360=CARTESIAN_POINT('Ctrl Pts',(9.50027713254189,30.0627585077754,0.));
#41361=CARTESIAN_POINT('Ctrl Pts',(9.50027713254189,30.0627585077753,30.0627585077753));
#41362=CARTESIAN_POINT('Ctrl Pts',(9.50027713254189,0.,30.0627585077754));
#41363=CARTESIAN_POINT('Ctrl Pts',(9.5002771325419,-30.0627585077753,30.0627585077753));
#41364=CARTESIAN_POINT('Ctrl Pts',(9.5002771325419,-30.0627585077754,0.));
#41365=CARTESIAN_POINT('Ctrl Pts',(9.5002771325419,-30.0627585077753,-30.0627585077753));
#41366=CARTESIAN_POINT('Ctrl Pts',(9.50027713254189,0.,-30.0627585077754));
#41367=CARTESIAN_POINT('Ctrl Pts',(9.50027713254189,28.750495460661,-30.0627585077753));
#41368=CARTESIAN_POINT('Ctrl Pts',(9.50027713254189,30.032840404991,-1.34087520118769));
#41369=CARTESIAN_POINT('Ctrl Pts',(8.45435372222587,30.0047244129961,-1.33961990745209));
#41370=CARTESIAN_POINT('Ctrl Pts',(8.45435372222587,30.0346145072029,-0.670143413137449));
#41371=CARTESIAN_POINT('Ctrl Pts',(8.45435372222587,30.0346145072029,0.));
#41372=CARTESIAN_POINT('Ctrl Pts',(8.45435372222587,30.0346145072029,30.0346145072029));
#41373=CARTESIAN_POINT('Ctrl Pts',(8.45435372222587,0.,30.0346145072029));
#41374=CARTESIAN_POINT('Ctrl Pts',(8.45435372222587,-30.0346145072029,30.0346145072029));
#41375=CARTESIAN_POINT('Ctrl Pts',(8.45435372222587,-30.0346145072029,0.));
#41376=CARTESIAN_POINT('Ctrl Pts',(8.45435372222587,-30.0346145072029,-30.0346145072029));
#41377=CARTESIAN_POINT('Ctrl Pts',(8.45435372222587,0.,-30.0346145072029));
#41378=CARTESIAN_POINT('Ctrl Pts',(8.45435372222587,28.7235799678431,-30.0346145072029));
#41379=CARTESIAN_POINT('Ctrl Pts',(8.45435372222587,30.0047244129961,-1.33961990745209));
#41380=CARTESIAN_POINT('Ctrl Pts',(7.67514864245731,29.9863740491064,-1.33880061938141));
#41381=CARTESIAN_POINT('Ctrl Pts',(7.67514864245731,30.0162458630552,-0.669733565164174));
#41382=CARTESIAN_POINT('Ctrl Pts',(7.67514864245731,30.0162458630552,0.));
#41383=CARTESIAN_POINT('Ctrl Pts',(7.67514864245731,30.0162458630552,30.0162458630552));
#41384=CARTESIAN_POINT('Ctrl Pts',(7.67514864245731,0.,30.0162458630552));
#41385=CARTESIAN_POINT('Ctrl Pts',(7.67514864245731,-30.0162458630552,30.0162458630552));
#41386=CARTESIAN_POINT('Ctrl Pts',(7.67514864245731,-30.0162458630552,0.));
#41387=CARTESIAN_POINT('Ctrl Pts',(7.67514864245731,-30.0162458630552,-30.0162458630552));
#41388=CARTESIAN_POINT('Ctrl Pts',(7.67514864245731,0.,-30.0162458630552));
#41389=CARTESIAN_POINT('Ctrl Pts',(7.67514864245731,28.7060131294556,-30.0162458630552));
#41390=CARTESIAN_POINT('Ctrl Pts',(7.67514864245731,29.9863740491064,-1.33880061938141));
#41391=CARTESIAN_POINT('Ctrl Pts',(7.15799654185577,29.9753522996976,-1.33830853171149));
#41392=CARTESIAN_POINT('Ctrl Pts',(7.15799654185577,30.0052131340045,-0.669487398838302));
#41393=CARTESIAN_POINT('Ctrl Pts',(7.15799654185577,30.0052131340045,0.));
#41394=CARTESIAN_POINT('Ctrl Pts',(7.15799654185577,30.0052131340045,30.0052131340045));
#41395=CARTESIAN_POINT('Ctrl Pts',(7.15799654185577,0.,30.0052131340045));
#41396=CARTESIAN_POINT('Ctrl Pts',(7.15799654185577,-30.0052131340045,30.0052131340045));
#41397=CARTESIAN_POINT('Ctrl Pts',(7.15799654185577,-30.0052131340045,0.));
#41398=CARTESIAN_POINT('Ctrl Pts',(7.15799654185577,-30.0052131340045,-30.0052131340045));
#41399=CARTESIAN_POINT('Ctrl Pts',(7.15799654185577,0.,-30.0052131340045));
#41400=CARTESIAN_POINT('Ctrl Pts',(7.15799654185577,28.695461987703,-30.0052131340045));
#41401=CARTESIAN_POINT('Ctrl Pts',(7.15799654185577,29.9753522996976,-1.33830853171149));
#41402=CARTESIAN_POINT('Ctrl Pts',(6.9,29.9701443537426,-1.33807601272607));
#41403=CARTESIAN_POINT('Ctrl Pts',(6.9,30.,-0.669371081466754));
#41404=CARTESIAN_POINT('Ctrl Pts',(6.9,30.,0.));
#41405=CARTESIAN_POINT('Ctrl Pts',(6.9,30.,30.));
#41406=CARTESIAN_POINT('Ctrl Pts',(6.9,0.,30.));
#41407=CARTESIAN_POINT('Ctrl Pts',(6.9,-30.,30.));
#41408=CARTESIAN_POINT('Ctrl Pts',(6.9,-30.,0.));
#41409=CARTESIAN_POINT('Ctrl Pts',(6.9,-30.,-30.));
#41410=CARTESIAN_POINT('Ctrl Pts',(6.9,0.,-30.));
#41411=CARTESIAN_POINT('Ctrl Pts',(6.9,28.6904764110968,-30.));
#41412=CARTESIAN_POINT('Ctrl Pts',(6.9,29.9701443537426,-1.33807601272607));
#41413=CARTESIAN_POINT('Ctrl Pts',(6.9,20.5775906479515,21.8303175223207));
#41414=CARTESIAN_POINT('Ctrl Pts',(7.85773098116326,22.0288565043892,20.4889265372405));
#41415=CARTESIAN_POINT('Ctrl Pts',(8.88781981167334,23.3171626725998,19.0414114324084));
#41416=CARTESIAN_POINT('Ctrl Pts',(10.5914578196776,25.1150390010341,16.6247285680552));
#41417=CARTESIAN_POINT('Ctrl Pts',(11.2365058953701,25.7254166302984,15.703976734769));
#41418=CARTESIAN_POINT('Ctrl Pts',(12.0558885382926,26.3926147460599,14.5853792872662));
#41419=CARTESIAN_POINT('Ctrl Pts',(12.1875764958397,26.4963665374952,14.4076425286694));
#41420=CARTESIAN_POINT('Ctrl Pts',(13.194901830313,27.2691057169114,13.0552778456719));
#41421=CARTESIAN_POINT('Ctrl Pts',(14.2258982134098,27.991732600527,11.6381637544796));
#41422=CARTESIAN_POINT('Ctrl Pts',(18.2616480823244,29.9350198014187,6.95587410790868));
#41423=CARTESIAN_POINT('Ctrl Pts',(21.0496416709525,30.7693084982877,4.29983295736294));
#41424=CARTESIAN_POINT('Ctrl Pts',(25.8000196361138,32.8040277065106,1.93741001991749));
#41425=CARTESIAN_POINT('Ctrl Pts',(26.8976561124457,33.3305524688301,1.74039351523169));
#41426=CARTESIAN_POINT('Ctrl Pts',(28.0045908801237,33.8378020212277,1.58669630450145));
#41427=CARTESIAN_POINT('Ctrl Pts',(28.5235971652406,34.0754855762016,1.54532623843659));
#41428=CARTESIAN_POINT('Ctrl Pts',(29.0834839543824,34.3307100593381,1.49828854871271));
#41429=CARTESIAN_POINT('Ctrl Pts',(29.1146288039499,34.3449058451715,1.49562082188434));
#41430=CARTESIAN_POINT('Ctrl Pts',(29.5949306848436,34.5637016811193,1.45589225448014));
#41431=CARTESIAN_POINT('Ctrl Pts',(30.0492939924726,34.7685410859787,1.44682754698748));
#41432=CARTESIAN_POINT('Ctrl Pts',(30.5,34.9699609326822,1.44976976333442));
#41433=CARTESIAN_POINT('Ctrl Pts',(6.45331003273164,6.83943894028999,8.65286216739172));
#41434=CARTESIAN_POINT('Ctrl Pts',(7.20830533428676,7.28712780725476,8.29622318255583));
#41435=CARTESIAN_POINT('Ctrl Pts',(7.99924796920644,7.69991572864563,7.91909532230128));
#41436=CARTESIAN_POINT('Ctrl Pts',(9.76163642871393,8.50127829248443,7.07028372020711));
#41437=CARTESIAN_POINT('Ctrl Pts',(10.7316626231511,8.87935281282541,6.57783879792861));
#41438=CARTESIAN_POINT('Ctrl Pts',(12.6608237755523,9.49392179513702,5.67260683532433));
#41439=CARTESIAN_POINT('Ctrl Pts',(13.6376935580087,9.74868549844379,5.20677839827646));
#41440=CARTESIAN_POINT('Ctrl Pts',(14.8683081444882,10.0072371758851,4.68571756497415));
#41441=CARTESIAN_POINT('Ctrl Pts',(15.814981546047,10.1933420307132,4.28615487511135));
#41442=CARTESIAN_POINT('Ctrl Pts',(16.7774761024725,10.3417484740057,3.90183726466219));
#41443=CARTESIAN_POINT('Ctrl Pts',(18.4438470226174,10.5575964922698,3.30966453460613));
#41444=CARTESIAN_POINT('Ctrl Pts',(19.4166260537866,10.6478897990577,2.98271399009538));
#41445=CARTESIAN_POINT('Ctrl Pts',(20.8624415465505,10.7552000633453,2.58750630277728));
#41446=CARTESIAN_POINT('Ctrl Pts',(21.8144010701942,10.8125125199158,2.34040933534242));
#41447=CARTESIAN_POINT('Ctrl Pts',(22.7817704456172,10.8543372932886,2.13286375196526));
#41448=CARTESIAN_POINT('Ctrl Pts',(23.3296603631192,10.875372496282,2.03163991938105));
#41449=CARTESIAN_POINT('Ctrl Pts',(23.4469280425865,10.8796667005721,2.01025391532514));
#41450=CARTESIAN_POINT('Ctrl Pts',(23.681028881355,10.8878000542955,1.96865773783261));
#41451=CARTESIAN_POINT('Ctrl Pts',(24.09412141496,10.9009272596694,1.89824222375213));
#41452=CARTESIAN_POINT('Ctrl Pts',(24.6899984645713,10.9167861221077,1.80575737992302));
#41453=CARTESIAN_POINT('Ctrl Pts',(25.4117472347962,10.9320835607492,1.7102381255629));
#41454=CARTESIAN_POINT('Ctrl Pts',(25.8944359856995,10.9403877892626,1.65861072075243));
#41455=CARTESIAN_POINT('Ctrl Pts',(26.36694263196,10.947884133746,1.61476081138875));
#41456=CARTESIAN_POINT('Ctrl Pts',(27.2927605647397,10.9593568588011,1.54499465236547));
#41457=CARTESIAN_POINT('Ctrl Pts',(28.2852623623167,10.9616475307267,1.51981821556059));
#41458=CARTESIAN_POINT('Ctrl Pts',(29.2044123671999,10.9652006081482,1.49506529955051));
#41459=CARTESIAN_POINT('Ctrl Pts',(29.5205491106405,10.9661656603817,1.48868169066078));
#41460=CARTESIAN_POINT('Ctrl Pts',(30.1691034959588,10.9670510696507,1.48263221141176));
#41461=CARTESIAN_POINT('Ctrl Pts',(31.3134334344235,10.9664912432219,1.4864605825931));
#41462=CARTESIAN_POINT('Ctrl Pts',(32.3203424123248,10.9645690748214,1.49997009105207));
#41463=CARTESIAN_POINT('Ctrl Pts',(33.1675465322483,10.9645713457497,1.49998069520819));
#41464=CARTESIAN_POINT('Ctrl Pts',(33.4947519346946,10.9645717110255,1.49998093738942));
#41465=CARTESIAN_POINT('Ctrl Pts',(34.1540738134337,10.9645721532421,1.49998231763443));
#41466=CARTESIAN_POINT('Ctrl Pts',(34.8114511007501,10.9645737361772,1.49998580542901));
#41467=CARTESIAN_POINT('Ctrl Pts',(35.7991041415375,10.9645740230236,1.49998654292928));
#41468=CARTESIAN_POINT('Ctrl Pts',(37.7734954411133,10.9645758157225,1.49999064614178));
#41469=CARTESIAN_POINT('Ctrl Pts',(39.5833333333333,10.9645797934319,1.5));
#41470=CARTESIAN_POINT('Ctrl Pts',(40.9,10.9645797934319,1.5));
#41471=CARTESIAN_POINT('Ctrl Pts',(6.63336813585096,9.34202246898051,11.0008793183436));
#41472=CARTESIAN_POINT('Ctrl Pts',(7.389696336477,9.9106502389341,10.5126404716241));
#41473=CARTESIAN_POINT('Ctrl Pts',(8.18028889045472,10.4323217834721,10.0000669136624));
#41474=CARTESIAN_POINT('Ctrl Pts',(9.94159575574686,11.439192222287,8.85353468669098));
#41475=CARTESIAN_POINT('Ctrl Pts',(10.9109419422817,11.9102705993651,8.192010210379));
#41476=CARTESIAN_POINT('Ctrl Pts',(12.8335218625484,12.6683977976686,6.98387303125938));
#41477=CARTESIAN_POINT('Ctrl Pts',(13.8091851210584,12.9798296118147,6.36343771133683));
#41478=CARTESIAN_POINT('Ctrl Pts',(15.031077490038,13.2915570052696,5.67481209887734));
#41479=CARTESIAN_POINT('Ctrl Pts',(15.9749773134882,13.5160612446606,5.14536755152679));
#41480=CARTESIAN_POINT('Ctrl Pts',(16.930312943506,13.6911692618856,4.63930769376668));
#41481=CARTESIAN_POINT('Ctrl Pts',(18.5806860927911,13.9445588072222,3.86175938608204));
#41482=CARTESIAN_POINT('Ctrl Pts',(19.5487190419049,14.0476485209229,3.43185831734754));
#41483=CARTESIAN_POINT('Ctrl Pts',(20.9744115808251,14.1690991173096,2.9163969121787));
#41484=CARTESIAN_POINT('Ctrl Pts',(21.9189583606343,14.2328177454446,2.59280390983885));
#41485=CARTESIAN_POINT('Ctrl Pts',(22.8721113115926,14.2778669302764,2.3228415983607));
#41486=CARTESIAN_POINT('Ctrl Pts',(23.4111206282026,14.3007194584988,2.19132406241537));
#41487=CARTESIAN_POINT('Ctrl Pts',(23.5272640974126,14.3053783578069,2.16340494095902));
#41488=CARTESIAN_POINT('Ctrl Pts',(23.7586042074431,14.3141392731536,2.10919630050473));
#41489=CARTESIAN_POINT('Ctrl Pts',(24.1668594457501,14.328140925801,2.01743796447886));
#41490=CARTESIAN_POINT('Ctrl Pts',(24.7549510427123,14.3447231768684,1.89707890772752));
#41491=CARTESIAN_POINT('Ctrl Pts',(25.4661619742722,14.3604369110457,1.77296928480103));
#41492=CARTESIAN_POINT('Ctrl Pts',(25.9407936523078,14.368979185674,1.70601541029858));
#41493=CARTESIAN_POINT('Ctrl Pts',(26.4047985025954,14.3768131131951,1.64920950338613));
#41494=CARTESIAN_POINT('Ctrl Pts',(27.3109130873599,14.3886741790608,1.55899536298033));
#41495=CARTESIAN_POINT('Ctrl Pts',(28.2968127703991,14.3906288624531,1.52586579774316));
#41496=CARTESIAN_POINT('Ctrl Pts',(29.216365869052,14.3942351181099,1.49337715415662));
#41497=CARTESIAN_POINT('Ctrl Pts',(29.5273677411776,14.3952146919186,1.48510498656914));
#41498=CARTESIAN_POINT('Ctrl Pts',(30.1704748351474,14.3961140069303,1.47720108681952));
#41499=CARTESIAN_POINT('Ctrl Pts',(31.3076822233502,14.3955480332033,1.48219673215098));
#41500=CARTESIAN_POINT('Ctrl Pts',(32.3162781940782,14.3936026936296,1.49994928257769));
#41501=CARTESIAN_POINT('Ctrl Pts',(33.1684720644414,14.3936066618447,1.49996698297726));
#41502=CARTESIAN_POINT('Ctrl Pts',(33.4950641584123,14.3936073001223,1.49996744488464));
#41503=CARTESIAN_POINT('Ctrl Pts',(34.1546952525894,14.3936080728485,1.49996977575843));
#41504=CARTESIAN_POINT('Ctrl Pts',(34.8117737683131,14.3936108388537,1.49997575137036));
#41505=CARTESIAN_POINT('Ctrl Pts',(35.7994747102213,14.3936113400866,1.49997700611746));
#41506=CARTESIAN_POINT('Ctrl Pts',(37.7736758948775,14.3936144726314,1.499984023326));
#41507=CARTESIAN_POINT('Ctrl Pts',(39.5833333333333,14.3936214232436,1.5));
#41508=CARTESIAN_POINT('Ctrl Pts',(40.9,14.3936214232436,1.5));
#41509=CARTESIAN_POINT('Ctrl Pts',(6.84643360079894,15.1545575883324,16.506001665025));
#41510=CARTESIAN_POINT('Ctrl Pts',(7.61273218496773,16.0159127642118,15.7040687667121));
#41511=CARTESIAN_POINT('Ctrl Pts',(8.4126771054426,16.7980113101253,14.8690272591124));
#41512=CARTESIAN_POINT('Ctrl Pts',(10.1879439641556,18.2945580567154,13.0164926384402));
#41513=CARTESIAN_POINT('Ctrl Pts',(11.1642689802371,18.9856854823124,11.9550510602025));
#41514=CARTESIAN_POINT('Ctrl Pts',(13.1036036726265,20.0861315198186,10.022452207883));
#41515=CARTESIAN_POINT('Ctrl Pts',(14.0826172183607,20.5290484396468,9.03879487952599));
#41516=CARTESIAN_POINT('Ctrl Pts',(15.3089235211201,20.9656035967448,7.95158583831005));
#41517=CARTESIAN_POINT('Ctrl Pts',(16.2536562498252,21.2790692641439,7.11690983506512));
#41518=CARTESIAN_POINT('Ctrl Pts',(17.2094234535122,21.5156901422925,6.32372298857519));
#41519=CARTESIAN_POINT('Ctrl Pts',(18.8492103514784,21.8541559656566,5.11428176787037));
#41520=CARTESIAN_POINT('Ctrl Pts',(19.8132789859545,21.9855288021883,4.44555314736777));
#41521=CARTESIAN_POINT('Ctrl Pts',(21.2105274130181,22.1378650260473,3.65671370764621));
#41522=CARTESIAN_POINT('Ctrl Pts',(22.1435262947163,22.2155499994864,3.15760868632203));
#41523=CARTESIAN_POINT('Ctrl Pts',(23.0712019161588,22.2672966100822,2.74759983583373));
#41524=CARTESIAN_POINT('Ctrl Pts',(23.5926643019344,22.2940508574533,2.54861011877022));
#41525=CARTESIAN_POINT('Ctrl Pts',(23.7065967589743,22.2995097248259,2.50584172092972));
#41526=CARTESIAN_POINT('Ctrl Pts',(23.9324349207312,22.3096292230889,2.42316535684891));
#41527=CARTESIAN_POINT('Ctrl Pts',(24.3308966188193,22.3255066595415,2.28324508302848));
#41528=CARTESIAN_POINT('Ctrl Pts',(24.9027307486986,22.3435822260676,2.1003169439008));
#41529=CARTESIAN_POINT('Ctrl Pts',(25.59120580204,22.3601136597684,1.91242242103882));
#41530=CARTESIAN_POINT('Ctrl Pts',(26.047911616652,22.3691489781575,1.81155274261714));
#41531=CARTESIAN_POINT('Ctrl Pts',(26.4927766852064,22.3777261422413,1.72621142470535));
#41532=CARTESIAN_POINT('Ctrl Pts',(27.3538144829413,22.3904445374984,1.59133675559695));
#41533=CARTESIAN_POINT('Ctrl Pts',(28.3239440765631,22.3916143651132,1.5395372712982));
#41534=CARTESIAN_POINT('Ctrl Pts',(29.2444087331683,22.3953365265065,1.48903537353034));
#41535=CARTESIAN_POINT('Ctrl Pts',(29.5434413064007,22.3963491807022,1.4765958448865));
#41536=CARTESIAN_POINT('Ctrl Pts',(30.1738228526165,22.3972793088217,1.46445321166482));
#41537=CARTESIAN_POINT('Ctrl Pts',(31.2943937060125,22.3966964278384,1.47211763918551));
#41538=CARTESIAN_POINT('Ctrl Pts',(32.3068807810286,22.3946917099991,1.49983279134389));
#41539=CARTESIAN_POINT('Ctrl Pts',(33.1706991860565,22.3946974029307,1.49988437406509));
#41540=CARTESIAN_POINT('Ctrl Pts',(33.4958573126071,22.3946983171246,1.49988713027318));
#41541=CARTESIAN_POINT('Ctrl Pts',(34.1562063695875,22.394699425001,1.49989458266055));
#41542=CARTESIAN_POINT('Ctrl Pts',(34.8125750960604,22.3947033892012,1.49991575825725));
#41543=CARTESIAN_POINT('Ctrl Pts',(35.8003855127834,22.3947041076693,1.49991999484083));
#41544=CARTESIAN_POINT('Ctrl Pts',(37.7741287617182,22.3947085973461,1.49994455667286));
#41545=CARTESIAN_POINT('Ctrl Pts',(39.5833333333333,22.394718559471,1.5));
#41546=CARTESIAN_POINT('Ctrl Pts',(40.9,22.394718559471,1.5));
#41547=CARTESIAN_POINT('Ctrl Pts',(6.90857970435318,20.8698550272217,22.1068727166734));
#41548=CARTESIAN_POINT('Ctrl Pts',(7.67983757144493,22.0336104135999,20.991774688754));
#41549=CARTESIAN_POINT('Ctrl Pts',(8.48444928201915,23.0860770683301,19.8332461961107));
#41550=CARTESIAN_POINT('Ctrl Pts',(10.2687663769551,25.0905346149111,17.2709888357559));
#41551=CARTESIAN_POINT('Ctrl Pts',(11.2490111943913,26.0108786577409,15.8072894822424));
#41552=CARTESIAN_POINT('Ctrl Pts',(13.2067599054631,27.4745835397,13.1283892637642));
#41553=CARTESIAN_POINT('Ctrl Pts',(14.1887708824686,28.0545611646472,11.7775873547894));
#41554=CARTESIAN_POINT('Ctrl Pts',(15.4301927253883,28.6258871350548,10.2708149751555));
#41555=CARTESIAN_POINT('Ctrl Pts',(16.3793034376203,29.0320485193235,9.12509880827949));
#41556=CARTESIAN_POINT('Ctrl Pts',(17.3459407209745,29.3355313348089,8.02905385413649));
#41557=CARTESIAN_POINT('Ctrl Pts',(19.00167863971,29.7645301224029,6.36442803225957));
#41558=CARTESIAN_POINT('Ctrl Pts',(19.9708024570657,29.9249381814105,5.44984750618437));
#41559=CARTESIAN_POINT('Ctrl Pts',(21.372654162153,30.1088343166973,4.37628680649795));
#41560=CARTESIAN_POINT('Ctrl Pts',(22.3059973273548,30.2002109026536,3.69883691082952));
#41561=CARTESIAN_POINT('Ctrl Pts',(23.2278577930092,30.2581794306252,3.14826448808765));
#41562=CARTESIAN_POINT('Ctrl Pts',(23.7415516356669,30.2885183156938,2.88362049576677));
#41563=CARTESIAN_POINT('Ctrl Pts',(23.8544946510477,30.2947200062411,2.82623659223919));
#41564=CARTESIAN_POINT('Ctrl Pts',(24.0777274663495,30.3060802342176,2.71573667925149));
#41565=CARTESIAN_POINT('Ctrl Pts',(24.4711727956184,30.3236351372296,2.52895535356894));
#41566=CARTESIAN_POINT('Ctrl Pts',(25.0334457271173,30.3429441514162,2.2860141148269));
#41567=CARTESIAN_POINT('Ctrl Pts',(25.7062144884658,30.3600503901634,2.03835403030805));
#41568=CARTESIAN_POINT('Ctrl Pts',(26.1486936133437,30.3694723684121,1.90670660027131));
#41569=CARTESIAN_POINT('Ctrl Pts',(26.5774366289029,30.378713979902,1.79594947825405));
#41570=CARTESIAN_POINT('Ctrl Pts',(27.3975110717082,30.3921981334468,1.62272694197857));
#41571=CARTESIAN_POINT('Ctrl Pts',(28.3508259392473,30.3926064111245,1.55227638555954));
#41572=CARTESIAN_POINT('Ctrl Pts',(29.2723062856311,30.3964396342324,1.48380439950633));
#41573=CARTESIAN_POINT('Ctrl Pts',(29.5594622066962,30.3974855836748,1.46775103384065));
#41574=CARTESIAN_POINT('Ctrl Pts',(30.1771168569175,30.3984465770314,1.45157152773897));
#41575=CARTESIAN_POINT('Ctrl Pts',(31.281071177308,30.3978463334885,1.46177125475314));
#41576=CARTESIAN_POINT('Ctrl Pts',(32.2974559939611,30.395781840626,1.49958178095819));
#41577=CARTESIAN_POINT('Ctrl Pts',(33.1729044426912,30.3957890263381,1.49970257782127));
#41578=CARTESIAN_POINT('Ctrl Pts',(33.4966295876143,30.395790177722,1.4997109685702));
#41579=CARTESIAN_POINT('Ctrl Pts',(34.1576977268015,30.3957915749199,1.4997293265115));
#41580=CARTESIAN_POINT('Ctrl Pts',(34.8133607699291,30.3957965718591,1.4997840805116));
#41581=CARTESIAN_POINT('Ctrl Pts',(35.8012813983217,30.3957974776822,1.49979479816103));
#41582=CARTESIAN_POINT('Ctrl Pts',(37.7745713511015,30.395803137258,1.49985796376524));
#41583=CARTESIAN_POINT('Ctrl Pts',(39.5833333333333,30.3958156956984,1.5));
#41584=CARTESIAN_POINT('Ctrl Pts',(40.9,30.3958156956984,1.5));
#41585=CARTESIAN_POINT('Ctrl Pts',(6.93528330520032,24.1234099037007,25.3195110382618));
#41586=CARTESIAN_POINT('Ctrl Pts',(7.70864561497005,25.4600205488393,24.0266258397084));
#41587=CARTESIAN_POINT('Ctrl Pts',(8.51531156164572,26.6675788409113,22.6840056101462));
#41588=CARTESIAN_POINT('Ctrl Pts',(10.3033767345502,28.9634999585434,19.7178334181139));
#41589=CARTESIAN_POINT('Ctrl Pts',(11.2853975328499,30.0157138764656,18.024966824446));
#41590=CARTESIAN_POINT('Ctrl Pts',(13.2504656206425,31.6887121402305,14.920608256729));
#41591=CARTESIAN_POINT('Ctrl Pts',(14.2338911783743,32.3479754973602,13.3603265157411));
#41592=CARTESIAN_POINT('Ctrl Pts',(15.4814489736579,32.9977120049687,11.6128587845954));
#41593=CARTESIAN_POINT('Ctrl Pts',(16.4323633322631,33.457701559807,10.2891584164032));
#41594=CARTESIAN_POINT('Ctrl Pts',(17.4036580739674,33.8004278805126,9.0188416170732));
#41595=CARTESIAN_POINT('Ctrl Pts',(19.0672887678301,34.2828730898378,7.09001985912387));
#41596=CARTESIAN_POINT('Ctrl Pts',(20.039114991915,34.4604737318841,6.03348815316115));
#41597=CARTESIAN_POINT('Ctrl Pts',(21.446277848711,34.6632929668278,4.79159535501521));
#41598=CARTESIAN_POINT('Ctrl Pts',(22.3811728101676,34.7627792680184,4.01020122074906));
#41599=CARTESIAN_POINT('Ctrl Pts',(23.303259548489,34.8244923190151,3.37635643636734));
#41600=CARTESIAN_POINT('Ctrl Pts',(23.8149974822579,34.8569118346704,3.07312481135071));
#41601=CARTESIAN_POINT('Ctrl Pts',(23.9276845297169,34.8635414236982,3.00725282827679));
#41602=CARTESIAN_POINT('Ctrl Pts',(24.1501932465706,34.8756163196439,2.88055633977634));
#41603=CARTESIAN_POINT('Ctrl Pts',(24.542110623408,34.8941314993691,2.6665697947521));
#41604=CARTESIAN_POINT('Ctrl Pts',(25.1010166003944,34.9141289755488,2.38896069563576));
#41605=CARTESIAN_POINT('Ctrl Pts',(25.7673676623319,34.9315307898226,2.10719515267297));
#41606=CARTESIAN_POINT('Ctrl Pts',(26.2032614590241,34.9411502230498,1.95837832513289));
#41607=CARTESIAN_POINT('Ctrl Pts',(26.6241220770204,34.9507523611203,1.83365744353246));
#41608=CARTESIAN_POINT('Ctrl Pts',(27.4227877709102,34.9646463474544,1.64008822157602));
#41609=CARTESIAN_POINT('Ctrl Pts',(28.3660425122777,34.9646178111256,1.55920845841383));
#41610=CARTESIAN_POINT('Ctrl Pts',(29.288154079426,34.9685099768711,1.48047877405357));
#41611=CARTESIAN_POINT('Ctrl Pts',(29.5685743108623,34.9695745039167,1.46254110097229));
#41612=CARTESIAN_POINT('Ctrl Pts',(30.178956622871,34.9705522790041,1.44412472938078));
#41613=CARTESIAN_POINT('Ctrl Pts',(31.2734286330481,34.9699406754865,1.45573528147979));
#41614=CARTESIAN_POINT('Ctrl Pts',(32.2920480078112,34.9678391394654,1.49937027232429));
#41615=CARTESIAN_POINT('Ctrl Pts',(33.1741467941407,34.9678459524318,1.4995472544355));
#41616=CARTESIAN_POINT('Ctrl Pts',(33.4970538821706,34.9678470414556,1.49956078207587));
#41617=CARTESIAN_POINT('Ctrl Pts',(34.1585338443543,34.967848364944,1.49958825610694));
#41618=CARTESIAN_POINT('Ctrl Pts',(34.8137969787744,34.9678530956497,1.49967176946748));
#41619=CARTESIAN_POINT('Ctrl Pts',(35.8017811867035,34.9678539534014,1.49968797974804));
#41620=CARTESIAN_POINT('Ctrl Pts',(37.7748158892396,34.9678593117154,1.49978412416472));
#41621=CARTESIAN_POINT('Ctrl Pts',(39.5833333333333,34.967871202114,1.5));
#41622=CARTESIAN_POINT('Ctrl Pts',(40.9,34.967871202114,1.5));
#41623=CARTESIAN_POINT('Origin',(0.3,5.20850103220104,-6.86619553270279));
#41624=CARTESIAN_POINT('',(0.6,5.35130101070365,-7.13002912825054));
#41625=CARTESIAN_POINT('',(0.,5.06570105369843,-6.60236193715504));
#41626=CARTESIAN_POINT('Origin',(0.,-8.88651760185943,-2.38113521494319));
#41627=CARTESIAN_POINT('',(6.5,-8.84627910967765,-0.918184763087449));
#41628=CARTESIAN_POINT('Origin',(0.,-6.50538238691624,-6.50538238691624));
#41629=CARTESIAN_POINT('',(6.5,-5.88386150345169,-7.65368850791103));
#41630=CARTESIAN_POINT('Origin',(0.,-2.38113521494319,-8.88651760185943));
#41631=CARTESIAN_POINT('',(6.5,0.492874024900538,-10.6529279712533));
#41632=CARTESIAN_POINT('Origin',(0.,2.38113521494319,-8.88651760185943));
#41633=CARTESIAN_POINT('',(6.5,6.56519030397928,-9.00160015149379));
#41634=CARTESIAN_POINT('Origin',(0.,6.50538238691624,-6.50538238691624));
#41635=CARTESIAN_POINT('',(6.5,9.60513338590479,-4.82764163104316));
#41636=CARTESIAN_POINT('Origin',(0.,8.88651760185943,-2.38113521494319));
#41637=CARTESIAN_POINT('',(6.5,9.70736730835527,-1.04558506087479));
#41638=CARTESIAN_POINT('Origin',(0.,0.,0.));
#41639=CARTESIAN_POINT('Origin',(0.,-6.50538238691624,6.50538238691624));
#41640=CARTESIAN_POINT('',(6.5,-1.09746863550251,9.43241662545793));
#41641=CARTESIAN_POINT('Origin',(0.,-2.38113521494319,8.88651760185943));
#41642=CARTESIAN_POINT('',(6.5,4.42649419509641,8.69927356878582));
#41643=CARTESIAN_POINT('Origin',(0.,2.38113521494319,8.88651760185943));
#41644=CARTESIAN_POINT('',(6.5,7.49114572377286,5.7458263941306));
#41645=CARTESIAN_POINT('Origin',(0.,6.50538238691624,6.50538238691624));
#41646=CARTESIAN_POINT('',(6.5,8.3761967530494,3.04891351349626));
#41647=CARTESIAN_POINT('Origin',(0.,8.88651760185943,2.38113521494319));
#41648=CARTESIAN_POINT('',(6.5,8.85459461060197,1.22051134579542));
#41649=CARTESIAN_POINT('Origin',(0.,-8.88651760185943,2.38113521494319));
#41650=CARTESIAN_POINT('',(6.5,-6.69138705702868,5.95268663799753));
#41651=CARTESIAN_POINT('Origin',(6.5,11.,0.));
#41652=CARTESIAN_POINT('Origin',(41.85,0.,0.));
#41653=CARTESIAN_POINT('',(42.2,-12.,-1.46957615897682E-15));
#41654=CARTESIAN_POINT('Origin',(42.2,0.,0.));
#41655=CARTESIAN_POINT('',(41.85,-13.,-1.59204083889156E-15));
#41656=CARTESIAN_POINT('Origin',(42.6,0.,0.));
#41657=CARTESIAN_POINT('',(42.6,-11.3,-1.38385088303651E-15));
#41658=CARTESIAN_POINT('Origin',(44.2,0.,0.));
#41659=CARTESIAN_POINT('',(44.2,-9.,-1.10218211923262E-15));
#41660=CARTESIAN_POINT('Origin',(55.3,0.,0.));
#41661=CARTESIAN_POINT('',(55.5,-8.79999999999999,-1.07768918324967E-15));
#41662=CARTESIAN_POINT('Origin',(55.5,0.,0.));
#41663=CARTESIAN_POINT('',(55.3,-9.,-1.10218211923262E-15));
#41664=CARTESIAN_POINT('Origin',(55.5,7.2,0.));
#41665=CARTESIAN_POINT('',(55.5,-7.19999999999999,-8.81745695386093E-16));
#41666=CARTESIAN_POINT('Origin',(55.5,0.,0.));
#41667=CARTESIAN_POINT('Origin',(56.,0.,0.));
#41668=CARTESIAN_POINT('',(56.5,-6.2,-7.59281015471359E-16));
#41669=CARTESIAN_POINT('Origin',(56.5,0.,0.));
#41670=CARTESIAN_POINT('',(56.,-6.7,-8.20513355428727E-16));
#41671=CARTESIAN_POINT('Origin',(56.75,0.,0.));
#41672=CARTESIAN_POINT('',(57.,-5.50000000000001,-6.73555739531045E-16));
#41673=CARTESIAN_POINT('Origin',(57.,0.,0.));
#41674=CARTESIAN_POINT('',(56.75,-5.85,-7.16418377501202E-16));
#41675=CARTESIAN_POINT('Origin',(85.35,0.,0.));
#41676=CARTESIAN_POINT('',(113.7,-5.5,-6.73555739531044E-16));
#41677=CARTESIAN_POINT('Origin',(113.7,0.,0.));
#41678=CARTESIAN_POINT('',(85.35,-5.5,-6.73555739531044E-16));
#41679=CARTESIAN_POINT('Origin',(113.85,0.,0.));
#41680=CARTESIAN_POINT('',(114.,-5.2,-6.36816335556624E-16));
#41681=CARTESIAN_POINT('Origin',(114.,0.,0.));
#41682=CARTESIAN_POINT('',(113.85,-5.35,-6.55186037543834E-16));
#41683=CARTESIAN_POINT('Origin',(114.,3.3,0.));
#41684=CARTESIAN_POINT('',(114.,-3.3,-4.04133443718627E-16));
#41685=CARTESIAN_POINT('Origin',(114.,0.,0.));
#41686=CARTESIAN_POINT('Origin',(114.3,0.,0.));
#41687=CARTESIAN_POINT('',(114.6,-3.3,-4.04133443718627E-16));
#41688=CARTESIAN_POINT('Origin',(114.6,0.,0.));
#41689=CARTESIAN_POINT('',(114.3,-3.3,-4.04133443718627E-16));
#41690=CARTESIAN_POINT('Origin',(114.7,0.,0.));
#41691=CARTESIAN_POINT('',(114.8,-3.5,-4.28626379701574E-16));
#41692=CARTESIAN_POINT('Origin',(114.8,0.,0.));
#41693=CARTESIAN_POINT('',(114.7,-3.4,-4.163799117101E-16));
#41694=CARTESIAN_POINT('Origin',(135.1,0.,0.));
#41695=CARTESIAN_POINT('',(155.4,-3.5,-4.28626379701574E-16));
#41696=CARTESIAN_POINT('Origin',(155.4,0.,0.));
#41697=CARTESIAN_POINT('',(135.1,-3.5,-4.28626379701574E-16));
#41698=CARTESIAN_POINT('Origin',(155.5,0.,0.));
#41699=CARTESIAN_POINT('',(155.6,-2.9,-3.55147571752733E-16));
#41700=CARTESIAN_POINT('Origin',(155.6,0.,0.));
#41701=CARTESIAN_POINT('',(155.5,-3.2,-3.91886975727153E-16));
#41702=CARTESIAN_POINT('Origin',(156.15,0.,0.));
#41703=CARTESIAN_POINT('',(156.7,-2.9,-3.55147571752732E-16));
#41704=CARTESIAN_POINT('Origin',(156.7,0.,0.));
#41705=CARTESIAN_POINT('',(156.15,-2.9,-3.55147571752732E-16));
#41706=CARTESIAN_POINT('Origin',(156.85,0.,0.));
#41707=CARTESIAN_POINT('',(156.85,-3.2,-3.91886975727153E-16));
#41708=CARTESIAN_POINT('Origin',(165.,0.,0.));
#41709=CARTESIAN_POINT('Origin',(173.058,0.,0.));
#41710=CARTESIAN_POINT('Origin',(173.25,0.,0.));
#41711=CARTESIAN_POINT('',(173.5,-3.00000000000001,-3.67394039744207E-16));
#41712=CARTESIAN_POINT('Origin',(173.5,0.,0.));
#41713=CARTESIAN_POINT('',(173.25,-3.25,-3.9801020972289E-16));
#41714=CARTESIAN_POINT('Origin',(173.5,0.,0.));
#60343=UNCERTAINTY_MEASURE_WITH_UNIT(LENGTH_MEASURE(0.01),#60366,
'DISTANCE_ACCURACY_VALUE',
'Maximum model space distance between geometric entities at asserted c
onnectivities');
#60353=UNCERTAINTY_MEASURE_WITH_UNIT(LENGTH_MEASURE(0.01),#60366,
'DISTANCE_ACCURACY_VALUE',
'Maximum model space distance between geometric entities at asserted c
onnectivities');
#60355=(
GEOMETRIC_REPRESENTATION_CONTEXT(3)
GLOBAL_UNCERTAINTY_ASSIGNED_CONTEXT((#60343))
GLOBAL_UNIT_ASSIGNED_CONTEXT((#60366,#60368,#60369))
REPRESENTATION_CONTEXT('','3D')
);
#60365=(
GEOMETRIC_REPRESENTATION_CONTEXT(3)
GLOBAL_UNCERTAINTY_ASSIGNED_CONTEXT((#60353))
GLOBAL_UNIT_ASSIGNED_CONTEXT((#60366,#60368,#60369))
REPRESENTATION_CONTEXT('','3D')
);
#60366=(
LENGTH_UNIT()
NAMED_UNIT(*)
SI_UNIT(.MILLI.,.METRE.)
);
#60368=(
NAMED_UNIT(*)
PLANE_ANGLE_UNIT()
SI_UNIT($,.RADIAN.)
);
#60369=(
NAMED_UNIT(*)
SI_UNIT($,.STERADIAN.)
SOLID_ANGLE_UNIT()
);
#60371=SHAPE_DEFINITION_REPRESENTATION(#60382,#60407);
#60382=PRODUCT_DEFINITION_SHAPE('',$,#60419);
#60407=SHAPE_REPRESENTATION('',(#18419),#60355);
#60417=PRODUCT_DEFINITION_CONTEXT('part definition',#60452,'design');
#60419=PRODUCT_DEFINITION('2026-10-25-00-06-14-899',
'01_Turbine_Wheel_and_Shaft_HX35_60x70_12B',#60430,#60417);
#60430=PRODUCT_DEFINITION_FORMATION('',$,#60455);
#60452=APPLICATION_CONTEXT(
'Core Data for Automotive Mechanical Design Process');
#60453=PRODUCT_CONTEXT('part definition',#60452,'mechanical');
#60455=PRODUCT('2026-10-25-00-06-14-899',
'01_Turbine_Wheel_and_Shaft_HX35_60x70_12B',$,(#60453));
#60521=COLOUR_RGB('Grey',0.48,0.52,0.57);
#60522=FILL_AREA_STYLE_COLOUR('',#60521);
#60523=FILL_AREA_STYLE('',(#60522));
#60524=SURFACE_STYLE_FILL_AREA(#60523);
#60525=SURFACE_SIDE_STYLE('',(#60524));
#60526=SURFACE_STYLE_USAGE(.BOTH.,#60525);
#60527=PRESENTATION_STYLE_ASSIGNMENT((#60526));
ENDSEC;
END-ISO-10303-21;
